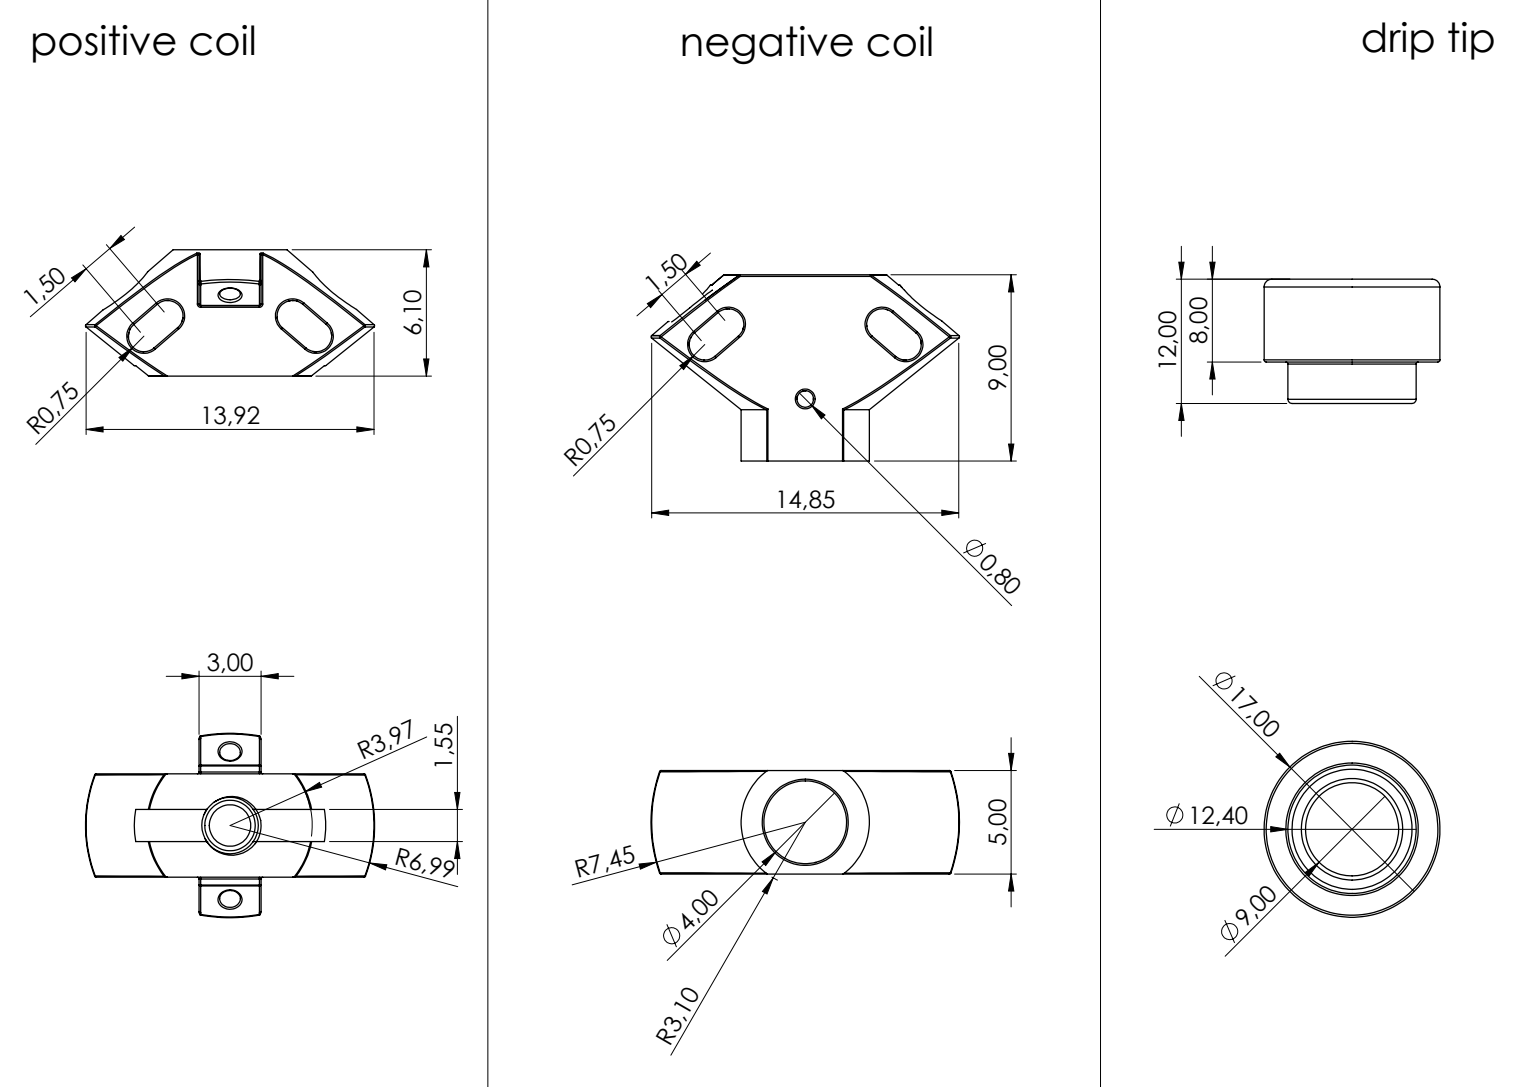
ISO-10303-21;
HEADER;
FILE_DESCRIPTION (('STEP AP214'),
    '1' );
FILE_NAME ('negative coil.step',
    '2026-10-05T20:10:51',
    ( '' ),
    ( '' ),
    'SwSTEP 2.0',
    'SolidWorks 2020',
    '' );
FILE_SCHEMA (( 'AUTOMOTIVE_DESIGN' ));
ENDSEC;

DATA;
#7=CARTESIAN_POINT ( 'NONE',  ( -7.144220599758281054, 7.299621885998258897, 0.7998128361456341429 ) ) ;
#9=CARTESIAN_POINT ( 'NONE',  ( 6.873057527484919937, 6.983264968346048818, 0.7998128361456352531 ) ) ;
#14=CARTESIAN_POINT ( 'NONE',  ( -4.828112100242303306, 4.805421336470338645, -0.7216878364870338292 ) ) ;
#18=CARTESIAN_POINT ( 'NONE',  ( 1.833030277982334422, 2.531131934864056632, -2.500000000000000444 ) ) ;
#23=CARTESIAN_POINT ( 'NONE',  ( -0.4770184558378520734, 2.994739774722604331, -1.942553401570029203 ) ) ;
#37=EDGE_LOOP ( 'NONE', ( #180346, #201044, #89611 ) ) ;
#40=CARTESIAN_POINT ( 'NONE',  ( 4.719646871332936477, 8.520355426614829142, -0.7216878364870357165 ) ) ;
#44=VERTEX_POINT ( 'NONE', #43221 ) ;
#53=CARTESIAN_POINT ( 'NONE',  ( -3.797692425603673705, 6.484372692295976570, 1.082531754730549967 ) ) ;
#55=CARTESIAN_POINT ( 'NONE',  ( 6.710359684120930091, 6.793450817754725257, 0.7998128361456352531 ) ) ;
#59=CARTESIAN_POINT ( 'NONE',  ( -4.167152111353897403, 5.955039778036558040, 1.599625672291270506 ) ) ;
#70=LINE ( 'NONE', #134411, #196122 ) ;
#72=CARTESIAN_POINT ( 'NONE',  ( 6.658462837642789012, 9.821938173008357253, 1.082531754730549078 ) ) ;
#83=ORIENTED_EDGE ( 'NONE', *, *, #112082, .F. ) ;
#101=CARTESIAN_POINT ( 'NONE',  ( 4.553559489343365740, 6.405848385690952718, -1.599625672291269396 ) ) ;
#107=CARTESIAN_POINT ( 'NONE',  ( -5.600926855776882540, 8.588146194164741232, -1.082531754730549967 ) ) ;
#108=DIRECTION ( 'NONE',  ( 0.000000000000000000, 0.000000000000000000, -1.000000000000000000 ) ) ;
#113=CARTESIAN_POINT ( 'NONE',  ( -4.911796789900812144, 8.952456364851418158, 0.7998128361456291469 ) ) ;
#119=ORIENTED_EDGE ( 'NONE', *, *, #79643, .F. ) ;
#122=CARTESIAN_POINT ( 'NONE',  ( -5.956828388357799042, 8.042995434541133193, 1.599625672291263179 ) ) ;
#125=CARTESIAN_POINT ( 'NONE',  ( 5.720439131930858956, 7.397432110343761025, 1.315134405782365956 ) ) ;
#128=CARTESIAN_POINT ( 'NONE',  ( 2.969872605471105320, 6.605953636083950364, 7.500000000000000000 ) ) ;
#130=CARTESIAN_POINT ( 'NONE',  ( 5.833751235630055376, 10.02806988486892514, 0.7998128361456331437 ) ) ;
#137=ADVANCED_FACE ( 'NONE', ( #75695 ), #126301, .T. ) ;
#139=CARTESIAN_POINT ( 'NONE',  ( -4.817943484809863008, 6.714296380401858499, 1.599625672291263179 ) ) ;
#143=CARTESIAN_POINT ( 'NONE',  ( -5.586841817283045408, 8.675676665875643678, 1.199719254218454489 ) ) ;
#147=CARTESIAN_POINT ( 'NONE',  ( 7.038091138825468107, 8.344099429118761790, -1.082531754730548412 ) ) ;
#149=CARTESIAN_POINT ( 'NONE',  ( -7.390603132780803719, 7.794994207765291172, -0.7216878364870338292 ) ) ;
#155=CARTESIAN_POINT ( 'NONE',  ( 4.667750024854814050, 8.667735138964429709, -0.7998128361456381397 ) ) ;
#169=CARTESIAN_POINT ( 'NONE',  ( 6.425920342564602983, 6.885296541689900351, -0.7293792964763821107 ) ) ;
#182=ORIENTED_EDGE ( 'NONE', *, *, #184994, .T. ) ;
#184=CARTESIAN_POINT ( 'NONE',  ( 4.649081266440608928, 8.305916344280937835, -0.4560373724170601606 ) ) ;
#196=CARTESIAN_POINT ( 'NONE',  ( -5.495582220874787538, 7.482514367559947033, -1.250084184017367539 ) ) ;
#210=DIRECTION ( 'NONE',  ( 0.000000000000000000, 0.000000000000000000, 1.000000000000000000 ) ) ;
#214=CARTESIAN_POINT ( 'NONE',  ( -3.644109427023046521, 7.473487774827342278, 0.000000000000000000 ) ) ;
#228=CARTESIAN_POINT ( 'NONE',  ( 4.505052181490820651, 8.477920988373101707, -0.7998128361456381397 ) ) ;
#229=CARTESIAN_POINT ( 'NONE',  ( -7.015401035077363900, 6.062865449010541141, 2.437084766375292144 ) ) ;
#231=CARTESIAN_POINT ( 'NONE',  ( 5.790741006368192778, 8.809596036521288198, -1.082531754730548412 ) ) ;
#247=CARTESIAN_POINT ( 'NONE',  ( -6.771371375382467583, 6.864631124226471037, -0.7998128361456362523 ) ) ;
#248=CARTESIAN_POINT ( 'NONE',  ( 4.146814880933355596, 5.931313009212638931, 1.599625672291261402 ) ) ;
#257=CARTESIAN_POINT ( 'NONE',  ( -6.563028877466991595, 9.814561569423593923, 1.199719254218452935 ) ) ;
#258=CARTESIAN_POINT ( 'NONE',  ( 6.099189001301251523, 8.209082816308541197, 1.599625672291268286 ) ) ;
#260=CARTESIAN_POINT ( 'NONE',  ( -6.387350227218078658, 6.552219065260997510, -2.500000000001207923 ) ) ;
#265=CARTESIAN_POINT ( 'NONE',  ( 5.391302360089590628, 6.318882837306503575, -1.199719254218452047 ) ) ;
#266=AXIS2_PLACEMENT_3D ( 'NONE', #151063, #68698, #100160 ) ;
#271=CARTESIAN_POINT ( 'NONE',  ( -6.579637281422358264, 6.781222396613637571, 0.3437121870633503828 ) ) ;
#281=CARTESIAN_POINT ( 'NONE',  ( -7.391130018105325661, 8.652015104991543026, -1.199719254218452047 ) ) ;
#310=CARTESIAN_POINT ( 'NONE',  ( 6.249382461256315580, 6.255644057745969988, -0.7998128361456481317 ) ) ;
#330=CARTESIAN_POINT ( 'NONE',  ( 4.797606254389322089, 6.690569611577942943, 1.599625672291268286 ) ) ;
#331=CARTESIAN_POINT ( 'NONE',  ( -3.363831509966363598, 5.978201624052440266, -1.082531754730548412 ) ) ;
#356=CARTESIAN_POINT ( 'NONE',  ( -6.791708605802965870, 6.888357893050385705, -0.7998128361456362523 ) ) ;
#358=CARTESIAN_POINT ( 'NONE',  ( 5.194182247366861738, 9.073980031987776584, 0.7216878364870317197 ) ) ;
#363=CARTESIAN_POINT ( 'NONE',  ( -5.336015975430226099, 8.383046517047350932, -1.199719254218453823 ) ) ;
#367=CARTESIAN_POINT ( 'NONE',  ( 2.915646864528636417, 6.623614785250545367, 0.2169541561525832329 ) ) ;
#371=CARTESIAN_POINT ( 'NONE',  ( -6.343235766347277149, 8.493804042195527870, -1.599625672291271394 ) ) ;
#378=CARTESIAN_POINT ( 'NONE',  ( 2.905190055078214595, 6.611415174225076186, 0.7998128361456271485 ) ) ;
#381=EDGE_CURVE ( 'NONE', #182271, #52415, #178195, .T. ) ;
#384=CARTESIAN_POINT ( 'NONE',  ( -4.610654757099099221, 7.536791762327691657, 1.199719254218452935 ) ) ;
#388=CARTESIAN_POINT ( 'NONE',  ( -6.834718835064852449, 8.106831741398025315, 1.082531754730549078 ) ) ;
#390=CARTESIAN_POINT ( 'NONE',  ( -7.227905289416804102, 8.565549271475310533, -1.082531754730549967 ) ) ;
#391=CARTESIAN_POINT ( 'NONE',  ( 7.201315867513990554, 8.430565262634994284, -1.199719254218452047 ) ) ;
#392=EDGE_CURVE ( 'NONE', #179985, #120674, #60482, .T. ) ;
#393=CARTESIAN_POINT ( 'NONE',  ( -4.977251789548269301, 4.979417640660637190, 0.7216878364870257245 ) ) ;
#395=CARTESIAN_POINT ( 'NONE',  ( -4.787437639401290745, 6.678706227425192488, 0.000000000000000000 ) ) ;
#411=CARTESIAN_POINT ( 'NONE',  ( -1.886825320689270225, 2.480000000000016858, -2.459652456995881753 ) ) ;
#412=CARTESIAN_POINT ( 'NONE',  ( 6.218145995260431214, 7.027935176161393294, 1.016989286988238206 ) ) ;
#433=CARTESIAN_POINT ( 'NONE',  ( 5.647444738788365726, 7.344714329438926548, -1.230740020431456028 ) ) ;
#436=B_SPLINE_CURVE_WITH_KNOTS ( 'NONE', 3,
 ( #78019, #42351, #109537, #112728, #74835, #144144, #160344, #111660 ),
 .UNSPECIFIED., .F., .F.,
 ( 4, 2, 2, 4 ),
 ( 0.0006312381939941720749, 0.001000335483781913384, 0.001184884128675783984, 0.001369432773569654585 ),
 .UNSPECIFIED. ) ;
#448=CARTESIAN_POINT ( 'NONE',  ( 6.339319342841494453, 9.553567112360518365, -1.199719254218452047 ) ) ;
#451=CARTESIAN_POINT ( 'NONE',  ( -5.492988512192097161, 6.437516681426083132, 1.199719254218452935 ) ) ;
#465=CARTESIAN_POINT ( 'NONE',  ( 3.898851692381625877, 6.706354853490643642, -1.199719254218452047 ) ) ;
#467=CARTESIAN_POINT ( 'NONE',  ( 5.332099551924443404, 9.442809587212341427, 0.000000000000000000 ) ) ;
#474=CARTESIAN_POINT ( 'NONE',  ( -6.902509602688821744, 8.185920970292658083, -1.082531754730549967 ) ) ;
#475=EDGE_LOOP ( 'NONE', ( #184370, #199799, #47164, #11058, #211319, #194077, #40319, #83, #128481 ) ) ;
#480=CARTESIAN_POINT ( 'NONE',  ( 6.176621499477501054, 9.363752961769195693, -1.199719254218452047 ) ) ;
#493=CARTESIAN_POINT ( 'NONE',  ( -5.722950238744243023, 7.770137593325314285, 1.443375672974058777 ) ) ;
#494=CARTESIAN_POINT ( 'NONE',  ( 5.722950238744211937, 5.849399164722627553, 0.7216878364870328300 ) ) ;
#500=DIRECTION ( 'NONE',  ( 0.000000000000000000, 0.000000000000000000, -1.000000000000000000 ) ) ;
#504=CARTESIAN_POINT ( 'NONE',  ( -4.604929450496978660, 5.401447776115099408, -1.199719254218453823 ) ) ;
#505=CARTESIAN_POINT ( 'NONE',  ( -6.455090533882201775, 8.624301270986276080, -1.443375672974066548 ) ) ;
#509=CARTESIAN_POINT ( 'NONE',  ( 4.543390873910903238, 7.354354215321133204, 1.082531754730548412 ) ) ;
#512=VERTEX_POINT ( 'NONE', #98341 ) ;
#526=CARTESIAN_POINT ( 'NONE',  ( -3.793249116773374396, 7.647484079536056356, 0.7998128361456352531 ) ) ;
#539=CARTESIAN_POINT ( 'NONE',  ( 5.063044020060520900, 4.871582543017558109, 0.7998128361456352531 ) ) ;
#543=ORIENTED_EDGE ( 'NONE', *, *, #68702, .T. ) ;
#578=CARTESIAN_POINT ( 'NONE',  ( 3.770576118376296471, 7.413106214832098750, 0.7216878364870257245 ) ) ;
#584=CARTESIAN_POINT ( 'NONE',  ( 3.702785349863636277, 7.334016984900627811, -0.7216878364870338292 ) ) ;
#597=CARTESIAN_POINT ( 'NONE',  ( -5.550083779947821760, 7.568460058062819407, -1.599625672291271394 ) ) ;
#603=B_SPLINE_CURVE_WITH_KNOTS ( 'NONE', 3,
 ( #59694, #174549, #207007, #60764, #12005, #143131 ),
 .UNSPECIFIED., .F., .F.,
 ( 4, 2, 4 ),
 ( 4.610090873601661862E-18, 9.933499788398740429E-05, 0.0001986699957679714476 ),
 .UNSPECIFIED. ) ;
#606=CARTESIAN_POINT ( 'NONE',  ( 6.556249800660121529, 9.806652646482286073, 1.199719254218452047 ) ) ;
#612=CARTESIAN_POINT ( 'NONE',  ( -6.749980374757255319, 8.968339418673846097, 1.599625672291269396 ) ) ;
#618=CARTESIAN_POINT ( 'NONE',  ( -6.617788377246204945, 6.893376992974917350, -0.7216878364870338292 ) ) ;
#622=CARTESIAN_POINT ( 'NONE',  ( -6.720001414228860881, 7.869031733802326123, -1.199719254218452047 ) ) ;
#627=AXIS2_PLACEMENT_3D ( 'NONE', #201676, #53323, #188656 ) ;
#646=CARTESIAN_POINT ( 'NONE',  ( -7.228432174741334038, 8.462200954400218578, -1.199719254218452047 ) ) ;
#647=CARTESIAN_POINT ( 'NONE',  ( 4.543917759235442944, 5.330267469643351852, 1.199719254218452935 ) ) ;
#649=CARTESIAN_POINT ( 'NONE',  ( -5.387385936583832802, 7.378645907471495846, -1.599625672291271394 ) ) ;
#676=CARTESIAN_POINT ( 'NONE',  ( -6.583366107887490770, 9.838288338247510367, 1.199719254218452935 ) ) ;
#696=DIRECTION ( 'NONE',  ( 0.000000000000000000, 0.000000000000000000, 1.000000000000000000 ) ) ;
#705=CARTESIAN_POINT ( 'NONE',  ( 3.413620815590684199, 7.204584394822967752, 0.7998128361456281477 ) ) ;
#717=CARTESIAN_POINT ( 'NONE',  ( 4.763071791759735163, 8.170823326046956936, 0.7639991172946744014 ) ) ;
#720=CARTESIAN_POINT ( 'NONE',  ( 4.848976215542928792, 5.686169002002086970, 1.199719254218452047 ) ) ;
#725=CARTESIAN_POINT ( 'NONE',  ( -5.448397627845328550, 7.449826213943242514, 1.599625672291263179 ) ) ;
#737=CARTESIAN_POINT ( 'NONE',  ( 6.590672070018850803, 7.822110515511036866, -1.082531754730548412 ) ) ;
#740=CARTESIAN_POINT ( 'NONE',  ( -5.822300622425855110, 5.757381912443740646, 0.7998128361456281477 ) ) ;
#751=CARTESIAN_POINT ( 'NONE',  ( 4.041212305325117882, 6.872442235258051646, -1.199719254218448494 ) ) ;
#752=CARTESIAN_POINT ( 'NONE',  ( 4.248501033035879004, 6.049946853332221153, -1.599625672291273171 ) ) ;
#758=VERTEX_POINT ( 'NONE', #154712 ) ;
#770=CARTESIAN_POINT ( 'NONE',  ( -5.570361349191150779, 5.866663122702686195, 0.5491554309224304653 ) ) ;
#774=CARTESIAN_POINT ( 'NONE',  ( 0.000000000000000000, 0.000000000000000000, 0.000000000000000000 ) ) ;
#776=CARTESIAN_POINT ( 'NONE',  ( 6.481679955784983349, 9.719654494127929922, -1.199719254218452047 ) ) ;
#783=CARTESIAN_POINT ( 'NONE',  ( 6.204791576909545192, 7.267953590263130259, -1.199719254218452047 ) ) ;
#790=CARTESIAN_POINT ( 'NONE',  ( 3.757017964762656703, 7.397288368949487491, -1.734723475976807094E-15 ) ) ;
#793=CARTESIAN_POINT ( 'NONE',  ( 5.709392085130549077, 9.675058176045386205, 0.000000000000000000 ) ) ;
#805=CARTESIAN_POINT ( 'NONE',  ( -6.292392690518209264, 8.434487120394948079, -1.443375672974066548 ) ) ;
#824=VERTEX_POINT ( 'NONE', #187194 ) ;
#825=ADVANCED_FACE ( 'NONE', ( #183991 ), #39943, .T. ) ;
#846=CARTESIAN_POINT ( 'NONE',  ( 6.964048179274811012, 8.153752959689313684, 1.199719254218452047 ) ) ;
#848=CARTESIAN_POINT ( 'NONE',  ( 6.225128807330042591, 7.291680359087043151, -1.199719254218452047 ) ) ;
#862=CARTESIAN_POINT ( 'NONE',  ( -5.483346782084204563, 5.361935765378481378, 0.000000000000000000 ) ) ;
#864=CARTESIAN_POINT ( 'NONE',  ( 6.360183458142179447, 6.592837920686898556, -0.7216878364870458196 ) ) ;
#874=CARTESIAN_POINT ( 'NONE',  ( -5.496904935697871863, 5.377753611261092637, 0.7998128361456281477 ) ) ;
#880=CARTESIAN_POINT ( 'NONE',  ( -7.105881907338169157, 8.423188659050232729, -1.082531754730549967 ) ) ;
#882=CARTESIAN_POINT ( 'NONE',  ( -5.478903473698268023, 5.564677938835638216, -0.7216878364870338292 ) ) ;
#908=CARTESIAN_POINT ( 'NONE',  ( -5.517242166118370150, 5.401480380085008193, 0.7998128361456281477 ) ) ;
#920=CARTESIAN_POINT ( 'NONE',  ( -5.476171693740270463, 7.594609835490887306, -1.347918582746489902 ) ) ;
#941=CARTESIAN_POINT ( 'NONE',  ( 7.062871678076271920, 7.204714810702593120, -0.7998128361456341429 ) ) ;
#961=EDGE_CURVE ( 'NONE', #137116, #194727, #203846, .T. ) ;
#964=CARTESIAN_POINT ( 'NONE',  ( 5.155843554946782703, 9.237177590738404831, -0.7998128361456481317 ) ) ;
#965=CARTESIAN_POINT ( 'NONE',  ( 6.249382461256315580, 6.255644057745969988, -0.7998128361456481317 ) ) ;
#967=CARTESIAN_POINT ( 'NONE',  ( 4.716257332707354699, 6.595662536282280719, -1.599625672291269396 ) ) ;
#978=FACE_OUTER_BOUND ( 'NONE', #59802, .T. ) ;
#979=CARTESIAN_POINT ( 'NONE',  ( 5.819104682239041537, 7.212836251160942957, -1.171789181936284896 ) ) ;
#981=CARTESIAN_POINT ( 'NONE',  ( -6.414416072596849538, 7.616478518518682073, -1.082531754730549967 ) ) ;
#982=CARTESIAN_POINT ( 'NONE',  ( 3.757017964762656703, 7.397288368949487491, -1.734723475976807094E-15 ) ) ;
#1007=CARTESIAN_POINT ( 'NONE',  ( 5.529746549527311039, 7.544733289238903851, -1.599625672291281386 ) ) ;
#1008=CARTESIAN_POINT ( 'NONE',  ( 3.549202351727371862, 7.362762853649070571, -0.7998128361456362523 ) ) ;
#1015=CARTESIAN_POINT ( 'NONE',  ( -6.966220764712169000, 6.002124920821316323, -2.420000000000000373 ) ) ;
#1024=DIRECTION ( 'NONE',  ( -1.000000000000000000, 0.000000000000000000, 0.000000000000000000 ) ) ;
#1027=CARTESIAN_POINT ( 'NONE',  ( -5.030511086842778923, 7.205508557346677279, -1.253558018337496582 ) ) ;
#1033=FACE_OUTER_BOUND ( 'NONE', #150305, .T. ) ;
#1038=CARTESIAN_POINT ( 'NONE',  ( 7.679767667498067496, 7.924426798361372093, 0.000000000000000000 ) ) ;
#1042=CARTESIAN_POINT ( 'NONE',  ( -6.466610638350029916, 6.780223854948245865, 0.3187201834274414058 ) ) ;
#1043=CARTESIAN_POINT ( 'NONE',  ( 7.225569521440261767, 7.394528961293920233, -0.7998128361456341429 ) ) ;
#1077=CARTESIAN_POINT ( 'NONE',  ( -6.794571259104023930, 7.956029886156682274, 1.199719254218452047 ) ) ;
#1079=CARTESIAN_POINT ( 'NONE',  ( 7.686546744304875389, 7.932335721302671949, 0.7998128361456291469 ) ) ;
#1094=CARTESIAN_POINT ( 'NONE',  ( 0.001041342783940506700, 2.586899276670884262, -2.002406093249768926 ) ) ;
#1100=EDGE_CURVE ( 'NONE', #39859, #170847, #133352, .T. ) ;
#1104=CARTESIAN_POINT ( 'NONE',  ( 5.643937085038755797, 9.806620042512378177, -0.7998128361456481317 ) ) ;
#1113=CARTESIAN_POINT ( 'NONE',  ( 6.129694847154206983, 8.244672969803623630, -1.443375672974078761 ) ) ;
#1126=CARTESIAN_POINT ( 'NONE',  ( -4.258669648468323743, 6.061810238003387141, 1.443375672974065660 ) ) ;
#1128=CARTESIAN_POINT ( 'NONE',  ( 6.384963997392946844, 6.413822516572072807, 0.7998128361456352531 ) ) ;
#1133=CARTESIAN_POINT ( 'NONE',  ( -5.191846479390389568, 5.021852078902356631, 0.7998128361456281477 ) ) ;
#1137=( BOUNDED_CURVE ( )  B_SPLINE_CURVE ( 2, ( #18392, #113862, #32530, #15194, #48792, #82334, #130120 ),
 .UNSPECIFIED., .F., .T. ) 
 B_SPLINE_CURVE_WITH_KNOTS ( ( 3, 2, 2, 3 ),
 ( 0.3749999999999998890, 0.3833333333333333592, 0.3916666666666668295, 0.4000000000000002998 ),
 .UNSPECIFIED. ) 
 CURVE ( )  GEOMETRIC_REPRESENTATION_ITEM ( )  RATIONAL_B_SPLINE_CURVE ( ( 1.000000000000001776, 0.8660254037844369313, 1.000000000000000000, 0.8660254037844387076, 1.000000000000000000, 0.8660254037844342667, 1.000000000000004441 ) ) 
 REPRESENTATION_ITEM ( '' )  );
#1178=CARTESIAN_POINT ( 'NONE',  ( 3.217027588192558074, 6.975225629525113824, -1.734723475976807094E-15 ) ) ;
#1180=CARTESIAN_POINT ( 'NONE',  ( -5.472651281771599763, 6.413789912602166687, 1.199719254218452935 ) ) ;
#1184=CARTESIAN_POINT ( 'NONE',  ( -6.251718229232857915, 7.426664367927358512, -1.082531754730549967 ) ) ;
#1189=CARTESIAN_POINT ( 'NONE',  ( -6.505933609711270549, 8.683618192786854095, -1.599625672291271394 ) ) ;
#1197=CARTESIAN_POINT ( 'NONE',  ( -6.200875153403786477, 8.327716660428123419, -1.599625672291271394 ) ) ;
#1200=CARTESIAN_POINT ( 'NONE',  ( 5.098657496608274720, 7.938328561423579011, 1.202842226815619142 ) ) ;
#1205=CARTESIAN_POINT ( 'NONE',  ( 5.345657705538078730, 9.458627433094950021, 0.7998128361456331437 ) ) ;
#1211=DIRECTION ( 'NONE',  ( 0.000000000000000000, 0.000000000000000000, 1.000000000000000000 ) ) ;
#1212=CARTESIAN_POINT ( 'NONE',  ( -3.983063267364693960, 7.868933921892603323, -0.7998128361456481317 ) ) ;
#1216=CARTESIAN_POINT ( 'NONE',  ( -5.749539660647037032, 8.865490816466966351, 1.199719254218454489 ) ) ;
#1223=CARTESIAN_POINT ( 'NONE',  ( -7.878696662872776812, 8.364436659539265406, -0.7216878364870338292 ) ) ;
#1229=CARTESIAN_POINT ( 'NONE',  ( 6.717138760927786834, 6.801359740696030443, -0.7998128361456481317 ) ) ;
#1243=CARTESIAN_POINT ( 'NONE',  ( 5.763319317650291040, 7.363698819737331647, -1.304181885133362195 ) ) ;
#1274=CARTESIAN_POINT ( 'NONE',  ( -5.386282318077409315, 7.574627448853999745, -1.244059264865501557 ) ) ;
#1291=CARTESIAN_POINT ( 'NONE',  ( -4.980641328173854632, 6.904110530993182948, 1.599625672291263179 ) ) ;
#1304=CARTESIAN_POINT ( 'NONE',  ( 6.866278450678116485, 6.975356045404744521, 0.000000000000000000 ) ) ;
#1307=CARTESIAN_POINT ( 'NONE',  ( 5.763624699140868834, 7.817591130454727200, -1.443375672974078761 ) ) ;
#1313=AXIS2_PLACEMENT_3D ( 'NONE', #163918, #211566, #65305 ) ;
#1323=CARTESIAN_POINT ( 'NONE',  ( -5.692444392891315097, 7.734547439830227411, -1.599625672291271394 ) ) ;
#1324=CARTESIAN_POINT ( 'NONE',  ( 6.703580607314123085, 6.785541894813420072, 0.000000000000000000 ) ) ;
#1333=CARTESIAN_POINT ( 'NONE',  ( -5.887983850084758330, 10.09134126839936840, 0.7998128361456291469 ) ) ;
#1334=CARTESIAN_POINT ( 'NONE',  ( 5.996449078994045223, 10.21788403546024782, 0.7998128361456331437 ) ) ;
#1336=DIRECTION ( 'NONE',  ( 0.7592566023653004592, -0.6507913734559639396, 0.000000000000000000 ) ) ;
#1340=CARTESIAN_POINT ( 'NONE',  ( 0.000000000000000000, 9.999999999999998224, -2.000000000000000000 ) ) ;
#1341=CARTESIAN_POINT ( 'NONE',  ( 3.718679271898170491, 7.560485927181699317, 0.7998128361456271485 ) ) ;
#1346=CARTESIAN_POINT ( 'NONE',  ( -6.458928793950097891, 6.861006557743732692, 0.6885227102202008398 ) ) ;
#1355=CARTESIAN_POINT ( 'NONE',  ( -4.516274566683622815, 5.401980094953223066, 1.082531754730549078 ) ) ;
#1408=CARTESIAN_POINT ( 'NONE',  ( 4.716257332707354699, 6.595662536282280719, -1.599625672291269396 ) ) ;
#1409=CARTESIAN_POINT ( 'NONE',  ( -4.394251184604987870, 5.259619482528146150, 1.082531754730549078 ) ) ;
#1433=CARTESIAN_POINT ( 'NONE',  ( -5.769876891067536206, 8.889217585290882795, 1.199719254218454489 ) ) ;
#1439=CARTESIAN_POINT ( 'NONE',  ( -4.995253251992230581, 4.792493313604505367, 0.000000000000000000 ) ) ;
#1446=CARTESIAN_POINT ( 'NONE',  ( -5.738844160334429567, 9.917344963690652548, 0.000000000000000000 ) ) ;
#1448=CARTESIAN_POINT ( 'NONE',  ( 5.011754246625688580, 8.023990808224052529, -1.135194352273690255 ) ) ;
#1453=CARTESIAN_POINT ( 'NONE',  ( 3.203469434578891661, 6.959407783642502565, -0.7998128361456362523 ) ) ;
#1458=CARTESIAN_POINT ( 'NONE',  ( -5.041653019435350380, 6.975290837464928728, -1.599625672291271394 ) ) ;
#1463=CARTESIAN_POINT ( 'NONE',  ( -6.997416678428844072, 8.296645891989347987, 1.082531754730549078 ) ) ;
#1466=CARTESIAN_POINT ( 'NONE',  ( 6.068156270568149324, 9.237210194708310951, 1.199719254218452047 ) ) ;
#1467=CARTESIAN_POINT ( 'NONE',  ( -3.919715807682309094, 6.626733304721049933, 1.082531754730549967 ) ) ;
#1485=CARTESIAN_POINT ( 'NONE',  ( -3.011287625495571607, 6.360174617139689346, -0.7852620323503290978 ) ) ;
#1486=CARTESIAN_POINT ( 'NONE',  ( 6.598740849494261873, 6.770918179921630475, -0.1579934589533253664 ) ) ;
#1495=CARTESIAN_POINT ( 'NONE',  ( 4.542476715900265916, 4.951051008190067826, -0.8264431066547142102 ) ) ;
#1505=CARTESIAN_POINT ( 'NONE',  ( 5.910429572389825026, 7.145202977605201511, -1.123150837922413547 ) ) ;
#1520=AXIS2_PLACEMENT_3D ( 'NONE', #146817, #128498, #131651 ) ;
#1524=CARTESIAN_POINT ( 'NONE',  ( -6.656127069666307072, 6.730179434224282886, 0.7998128361456341429 ) ) ;
#1538=CARTESIAN_POINT ( 'NONE',  ( 5.571474780572990504, 5.464751763615448787, 0.7998128361456352531 ) ) ;
#1540=CARTESIAN_POINT ( 'NONE',  ( 5.643937085038755797, 9.806620042512378177, -0.7998128361456481317 ) ) ;
#1541=CARTESIAN_POINT ( 'NONE',  ( -5.346851039111055748, 6.199209027673978412, -2.420000000000000373 ) ) ;
#1546=CARTESIAN_POINT ( 'NONE',  ( -7.743115126736118015, 8.206258200713163475, 0.7216878364870317197 ) ) ;
#1552=CARTESIAN_POINT ( 'NONE',  ( 6.016786309414542622, 10.24161080428416426, 0.7998128361456341429 ) ) ;
#1559=LINE ( 'NONE', #22067, #152655 ) ;
#1565=CARTESIAN_POINT ( 'NONE',  ( -6.211043768836215229, 8.339580045099285854, 1.443375672974064550 ) ) ;
#1566=CARTESIAN_POINT ( 'NONE',  ( 3.933273961740286317, 7.602920365423422311, 0.7216878364870257245 ) ) ;
#1576=CARTESIAN_POINT ( 'NONE',  ( -3.298376509874564988, 7.070132704820777825, 0.000000000000000000 ) ) ;
#1577=CARTESIAN_POINT ( 'NONE',  ( -6.956742217587851052, 7.288823140040177506, 0.000000000000000000 ) ) ;
#1581=CARTESIAN_POINT ( 'NONE',  ( 5.112833325684902341, 7.058334528089426740, -1.443375672974078761 ) ) ;
#1592=CARTESIAN_POINT ( 'NONE',  ( -5.757633847399098670, 7.274473465504208036, 1.200491007486852002 ) ) ;
#1596=CARTESIAN_POINT ( 'NONE',  ( 0.000000000000000000, 8.920000000000001705, -2.000000000000000000 ) ) ;
#1597=CARTESIAN_POINT ( 'NONE',  ( 5.085717018901939390, 5.105960408239938353, 0.000000000000000000 ) ) ;
#1601=CARTESIAN_POINT ( 'NONE',  ( -4.281342646865346602, 8.216926531310035031, 0.7998128361456352531 ) ) ;
#1614=CARTESIAN_POINT ( 'NONE',  ( 4.903208829997618423, 5.749440385532527564, -1.199719254218450271 ) ) ;
#1624=CARTESIAN_POINT ( 'NONE',  ( -3.947104627881522720, 8.980740528188976057, -0.7749999999999979128 ) ) ;
#1627=CARTESIAN_POINT ( 'NONE',  ( 2.993041990875914493, 6.420974562437304911, 0.3677586026352899218 ) ) ;
#1652=CARTESIAN_POINT ( 'NONE',  ( 5.316205630334249754, 7.295602216847000498, -1.443375672974078761 ) ) ;
#1660=CARTESIAN_POINT ( 'NONE',  ( 5.628043163004202931, 8.619781885929965526, -1.082531754730548412 ) ) ;
#1675=CARTESIAN_POINT ( 'NONE',  ( -7.442499979258930587, 7.647614495415686164, -0.7998128361456362523 ) ) ;
#1685=CARTESIAN_POINT ( 'NONE',  ( -5.029148636026397945, 4.832037928311032182, 0.7998128361456281477 ) ) ;
#1687=CARTESIAN_POINT ( 'NONE',  ( 5.194182247366881278, 5.232503174782402233, 0.7216878364870328300 ) ) ;
#1693=CARTESIAN_POINT ( 'NONE',  ( -7.449279056065764237, 7.655523418356991350, 0.7998128361456341429 ) ) ;
#1699=CARTESIAN_POINT ( 'NONE',  ( -4.326460416536637155, 8.061637896019123062, 0.000000000000000000 ) ) ;
#1702=CARTESIAN_POINT ( 'NONE',  ( -4.938913097128142304, 8.984092056616635347, -0.7998128361456362523 ) ) ;
#1721=CARTESIAN_POINT ( 'NONE',  ( -3.038435823238377687, 6.558942537171132514, -0.7216878364870458196 ) ) ;
#1723=CARTESIAN_POINT ( 'NONE',  ( -5.289089322662584358, 5.343228095960675716, 0.000000000000000000 ) ) ;
#1724=CARTESIAN_POINT ( 'NONE',  ( 3.923105346307896202, 5.670318552149568703, -1.599625672291269396 ) ) ;
#1725=CARTESIAN_POINT ( 'NONE',  ( -4.142898457427624415, 6.991076079377632091, 1.199719254218452935 ) ) ;
#1726=CARTESIAN_POINT ( 'NONE',  ( -6.791708605802965870, 6.888357893050385705, -0.7998128361456362523 ) ) ;
#1782=CARTESIAN_POINT ( 'NONE',  ( 5.435893244436359240, 5.306573304789342416, -0.7998128361456481317 ) ) ;
#1795=CARTESIAN_POINT ( 'NONE',  ( 4.599920620972065777, 8.367456947080912144, 0.1478172174028801744 ) ) ;
#1798=CARTESIAN_POINT ( 'NONE',  ( 6.536439455564150514, 9.679577560583279450, 1.082531754730549078 ) ) ;
#1802=CARTESIAN_POINT ( 'NONE',  ( -6.608673532018475960, 6.674816973635147477, -0.7998128361456362523 ) ) ;
#1807=CARTESIAN_POINT ( 'NONE',  ( -7.878696662872776812, 8.364436659539265406, -0.7216878364870338292 ) ) ;
#1815=CARTESIAN_POINT ( 'NONE',  ( 6.102578539926878598, 7.252668063737060855, -1.082531754730548412 ) ) ;
#1818=CARTESIAN_POINT ( 'NONE',  ( -6.296835998904160014, 6.311006518335105397, 0.000000000000000000 ) ) ;
#1830=CARTESIAN_POINT ( 'NONE',  ( 3.705121118284530279, 7.544668081299086282, -1.734723475976807094E-15 ) ) ;
#1831=CARTESIAN_POINT ( 'NONE',  ( 3.549202351727371862, 7.362762853649070571, -0.7998128361456362523 ) ) ;
#1851=LINE ( 'NONE', #51717, #123874 ) ;
#1854=CARTESIAN_POINT ( 'NONE',  ( 8.018721507839716267, 8.319872945426633137, -0.7998128361456341429 ) ) ;
#1862=CARTESIAN_POINT ( 'NONE',  ( 6.313256805818848960, 7.394496357324014113, 1.199719254218452047 ) ) ;
#1867=CARTESIAN_POINT ( 'NONE',  ( 3.906157654512984134, 7.571284673658201569, -0.7216878364870338292 ) ) ;
#1870=CARTESIAN_POINT ( 'NONE',  ( 6.292392690518195941, 8.434487120394948079, -1.443375672974078761 ) ) ;
#1882=CARTESIAN_POINT ( 'NONE',  ( 6.157602363183391603, 6.969851231138187941, -0.9158007892692658913 ) ) ;
#1883=CARTESIAN_POINT ( 'NONE',  ( -7.621091744657483069, 8.063897588288083895, 0.7216878364870317197 ) ) ;
#1920=CARTESIAN_POINT ( 'NONE',  ( 6.638652492546827766, 7.774124658506663010, 1.199719254218452047 ) ) ;
#1923=CARTESIAN_POINT ( 'NONE',  ( 6.526270840131753737, 8.707344961610770540, -1.599625672291283607 ) ) ;
#1936=CARTESIAN_POINT ( 'NONE',  ( -5.093022980588950865, 5.970890227889075419, -1.199719254218453823 ) ) ;
#1938=CARTESIAN_POINT ( 'NONE',  ( 4.868786560638885597, 7.733982516503781213, 1.082531754730548412 ) ) ;
#1946=CARTESIAN_POINT ( 'NONE',  ( -4.496464221587651799, 5.274905009054215554, 1.199719254218452935 ) ) ;
#1952=CARTESIAN_POINT ( 'NONE',  ( -7.770231434407805615, 8.237893892996801526, 0.000000000000000000 ) ) ;
#1953=EDGE_LOOP ( 'NONE', ( #157859, #138577, #171255, #137292, #164830, #143916, #204873, #56553, #39831, #143622, #110813, #20199, #67902, #39672 ) ) ;
#1954=CARTESIAN_POINT ( 'NONE',  ( -4.665414256878287702, 8.457084043084382330, -0.7216878364870338292 ) ) ;
#1977=CARTESIAN_POINT ( 'NONE',  ( -3.630551273409382329, 7.457669928944732796, 0.7998128361456352531 ) ) ;
#1979=DIRECTION ( 'NONE',  ( 0.7592566023653005702, -0.6507913734559639396, 0.000000000000000000 ) ) ;
#1988=CARTESIAN_POINT ( 'NONE',  ( -4.839158742459761520, 8.201312040681516535, -0.9517655008395020655 ) ) ;
#1990=CYLINDRICAL_SURFACE ( 'NONE', #71546, 1.250000000000000000 ) ;
#2005=CARTESIAN_POINT ( 'NONE',  ( 6.873057527484919937, 6.983264968346048818, 0.7998128361456352531 ) ) ;
#2026=CARTESIAN_POINT ( 'NONE',  ( 7.191674137406095291, 7.354984346587396082, 0.000000000000000000 ) ) ;
#2027=CARTESIAN_POINT ( 'NONE',  ( 4.037295881819344956, 7.932205305423046582, -0.7998128361456362523 ) ) ;
#2029=CARTESIAN_POINT ( 'NONE',  ( 4.420840606507738357, 7.315341919971147355, 1.199719254218451159 ) ) ;
#2041=CARTESIAN_POINT ( 'NONE',  ( 5.228576739797318851, 7.698598165248225378, -1.206158463488806953 ) ) ;
#2042=CARTESIAN_POINT ( 'NONE',  ( -6.278834536460198734, 6.497930845391236332, 0.7216878364870257245 ) ) ;
#2043=CARTESIAN_POINT ( 'NONE',  ( 5.451787166470912993, 6.493411461371761284, -1.082531754730548412 ) ) ;
#2055=ORIENTED_EDGE ( 'NONE', *, *, #133829, .T. ) ;
#2065=CARTESIAN_POINT ( 'NONE',  ( -4.082413651046300274, 6.816547455312373494, 1.082531754730549967 ) ) ;
#2071=CARTESIAN_POINT ( 'NONE',  ( 6.690022453700429139, 6.769724048930809701, 0.7998128361456331437 ) ) ;
#2095=CARTESIAN_POINT ( 'NONE',  ( -6.966220764712148572, 6.002124920821316323, 2.420000000000000373 ) ) ;
#2099=CARTESIAN_POINT ( 'NONE',  ( 5.182959862174088883, 9.268813282503625572, 0.7998128361456331437 ) ) ;
#2104=CARTESIAN_POINT ( 'NONE',  ( -5.349061533644712263, 7.606979636585072591, 1.237473162191610188 ) ) ;
#2105=CARTESIAN_POINT ( 'NONE',  ( 5.515134625708930649, 9.656350506627580543, 0.000000000000000000 ) ) ;
#2135=CARTESIAN_POINT ( 'NONE',  ( -6.257970421159510188, 9.458660037064859694, 1.199719254218452047 ) ) ;
#2137=CARTESIAN_POINT ( 'NONE',  ( 5.365994935958575240, 9.482354201918870018, 0.7998128361456341429 ) ) ;
#2138=CARTESIAN_POINT ( 'NONE',  ( 2.972033609136344623, 6.549060441754430251, -0.4946758370507741698 ) ) ;
#2146=FACE_OUTER_BOUND ( 'NONE', #82357, .T. ) ;
#2158=CARTESIAN_POINT ( 'NONE',  ( 7.666209513884374438, 7.908608952478760834, 0.7998128361456281477 ) ) ;
#2167=CARTESIAN_POINT ( 'NONE',  ( 6.156811154381533591, 9.236677875870187293, -1.082531754730548412 ) ) ;
#2171=CARTESIAN_POINT ( 'NONE',  ( -3.179715765502671321, 5.975770656120749535, -2.419999999999998597 ) ) ;
#2172=ORIENTED_EDGE ( 'NONE', *, *, #47152, .T. ) ;
#2182=CARTESIAN_POINT ( 'NONE',  ( -4.150204419558982671, 7.856005899545188242, 0.7216878364870338292 ) ) ;
#2185=CARTESIAN_POINT ( 'NONE',  ( 5.550083779947807550, 7.568460058062819407, -1.599625672291283607 ) ) ;
#2188=CARTESIAN_POINT ( 'NONE',  ( -7.095713291905736853, 9.371694488680407886, 1.599625672291269396 ) ) ;
#2190=CARTESIAN_POINT ( 'NONE',  ( -2.844178363816758814, 6.540234867753325076, -0.7998128361456481317 ) ) ;
#2202=CARTESIAN_POINT ( 'NONE',  ( -0.3254290916866059979, 3.359077955639389046, -1.974305197405200163 ) ) ;
#2231=CARTESIAN_POINT ( 'NONE',  ( 3.879041347285658414, 6.579279767591636130, -1.082531754730548412 ) ) ;
#2236=CARTESIAN_POINT ( 'NONE',  ( 5.174371902270911150, 6.065797303184739420, 1.199719254218452047 ) ) ;
#2239=CARTESIAN_POINT ( 'NONE',  ( -5.795184315198522285, 5.725746220678519904, -0.7998128361456362523 ) ) ;
#2240=CARTESIAN_POINT ( 'NONE',  ( -5.842637852846352509, 5.781108681267656202, 0.7998128361456282587 ) ) ;
#2243=CARTESIAN_POINT ( 'NONE',  ( -6.427974226210522168, 6.671927150099951298, 0.000000000000000000 ) ) ;
#2249=VERTEX_POINT ( 'NONE', #52631 ) ;
#2250=CARTESIAN_POINT ( 'NONE',  ( -7.273023059088104425, 7.449891421883056530, 0.000000000000000000 ) ) ;
#2255=CARTESIAN_POINT ( 'NONE',  ( 3.598535064101026748, 7.346084821328116909, 0.3627869759331026622 ) ) ;
#2256=CARTESIAN_POINT ( 'NONE',  ( 6.535912570239620578, 9.782925877658371405, 1.199719254218452047 ) ) ;
#2258=CARTESIAN_POINT ( 'NONE',  ( -6.466312919074983512, 6.508729591867735031, -0.7998128361456362523 ) ) ;
#2260=CARTESIAN_POINT ( 'NONE',  ( 5.017113787211129328, 8.018716392533608683, 1.139262206072016559 ) ) ;
#2265=CARTESIAN_POINT ( 'NONE',  ( 7.018280793729500644, 8.217024343219755167, -1.199719254218452047 ) ) ;
#2272=CARTESIAN_POINT ( 'NONE',  ( -3.467853430045390706, 7.267855778353407459, 0.7998128361456352531 ) ) ;
#2276=CARTESIAN_POINT ( 'NONE',  ( -6.557303570864871034, 7.679217583210999010, -1.199719254218452047 ) ) ;
#2280=CARTESIAN_POINT ( 'NONE',  ( 6.902509602688803980, 9.146290184594002781, -1.443375672974064550 ) ) ;
#2282=CARTESIAN_POINT ( 'NONE',  ( -7.417719440008134768, 7.826629899530511025, 0.7216878364870317197 ) ) ;
#2288=CARTESIAN_POINT ( 'NONE',  ( 5.773793314573267388, 7.829454515125894964, 1.599625672291268286 ) ) ;
#2304=CARTESIAN_POINT ( 'NONE',  ( 5.862225131719664972, 7.287605523280396902, -1.268052015211480033 ) ) ;
#2324=ADVANCED_FACE ( 'NONE', ( #36371 ), #212046, .T. ) ;
#2333=CARTESIAN_POINT ( 'NONE',  ( -6.444026653998019327, 6.794751805161505231, -0.4079633569072909638 ) ) ;
#2352=CARTESIAN_POINT ( 'NONE',  ( -3.820365424000704557, 7.679119771301277098, -0.7998128361456481317 ) ) ;
#2366=VERTEX_POINT ( 'NONE', #89981 ) ;
#2367=CARTESIAN_POINT ( 'NONE',  ( 7.367930134383754215, 7.560616343061329125, -0.7998128361456341429 ) ) ;
#2368=CARTESIAN_POINT ( 'NONE',  ( 3.464990776744291345, 6.200183785247111778, 1.199719254218452047 ) ) ;
#2370=CARTESIAN_POINT ( 'NONE',  ( 7.485510208076452621, 7.905719128943566432, 0.000000000000000000 ) ) ;
#2378=TOROIDAL_SURFACE ( 'NONE', #154552, 2.080000000000000071, 0.08000000000000000167 ) ;
#2384=CARTESIAN_POINT ( 'NONE',  ( -6.120580001926503755, 6.105374521861167914, -0.7998128361456362523 ) ) ;
#2385=CARTESIAN_POINT ( 'NONE',  ( 5.554000203453580475, 6.508696987897830688, -1.199719254218452047 ) ) ;
#2393=CARTESIAN_POINT ( 'NONE',  ( -7.208094944320834863, 8.438474185576302133, -1.199719254218452047 ) ) ;
#2394=CARTESIAN_POINT ( 'NONE',  ( 6.912678218121202534, 9.158153569265168770, 1.599625672291268286 ) ) ;
#2401=CARTESIAN_POINT ( 'NONE',  ( 4.549643065837591038, 7.465611455855944101, -1.199719254218452047 ) ) ;
#2409=CARTESIAN_POINT ( 'NONE',  ( -4.709679585977568195, 8.347295923589904021, 0.7007048023343342980 ) ) ;
#2419=CARTESIAN_POINT ( 'NONE',  ( -2.997761361953021009, 6.511488999004883205, -0.7216878364870458196 ) ) ;
#2422=CARTESIAN_POINT ( 'NONE',  ( -6.966220764712148572, 6.002124920821316323, 2.500000000000000444 ) ) ;
#2427=CARTESIAN_POINT ( 'NONE',  ( 3.255366281057017197, 6.812028071292901998, -0.7216878364870338292 ) ) ;
#2467=CARTESIAN_POINT ( 'NONE',  ( 4.370663978927085580, 5.060324124126027279, -1.009771797811724214 ) ) ;
#2469=ADVANCED_FACE ( 'NONE', ( #168689 ), #64454, .T. ) ;
#2470=CARTESIAN_POINT ( 'NONE',  ( 3.542423274920540432, 7.354853930707762721, -1.734723475976807094E-15 ) ) ;
#2471=CARTESIAN_POINT ( 'NONE',  ( -5.641601317062259646, 5.754492089426966217, -0.7216878364870338292 ) ) ;
#2497=CARTESIAN_POINT ( 'NONE',  ( -5.094831863685302942, 9.165997284266655498, 0.7998128361456291469 ) ) ;
#2499=CARTESIAN_POINT ( 'NONE',  ( 7.309254211098760834, 8.660456346770972758, 1.082531754730549967 ) ) ;
#2505=CARTESIAN_POINT ( 'NONE',  ( -5.157951095356222204, 4.982307464195829816, 0.000000000000000000 ) ) ;
#2512=CARTESIAN_POINT ( 'NONE',  ( -5.641074431737709283, 8.738948049406083385, -1.199719254218452047 ) ) ;
#2519=CARTESIAN_POINT ( 'NONE',  ( 4.523580528814945545, 5.306540700819438960, 1.199719254218452047 ) ) ;
#2524=CARTESIAN_POINT ( 'NONE',  ( -5.692444392891315097, 7.734547439830227411, -1.599625672291271394 ) ) ;
#2528=CARTESIAN_POINT ( 'NONE',  ( -5.912764389335557702, 8.951956649983198844, 1.082531754730550855 ) ) ;
#2531=CARTESIAN_POINT ( 'NONE',  ( 5.031484404002891431, 5.042689024191078673, 0.7216878364870328300 ) ) ;
#2532=CARTESIAN_POINT ( 'NONE',  ( -6.071018923869249129, 10.30488218781460574, 0.7998128361456291469 ) ) ;
#2551=CARTESIAN_POINT ( 'NONE',  ( 6.468016842275610578, 6.857101109195174793, 0.6445861549769070775 ) ) ;
#2557=PLANE ( 'NONE',  #139685 ) ;
#2564=B_SPLINE_CURVE_WITH_KNOTS ( 'NONE', 3,
 ( #171227, #154989, #56421, #6574 ),
 .UNSPECIFIED., .F., .F.,
 ( 4, 4 ),
 ( 5.038702538383248430E-05, 0.0001172081591904372197 ),
 .UNSPECIFIED. ) ;
#2576=CARTESIAN_POINT ( 'NONE',  ( 5.488371254093075358, 7.473176909139983337, -1.250075884424824757 ) ) ;
#2592=CARTESIAN_POINT ( 'NONE',  ( 7.526711554241970248, 8.810193563817646734, -1.199719254218452047 ) ) ;
#2595=CARTESIAN_POINT ( 'NONE',  ( -4.932134020321308654, 8.976183133675331050, 0.7998128361456291469 ) ) ;
#2608=CARTESIAN_POINT ( 'NONE',  ( 4.603875680292229156, 7.528882839386387360, 1.199719254218452047 ) ) ;
#2615=CARTESIAN_POINT ( 'NONE',  ( -7.227905289416814760, 7.605180057173966723, -0.7216878364870338292 ) ) ;
#2620=CARTESIAN_POINT ( 'NONE',  ( 5.352436782344940802, 9.466536356036257871, 0.000000000000000000 ) ) ;
#2631=CARTESIAN_POINT ( 'NONE',  ( -6.048345925472225382, 8.149765894507963182, 1.443375672974058777 ) ) ;
#2632=CARTESIAN_POINT ( 'NONE',  ( 5.221298555038576872, 9.105615724271411082, 0.000000000000000000 ) ) ;
#2643=CARTESIAN_POINT ( 'NONE',  ( -4.767627293860968507, 5.591261926706423857, -1.199719254218453823 ) ) ;
#2644=CARTESIAN_POINT ( 'NONE',  ( -4.065465959251405081, 5.836405933916976707, -1.599625672291271394 ) ) ;
#2647=CARTESIAN_POINT ( 'NONE',  ( 4.353576723319599218, 8.093273587265928271, -0.7216878364870357165 ) ) ;
#2660=CARTESIAN_POINT ( 'NONE',  ( -6.370507937826336509, 6.842553425211714391, 0.6026486057824770315 ) ) ;
#2665=CARTESIAN_POINT ( 'NONE',  ( 4.638297949650961982, 5.544340708415133712, -1.082531754730548412 ) ) ;
#2668=CARTESIAN_POINT ( 'NONE',  ( -4.793689830883590020, 7.750332681742931662, 1.199719254218452935 ) ) ;
#2682=CARTESIAN_POINT ( 'NONE',  ( 5.551137550152489553, 5.441024994791534120, 0.7998128361456352531 ) ) ;
#2693=CARTESIAN_POINT ( 'NONE',  ( 5.346851039111029991, 6.199209027673978412, 7.500000000000000000 ) ) ;
#2719=CARTESIAN_POINT ( 'NONE',  ( 4.421367491832258523, 8.172362817197399210, 0.7216878364870257245 ) ) ;
#2724=CARTESIAN_POINT ( 'NONE',  ( 6.658462837642799670, 7.901199744405670522, 1.082531754730549967 ) ) ;
#2739=CARTESIAN_POINT ( 'NONE',  ( -5.582925393777276035, 9.735439736040634173, 0.7998128361456291469 ) ) ;
#2750=CARTESIAN_POINT ( 'NONE',  ( 5.031484404002889654, 6.003058238492422483, 1.082531754730549078 ) ) ;
#2757=CARTESIAN_POINT ( 'NONE',  ( -6.720001414228860881, 7.869031733802326123, -1.199719254218452047 ) ) ;
#2762=CARTESIAN_POINT ( 'NONE',  ( -5.560252395380252288, 7.580323442733986283, 1.443375672974058777 ) ) ;
#2765=CARTESIAN_POINT ( 'NONE',  ( -5.250750630242457362, 9.347902511916677426, 0.000000000000000000 ) ) ;
#2785=CARTESIAN_POINT ( 'NONE',  ( -2.875737979874388284, 6.369128386579808954, -0.7216878364870458196 ) ) ;
#2787=CARTESIAN_POINT ( 'NONE',  ( -3.811250578772977349, 7.460559751961507224, -0.7216878364870458196 ) ) ;
#2788=CARTESIAN_POINT ( 'NONE',  ( 5.899733120602060232, 6.912052057904395141, -1.199719254218452047 ) ) ;
#2789=CARTESIAN_POINT ( 'NONE',  ( -6.005335696210345020, 5.970922831858983315, 0.7998128361456281477 ) ) ;
#2790=CARTESIAN_POINT ( 'NONE',  ( -6.967964602780620353, 7.093989889524320525, 0.000000000000000000 ) ) ;
#2813=CARTESIAN_POINT ( 'NONE',  ( -7.095713291905736853, 9.371694488680407886, 1.599625672291269396 ) ) ;
#2834=DIRECTION ( 'NONE',  ( -0.6507913734559641616, -0.7592566023653004592, 0.000000000000000000 ) ) ;
#2837=CARTESIAN_POINT ( 'NONE',  ( 2.977454500823585093, 6.499579965040511276, -0.5808385047149626779 ) ) ;
#2845=CARTESIAN_POINT ( 'NONE',  ( 5.734172623936983904, 5.654565914206774124, 0.7998128361456352531 ) ) ;
#2847=CARTESIAN_POINT ( 'NONE',  ( -3.894033820048823813, 8.999999999999998224, -0.7749999999999979128 ) ) ;
#2858=CARTESIAN_POINT ( 'NONE',  ( 4.594747986498664005, 8.374059380672374431, -0.03693212167796278145 ) ) ;
#2861=CARTESIAN_POINT ( 'NONE',  ( 7.851580356089786328, 8.332800968292465527, 0.000000000000000000 ) ) ;
#2867=CARTESIAN_POINT ( 'NONE',  ( -5.367048706163331850, 7.354919138647580290, -1.599625672291271394 ) ) ;
#2879=CARTESIAN_POINT ( 'NONE',  ( 6.373741612200174878, 6.608655767087927124, 0.7216878364870328300 ) ) ;
#2882=CARTESIAN_POINT ( 'NONE',  ( -7.123883369337781879, 7.275895117174344229, 0.7998128361456341429 ) ) ;
#2893=CARTESIAN_POINT ( 'NONE',  ( 5.876533236880477240, 5.820653295974182129, 0.7998128361456352531 ) ) ;
#2894=CARTESIAN_POINT ( 'NONE',  ( 4.552505719138623341, 8.533283448962240669, 0.7998128361456341429 ) ) ;
#2917=ORIENTED_EDGE ( 'NONE', *, *, #1100, .F. ) ;
#2918=CARTESIAN_POINT ( 'NONE',  ( 5.948130214252392634, 7.161930257618140949, 1.164772078525571075 ) ) ;
#2924=CARTESIAN_POINT ( 'NONE',  ( 2.898410978271408922, 6.603506251283770112, -0.7998128361456362523 ) ) ;
#2930=CARTESIAN_POINT ( 'NONE',  ( 5.722423353419669567, 8.833855124701747386, 1.199719254218451159 ) ) ;
#2935=CARTESIAN_POINT ( 'NONE',  ( 4.082413651490639062, 7.776916670132135501, 0.000000000000000000 ) ) ;
#2938=CARTESIAN_POINT ( 'NONE',  ( 2.891631901464575272, 6.595597328342462262, 0.000000000000000000 ) ) ;
#2947=CARTESIAN_POINT ( 'NONE',  ( 4.379179108948761723, 7.028642110670195287, -1.191602461106481936 ) ) ;
#2950=CARTESIAN_POINT ( 'NONE',  ( 6.403672513108120690, 6.804938187689173468, -0.5019199613840990004 ) ) ;
#2952=CARTESIAN_POINT ( 'NONE',  ( -6.997416678428844072, 8.296645891989347987, 1.082531754730549078 ) ) ;
#2969=DIRECTION ( 'NONE',  ( 1.000000000000000000, 0.000000000000000000, 0.000000000000000000 ) ) ;
#2989=CARTESIAN_POINT ( 'NONE',  ( 7.178115983792402233, 7.339166500704784823, 0.7998128361456281477 ) ) ;
#2991=CARTESIAN_POINT ( 'NONE',  ( 7.212011367826596242, 7.378711115411311638, 0.000000000000000000 ) ) ;
#3003=CARTESIAN_POINT ( 'NONE',  ( -4.610654757099099221, 7.536791762327691657, 1.199719254218452935 ) ) ;
#3005=CARTESIAN_POINT ( 'NONE',  ( 5.194182247366868843, 8.113610817686430110, 1.082531754730548412 ) ) ;
#3013=CARTESIAN_POINT ( 'NONE',  ( -4.442231607132987925, 5.211633625523774960, -1.199719254218453823 ) ) ;
#3021=CARTESIAN_POINT ( 'NONE',  ( -6.075462232699549325, 9.141770800574526845, 1.082531754730549967 ) ) ;
#3023=CARTESIAN_POINT ( 'NONE',  ( -4.475600106286965918, 8.235634200727838916, 0.7216878364870338292 ) ) ;
#3046=CARTESIAN_POINT ( 'NONE',  ( -6.479871072688648148, 6.524547437750345402, 0.000000000000000000 ) ) ;
#3048=CYLINDRICAL_SURFACE ( 'NONE', #146909, 1.250000000000000000 ) ;
#3056=CARTESIAN_POINT ( 'NONE',  ( -4.762026763822442277, 8.287006692039220468, -0.8189809589772244491 ) ) ;
#3095=CARTESIAN_POINT ( 'NONE',  ( 5.855142236255289845, 7.924361590421551860, -1.599625672291281386 ) ) ;
#3096=CARTESIAN_POINT ( 'NONE',  ( 4.688087255275310561, 8.691461907788344377, -0.7998128361456381397 ) ) ;
#3098=CARTESIAN_POINT ( 'NONE',  ( 4.258142763143749399, 7.125527769379820242, 1.199719254218451159 ) ) ;
#3101=CARTESIAN_POINT ( 'NONE',  ( -4.064664930713566271, 3.791393346161858080, -2.445650103046228985 ) ) ;
#3110=CARTESIAN_POINT ( 'NONE',  ( 5.834480046583573554, 7.201333694826374199, -1.164487238324034557 ) ) ;
#3112=CARTESIAN_POINT ( 'NONE',  ( -6.143253000323532831, 7.300121600866474658, 1.082531754730548412 ) ) ;
#3113=CARTESIAN_POINT ( 'NONE',  ( 5.722950238744211937, 5.849399164722627553, 0.7216878364870328300 ) ) ;
#3121=EDGE_CURVE ( 'NONE', #36876, #158170, #96130, .T. ) ;
#3134=CARTESIAN_POINT ( 'NONE',  ( -6.414416072596857532, 6.656109304217339151, -0.7216878364870338292 ) ) ;
#3139=CARTESIAN_POINT ( 'NONE',  ( 6.801350335910821165, 7.963938809097990124, 1.199719254218452047 ) ) ;
#3162=CARTESIAN_POINT ( 'NONE',  ( -5.398914348987532641, 6.259949555863199677, -2.500000000000000444 ) ) ;
#3167=CARTESIAN_POINT ( 'NONE',  ( 7.343676480457483002, 8.596652644402405841, -1.199719254218452047 ) ) ;
#3171=CARTESIAN_POINT ( 'NONE',  ( 5.677832469072920496, 9.846164657218904992, 0.000000000000000000 ) ) ;
#3198=CARTESIAN_POINT ( 'NONE',  ( 4.584065335196260804, 6.441438539186039591, 1.443375672974065660 ) ) ;
#3204=CARTESIAN_POINT ( 'NONE',  ( -5.759181390754928742, 9.941071732514568993, 0.000000000000000000 ) ) ;
#3206=CARTESIAN_POINT ( 'NONE',  ( 6.770317605177710085, 8.992066187497757213, 1.599625672291268286 ) ) ;
#3211=CARTESIAN_POINT ( 'NONE',  ( -3.024877669624710386, 6.543124691288523920, 0.000000000000000000 ) ) ;
#3216=CARTESIAN_POINT ( 'NONE',  ( 0.000000000000000000, 2.999999999999999112, -2.500000000000000444 ) ) ;
#3233=CARTESIAN_POINT ( 'NONE',  ( 5.982890925380405456, 10.20206618957764100, 0.000000000000000000 ) ) ;
#3242=CARTESIAN_POINT ( 'NONE',  ( 6.455090533882185788, 8.624301270986276080, -1.443375672974078761 ) ) ;
#3253=CARTESIAN_POINT ( 'NONE',  ( -5.153507786970275006, 7.105788066255672497, -1.443375672974066548 ) ) ;
#3256=CARTESIAN_POINT ( 'NONE',  ( 6.984385409695311964, 8.177479728513226576, 1.199719254218452935 ) ) ;
#3261=CARTESIAN_POINT ( 'NONE',  ( -8.100070429521727178, 8.414780020722290033, 0.7998128361456341429 ) ) ;
#3263=SPHERICAL_SURFACE ( 'NONE', #125756, 0.08000000000000000167 ) ;
#3273=LINE ( 'NONE', #134409, #50861 ) ;
#3275=CARTESIAN_POINT ( 'NONE',  ( 3.714048807681376463, 7.355992446056095702, -0.08329438042602502201 ) ) ;
#3310=CARTESIAN_POINT ( 'NONE',  ( -5.255720823952942489, 6.160704378480398979, -1.199719254218453823 ) ) ;
#3314=CARTESIAN_POINT ( 'NONE',  ( -6.577113915960849155, 6.845923454808663600, -0.7216878364870338292 ) ) ;
#3321=CARTESIAN_POINT ( 'NONE',  ( -7.123883369337781879, 7.275895117174344229, 0.7998128361456341429 ) ) ;
#3329=CARTESIAN_POINT ( 'NONE',  ( -6.656127069666307072, 6.730179434224282886, 0.7998128361456341429 ) ) ;
#3331=CARTESIAN_POINT ( 'NONE',  ( 4.639288533706844575, 8.435234533841581950, -0.4270733708018232822 ) ) ;
#3336=CARTESIAN_POINT ( 'NONE',  ( 5.806634928402749196, 9.996434193103704402, -0.7998128361456481317 ) ) ;
#3355=CARTESIAN_POINT ( 'NONE',  ( -6.983858524370814003, 9.241197259889665006, 1.443375672974064550 ) ) ;
#3362=CARTESIAN_POINT ( 'NONE',  ( 5.830888582329017744, 8.960397891762626799, -1.199719254218452047 ) ) ;
#3377=CARTESIAN_POINT ( 'NONE',  ( 6.007156502879952953, 7.179297369210805080, -1.191424252104013037 ) ) ;
#3390=ORIENTED_EDGE ( 'NONE', *, *, #85316, .T. ) ;
#3400=CARTESIAN_POINT ( 'NONE',  ( -4.669937115657131876, 8.128295656576590034, -0.7159178489368930309 ) ) ;
#3405=CARTESIAN_POINT ( 'NONE',  ( -6.486551268120854807, 6.767445667853342783, -0.2095380678983837508 ) ) ;
#3425=CARTESIAN_POINT ( 'NONE',  ( -5.978219388983010418, 5.939287140093762574, -0.7998128361456362523 ) ) ;
#3441=CARTESIAN_POINT ( 'NONE',  ( 4.004454267989866700, 5.765225627445230927, 1.599625672291262513 ) ) ;
#3452=CARTESIAN_POINT ( 'NONE',  ( 4.868786560638885597, 7.733982516503781213, 1.082531754730548412 ) ) ;
#3456=CARTESIAN_POINT ( 'NONE',  ( -6.074935347375019390, 9.245119117649618801, 1.199719254218452047 ) ) ;
#3457=CARTESIAN_POINT ( 'NONE',  ( 4.193214648376505593, 8.114110533073061404, 0.000000000000000000 ) ) ;
#3466=CARTESIAN_POINT ( 'NONE',  ( -3.156015896931072540, 6.904045323053366268, 0.000000000000000000 ) ) ;
#3467=CARTESIAN_POINT ( 'NONE',  ( 5.671053392266061977, 9.838255734277600695, 0.7998128361456331437 ) ) ;
#3474=CARTESIAN_POINT ( 'NONE',  ( 5.525830126021535449, 8.604496359403894346, -1.199719254218452047 ) ) ;
#3479=CARTESIAN_POINT ( 'NONE',  ( -5.242543201390849283, 7.800132786123255002, 1.293859303942331840 ) ) ;
#3488=CARTESIAN_POINT ( 'NONE',  ( -3.309598895067336510, 6.875299454304925284, 0.000000000000000000 ) ) ;
#3491=CARTESIAN_POINT ( 'NONE',  ( -5.339680242214989825, 4.685059543140638105, 2.440369273555149210 ) ) ;
#3497=CARTESIAN_POINT ( 'NONE',  ( 3.933273961740298752, 5.682181936820735579, 1.443375672974058777 ) ) ;
#3501=CARTESIAN_POINT ( 'NONE',  ( -6.069210040772897052, 7.109775131437022999, -1.199719254218453823 ) ) ;
#3526=EDGE_LOOP ( 'NONE', ( #192939, #177773 ) ) ;
#3538=CARTESIAN_POINT ( 'NONE',  ( 0.4774960025711667555, 3.000292809610445754, 1.942428730326982711 ) ) ;
#3540=CARTESIAN_POINT ( 'NONE',  ( 6.215487077222150880, 6.216099443039444949, 0.000000000000000000 ) ) ;
#3542=CARTESIAN_POINT ( 'NONE',  ( -4.584065335196305213, 6.441438539186039591, 1.443375672974058777 ) ) ;
#3564=ORIENTED_EDGE ( 'NONE', *, *, #105759, .T. ) ;
#3565=CARTESIAN_POINT ( 'NONE',  ( -5.257529707049291900, 9.355811434857983500, 0.7998128361456291469 ) ) ;
#3578=CARTESIAN_POINT ( 'NONE',  ( -6.180537922983287302, 8.303989891604203422, -1.599625672291271394 ) ) ;
#3580=FACE_OUTER_BOUND ( 'NONE', #92498, .T. ) ;
#3589=CARTESIAN_POINT ( 'NONE',  ( -5.576146316970437944, 9.727530813099326323, 0.000000000000000000 ) ) ;
#3592=CARTESIAN_POINT ( 'NONE',  ( -7.105881907338169157, 8.423188659050232729, -1.082531754730549967 ) ) ;
#3597=CARTESIAN_POINT ( 'NONE',  ( 3.675669042636310557, 6.342012078834061484, -1.082531754730549967 ) ) ;
#3598=CARTESIAN_POINT ( 'NONE',  ( -4.516274566683622815, 5.401980094953223066, 1.082531754730549078 ) ) ;
#3616=CARTESIAN_POINT ( 'NONE',  ( 6.596403382356258227, 6.772441155557838321, -0.1798620802159808241 ) ) ;
#3622=( BOUNDED_CURVE ( )  B_SPLINE_CURVE ( 2, ( #210191, #208060, #46661, #58630, #142045, #10921, #27183 ),
 .UNSPECIFIED., .F., .T. ) 
 B_SPLINE_CURVE_WITH_KNOTS ( ( 3, 2, 2, 3 ),
 ( 0.3500000000000000888, 0.3583333333333333925, 0.3666666666666666963, 0.3750000000000000000 ),
 .UNSPECIFIED. ) 
 CURVE ( )  GEOMETRIC_REPRESENTATION_ITEM ( )  RATIONAL_B_SPLINE_CURVE ( ( 0.9999999999999982236, 0.8660254037844404840, 1.000000000000000000, 0.8660254037844387076, 1.000000000000000000, 0.8660254037844387076, 1.000000000000000000 ) ) 
 REPRESENTATION_ITEM ( '' )  );
#3636=CARTESIAN_POINT ( 'NONE',  ( 5.886377668569586774, 7.162856863344262415, 1.137212067324339104 ) ) ;
#3651=EDGE_CURVE ( 'NONE', #96370, #115058, #48028, .T. ) ;
#3654=CARTESIAN_POINT ( 'NONE',  ( -5.108390017298964914, 9.181815130149269422, 0.000000000000000000 ) ) ;
#3666=CARTESIAN_POINT ( 'NONE',  ( 6.222266154028957885, 6.224008365980749247, 0.7998128361456352531 ) ) ;
#3673=( BOUNDED_SURFACE ( )  B_SPLINE_SURFACE ( 1, 2, ( 
 ( #76699, #125547, #9572, #157984, #209883, #127687, #61521, #96181, #109286, #95114, #161163, #26882, #192571, #92985, #12749, #110348, #159030, #176351, #78823, #144944, #210951, #62577, #126608, #79892, #190445, #94051, #11695, #75649, #77769, #10623, #142815, #194713, #60451, #112472, #178481, #42104, #108217, #174241, #25814, #208821, #195790, #183794, #101481, #18075, #14875, #83084, #167551, #149163, #131893, #35403, #47428, #117802, #113543, #179546, #196850, #198953, #65747, #19152, #132948, #48487, #17008, #99361, #214119, #31167, #114605, #82024, #50595, #740, #66806, #148116, #129810, #115655, #97240, #130853, #147059, #181650, #67876, #116720, #80967, #63655, #64710, #213079, #182720, #163294, #32221, #146002, #212012, #200029, #34338, #180596, #98294, #100413, #51681, #166483, #84162, #164356, #15940, #197901, #49531, #165412, #150250, #33276, #1818, #134022, #40776, #151314, #121027, #119939, #169681, #20214, #154512, #86302, #152372, #123178, #70017, #106882, #136133, #37549, #203229, #72161, #88452, #170752, #102549, #171822, #3950, #185915, #22338, #71090, #172908, #205371, #137207, #138270, #186994, #87374, #38625, #153444, #73234, #103629, #202149, #204284, #89527, #53810, #155580, #21269, #168612, #118862, #5016, #54874, #104701, #6093, #189137, #55941, #122094, #139341, #188058, #39687, #105798, #85225, #68953, #23416, #7164, #57006, #135074, #2882, #201087, #52728, #184848, #36476, #12511, #177162, #158778, #156653, #209634, #141507, #206444, #76451, #207516, #26631, #127436, #91673, #190194, #28780, #9321, #191252, #8246, #74330, #59135, #144704, #94863, #24482, #11444, #125294, #109027, #173990, #41852, #124234, #25562, #128503, #107962, #77519, #160917, #159842, #43977, #112231, #90594, #142559, #157726, #60199, #42917, #110096, #208565, #58071, #75395, #46113, #93802, #176107, #140432, #27707, #210715, #175046, #61274, #111162, #92733, #126360, #10374, #192319, #143640, #193406, #62343, #45050, #78582, #194471, #132266, #183105, #85604, #3261, #118176, #48860, #32597, #151692, #116037 ),
 ( #134399, #2190, #148492, #69329, #66123, #17384, #68266, #117104, #86674, #36845, #34714, #184163, #114974, #165799, #102927, #201461, #131231, #35784, #99728, #1133, #198274, #59, #16317, #49916, #20588, #82402, #101860, #135440, #52049, #150629, #4322, #197219, #100785, #182024, #166867, #149547, #200401, #18461, #98672, #33654, #152741, #167928, #19527, #180975, #53105, #168989, #83468, #119238, #185221, #164728, #84539, #67195, #133332, #199336, #50982, #111272, #60308, #203596, #45158, #71465, #125398, #27816, #159954, #126467, #202529, #186293, #93913, #55248, #11558, #137578, #110204, #6468, #77628, #88829, #5388, #192430, #72544, #191363, #10484, #70392, #21633, #138642, #176214, #207622, #121395, #154884, #109142, #175155, #59239, #26741, #43030, #61387, #105083, #187368, #44085, #143750, #38998, #209745, #171121, #153817, #104004, #22715, #87741, #92844, #158888, #177275, #76558, #142668, #127546, #208679, #193517, #28891, #136509, #54178, #94975, #161021, #120318, #37930, #170048, #97109, #29959, #32082, #13687, #597, #165273, #146928, #144814, #197762, #129674, #194576, #64582, #195659, #14746, #115519, #79757, #178351, #16868, #211881, #179414, #210821, #46222, #63522, #65607, #212945, #100271, #213987, #47293, #98170, #180466, #80838, #112339, #113408, #163161, #131757, #15805, #164218, #130723, #62446, #196714, #96045, #31035, #145873, #48355, #149022, #81891, #162098, #128609, #114466, #147977, #49400, #181514, #33143, #198814, #78689, #66663, #99223, #50460, #12616, #82948, #132810, #116579, #182574, #34196, #84012, #102400, #1675, #119785, #153285, #201995, #200937, #22182, #121941, #17928, #53653, #52585, #36322, #101330, #21115, #167411, #19003, #204131, #151168, #187907, #2739, #118713, #69871, #4861, #169535, #37398, #183650, #38475, #85084, #184701, #103473, #152226, #39537, #72009, #3797, #70940, #87221, #137050, #203076, #55784, #68810, #54720, #120869, #134932, #135980, #168468, #186843, #185766, #20066, #104552, #170596, #88298, #154359, #5938, #86155, #166336, #150103, #138122 ) ),
 .UNSPECIFIED., .F., .F., .T. ) 
 B_SPLINE_SURFACE_WITH_KNOTS ( ( 2, 2 ),
 ( 3, 2, 2, 2, 2, 2, 2, 2, 2, 2, 2, 2, 2, 2, 2, 2, 2, 2, 2, 2, 2, 2, 2, 2, 2, 2, 2, 2, 2, 2, 2, 2, 2, 2, 2, 2, 2, 2, 2, 2, 2, 2, 2, 2, 2, 2, 2, 2, 2, 2, 2, 2, 2, 2, 2, 2, 2, 2, 2, 2, 2, 2, 2, 2, 2, 2, 2, 2, 2, 2, 2, 2, 2, 2, 2, 2, 2, 2, 2, 2, 2, 2, 2, 2, 2, 2, 2, 2, 2, 2, 2, 2, 2, 2, 2, 2, 2, 2, 2, 2, 2, 2, 2, 2, 2, 2, 2, 2, 2, 2, 2, 2, 2, 2, 2, 2, 2, 2, 2, 2, 3 ),
 ( 0.000000000000000000, 1.000000000000000000 ),
 ( 0.000000000000000000, 0.008333333333333333218, 0.01666666666666666644, 0.02500000000000000139, 0.03333333333333333287, 0.04166666666666666435, 0.05000000000000000278, 0.05833333333333333426, 0.06666666666666666574, 0.07499999999999999722, 0.08333333333333332871, 0.09166666666666666019, 0.1000000000000000056, 0.1083333333333333370, 0.1166666666666666685, 0.1250000000000000000, 0.1333333333333333315, 0.1416666666666666630, 0.1499999999999999944, 0.1583333333333333259, 0.1666666666666666574, 0.1749999999999999889, 0.1833333333333333204, 0.1916666666666666796, 0.2000000000000000111, 0.2083333333333333426, 0.2166666666666666741, 0.2250000000000000056, 0.2333333333333333370, 0.2416666666666666685, 0.2500000000000000000, 0.2583333333333333592, 0.2666666666666666630, 0.2750000000000000222, 0.2833333333333333259, 0.2916666666666666852, 0.2999999999999999889, 0.3083333333333333481, 0.3166666666666666519, 0.3250000000000000111, 0.3333333333333333148, 0.3416666666666666741, 0.3499999999999999778, 0.3583333333333333370, 0.3666666666666666408, 0.3750000000000000000, 0.3833333333333333592, 0.3916666666666666630, 0.4000000000000000222, 0.4083333333333333259, 0.4166666666666666852, 0.4249999999999999889, 0.4333333333333333481, 0.4416666666666666519, 0.4500000000000000111, 0.4583333333333333148, 0.4666666666666666741, 0.4749999999999999778, 0.4833333333333333370, 0.4916666666666666408, 0.5000000000000000000, 0.5083333333333333037, 0.5166666666666667185, 0.5250000000000000222, 0.5333333333333333259, 0.5416666666666666297, 0.5500000000000000444, 0.5583333333333333481, 0.5666666666666666519, 0.5749999999999999556, 0.5833333333333333703, 0.5916666666666666741, 0.5999999999999999778, 0.6083333333333332815, 0.6166666666666666963, 0.6250000000000000000, 0.6333333333333333037, 0.6416666666666667185, 0.6500000000000000222, 0.6583333333333333259, 0.6666666666666666297, 0.6750000000000000444, 0.6833333333333333481, 0.6916666666666666519, 0.6999999999999999556, 0.7083333333333333703, 0.7166666666666666741, 0.7249999999999999778, 0.7333333333333332815, 0.7416666666666666963, 0.7500000000000000000, 0.7583333333333333037, 0.7666666666666667185, 0.7750000000000000222, 0.7833333333333333259, 0.7916666666666666297, 0.8000000000000000444, 0.8083333333333333481, 0.8166666666666666519, 0.8249999999999999556, 0.8333333333333333703, 0.8416666666666666741, 0.8499999999999999778, 0.8583333333333332815, 0.8666666666666666963, 0.8750000000000000000, 0.8833333333333333037, 0.8916666666666667185, 0.9000000000000000222, 0.9083333333333333259, 0.9166666666666666297, 0.9250000000000000444, 0.9333333333333333481, 0.9416666666666666519, 0.9499999999999999556, 0.9583333333333333703, 0.9666666666666666741, 0.9749999999999999778, 0.9833333333333332815, 0.9916666666666666963, 1.000000000000000000 ),
 .UNSPECIFIED. ) 
 GEOMETRIC_REPRESENTATION_ITEM ( )  RATIONAL_B_SPLINE_SURFACE ( (
 ( 1.000000000000000000, 0.8660254037844387076, 1.000000000000000000, 0.8660254037844387076, 1.000000000000000000, 0.8660254037844387076, 1.000000000000000000, 0.8660254037844387076, 1.000000000000000000, 0.8660254037844387076, 1.000000000000000000, 0.8660254037844387076, 1.000000000000000000, 0.8660254037844387076, 1.000000000000000000, 0.8660254037844387076, 1.000000000000000000, 0.8660254037844387076, 1.000000000000000000, 0.8660254037844387076, 1.000000000000000000, 0.8660254037844387076, 1.000000000000000000, 0.8660254037844387076, 1.000000000000000000, 0.8660254037844387076, 1.000000000000000000, 0.8660254037844387076, 1.000000000000000000, 0.8660254037844387076, 1.000000000000000000, 0.8660254037844387076, 1.000000000000000000, 0.8660254037844387076, 1.000000000000000000, 0.8660254037844387076, 1.000000000000000000, 0.8660254037844387076, 1.000000000000000000, 0.8660254037844387076, 1.000000000000000000, 0.8660254037844387076, 1.000000000000000000, 0.8660254037844387076, 1.000000000000000000, 0.8660254037844387076, 1.000000000000000000, 0.8660254037844387076, 1.000000000000000000, 0.8660254037844387076, 1.000000000000000000, 0.8660254037844387076, 1.000000000000000000, 0.8660254037844387076, 1.000000000000000000, 0.8660254037844387076, 1.000000000000000000, 0.8660254037844387076, 1.000000000000000000, 0.8660254037844387076, 1.000000000000000000, 0.8660254037844387076, 1.000000000000000000, 0.8660254037844387076, 1.000000000000000000, 0.8660254037844387076, 1.000000000000000000, 0.8660254037844387076, 1.000000000000000000, 0.8660254037844387076, 1.000000000000000000, 0.8660254037844387076, 1.000000000000000000, 0.8660254037844387076, 1.000000000000000000, 0.8660254037844387076, 1.000000000000000000, 0.8660254037844387076, 1.000000000000000000, 0.8660254037844387076, 1.000000000000000000, 0.8660254037844387076, 1.000000000000000000, 0.8660254037844387076, 1.000000000000000000, 0.8660254037844387076, 1.000000000000000000, 0.8660254037844387076, 1.000000000000000000, 0.8660254037844387076, 1.000000000000000000, 0.8660254037844387076, 1.000000000000000000, 0.8660254037844387076, 1.000000000000000000, 0.8660254037844387076, 1.000000000000000000, 0.8660254037844387076, 1.000000000000000000, 0.8660254037844387076, 1.000000000000000000, 0.8660254037844387076, 1.000000000000000000, 0.8660254037844387076, 1.000000000000000000, 0.8660254037844387076, 1.000000000000000000, 0.8660254037844387076, 1.000000000000000000, 0.8660254037844387076, 1.000000000000000000, 0.8660254037844387076, 1.000000000000000000, 0.8660254037844387076, 1.000000000000000000, 0.8660254037844387076, 1.000000000000000000, 0.8660254037844387076, 1.000000000000000000, 0.8660254037844387076, 1.000000000000000000, 0.8660254037844387076, 1.000000000000000000, 0.8660254037844387076, 1.000000000000000000, 0.8660254037844387076, 1.000000000000000000, 0.8660254037844387076, 1.000000000000000000, 0.8660254037844387076, 1.000000000000000000, 0.8660254037844387076, 1.000000000000000000, 0.8660254037844387076, 1.000000000000000000, 0.8660254037844387076, 1.000000000000000000, 0.8660254037844387076, 1.000000000000000000, 0.8660254037844387076, 1.000000000000000000, 0.8660254037844387076, 1.000000000000000000, 0.8660254037844387076, 1.000000000000000000, 0.8660254037844387076, 1.000000000000000000, 0.8660254037844387076, 1.000000000000000000, 0.8660254037844387076, 1.000000000000000000, 0.8660254037844387076, 1.000000000000000000, 0.8660254037844387076, 1.000000000000000000, 0.8660254037844387076, 1.000000000000000000, 0.8660254037844387076, 1.000000000000000000, 0.8660254037844387076, 1.000000000000000000, 0.8660254037844387076, 1.000000000000000000, 0.8660254037844387076, 1.000000000000000000, 0.8660254037844387076, 1.000000000000000000, 0.8660254037844387076, 1.000000000000000000, 0.8660254037844387076, 1.000000000000000000, 0.8660254037844387076, 1.000000000000000000, 0.8660254037844387076, 1.000000000000000000, 0.8660254037844387076, 1.000000000000000000, 0.8660254037844387076, 1.000000000000000000, 0.8660254037844387076, 1.000000000000000000, 0.8660254037844387076, 1.000000000000000000, 0.8660254037844387076, 1.000000000000000000, 0.8660254037844387076, 1.000000000000000000, 0.8660254037844387076, 1.000000000000000000, 0.8660254037844387076, 1.000000000000000000, 0.8660254037844387076, 1.000000000000000000, 0.8660254037844387076, 1.000000000000000000, 0.8660254037844387076, 1.000000000000000000, 0.8660254037844387076, 1.000000000000000000, 0.8660254037844387076, 1.000000000000000000, 0.8660254037844387076, 1.000000000000000000, 0.8660254037844387076, 1.000000000000000000, 0.8660254037844387076, 1.000000000000000000, 0.8660254037844387076, 1.000000000000000000, 0.8660254037844387076, 1.000000000000000000, 0.8660254037844387076, 1.000000000000000000, 0.8660254037844387076, 1.000000000000000000, 0.8660254037844387076, 1.000000000000000000, 0.8660254037844387076, 1.000000000000000000, 0.8660254037844387076, 1.000000000000000000, 0.8660254037844387076, 1.000000000000000000, 0.8660254037844387076, 1.000000000000000000, 0.8660254037844387076, 1.000000000000000000, 0.8660254037844387076, 1.000000000000000000, 0.8660254037844387076, 1.000000000000000000, 0.8660254037844387076, 1.000000000000000000, 0.8660254037844387076, 1.000000000000000000, 0.8660254037844387076, 1.000000000000000000, 0.8660254037844387076, 1.000000000000000000, 0.8660254037844387076, 1.000000000000000000),
 ( 1.000000000000000000, 0.8660254037844387076, 1.000000000000000000, 0.8660254037844387076, 1.000000000000000000, 0.8660254037844387076, 1.000000000000000000, 0.8660254037844387076, 1.000000000000000000, 0.8660254037844387076, 1.000000000000000000, 0.8660254037844387076, 1.000000000000000000, 0.8660254037844387076, 1.000000000000000000, 0.8660254037844387076, 1.000000000000000000, 0.8660254037844387076, 1.000000000000000000, 0.8660254037844387076, 1.000000000000000000, 0.8660254037844387076, 1.000000000000000000, 0.8660254037844387076, 1.000000000000000000, 0.8660254037844387076, 1.000000000000000000, 0.8660254037844387076, 1.000000000000000000, 0.8660254037844387076, 1.000000000000000000, 0.8660254037844387076, 1.000000000000000000, 0.8660254037844387076, 1.000000000000000000, 0.8660254037844387076, 1.000000000000000000, 0.8660254037844387076, 1.000000000000000000, 0.8660254037844387076, 1.000000000000000000, 0.8660254037844387076, 1.000000000000000000, 0.8660254037844387076, 1.000000000000000000, 0.8660254037844387076, 1.000000000000000000, 0.8660254037844387076, 1.000000000000000000, 0.8660254037844387076, 1.000000000000000000, 0.8660254037844387076, 1.000000000000000000, 0.8660254037844387076, 1.000000000000000000, 0.8660254037844387076, 1.000000000000000000, 0.8660254037844387076, 1.000000000000000000, 0.8660254037844387076, 1.000000000000000000, 0.8660254037844387076, 1.000000000000000000, 0.8660254037844387076, 1.000000000000000000, 0.8660254037844387076, 1.000000000000000000, 0.8660254037844387076, 1.000000000000000000, 0.8660254037844387076, 1.000000000000000000, 0.8660254037844387076, 1.000000000000000000, 0.8660254037844387076, 1.000000000000000000, 0.8660254037844387076, 1.000000000000000000, 0.8660254037844387076, 1.000000000000000000, 0.8660254037844387076, 1.000000000000000000, 0.8660254037844387076, 1.000000000000000000, 0.8660254037844387076, 1.000000000000000000, 0.8660254037844387076, 1.000000000000000000, 0.8660254037844387076, 1.000000000000000000, 0.8660254037844387076, 1.000000000000000000, 0.8660254037844387076, 1.000000000000000000, 0.8660254037844387076, 1.000000000000000000, 0.8660254037844387076, 1.000000000000000000, 0.8660254037844387076, 1.000000000000000000, 0.8660254037844387076, 1.000000000000000000, 0.8660254037844387076, 1.000000000000000000, 0.8660254037844387076, 1.000000000000000000, 0.8660254037844387076, 1.000000000000000000, 0.8660254037844387076, 1.000000000000000000, 0.8660254037844387076, 1.000000000000000000, 0.8660254037844387076, 1.000000000000000000, 0.8660254037844387076, 1.000000000000000000, 0.8660254037844387076, 1.000000000000000000, 0.8660254037844387076, 1.000000000000000000, 0.8660254037844387076, 1.000000000000000000, 0.8660254037844387076, 1.000000000000000000, 0.8660254037844387076, 1.000000000000000000, 0.8660254037844387076, 1.000000000000000000, 0.8660254037844387076, 1.000000000000000000, 0.8660254037844387076, 1.000000000000000000, 0.8660254037844387076, 1.000000000000000000, 0.8660254037844387076, 1.000000000000000000, 0.8660254037844387076, 1.000000000000000000, 0.8660254037844387076, 1.000000000000000000, 0.8660254037844387076, 1.000000000000000000, 0.8660254037844387076, 1.000000000000000000, 0.8660254037844387076, 1.000000000000000000, 0.8660254037844387076, 1.000000000000000000, 0.8660254037844387076, 1.000000000000000000, 0.8660254037844387076, 1.000000000000000000, 0.8660254037844387076, 1.000000000000000000, 0.8660254037844387076, 1.000000000000000000, 0.8660254037844387076, 1.000000000000000000, 0.8660254037844387076, 1.000000000000000000, 0.8660254037844387076, 1.000000000000000000, 0.8660254037844387076, 1.000000000000000000, 0.8660254037844387076, 1.000000000000000000, 0.8660254037844387076, 1.000000000000000000, 0.8660254037844387076, 1.000000000000000000, 0.8660254037844387076, 1.000000000000000000, 0.8660254037844387076, 1.000000000000000000, 0.8660254037844387076, 1.000000000000000000, 0.8660254037844387076, 1.000000000000000000, 0.8660254037844387076, 1.000000000000000000, 0.8660254037844387076, 1.000000000000000000, 0.8660254037844387076, 1.000000000000000000, 0.8660254037844387076, 1.000000000000000000, 0.8660254037844387076, 1.000000000000000000, 0.8660254037844387076, 1.000000000000000000, 0.8660254037844387076, 1.000000000000000000, 0.8660254037844387076, 1.000000000000000000, 0.8660254037844387076, 1.000000000000000000, 0.8660254037844387076, 1.000000000000000000, 0.8660254037844387076, 1.000000000000000000, 0.8660254037844387076, 1.000000000000000000, 0.8660254037844387076, 1.000000000000000000, 0.8660254037844387076, 1.000000000000000000, 0.8660254037844387076, 1.000000000000000000, 0.8660254037844387076, 1.000000000000000000, 0.8660254037844387076, 1.000000000000000000, 0.8660254037844387076, 1.000000000000000000, 0.8660254037844387076, 1.000000000000000000, 0.8660254037844387076, 1.000000000000000000, 0.8660254037844387076, 1.000000000000000000, 0.8660254037844387076, 1.000000000000000000, 0.8660254037844387076, 1.000000000000000000, 0.8660254037844387076, 1.000000000000000000, 0.8660254037844387076, 1.000000000000000000, 0.8660254037844387076, 1.000000000000000000, 0.8660254037844387076, 1.000000000000000000, 0.8660254037844387076, 1.000000000000000000, 0.8660254037844387076, 1.000000000000000000, 0.8660254037844387076, 1.000000000000000000, 0.8660254037844387076, 1.000000000000000000, 0.8660254037844387076, 1.000000000000000000) ) ) 
 REPRESENTATION_ITEM ( '' )  SURFACE ( )  );
#3674=CARTESIAN_POINT ( 'NONE',  ( -7.065207446052822249, 7.415365906582643163, -0.7216878364870338292 ) ) ;
#3678=CARTESIAN_POINT ( 'NONE',  ( 5.338878628731272613, 9.450718510153643948, -0.7998128361456481317 ) ) ;
#3686=DIRECTION ( 'NONE',  ( 0.000000000000000000, 0.000000000000000000, -1.000000000000000000 ) ) ;
#3693=CARTESIAN_POINT ( 'NONE',  ( -6.116136693540540570, 10.14959355252370266, 0.000000000000000000 ) ) ;
#3694=CARTESIAN_POINT ( 'NONE',  ( 5.045042558060919724, 8.899983727797476263, -0.7216878364870458196 ) ) ;
#3704=CARTESIAN_POINT ( 'NONE',  ( -3.959863383643135393, 6.777535159962392086, 1.199719254218452935 ) ) ;
#3705=CARTESIAN_POINT ( 'NONE',  ( -3.526002468005825286, 6.271364091718859335, -1.199719254218450271 ) ) ;
#3707=CARTESIAN_POINT ( 'NONE',  ( 6.658462837642799670, 6.940830530104329377, 0.7216878364870328300 ) ) ;
#3715=CARTESIAN_POINT ( 'NONE',  ( -6.257301848505791853, 6.998106085372876706, 0.9978569239010106617 ) ) ;
#3720=CARTESIAN_POINT ( 'NONE',  ( -4.603423314590644466, 8.384863137925270493, -0.01591256823598764802 ) ) ;
#3726=CARTESIAN_POINT ( 'NONE',  ( 3.607878275012313285, 6.262922849939428716, 1.082531754730549078 ) ) ;
#3729=CARTESIAN_POINT ( 'NONE',  ( -4.468294144155606773, 7.370704380560280100, 1.199719254218452935 ) ) ;
#3740=CARTESIAN_POINT ( 'NONE',  ( 3.528865121306874464, 7.339036084825155015, -0.7998128361456362523 ) ) ;
#3776=CIRCLE ( 'NONE', #107649, 0.07999999999999994615 ) ;
#3777=CARTESIAN_POINT ( 'NONE',  ( 5.614485009834906393, 6.683225611963085733, -1.082531754730548412 ) ) ;
#3782=CARTESIAN_POINT ( 'NONE',  ( 5.763624699140868834, 7.817591130454727200, -1.443375672974078761 ) ) ;
#3797=CARTESIAN_POINT ( 'NONE',  ( -5.772739544368596043, 9.956889578397179363, -0.7998128361456362523 ) ) ;
#3807=CARTESIAN_POINT ( 'NONE',  ( -2.993318053567081360, 6.714231172462041819, 0.000000000000000000 ) ) ;
#3809=CARTESIAN_POINT ( 'NONE',  ( 3.729901657090938460, 7.365652676665848553, 0.7216878364870257245 ) ) ;
#3816=CARTESIAN_POINT ( 'NONE',  ( -7.435720902452096936, 7.639705572474380091, 0.000000000000000000 ) ) ;
#3821=CARTESIAN_POINT ( 'NONE',  ( -5.966997003790217136, 9.975597247814986801, -0.7216878364870338292 ) ) ;
#3824=CARTESIAN_POINT ( 'NONE',  ( -6.587282531393266360, 8.778525268082516320, 1.599625672291269396 ) ) ;
#3846=CARTESIAN_POINT ( 'NONE',  ( -4.543390873910949423, 6.393985001019784953, 1.443375672974058777 ) ) ;
#3848=CARTESIAN_POINT ( 'NONE',  ( 4.064412189046650248, 7.963840997188264659, 0.7998128361456271485 ) ) ;
#3849=CARTESIAN_POINT ( 'NONE',  ( -5.842637852846353397, 5.781108681267656202, 0.7998128361456281477 ) ) ;
#3850=CARTESIAN_POINT ( 'NONE',  ( -5.745623237141265882, 9.925253886631958622, 0.7998128361456291469 ) ) ;
#3854=EDGE_CURVE ( 'NONE', #157380, #188684, #180468, .T. ) ;
#3858=ORIENTED_EDGE ( 'NONE', *, *, #8612, .T. ) ;
#3882=AXIS2_PLACEMENT_3D ( 'NONE', #113039, #62086, #78321 ) ;
#3905=ORIENTED_EDGE ( 'NONE', *, *, #25840, .T. ) ;
#3908=CARTESIAN_POINT ( 'NONE',  ( 4.213551878797002992, 8.137837301896977849, 0.000000000000000000 ) ) ;
#3925=CARTESIAN_POINT ( 'NONE',  ( 5.890091390494168522, 5.836471141856793388, 0.000000000000000000 ) ) ;
#3930=CARTESIAN_POINT ( 'NONE',  ( -5.237192476628793614, 9.332084666034067055, 0.7998128361456291469 ) ) ;
#3947=CARTESIAN_POINT ( 'NONE',  ( 6.048345925472191631, 7.189396680206621149, 1.082531754730549967 ) ) ;
#3950=CARTESIAN_POINT ( 'NONE',  ( -6.069210040772897052, 7.109775131437022999, -1.199719254218453823 ) ) ;
#3961=CARTESIAN_POINT ( 'NONE',  ( 3.607351389687783794, 6.366271167014519783, 1.199719254218451159 ) ) ;
#3962=CARTESIAN_POINT ( 'NONE',  ( 4.064412189046650248, 7.963840997188264659, 0.7998128361456271485 ) ) ;
#3983=CARTESIAN_POINT ( 'NONE',  ( 5.894874513638865388, 7.262872338272549300, -1.253420816524719150 ) ) ;
#3984=DIRECTION ( 'NONE',  ( -0.000000000000000000, -1.000000000000000000, -0.000000000000000000 ) ) ;
#3992=CARTESIAN_POINT ( 'NONE',  ( 4.115782150200256950, 6.959440387612411349, 1.199719254218452047 ) ) ;
#3997=CARTESIAN_POINT ( 'NONE',  ( 6.099189001301251523, 8.209082816308541197, 1.599625672291268286 ) ) ;
#4002=CARTESIAN_POINT ( 'NONE',  ( 4.068855497876973537, 7.761098824249525130, -0.7216878364870338292 ) ) ;
#4005=CARTESIAN_POINT ( 'NONE',  ( 7.024532985656128936, 9.288650798055913427, 1.443375672974065660 ) ) ;
#4017=CARTESIAN_POINT ( 'NONE',  ( 6.490673131624099312, 6.748652840683030618, -0.08655830178419705867 ) ) ;
#4018=CARTESIAN_POINT ( 'NONE',  ( -5.804299160426224624, 9.785783097223662352, -0.7216878364870338292 ) ) ;
#4025=CARTESIAN_POINT ( 'NONE',  ( -5.480535539083196461, 6.054881262792200403, 1.008611741575331289 ) ) ;
#4036=ORIENTED_EDGE ( 'NONE', *, *, #72494, .F. ) ;
#4052=CARTESIAN_POINT ( 'NONE',  ( 4.830447868218803897, 8.857549289555754157, -0.7998128361456481317 ) ) ;
#4054=CARTESIAN_POINT ( 'NONE',  ( 7.550965208168244125, 7.774157262476569130, -0.7998128361456341429 ) ) ;
#4069=CARTESIAN_POINT ( 'NONE',  ( -3.447516199624892419, 7.244129009529488350, 0.7998128361456352531 ) ) ;
#4071=CARTESIAN_POINT ( 'NONE',  ( 6.997416677984476863, 7.336276677169590421, 0.000000000000000000 ) ) ;
#4087=CARTESIAN_POINT ( 'NONE',  ( -6.780486220610186798, 8.043560357867583832, -1.082531754730549967 ) ) ;
#4089=CARTESIAN_POINT ( 'NONE',  ( -5.560252395380252288, 7.580323442733986283, 1.443375672974058777 ) ) ;
#4113=CARTESIAN_POINT ( 'NONE',  ( -6.317173229324657413, 6.334733287159020954, 0.000000000000000000 ) ) ;
#4123=CARTESIAN_POINT ( 'NONE',  ( 6.966220764712146796, 6.002124920821316323, -2.500000000000000444 ) ) ;
#4124=CARTESIAN_POINT ( 'NONE',  ( -5.393601776927423153, 7.665310133586674901, -1.338224700579364379 ) ) ;
#4145=CARTESIAN_POINT ( 'NONE',  ( 4.618660464418627321, 8.442828270562628745, 0.5404566954739065121 ) ) ;
#4147=CARTESIAN_POINT ( 'NONE',  ( 2.969872605471133742, 6.610326516918480166, 0.1088621377024363707 ) ) ;
#4152=DIRECTION ( 'NONE',  ( 0.000000000000000000, 0.000000000000000000, -1.000000000000000000 ) ) ;
#4156=CARTESIAN_POINT ( 'NONE',  ( 4.386945222473598527, 7.275797305264619652, -1.199719254218452047 ) ) ;
#4164=CARTESIAN_POINT ( 'NONE',  ( 4.877901405866606588, 8.912911750144889567, 0.7998128361456341429 ) ) ;
#4166=CARTESIAN_POINT ( 'NONE',  ( 4.342354338126830804, 8.288106837781779035, -0.7998128361456381397 ) ) ;
#4179=CARTESIAN_POINT ( 'NONE',  ( 4.807910157829258679, 8.239027388120819140, -0.8806314816870459694 ) ) ;
#4181=CARTESIAN_POINT ( 'NONE',  ( -6.753369912938502750, 7.051555451282599307, 0.000000000000000000 ) ) ;
#4182=CARTESIAN_POINT ( 'NONE',  ( 5.722950238744200391, 7.770137593325314285, 1.443375672974065660 ) ) ;
#4191=CARTESIAN_POINT ( 'NONE',  ( 3.697477691155363289, 7.355658039646863600, 0.1550784054364961473 ) ) ;
#4193=ORIENTED_EDGE ( 'NONE', *, *, #105660, .F. ) ;
#4200=( BOUNDED_SURFACE ( )  B_SPLINE_SURFACE ( 1, 2, ( 
 ( #106976, #176197, #23515, #156751, #92826, #174080, #142651, #206537, #192413, #110187, #93896, #25651, #140524, #40871, #173001, #61370, #205469, #58167, #39788, #8339, #158870, #89621, #155673, #73331, #57101, #123269, #189232, #24582, #41942, #108055, #91762, #157817, #47274, #64562, #129654, #131739, #98153, #32064, #63501, #48337, #115501, #213970, #195639, #81872, #13667, #65590, #147957, #197744, #46202, #28870, #149002, #112318, #62428, #49382, #113387, #78670, #181496, #196697, #164199, #163143, #130706, #96027, #33124, #99203, #162078, #29941, #165253, #578, #16846, #114448, #82929, #66644, #12597, #161003, #193500, #178333, #179396, #94955, #45141, #15787, #111253, #177256, #144796, #212927, #210803, #128591, #194557, #79739, #145856, #180447, #31016, #211862, #97090, #80819, #14727, #146908, #170577, #103454, #3777, #102380, #17907, #152207, #137029, #203055, #52565, #135961, #150082, #132789, #88273, #83993, #101310, #1652, #198791, #69851, #116560, #2719, #50441, #18981, #201977, #85064, #67710, #184682, #199868, #118696, #117636, #54699, #183628, #133860, #51511, #120850, #182553, #35235, #53633, #36303, #21097, #119766, #168449, #167391, #185745, #186823, #38453, #20048, #37379, #151149, #34177, #154340, #68791, #134910, #200918, #100249, #169515, #166318, #86136, #87200, #153264, #4840, #70918, #104531, #22159, #5916, #57900, #56837, #76286, #123008, #89354, #139165, #208403, #204112, #188962, #75227, #206278, #174883, #125127, #40603, #55764, #106709, #73066, #207352, #60037, #74163, #24311, #172735, #93631, #8075, #140255, #155403, #6986, #205196, #25397, #156486, #105615, #142395, #92572, #90417, #121921, #23242, #124065, #190030, #157557, #41683, #10212, #191085, #42754, #107794, #141338, #126190, #158615, #173819, #26464, #91497, #192152, #43816, #109930, #9151, #187888, #27536, #58972, #108858, #175940, #159673, #171645, #71990, #138101, #39517, #195381, #162886, #128340, #180199, #31821, #194306, #62183, #97897, #181247, #163956, #80557, #15534, #131491, #44885, #193238, #65344, #210547 ),
 ( #197495, #94702, #61107, #130456, #114201, #129401, #160743, #64311, #145608, #127266, #196444, #48089, #176996, #110991, #45947, #81618, #147702, #112067, #178068, #213720, #32874, #49138, #146656, #115254, #98951, #28612, #12337, #11275, #29685, #95769, #78418, #77354, #143467, #209463, #144538, #161824, #30758, #13413, #79488, #211603, #63239, #47012, #212670, #113128, #179133, #96837, #14468, #51263, #68545, #185508, #102141, #134674, #18736, #132548, #2470, #69612, #135720, #34990, #200677, #50195, #165002, #169273, #198547, #1408, #182305, #82678, #52326, #148761, #117388, #330, #67468, #118456, #133616, #33932, #167149, #166073, #101061, #83745, #201744, #149838, #116314, #100008, #53385, #66403, #199618, #184442, #84820, #19807, #36060, #17661, #183384, #150908, #168208, #85891, #119521, #151968, #3540, #37131, #20859, #103211, #16595, #161462, #13042, #79121, #97532, #14098, #177706, #148403, #164641, #145237, #61814, #95410, #62867, #212305, #15172, #80188, #82308, #48769, #197131, #146293, #213366, #66032, #16225, #63940, #32505, #178778, #214402, #98580, #132180, #211242, #193935, #99637, #129034, #195010, #198186, #130094, #29316, #49821, #147337, #114884, #113838, #81259, #196089, #47721, #46643, #112765, #30390, #163589, #179834, #96478, #115946, #181935, #162525, #127982, #31455, #64987, #131142, #180883, #33566, #165705, #17294, #144183, #210174, #45582, #111699, #106892, #19433, #186201, #118086, #172919, #40787, #24494, #150536, #133237, #41862, #2099, #166775, #90605, #85513, #183011, #156665, #86584, #202436, #53013, #20499, #200312, #8257, #74340, #51963, #134304, #140444, #107972, #206455, #152650, #58082, #124244, #117012, #50889, #190203, #68174, #167835, #199242, #174000, #54090, #1038, #83371, #34628, #102840, #149455, #100698, #18371, #67101, #84448, #4234, #151599, #120228, #184072, #185129, #3167, #168896, #35691, #101767, #70304, #119147, #69238, #136420, #135355, #201372, #36754, #98736, #163743, #179987, #32657, #164793, #178932, #15322, #2256, #34777, #212457, #162680, #132333 ) ),
 .UNSPECIFIED., .F., .F., .T. ) 
 B_SPLINE_SURFACE_WITH_KNOTS ( ( 2, 2 ),
 ( 3, 2, 2, 2, 2, 2, 2, 2, 2, 2, 2, 2, 2, 2, 2, 2, 2, 2, 2, 2, 2, 2, 2, 2, 2, 2, 2, 2, 2, 2, 2, 2, 2, 2, 2, 2, 2, 2, 2, 2, 2, 2, 2, 2, 2, 2, 2, 2, 2, 2, 2, 2, 2, 2, 2, 2, 2, 2, 2, 2, 2, 2, 2, 2, 2, 2, 2, 2, 2, 2, 2, 2, 2, 2, 2, 2, 2, 2, 2, 2, 2, 2, 2, 2, 2, 2, 2, 2, 2, 2, 2, 2, 2, 2, 2, 2, 2, 2, 2, 2, 2, 2, 2, 2, 2, 2, 2, 2, 2, 2, 2, 2, 2, 2, 2, 2, 2, 2, 2, 2, 3 ),
 ( 0.000000000000000000, 1.000000000000000000 ),
 ( 0.000000000000000000, 0.008333333333333333218, 0.01666666666666666644, 0.02500000000000000139, 0.03333333333333333287, 0.04166666666666666435, 0.05000000000000000278, 0.05833333333333333426, 0.06666666666666666574, 0.07499999999999999722, 0.08333333333333332871, 0.09166666666666666019, 0.1000000000000000056, 0.1083333333333333370, 0.1166666666666666685, 0.1250000000000000000, 0.1333333333333333315, 0.1416666666666666630, 0.1499999999999999944, 0.1583333333333333259, 0.1666666666666666574, 0.1749999999999999889, 0.1833333333333333204, 0.1916666666666666796, 0.2000000000000000111, 0.2083333333333333426, 0.2166666666666666741, 0.2250000000000000056, 0.2333333333333333370, 0.2416666666666666685, 0.2500000000000000000, 0.2583333333333333592, 0.2666666666666666630, 0.2750000000000000222, 0.2833333333333333259, 0.2916666666666666852, 0.2999999999999999889, 0.3083333333333333481, 0.3166666666666666519, 0.3250000000000000111, 0.3333333333333333148, 0.3416666666666666741, 0.3499999999999999778, 0.3583333333333333370, 0.3666666666666666408, 0.3750000000000000000, 0.3833333333333333592, 0.3916666666666666630, 0.4000000000000000222, 0.4083333333333333259, 0.4166666666666666852, 0.4249999999999999889, 0.4333333333333333481, 0.4416666666666666519, 0.4500000000000000111, 0.4583333333333333148, 0.4666666666666666741, 0.4749999999999999778, 0.4833333333333333370, 0.4916666666666666408, 0.5000000000000000000, 0.5083333333333333037, 0.5166666666666667185, 0.5250000000000000222, 0.5333333333333333259, 0.5416666666666666297, 0.5500000000000000444, 0.5583333333333333481, 0.5666666666666666519, 0.5749999999999999556, 0.5833333333333333703, 0.5916666666666666741, 0.5999999999999999778, 0.6083333333333332815, 0.6166666666666666963, 0.6250000000000000000, 0.6333333333333333037, 0.6416666666666667185, 0.6500000000000000222, 0.6583333333333333259, 0.6666666666666666297, 0.6750000000000000444, 0.6833333333333333481, 0.6916666666666666519, 0.6999999999999999556, 0.7083333333333333703, 0.7166666666666666741, 0.7249999999999999778, 0.7333333333333332815, 0.7416666666666666963, 0.7500000000000000000, 0.7583333333333333037, 0.7666666666666667185, 0.7750000000000000222, 0.7833333333333333259, 0.7916666666666666297, 0.8000000000000000444, 0.8083333333333333481, 0.8166666666666666519, 0.8249999999999999556, 0.8333333333333333703, 0.8416666666666666741, 0.8499999999999999778, 0.8583333333333332815, 0.8666666666666666963, 0.8750000000000000000, 0.8833333333333333037, 0.8916666666666667185, 0.9000000000000000222, 0.9083333333333333259, 0.9166666666666666297, 0.9250000000000000444, 0.9333333333333333481, 0.9416666666666666519, 0.9499999999999999556, 0.9583333333333333703, 0.9666666666666666741, 0.9749999999999999778, 0.9833333333333332815, 0.9916666666666666963, 1.000000000000000000 ),
 .UNSPECIFIED. ) 
 GEOMETRIC_REPRESENTATION_ITEM ( )  RATIONAL_B_SPLINE_SURFACE ( (
 ( 1.000000000000000000, 0.8660254037844387076, 1.000000000000000000, 0.8660254037844387076, 1.000000000000000000, 0.8660254037844387076, 1.000000000000000000, 0.8660254037844387076, 1.000000000000000000, 0.8660254037844387076, 1.000000000000000000, 0.8660254037844387076, 1.000000000000000000, 0.8660254037844387076, 1.000000000000000000, 0.8660254037844387076, 1.000000000000000000, 0.8660254037844387076, 1.000000000000000000, 0.8660254037844387076, 1.000000000000000000, 0.8660254037844387076, 1.000000000000000000, 0.8660254037844387076, 1.000000000000000000, 0.8660254037844387076, 1.000000000000000000, 0.8660254037844387076, 1.000000000000000000, 0.8660254037844387076, 1.000000000000000000, 0.8660254037844387076, 1.000000000000000000, 0.8660254037844387076, 1.000000000000000000, 0.8660254037844387076, 1.000000000000000000, 0.8660254037844387076, 1.000000000000000000, 0.8660254037844387076, 1.000000000000000000, 0.8660254037844387076, 1.000000000000000000, 0.8660254037844387076, 1.000000000000000000, 0.8660254037844387076, 1.000000000000000000, 0.8660254037844387076, 1.000000000000000000, 0.8660254037844387076, 1.000000000000000000, 0.8660254037844387076, 1.000000000000000000, 0.8660254037844387076, 1.000000000000000000, 0.8660254037844387076, 1.000000000000000000, 0.8660254037844387076, 1.000000000000000000, 0.8660254037844387076, 1.000000000000000000, 0.8660254037844387076, 1.000000000000000000, 0.8660254037844387076, 1.000000000000000000, 0.8660254037844387076, 1.000000000000000000, 0.8660254037844387076, 1.000000000000000000, 0.8660254037844387076, 1.000000000000000000, 0.8660254037844387076, 1.000000000000000000, 0.8660254037844387076, 1.000000000000000000, 0.8660254037844387076, 1.000000000000000000, 0.8660254037844387076, 1.000000000000000000, 0.8660254037844387076, 1.000000000000000000, 0.8660254037844387076, 1.000000000000000000, 0.8660254037844387076, 1.000000000000000000, 0.8660254037844387076, 1.000000000000000000, 0.8660254037844387076, 1.000000000000000000, 0.8660254037844387076, 1.000000000000000000, 0.8660254037844387076, 1.000000000000000000, 0.8660254037844387076, 1.000000000000000000, 0.8660254037844387076, 1.000000000000000000, 0.8660254037844387076, 1.000000000000000000, 0.8660254037844387076, 1.000000000000000000, 0.8660254037844387076, 1.000000000000000000, 0.8660254037844387076, 1.000000000000000000, 0.8660254037844387076, 1.000000000000000000, 0.8660254037844387076, 1.000000000000000000, 0.8660254037844387076, 1.000000000000000000, 0.8660254037844387076, 1.000000000000000000, 0.8660254037844387076, 1.000000000000000000, 0.8660254037844387076, 1.000000000000000000, 0.8660254037844387076, 1.000000000000000000, 0.8660254037844387076, 1.000000000000000000, 0.8660254037844387076, 1.000000000000000000, 0.8660254037844387076, 1.000000000000000000, 0.8660254037844387076, 1.000000000000000000, 0.8660254037844387076, 1.000000000000000000, 0.8660254037844387076, 1.000000000000000000, 0.8660254037844387076, 1.000000000000000000, 0.8660254037844387076, 1.000000000000000000, 0.8660254037844387076, 1.000000000000000000, 0.8660254037844387076, 1.000000000000000000, 0.8660254037844387076, 1.000000000000000000, 0.8660254037844387076, 1.000000000000000000, 0.8660254037844387076, 1.000000000000000000, 0.8660254037844387076, 1.000000000000000000, 0.8660254037844387076, 1.000000000000000000, 0.8660254037844387076, 1.000000000000000000, 0.8660254037844387076, 1.000000000000000000, 0.8660254037844387076, 1.000000000000000000, 0.8660254037844387076, 1.000000000000000000, 0.8660254037844387076, 1.000000000000000000, 0.8660254037844387076, 1.000000000000000000, 0.8660254037844387076, 1.000000000000000000, 0.8660254037844387076, 1.000000000000000000, 0.8660254037844387076, 1.000000000000000000, 0.8660254037844387076, 1.000000000000000000, 0.8660254037844387076, 1.000000000000000000, 0.8660254037844387076, 1.000000000000000000, 0.8660254037844387076, 1.000000000000000000, 0.8660254037844387076, 1.000000000000000000, 0.8660254037844387076, 1.000000000000000000, 0.8660254037844387076, 1.000000000000000000, 0.8660254037844387076, 1.000000000000000000, 0.8660254037844387076, 1.000000000000000000, 0.8660254037844387076, 1.000000000000000000, 0.8660254037844387076, 1.000000000000000000, 0.8660254037844387076, 1.000000000000000000, 0.8660254037844387076, 1.000000000000000000, 0.8660254037844387076, 1.000000000000000000, 0.8660254037844387076, 1.000000000000000000, 0.8660254037844387076, 1.000000000000000000, 0.8660254037844387076, 1.000000000000000000, 0.8660254037844387076, 1.000000000000000000, 0.8660254037844387076, 1.000000000000000000, 0.8660254037844387076, 1.000000000000000000, 0.8660254037844387076, 1.000000000000000000, 0.8660254037844387076, 1.000000000000000000, 0.8660254037844387076, 1.000000000000000000, 0.8660254037844387076, 1.000000000000000000, 0.8660254037844387076, 1.000000000000000000, 0.8660254037844387076, 1.000000000000000000, 0.8660254037844387076, 1.000000000000000000, 0.8660254037844387076, 1.000000000000000000, 0.8660254037844387076, 1.000000000000000000, 0.8660254037844387076, 1.000000000000000000, 0.8660254037844387076, 1.000000000000000000, 0.8660254037844387076, 1.000000000000000000, 0.8660254037844387076, 1.000000000000000000, 0.8660254037844387076, 1.000000000000000000, 0.8660254037844387076, 1.000000000000000000, 0.8660254037844387076, 1.000000000000000000, 0.8660254037844387076, 1.000000000000000000),
 ( 1.000000000000000000, 0.8660254037844387076, 1.000000000000000000, 0.8660254037844387076, 1.000000000000000000, 0.8660254037844387076, 1.000000000000000000, 0.8660254037844387076, 1.000000000000000000, 0.8660254037844387076, 1.000000000000000000, 0.8660254037844387076, 1.000000000000000000, 0.8660254037844387076, 1.000000000000000000, 0.8660254037844387076, 1.000000000000000000, 0.8660254037844387076, 1.000000000000000000, 0.8660254037844387076, 1.000000000000000000, 0.8660254037844387076, 1.000000000000000000, 0.8660254037844387076, 1.000000000000000000, 0.8660254037844387076, 1.000000000000000000, 0.8660254037844387076, 1.000000000000000000, 0.8660254037844387076, 1.000000000000000000, 0.8660254037844387076, 1.000000000000000000, 0.8660254037844387076, 1.000000000000000000, 0.8660254037844387076, 1.000000000000000000, 0.8660254037844387076, 1.000000000000000000, 0.8660254037844387076, 1.000000000000000000, 0.8660254037844387076, 1.000000000000000000, 0.8660254037844387076, 1.000000000000000000, 0.8660254037844387076, 1.000000000000000000, 0.8660254037844387076, 1.000000000000000000, 0.8660254037844387076, 1.000000000000000000, 0.8660254037844387076, 1.000000000000000000, 0.8660254037844387076, 1.000000000000000000, 0.8660254037844387076, 1.000000000000000000, 0.8660254037844387076, 1.000000000000000000, 0.8660254037844387076, 1.000000000000000000, 0.8660254037844387076, 1.000000000000000000, 0.8660254037844387076, 1.000000000000000000, 0.8660254037844387076, 1.000000000000000000, 0.8660254037844387076, 1.000000000000000000, 0.8660254037844387076, 1.000000000000000000, 0.8660254037844387076, 1.000000000000000000, 0.8660254037844387076, 1.000000000000000000, 0.8660254037844387076, 1.000000000000000000, 0.8660254037844387076, 1.000000000000000000, 0.8660254037844387076, 1.000000000000000000, 0.8660254037844387076, 1.000000000000000000, 0.8660254037844387076, 1.000000000000000000, 0.8660254037844387076, 1.000000000000000000, 0.8660254037844387076, 1.000000000000000000, 0.8660254037844387076, 1.000000000000000000, 0.8660254037844387076, 1.000000000000000000, 0.8660254037844387076, 1.000000000000000000, 0.8660254037844387076, 1.000000000000000000, 0.8660254037844387076, 1.000000000000000000, 0.8660254037844387076, 1.000000000000000000, 0.8660254037844387076, 1.000000000000000000, 0.8660254037844387076, 1.000000000000000000, 0.8660254037844387076, 1.000000000000000000, 0.8660254037844387076, 1.000000000000000000, 0.8660254037844387076, 1.000000000000000000, 0.8660254037844387076, 1.000000000000000000, 0.8660254037844387076, 1.000000000000000000, 0.8660254037844387076, 1.000000000000000000, 0.8660254037844387076, 1.000000000000000000, 0.8660254037844387076, 1.000000000000000000, 0.8660254037844387076, 1.000000000000000000, 0.8660254037844387076, 1.000000000000000000, 0.8660254037844387076, 1.000000000000000000, 0.8660254037844387076, 1.000000000000000000, 0.8660254037844387076, 1.000000000000000000, 0.8660254037844387076, 1.000000000000000000, 0.8660254037844387076, 1.000000000000000000, 0.8660254037844387076, 1.000000000000000000, 0.8660254037844387076, 1.000000000000000000, 0.8660254037844387076, 1.000000000000000000, 0.8660254037844387076, 1.000000000000000000, 0.8660254037844387076, 1.000000000000000000, 0.8660254037844387076, 1.000000000000000000, 0.8660254037844387076, 1.000000000000000000, 0.8660254037844387076, 1.000000000000000000, 0.8660254037844387076, 1.000000000000000000, 0.8660254037844387076, 1.000000000000000000, 0.8660254037844387076, 1.000000000000000000, 0.8660254037844387076, 1.000000000000000000, 0.8660254037844387076, 1.000000000000000000, 0.8660254037844387076, 1.000000000000000000, 0.8660254037844387076, 1.000000000000000000, 0.8660254037844387076, 1.000000000000000000, 0.8660254037844387076, 1.000000000000000000, 0.8660254037844387076, 1.000000000000000000, 0.8660254037844387076, 1.000000000000000000, 0.8660254037844387076, 1.000000000000000000, 0.8660254037844387076, 1.000000000000000000, 0.8660254037844387076, 1.000000000000000000, 0.8660254037844387076, 1.000000000000000000, 0.8660254037844387076, 1.000000000000000000, 0.8660254037844387076, 1.000000000000000000, 0.8660254037844387076, 1.000000000000000000, 0.8660254037844387076, 1.000000000000000000, 0.8660254037844387076, 1.000000000000000000, 0.8660254037844387076, 1.000000000000000000, 0.8660254037844387076, 1.000000000000000000, 0.8660254037844387076, 1.000000000000000000, 0.8660254037844387076, 1.000000000000000000, 0.8660254037844387076, 1.000000000000000000, 0.8660254037844387076, 1.000000000000000000, 0.8660254037844387076, 1.000000000000000000, 0.8660254037844387076, 1.000000000000000000, 0.8660254037844387076, 1.000000000000000000, 0.8660254037844387076, 1.000000000000000000, 0.8660254037844387076, 1.000000000000000000, 0.8660254037844387076, 1.000000000000000000, 0.8660254037844387076, 1.000000000000000000, 0.8660254037844387076, 1.000000000000000000, 0.8660254037844387076, 1.000000000000000000, 0.8660254037844387076, 1.000000000000000000, 0.8660254037844387076, 1.000000000000000000, 0.8660254037844387076, 1.000000000000000000, 0.8660254037844387076, 1.000000000000000000, 0.8660254037844387076, 1.000000000000000000, 0.8660254037844387076, 1.000000000000000000, 0.8660254037844387076, 1.000000000000000000, 0.8660254037844387076, 1.000000000000000000, 0.8660254037844387076, 1.000000000000000000, 0.8660254037844387076, 1.000000000000000000) ) ) 
 REPRESENTATION_ITEM ( '' )  SURFACE ( )  );
#4202=CARTESIAN_POINT ( 'NONE',  ( -4.868786560638931782, 6.773613302202437403, 1.443375672974058777 ) ) ;
#4207=CARTESIAN_POINT ( 'NONE',  ( 5.180097208873055692, 8.201141289397330780, -1.199719254218450271 ) ) ;
#4227=ORIENTED_EDGE ( 'NONE', *, *, #28879, .T. ) ;
#4234=CARTESIAN_POINT ( 'NONE',  ( 6.749980374757213575, 8.968339418673846097, 1.599625672291268286 ) ) ;
#4248=CARTESIAN_POINT ( 'NONE',  ( 1.807716826991497161, 2.517780620582467765, 2.499994708711101854 ) ) ;
#4263=CARTESIAN_POINT ( 'NONE',  ( 4.963693636378940788, 5.923969009597785274, -1.082531754730548412 ) ) ;
#4270=CARTESIAN_POINT ( 'NONE',  ( 6.230854113932139171, 9.427024345299638952, 1.199719254218452047 ) ) ;
#4276=ORIENTED_EDGE ( 'NONE', *, *, #48686, .F. ) ;
#4284=CARTESIAN_POINT ( 'NONE',  ( -5.015590482412729756, 4.816220082428420923, 0.000000000000000000 ) ) ;
#4285=CARTESIAN_POINT ( 'NONE',  ( -4.462041952228944730, 7.259447140025469203, -1.082531754730549967 ) ) ;
#4293=CARTESIAN_POINT ( 'NONE',  ( 5.820193082016415609, 10.01225203898631655, 0.000000000000000000 ) ) ;
#4302=CARTESIAN_POINT ( 'NONE',  ( 5.076602173674213070, 4.887400388900169368, 0.000000000000000000 ) ) ;
#4312=CARTESIAN_POINT ( 'NONE',  ( -3.147653791585729444, 8.999999999999998224, 2.419999999999999485 ) ) ;
#4314=CARTESIAN_POINT ( 'NONE',  ( -5.560252395380252288, 7.580323442733986283, 1.443375672974058777 ) ) ;
#4317=CARTESIAN_POINT ( 'NONE',  ( 5.854088466050551887, 10.05179665369283981, 0.7998128361456341429 ) ) ;
#4320=CARTESIAN_POINT ( 'NONE',  ( -8.106849506328558164, 8.422688943663599659, 0.000000000000000000 ) ) ;
#4322=CARTESIAN_POINT ( 'NONE',  ( -5.340986169140711226, 5.195848383611072485, 0.000000000000000000 ) ) ;
#4336=CARTESIAN_POINT ( 'NONE',  ( -0.4437274321079128780, 2.826106777454868713, -1.950208266479945163 ) ) ;
#4367=CARTESIAN_POINT ( 'NONE',  ( -4.796552484184649856, 8.818004674849227342, -0.7998128361456362523 ) ) ;
#4371=CARTESIAN_POINT ( 'NONE',  ( -4.122561227007127016, 6.967349310553715647, 1.199719254218452935 ) ) ;
#4375=CARTESIAN_POINT ( 'NONE',  ( -5.221298554594238084, 8.145246509451649075, 1.082531754730549967 ) ) ;
#4377=CARTESIAN_POINT ( 'NONE',  ( 2.969872605471133742, 6.602209919732136001, 0.2729278363745436531 ) ) ;
#4381=CARTESIAN_POINT ( 'NONE',  ( -6.099189001301292379, 8.209082816308541197, 1.599625672291263179 ) ) ;
#4389=CARTESIAN_POINT ( 'NONE',  ( -7.228432174741334038, 8.462200954400218578, -1.199719254218452047 ) ) ;
#4391=CARTESIAN_POINT ( 'NONE',  ( 4.595358334023878832, 8.489709390108890474, -0.01759220550971198060 ) ) ;
#4394=CARTESIAN_POINT ( 'NONE',  ( 3.809456170543648046, 8.470288933811609411, 2.500000000000000444 ) ) ;
#4396=CARTESIAN_POINT ( 'NONE',  ( 4.411198876399872404, 6.239761003923544713, -1.599625672291273171 ) ) ;
#4410=CARTESIAN_POINT ( 'NONE',  ( 4.529832720297257254, 8.298905583739861314, 0.000000000000000000 ) ) ;
#4420=CARTESIAN_POINT ( 'NONE',  ( 6.690022453700429139, 6.769724048930809701, 0.7998128361456331437 ) ) ;
#4435=CARTESIAN_POINT ( 'NONE',  ( 5.494857653270467601, 7.581134149042087600, -1.337725346733337872 ) ) ;
#4456=CARTESIAN_POINT ( 'NONE',  ( -4.866920030118153662, 7.975534482151904747, -1.006773929442051685 ) ) ;
#4461=CARTESIAN_POINT ( 'NONE',  ( -6.502837976706968171, 6.831778935668112673, 0.5908271424688981144 ) ) ;
#4470=( BOUNDED_CURVE ( )  B_SPLINE_CURVE ( 2, ( #155751, #19326, #53979 ),
 .UNSPECIFIED., .F., .T. ) 
 B_SPLINE_CURVE_WITH_KNOTS ( ( 3, 3 ),
 ( 0.4749999999999995892, 0.4816879153505086442 ),
 .UNSPECIFIED. ) 
 CURVE ( )  GEOMETRIC_REPRESENTATION_ITEM ( )  RATIONAL_B_SPLINE_CURVE ( ( 1.000000000000006217, 0.8924787089670062068, 0.9575398082074682016 ) ) 
 REPRESENTATION_ITEM ( '' )  );
#4479=CARTESIAN_POINT ( 'NONE',  ( -4.847922445338252118, 7.813604065273374921, -1.199719254218453823 ) ) ;
#4481=ORIENTED_EDGE ( 'NONE', *, *, #22105, .F. ) ;
#4498=CARTESIAN_POINT ( 'NONE',  ( 3.088225128862704949, 6.824956093640315302, 0.7998128361456281477 ) ) ;
#4500=CARTESIAN_POINT ( 'NONE',  ( 7.987161891782087686, 8.490979426600148372, -0.7216878364870317197 ) ) ;
#4505=CARTESIAN_POINT ( 'NONE',  ( -6.385081391588430577, 6.907945078588741517, 0.8473268098342846555 ) ) ;
#4512=CARTESIAN_POINT ( 'NONE',  ( -6.448838341955544173, 7.552674816150118708, 1.199719254218452047 ) ) ;
#4514=CARTESIAN_POINT ( 'NONE',  ( 6.201928923608456046, 6.200281597156833691, 0.7998128361456352531 ) ) ;
#4523=CARTESIAN_POINT ( 'NONE',  ( -3.644109427023046521, 7.473487774827342278, 0.000000000000000000 ) ) ;
#4524=CARTESIAN_POINT ( 'NONE',  ( 7.075376061485196821, 9.347967719856493218, 1.599625672291268286 ) ) ;
#4526=FACE_OUTER_BOUND ( 'NONE', #155740, .T. ) ;
#4531=CARTESIAN_POINT ( 'NONE',  ( 6.550524494058025837, 7.671308660269694712, -1.199719254218452047 ) ) ;
#4536=CARTESIAN_POINT ( 'NONE',  ( -4.785410049391000342, 8.260660143818395085, 0.8633373473483215710 ) ) ;
#4547=CARTESIAN_POINT ( 'NONE',  ( -4.787437638956927977, 7.639075441208117212, -1.082531754730549967 ) ) ;
#4558=CARTESIAN_POINT ( 'NONE',  ( 4.638297949650961982, 5.544340708415133712, -1.082531754730548412 ) ) ;
#4561=CARTESIAN_POINT ( 'NONE',  ( -6.286140498591554326, 7.362860665558790707, 1.199719254218452047 ) ) ;
#4565=EDGE_CURVE ( 'NONE', #112384, #212524, #189638, .T. ) ;
#4575=CARTESIAN_POINT ( 'NONE',  ( 4.934241560730721510, 4.721313007132757811, 0.000000000000000000 ) ) ;
#4580=CARTESIAN_POINT ( 'NONE',  ( 4.875038752565570732, 7.845239757038595663, -1.199719254218452047 ) ) ;
#4599=CARTESIAN_POINT ( 'NONE',  ( -0.3866901564497973731, 3.102326550341738098, 2.027579305719746205 ) ) ;
#4601=CARTESIAN_POINT ( 'NONE',  ( -4.611181642423629157, 7.433443445252599702, 1.082531754730549967 ) ) ;
#4626=CARTESIAN_POINT ( 'NONE',  ( -5.932574734431526942, 9.079031735882207244, 1.199719254218454489 ) ) ;
#4643=CARTESIAN_POINT ( 'NONE',  ( -7.208094944320834863, 8.438474185576302133, -1.199719254218452047 ) ) ;
#4645=CARTESIAN_POINT ( 'NONE',  ( 5.207906507908255378, 7.834591108650524660, -1.266300940072472736 ) ) ;
#4649=CARTESIAN_POINT ( 'NONE',  ( 3.054329744828568227, 6.785411478933790264, 0.000000000000000000 ) ) ;
#4654=CARTESIAN_POINT ( 'NONE',  ( -5.749539660647037032, 8.865490816466966351, 1.199719254218454489 ) ) ;
#4657=CARTESIAN_POINT ( 'NONE',  ( -3.461074353238556167, 7.259946855412102273, 0.000000000000000000 ) ) ;
#4661=CARTESIAN_POINT ( 'NONE',  ( 5.194182247366881278, 5.232503174782402233, 0.7216878364870328300 ) ) ;
#4662=CARTESIAN_POINT ( 'NONE',  ( -4.868786560638931782, 6.773613302202437403, 1.443375672974058777 ) ) ;
#4667=CARTESIAN_POINT ( 'NONE',  ( -5.123001941117347968, 7.070197912760590064, 1.599625672291263401 ) ) ;
#4676=CARTESIAN_POINT ( 'NONE',  ( 4.960304097753311048, 6.880383762169266504, 1.599625672291268286 ) ) ;
#4681=CARTESIAN_POINT ( 'NONE',  ( 5.057296774772758852, 7.978757421411086348, 1.172581024337983724 ) ) ;
#4688=CARTESIAN_POINT ( 'NONE',  ( 5.851225812749518695, 8.984124660586543243, -1.199719254218452047 ) ) ;
#4698=CARTESIAN_POINT ( 'NONE',  ( 5.582388601459258304, 7.396495182493852738, 1.242574333668546638 ) ) ;
#4718=CARTESIAN_POINT ( 'NONE',  ( -4.471156797456668386, 8.438376373666578445, -0.7998128361456362523 ) ) ;
#4723=CARTESIAN_POINT ( 'NONE',  ( 8.014278199453780616, 8.522615118883788199, 0.000000000000000000 ) ) ;
#4731=CARTESIAN_POINT ( 'NONE',  ( 4.199993725183334803, 8.122019456014369254, -0.7998128361456362523 ) ) ;
#4733=CARTESIAN_POINT ( 'NONE',  ( 7.614839552730775729, 8.913009562054615031, 1.199719254218452047 ) ) ;
#4742=CARTESIAN_POINT ( 'NONE',  ( 3.675669042636310557, 6.342012078834061484, -1.082531754730549967 ) ) ;
#4749=CARTESIAN_POINT ( 'NONE',  ( 4.517335436343452137, 8.499999999999996447, 0.7749999999999996891 ) ) ;
#4756=CARTESIAN_POINT ( 'NONE',  ( -5.939880696562884310, 9.943961556049767836, 0.7216878364870267237 ) ) ;
#4757=CARTESIAN_POINT ( 'NONE',  ( 6.292392690518195941, 8.434487120394948079, -1.443375672974078761 ) ) ;
#4766=CARTESIAN_POINT ( 'NONE',  ( -4.797606254389363833, 6.690569611577942943, 1.599625672291263179 ) ) ;
#4767=CARTESIAN_POINT ( 'NONE',  ( -5.157951095356222204, 4.982307464195829816, 0.000000000000000000 ) ) ;
#4769=CARTESIAN_POINT ( 'NONE',  ( 6.170369307550823912, 7.331757292631694511, 1.082531754730549967 ) ) ;
#4781=CARTESIAN_POINT ( 'NONE',  ( -4.634775730458505549, 8.344889633747440527, 0.3497604727749434872 ) ) ;
#4788=DIRECTION ( 'NONE',  ( 0.000000000000000000, 0.000000000000000000, -1.000000000000000000 ) ) ;
#4789=CARTESIAN_POINT ( 'NONE',  ( -5.601453741101424022, 6.564059448486966986, -1.199719254218453823 ) ) ;
#4800=CARTESIAN_POINT ( 'NONE',  ( 6.527324610336440180, 6.579909898339485252, 0.7998128361456331437 ) ) ;
#4812=VECTOR ( 'NONE', #172412, 1000.000000000000000 ) ;
#4819=ADVANCED_FACE ( 'NONE', ( #193864 ), #44446, .F. ) ;
#4840=CARTESIAN_POINT ( 'NONE',  ( 6.861835142292147083, 7.178098218861903135, 0.7216878364870328300 ) ) ;
#4844=CARTESIAN_POINT ( 'NONE',  ( 6.848276988234151652, 7.162280372460873679, -0.7216878364870317197 ) ) ;
#4861=CARTESIAN_POINT ( 'NONE',  ( -6.149505192250180663, 9.332117270003974951, -1.199719254218452047 ) ) ;
#4873=CARTESIAN_POINT ( 'NONE',  ( 3.228249973385329596, 6.780392379009261283, -1.734723475976807094E-15 ) ) ;
#4879=CARTESIAN_POINT ( 'NONE',  ( -5.340986169140711226, 5.195848383611072485, 0.000000000000000000 ) ) ;
#4885=CARTESIAN_POINT ( 'NONE',  ( -7.607533591043815768, 8.048079742405473525, 0.000000000000000000 ) ) ;
#4888=CARTESIAN_POINT ( 'NONE',  ( -7.099629715411508890, 8.311931418515415615, 1.199719254218452047 ) ) ;
#4901=DIRECTION ( 'NONE',  ( 0.000000000000000000, 0.000000000000000000, -1.000000000000000000 ) ) ;
#4908=CARTESIAN_POINT ( 'NONE',  ( -3.675669043080673770, 7.302381293653823491, 0.000000000000000000 ) ) ;
#4910=CARTESIAN_POINT ( 'NONE',  ( -5.112833325684916552, 7.058334528089422300, -1.443375672974066548 ) ) ;
#4911=CARTESIAN_POINT ( 'NONE',  ( 6.073126464278658432, 6.050012061272033392, 0.000000000000000000 ) ) ;
#4912=CARTESIAN_POINT ( 'NONE',  ( -3.820365424000704557, 7.679119771301277098, -0.7998128361456481317 ) ) ;
#4913=CARTESIAN_POINT ( 'NONE',  ( -5.284646014276622950, 9.387447126623207794, -0.7998128361456362523 ) ) ;
#4916=CARTESIAN_POINT ( 'NONE',  ( -5.608757509019071996, 5.629766575911039794, 0.4613631940431175416 ) ) ;
#4953=CLOSED_SHELL ( 'NONE', ( #198823, #171874, #825, #2469, #197741, #47697, #205413, #23197, #90561, #130667, #13106, #154164, #153476, #166301, #75225, #119571, #52703, #143729, #195068, #161161, #126757, #47786, #65725, #174690, #143847, #18503, #204388, #101033, #122550, #30052, #10413, #172137, #207688, #84503, #29165, #150410, #141036, #5117, #4819, #68995, #99839, #26329, #6086, #132105, #19712, #123390, #62771, #210940, #171934, #209739, #197319, #116928, #181368, #46215, #138304, #178206, #142040, #28362, #61359, #44869, #213826, #86494, #16855, #187300, #196987, #43023, #199535, #35756, #61310, #210611, #60406, #68147, #123510, #56246, #208109, #58868, #69918, #92443, #15911, #20778, #133964, #210996, #148626, #204370, #8727, #7986, #142207, #169369, #81246, #155525, #142497, #163536, #179890, #78945, #54584, #94614, #28852, #9276, #133817, #74015, #124376, #37654, #174784, #210032, #154511, #146239, #144646, #38233, #140053, #141252, #86624, #128257, #90630, #144786, #11620, #146903, #200229, #192889, #131589, #2324, #108393, #104607, #205436, #64327, #112460, #121265, #19638, #25767, #80358, #104194, #113853, #151358, #86956, #137, #119208, #195211, #118228, #156600, #210578, #154061, #27655, #175607, #29382, #41806, #20517, #94911, #108688, #143589, #118366, #107722, #173726, #111324, #31661, #61863, #198603, #35667, #134368, #190241, #104712, #11185, #40373, #193838, #205563, #120359, #105962, #189169, #134276, #10673, #57150, #172933, #49558, #23348, #13844, #89786, #197363, #159829 ) ) ;
#4961=FACE_OUTER_BOUND ( 'NONE', #116639, .T. ) ;
#4969=CARTESIAN_POINT ( 'NONE',  ( 3.739016502318667445, 7.584212696005614873, 0.7998128361456271485 ) ) ;
#4987=CARTESIAN_POINT ( 'NONE',  ( 4.746236293235721604, 7.694970221153795364, 1.199719254218451159 ) ) ;
#4993=CARTESIAN_POINT ( 'NONE',  ( -5.749539660647037032, 8.865490816466966351, 1.199719254218454489 ) ) ;
#4998=CARTESIAN_POINT ( 'NONE',  ( 4.766573523656222555, 7.718696989977711809, 1.199719254218452047 ) ) ;
#4999=EDGE_CURVE ( 'NONE', #50747, #93524, #187783, .T. ) ;
#5013=CARTESIAN_POINT ( 'NONE',  ( 7.051649292883499953, 7.399548061218447437, -0.7216878364870317197 ) ) ;
#5015=CARTESIAN_POINT ( 'NONE',  ( -3.689227196694341515, 7.318199139536432973, -0.7216878364870458196 ) ) ;
#5016=CARTESIAN_POINT ( 'NONE',  ( -5.315678745009726924, 8.359319748223434487, -1.199719254218453823 ) ) ;
#5018=CARTESIAN_POINT ( 'NONE',  ( -5.800227658267527175, 5.731630120925694349, -0.5022995730114099278 ) ) ;
#5027=CARTESIAN_POINT ( 'NONE',  ( 4.716257332707354699, 6.595662536282280719, -1.599625672291269396 ) ) ;
#5028=CARTESIAN_POINT ( 'NONE',  ( 4.712340909201580885, 7.655425606447271214, -1.199719254218452047 ) ) ;
#5052=CARTESIAN_POINT ( 'NONE',  ( 4.258669648468303315, 7.982548666606043675, 0.7216878364870509266 ) ) ;
#5055=CARTESIAN_POINT ( 'NONE',  ( 4.736594563127852098, 6.619389305106191834, -1.599625672291273171 ) ) ;
#5059=CARTESIAN_POINT ( 'NONE',  ( 7.506374323821472849, 8.786466794993730289, -1.199719254218452047 ) ) ;
#5064=CARTESIAN_POINT ( 'NONE',  ( 6.102578539926878598, 7.252668063737060855, -1.082531754730548412 ) ) ;
#5068=CARTESIAN_POINT ( 'NONE',  ( 4.065465959251388206, 5.836405933916976707, -1.599625672291269396 ) ) ;
#5079=CARTESIAN_POINT ( 'NONE',  ( 5.925280661667059690, 7.134359284303951831, -1.114000666120490868 ) ) ;
#5080=CARTESIAN_POINT ( 'NONE',  ( -5.790741006812557323, 9.769965251341050205, 0.000000000000000000 ) ) ;
#5089=CARTESIAN_POINT ( 'NONE',  ( 0.3993783336448741283, 2.892526381812567493, -2.025045271722654583 ) ) ;
#5113=CARTESIAN_POINT ( 'NONE',  ( 6.180537922983273091, 8.303989891604203422, -1.599625672291281386 ) ) ;
#5115=CARTESIAN_POINT ( 'NONE',  ( 7.700104897918568447, 7.948153567185284096, 0.000000000000000000 ) ) ;
#5117=ADVANCED_FACE ( 'NONE', ( #213302 ), #31385, .F. ) ;
#5131=CARTESIAN_POINT ( 'NONE',  ( -5.659602779061863487, 5.567567761852417085, 0.7998128361456281477 ) ) ;
#5133=CARTESIAN_POINT ( 'NONE',  ( 4.855228407025239612, 8.678533884922511987, 0.000000000000000000 ) ) ;
#5141=EDGE_CURVE ( 'NONE', #176704, #206450, #9819, .T. ) ;
#5142=CARTESIAN_POINT ( 'NONE',  ( -5.646044625448194410, 5.551749915969804938, 0.000000000000000000 ) ) ;
#5148=CARTESIAN_POINT ( 'NONE',  ( -3.474632506852224356, 7.275764701294714420, -0.7998128361456481317 ) ) ;
#5150=CARTESIAN_POINT ( 'NONE',  ( -6.346625304972878467, 7.537389289624049304, 1.082531754730548412 ) ) ;
#5163=AXIS2_PLACEMENT_3D ( 'NONE', #101028, #113373, #44052 ) ;
#5176=CARTESIAN_POINT ( 'NONE',  ( -4.444040490229335560, 8.406740681901359480, 0.7998128361456352531 ) ) ;
#5187=CARTESIAN_POINT ( 'NONE',  ( -6.586110727467836767, 6.776993156853382771, -0.3129968654442937814 ) ) ;
#5202=EDGE_CURVE ( 'NONE', #60255, #183115, #50764, .T. ) ;
#5209=CARTESIAN_POINT ( 'NONE',  ( 1.899821779672239419, 8.994870868756308369, -0.7749999999999996891 ) ) ;
#5218=CARTESIAN_POINT ( 'NONE',  ( 5.574337433874081427, 6.532423756721743580, -1.199719254218452047 ) ) ;
#5227=CARTESIAN_POINT ( 'NONE',  ( 5.580062740476173566, 8.667767742934335828, 1.199719254218451159 ) ) ;
#5229=CARTESIAN_POINT ( 'NONE',  ( 5.559725510055676168, 8.644040974110419384, 1.199719254218451159 ) ) ;
#5241=CARTESIAN_POINT ( 'NONE',  ( 6.093313910611117379, 7.014445836765536235, -0.9825430356366869900 ) ) ;
#5243=CARTESIAN_POINT ( 'NONE',  ( 6.224601922449876312, 6.434659462379210382, 0.000000000000000000 ) ) ;
#5245=B_SPLINE_CURVE_WITH_KNOTS ( 'NONE', 3,
 ( #15324, #153623, #169858, #51049, #47881, #116099 ),
 .UNSPECIFIED., .F., .F.,
 ( 4, 2, 4 ),
 ( 0.000000000000000000, 0.002403937268455933786, 0.004807874536911865837 ),
 .UNSPECIFIED. ) ;
#5251=CARTESIAN_POINT ( 'NONE',  ( -4.496464221587651799, 5.274905009054215554, 1.199719254218452935 ) ) ;
#5256=CARTESIAN_POINT ( 'NONE',  ( 0.3910932212915787520, 3.280071935319364584, -1.963192794826990495 ) ) ;
#5261=CARTESIAN_POINT ( 'NONE',  ( -5.777182852754558340, 5.912670547734647286, 0.000000000000000000 ) ) ;
#5266=CARTESIAN_POINT ( 'NONE',  ( 5.722423353419669567, 8.833855124701747386, 1.199719254218451159 ) ) ;
#5274=DIRECTION ( 'NONE',  ( 0.000000000000000000, 1.000000000000000000, 0.000000000000000000 ) ) ;
#5300=EDGE_LOOP ( 'NONE', ( #79413, #9856, #93170, #114096 ) ) ;
#5321=CARTESIAN_POINT ( 'NONE',  ( 4.177320726786311056, 5.966903162707725805, -1.443375672974068769 ) ) ;
#5329=CARTESIAN_POINT ( 'NONE',  ( 5.580062740476173566, 8.667767742934335828, 1.199719254218451159 ) ) ;
#5332=CARTESIAN_POINT ( 'NONE',  ( -5.817857314039913241, 5.960124085900898372, 0.000000000000000000 ) ) ;
#5343=AXIS2_PLACEMENT_3D ( 'NONE', #191787, #206976, #175571 ) ;
#5364=CARTESIAN_POINT ( 'NONE',  ( 7.363486825997814123, 7.763358516518489516, 0.000000000000000000 ) ) ;
#5379=CARTESIAN_POINT ( 'NONE',  ( -4.326460416536637155, 8.061637896019123062, 0.000000000000000000 ) ) ;
#5383=CARTESIAN_POINT ( 'NONE',  ( 5.515134625708930649, 9.656350506627580543, 0.000000000000000000 ) ) ;
#5388=CARTESIAN_POINT ( 'NONE',  ( -4.359828915246279024, 7.244161613499399799, -1.199719254218455378 ) ) ;
#5389=CARTESIAN_POINT ( 'NONE',  ( 7.065207446497155708, 9.336104335703744539, 0.000000000000000000 ) ) ;
#5397=DIRECTION ( 'NONE',  ( -1.000000000000000000, 0.000000000000000000, 0.000000000000000000 ) ) ;
#5432=CARTESIAN_POINT ( 'NONE',  ( -6.577640801285370209, 7.702944352034914566, -1.199719254218452047 ) ) ;
#5436=CARTESIAN_POINT ( 'NONE',  ( -4.936050443827081580, 7.916420063510339666, 1.199719254218452935 ) ) ;
#5441=CARTESIAN_POINT ( 'NONE',  ( -7.892254816486440561, 8.380254505421877553, 0.000000000000000000 ) ) ;
#5442=CARTESIAN_POINT ( 'NONE',  ( 6.902509602688803980, 9.146290184594002781, -1.443375672974064550 ) ) ;
#5448=CARTESIAN_POINT ( 'NONE',  ( -3.169574050544739841, 6.919863168935977527, -0.7998128361456481317 ) ) ;
#5455=CARTESIAN_POINT ( 'NONE',  ( -5.935437387732586778, 10.14670372898850381, -0.7998128361456362523 ) ) ;
#5456=EDGE_LOOP ( 'NONE', ( #57254, #59418, #188811, #140618 ) ) ;
#5457=CARTESIAN_POINT ( 'NONE',  ( 4.749341595749815070, 8.305088035112140332, 0.7662636247844747395 ) ) ;
#5460=CARTESIAN_POINT ( 'NONE',  ( 4.370663978927085580, 5.060324124126027279, -1.009771797811724214 ) ) ;
#5462=CARTESIAN_POINT ( 'NONE',  ( 6.481679955784983349, 9.719654494127929922, -1.199719254218452047 ) ) ;
#5474=CARTESIAN_POINT ( 'NONE',  ( -7.747558435566414659, 8.003516027774422170, -0.7998128361456362523 ) ) ;
#5486=CARTESIAN_POINT ( 'NONE',  ( 7.126746022638799971, 8.343567110280638133, 1.199719254218452047 ) ) ;
#5498=CARTESIAN_POINT ( 'NONE',  ( -0.3706017150059756071, 3.173913102025869737, -2.032929028842745733 ) ) ;
#5499=CARTESIAN_POINT ( 'NONE',  ( 6.564609147483420060, 6.793222102749934876, 0.3624652974001541517 ) ) ;
#5525=CARTESIAN_POINT ( 'NONE',  ( -6.387810837761664473, 6.908839790476999809, 0.8166356711787735589 ) ) ;
#5544=CARTESIAN_POINT ( 'NONE',  ( -5.257529707049291900, 9.355811434857983500, 0.7998128361456291469 ) ) ;
#5561=CARTESIAN_POINT ( 'NONE',  ( 4.248501033035879004, 6.049946853332221153, -1.599625672291273171 ) ) ;
#5565=CARTESIAN_POINT ( 'NONE',  ( 5.095443103064356549, 4.909381473188671130, 0.08826871305007774615 ) ) ;
#5578=CARTESIAN_POINT ( 'NONE',  ( 6.066347387471824781, 6.042103138330730872, -0.7998128361456481317 ) ) ;
#5589=CARTESIAN_POINT ( 'NONE',  ( -5.842637852846353397, 5.781108681267656202, 0.7998128361456281477 ) ) ;
#5590=CARTESIAN_POINT ( 'NONE',  ( 4.004454267989866700, 5.765225627445230927, 1.599625672291262513 ) ) ;
#5594=CARTESIAN_POINT ( 'NONE',  ( -6.473091995881817162, 6.516638514809040217, 0.7998128361456281477 ) ) ;
#5596=CARTESIAN_POINT ( 'NONE',  ( 6.658989722967328717, 7.797851427330578566, 1.199719254218452935 ) ) ;
#5601=CARTESIAN_POINT ( 'NONE',  ( -4.586114404036374381, 8.497146329035404122, -0.08355658565369419866 ) ) ;
#5610=CARTESIAN_POINT ( 'NONE',  ( -5.275531169048909952, 7.248148678680751189, -1.443375672974066548 ) ) ;
#5623=CARTESIAN_POINT ( 'NONE',  ( 4.041739190649647817, 6.769093918182960579, -1.082531754730548412 ) ) ;
#5626=CARTESIAN_POINT ( 'NONE',  ( -5.586841817283045408, 8.675676665875643678, 1.199719254218454489 ) ) ;
#5640=CARTESIAN_POINT ( 'NONE',  ( 3.627688620108284745, 6.389997935838436227, 1.199719254218452047 ) ) ;
#5667=CARTESIAN_POINT ( 'NONE',  ( -5.234856708652269042, 7.200695141551334721, 1.443375672974058777 ) ) ;
#5693=CARTESIAN_POINT ( 'NONE',  ( -6.794571259104023930, 7.956029886156682274, 1.199719254218452047 ) ) ;
#5695=CARTESIAN_POINT ( 'NONE',  ( 6.821160681006781523, 9.051383109298340557, 1.443375672974063439 ) ) ;
#5700=CARTESIAN_POINT ( 'NONE',  ( -5.320648938720212051, 5.172121614787156929, 0.000000000000000000 ) ) ;
#5703=CARTESIAN_POINT ( 'NONE',  ( 5.885648082108199119, 6.999582529615296700, 1.082531754730549967 ) ) ;
#5708=CARTESIAN_POINT ( 'NONE',  ( -4.625266680917477835, 5.425174544939014964, -1.199719254218453823 ) ) ;
#5710=CARTESIAN_POINT ( 'NONE',  ( 5.300918301777743480, 7.749796750553542779, -1.302405036909856761 ) ) ;
#5714=CARTESIAN_POINT ( 'NONE',  ( 5.123001941117305336, 7.070197912760590064, 1.599625672291268286 ) ) ;
#5720=CARTESIAN_POINT ( 'NONE',  ( -7.123883369337781879, 7.275895117174344229, 0.7998128361456341429 ) ) ;
#5723=CARTESIAN_POINT ( 'NONE',  ( -3.902768115887413014, 5.646591783325653147, -1.599625672291283607 ) ) ;
#5726=CARTESIAN_POINT ( 'NONE',  ( 4.692530564105613422, 7.528350520548263702, -1.082531754730548412 ) ) ;
#5727=CARTESIAN_POINT ( 'NONE',  ( 5.546694241322223107, 5.643767167730274537, -0.7216878364870458196 ) ) ;
#5728=CARTESIAN_POINT ( 'NONE',  ( -5.112833325684920993, 6.097965313788082931, -1.082531754730549967 ) ) ;
#5735=CARTESIAN_POINT ( 'NONE',  ( 5.174371902270911150, 6.065797303184739420, 1.199719254218452047 ) ) ;
#5748=CARTESIAN_POINT ( 'NONE',  ( 5.669760509565840323, 7.437725440679550992, 1.325564871123290356 ) ) ;
#5751=CARTESIAN_POINT ( 'NONE',  ( 0.4461838333974484927, 2.877219473291486640, 1.949594826320268481 ) ) ;
#5757=CARTESIAN_POINT ( 'NONE',  ( 6.710359684120930091, 6.793450817754725257, 0.7998128361456352531 ) ) ;
#5767=CARTESIAN_POINT ( 'NONE',  ( 6.307155384238837037, 6.868572428096745064, 0.7081091520576547893 ) ) ;
#5786=CARTESIAN_POINT ( 'NONE',  ( -6.954406449166956605, 7.078172043641714595, -0.7998128361456362523 ) ) ;
#5791=CARTESIAN_POINT ( 'NONE',  ( -3.746784212325278141, 7.355493017976345804, 0.6363135798663853704 ) ) ;
#5800=CARTESIAN_POINT ( 'NONE',  ( 6.384963997392946844, 6.413822516572072807, 0.7998128361456352531 ) ) ;
#5811=CARTESIAN_POINT ( 'NONE',  ( 4.913904330310220558, 4.697586238308844919, 0.000000000000000000 ) ) ;
#5815=CARTESIAN_POINT ( 'NONE',  ( 5.370438244344566847, 5.438135171256338829, 0.000000000000000000 ) ) ;
#5823=DIRECTION ( 'NONE',  ( 1.000000000000000000, -3.135042426464105837E-15, 0.000000000000000000 ) ) ;
#5834=CARTESIAN_POINT ( 'NONE',  ( -5.478903473698241378, 9.406154796041011679, -0.7216878364870338292 ) ) ;
#5835=CARTESIAN_POINT ( 'NONE',  ( 6.888951449519509218, 7.209733910627123876, -0.7216878364870317197 ) ) ;
#5844=ORIENTED_EDGE ( 'NONE', *, *, #102451, .F. ) ;
#5845=CARTESIAN_POINT ( 'NONE',  ( -4.960304097753355457, 6.880383762169266504, 1.599625672291263179 ) ) ;
#5846=CARTESIAN_POINT ( 'NONE',  ( -3.634467696915153034, 6.397906858779740524, 1.199719254218452935 ) ) ;
#5849=CARTESIAN_POINT ( 'NONE',  ( 5.519577934094851202, 8.493239118869080784, 1.082531754730547524 ) ) ;
#5859=CARTESIAN_POINT ( 'NONE',  ( -4.640257700270903563, 8.337993449908045918, -0.3781808898682629261 ) ) ;
#5863=CARTESIAN_POINT ( 'NONE',  ( 5.289089323106923146, 6.303597310780433283, -1.082531754730548412 ) ) ;
#5867=CARTESIAN_POINT ( 'NONE',  ( -6.479871072688648148, 6.524547437750345402, 0.000000000000000000 ) ) ;
#5878=CARTESIAN_POINT ( 'NONE',  ( 5.123001941117305336, 7.070197912760590064, 1.599625672291268286 ) ) ;
#5916=CARTESIAN_POINT ( 'NONE',  ( 5.966997003790217136, 8.054858819212300958, -1.443375672974078761 ) ) ;
#5923=CARTESIAN_POINT ( 'NONE',  ( 5.356880090730850696, 9.263794182579101033, 0.7216878364870317197 ) ) ;
#5938=CARTESIAN_POINT ( 'NONE',  ( -7.608060475923978494, 8.905100639113307182, 1.199719254218452047 ) ) ;
#5950=CARTESIAN_POINT ( 'NONE',  ( 3.879041346841291649, 7.539648981374564407, 1.040834085586084257E-14 ) ) ;
#5956=CARTESIAN_POINT ( 'NONE',  ( -6.050681693448748177, 10.28115541899069463, 0.7998128361456291469 ) ) ;
#5961=CARTESIAN_POINT ( 'NONE',  ( -6.617788377246196951, 7.853746207276256719, -1.082531754730549967 ) ) ;
#5965=CARTESIAN_POINT ( 'NONE',  ( -7.425025402139490360, 8.691559719698066289, 1.199719254218452047 ) ) ;
#5970=CARTESIAN_POINT ( 'NONE',  ( -4.984557751679625781, 5.844347460828191565, 1.199719254218452935 ) ) ;
#5985=CARTESIAN_POINT ( 'NONE',  ( -4.990809943606281607, 6.915973915664348937, -1.443375672974066548 ) ) ;
#5987=CARTESIAN_POINT ( 'NONE',  ( -5.600926855776901192, 5.707038551260711579, -0.7216878364870338292 ) ) ;
#5989=CARTESIAN_POINT ( 'NONE',  ( 4.389807875774629942, 8.343469298370917997, 0.7998128361456271485 ) ) ;
#5990=CARTESIAN_POINT ( 'NONE',  ( -6.981522756394290319, 7.109807735406931783, 0.7998128361456341429 ) ) ;
#5991=CARTESIAN_POINT ( 'NONE',  ( -6.200875153403786477, 8.327716660428123419, -1.599625672291271394 ) ) ;
#6012=CARTESIAN_POINT ( 'NONE',  ( 5.037736595929563244, 8.035053907629919223, -1.199719254218452047 ) ) ;
#6039=CARTESIAN_POINT ( 'NONE',  ( 5.085343294144600179, 4.914812813773358435, 0.1758235994440172922 ) ) ;
#6040=CARTESIAN_POINT ( 'NONE',  ( -1.855128211190531395, 8.960462962215050453, -0.7749999999999996891 ) ) ;
#6047=ORIENTED_EDGE ( 'NONE', *, *, #50358, .F. ) ;
#6051=CARTESIAN_POINT ( 'NONE',  ( 6.008198349511364000, 7.038594824965278995, 1.199719254218453823 ) ) ;
#6054=LINE ( 'NONE', #55898, #37491 ) ;
#6069=CARTESIAN_POINT ( 'NONE',  ( 4.258142763143749399, 7.125527769379820242, 1.199719254218451159 ) ) ;
#6074=CARTESIAN_POINT ( 'NONE',  ( -5.250750630242457362, 9.347902511916677426, 0.000000000000000000 ) ) ;
#6078=CARTESIAN_POINT ( 'NONE',  ( 6.086684617892325733, 6.065829907154645539, -0.7998128361456481317 ) ) ;
#6086=ADVANCED_FACE ( 'NONE', ( #204780 ), #118293, .F. ) ;
#6090=CARTESIAN_POINT ( 'NONE',  ( 5.370438244788902971, 9.279612028980123384, -0.7216878364870458196 ) ) ;
#6092=CARTESIAN_POINT ( 'NONE',  ( -5.343321937561608337, 5.406499480009534508, 0.7216878364870257245 ) ) ;
#6093=CARTESIAN_POINT ( 'NONE',  ( -6.934069218746458318, 7.054445274817795486, -0.7998128361456362523 ) ) ;
#6104=CARTESIAN_POINT ( 'NONE',  ( 6.378184920586140727, 6.405913593630768510, 0.000000000000000000 ) ) ;
#6105=CARTESIAN_POINT ( 'NONE',  ( 6.059568310664962709, 6.034194215389424798, 0.7998128361456352531 ) ) ;
#6123=CARTESIAN_POINT ( 'NONE',  ( 5.662876554447811017, 7.443216037249618999, -1.326882488215734845 ) ) ;
#6132=CARTESIAN_POINT ( 'NONE',  ( 5.086243903782109221, 5.962981304947771122, -1.199719254218452047 ) ) ;
#6136=CARTESIAN_POINT ( 'NONE',  ( 5.110497557708379546, 4.926945003606695295, -0.7998128361456481317 ) ) ;
#6140=CARTESIAN_POINT ( 'NONE',  ( 6.238160076063542725, 6.450477308261824305, -0.7216878364870458196 ) ) ;
#6142=CARTESIAN_POINT ( 'NONE',  ( -4.145761110728687804, 8.058748072483927771, -0.7998128361456481317 ) ) ;
#6144=CARTESIAN_POINT ( 'NONE',  ( 3.203469434578891661, 6.959407783642502565, -0.7998128361456362523 ) ) ;
#6156=CARTESIAN_POINT ( 'NONE',  ( 6.361499291607088935, 6.832587723092125032, 0.6030276918116053153 ) ) ;
#6157=CARTESIAN_POINT ( 'NONE',  ( -6.563555762791521531, 9.711213252348503744, 1.082531754730549967 ) ) ;
#6166=CARTESIAN_POINT ( 'NONE',  ( 0.4134119952316945845, 3.004821906555924738, -2.020258976488587432 ) ) ;
#6178=VECTOR ( 'NONE', #132004, 1000.000000000000000 ) ;
#6188=ORIENTED_EDGE ( 'NONE', *, *, #207750, .F. ) ;
#6192=CARTESIAN_POINT ( 'NONE',  ( 6.156284269057003655, 9.340026192945279249, -1.199719254218452047 ) ) ;
#6194=CARTESIAN_POINT ( 'NONE',  ( 7.374709211190586089, 7.568525266002632534, 0.000000000000000000 ) ) ;
#6208=CARTESIAN_POINT ( 'NONE',  ( -3.935609729716867289, 7.813571461303467913, 0.7998128361456352531 ) ) ;
#6210=CARTESIAN_POINT ( 'NONE',  ( 6.549997608733495902, 7.774656977344789333, -1.082531754730548412 ) ) ;
#6220=CARTESIAN_POINT ( 'NONE',  ( -5.041653019435350380, 6.975290837464928728, -1.599625672291271394 ) ) ;
#6223=CARTESIAN_POINT ( 'NONE',  ( -5.180624094197616714, 5.216685329418210948, 0.7216878364870257245 ) ) ;
#6227=CARTESIAN_POINT ( 'NONE',  ( -3.851398154733808088, 6.650992392901508232, -1.199719254218450271 ) ) ;
#6236=EDGE_CURVE ( 'NONE', #94475, #67360, #7009, .T. ) ;
#6253=CARTESIAN_POINT ( 'NONE',  ( -3.955946960137363799, 7.837298230127379917, 0.7998128361456352531 ) ) ;
#6264=CARTESIAN_POINT ( 'NONE',  ( -6.245422037512663671, 7.006708691962935553, -1.003398212925192157 ) ) ;
#6271=DIRECTION ( 'NONE',  ( 0.6029061840396385819, 0.7978120914393070917, 0.000000000000000000 ) ) ;
#6279=CARTESIAN_POINT ( 'NONE',  ( -6.466312919074983512, 6.508729591867735031, -0.7998128361456362523 ) ) ;
#6286=DIRECTION ( 'NONE',  ( 0.000000000000000000, 1.000000000000000000, 0.000000000000000000 ) ) ;
#6297=CARTESIAN_POINT ( 'NONE',  ( 5.086243903782109221, 5.962981304947771122, -1.199719254218452047 ) ) ;
#6299=CARTESIAN_POINT ( 'NONE',  ( 3.987289958883693419, 7.308088843452864580, 0.8820050823528166051 ) ) ;
#6307=CARTESIAN_POINT ( 'NONE',  ( 7.374709211190586089, 7.568525266002632534, 0.000000000000000000 ) ) ;
#6309=CARTESIAN_POINT ( 'NONE',  ( 4.667750024854814050, 8.667735138964429709, -0.7998128361456381397 ) ) ;
#6322=CARTESIAN_POINT ( 'NONE',  ( 6.490673131624099312, 6.748652840683030618, -0.08655830178419705867 ) ) ;
#6324=CARTESIAN_POINT ( 'NONE',  ( 6.061904079085887354, 6.244845311787889486, 0.000000000000000000 ) ) ;
#6333=CARTESIAN_POINT ( 'NONE',  ( -3.149236820124241110, 6.896136400112061970, -0.7998128361456481317 ) ) ;
#6343=CARTESIAN_POINT ( 'NONE',  ( -5.058600711230246461, 7.955432358860325515, 1.082531754730549967 ) ) ;
#6347=CARTESIAN_POINT ( 'NONE',  ( 4.681308178468477799, 8.683552984847038303, 0.000000000000000000 ) ) ;
#6353=EDGE_CURVE ( 'NONE', #29314, #824, #190404, .T. ) ;
#6367=CARTESIAN_POINT ( 'NONE',  ( 6.879836604291781121, 6.991173891287354003, -0.7998128361456341429 ) ) ;
#6406=CARTESIAN_POINT ( 'NONE',  ( 5.289089323106923146, 6.303597310780433283, -1.082531754730548412 ) ) ;
#6411=CARTESIAN_POINT ( 'NONE',  ( -3.947104627881522720, 8.980740528188976057, -0.7749999999999979128 ) ) ;
#6413=CARTESIAN_POINT ( 'NONE',  ( 6.016786309414542622, 10.24161080428416426, 0.7998128361456341429 ) ) ;
#6417=CARTESIAN_POINT ( 'NONE',  ( -5.343321937561608337, 5.406499480009534508, 0.7216878364870257245 ) ) ;
#6422=CARTESIAN_POINT ( 'NONE',  ( -4.260029445439560192, 7.236136616047151193, 2.499999999999999556 ) ) ;
#6429=CARTESIAN_POINT ( 'NONE',  ( 4.787437639401280087, 6.678706227425192488, 0.000000000000000000 ) ) ;
#6446=CARTESIAN_POINT ( 'NONE',  ( 4.716257332707354699, 6.595662536282280719, -1.599625672291269396 ) ) ;
#6459=CARTESIAN_POINT ( 'NONE',  ( -6.468648687495877958, 6.719380688266201496, 0.000000000000000000 ) ) ;
#6462=CARTESIAN_POINT ( 'NONE',  ( 5.742760583840166966, 8.857581893525663830, 1.199719254218452047 ) ) ;
#6468=CARTESIAN_POINT ( 'NONE',  ( -3.793249116773374396, 7.647484079536056356, 0.7998128361456352531 ) ) ;
#6472=DIRECTION ( 'NONE',  ( 0.7592566023652990159, -0.6507913734559659380, 0.000000000000000000 ) ) ;
#6497=EDGE_LOOP ( 'NONE', ( #136821, #141895, #174489, #183087 ) ) ;
#6512=CARTESIAN_POINT ( 'NONE',  ( -6.933015448541747006, 9.181880338089085214, 1.599625672291269396 ) ) ;
#6515=CARTESIAN_POINT ( 'NONE',  ( -4.437261413422502798, 8.398831758960053406, 0.000000000000000000 ) ) ;
#6516=CARTESIAN_POINT ( 'NONE',  ( -5.061990249855849555, 6.999017606288843396, -1.599625672291271394 ) ) ;
#6520=CARTESIAN_POINT ( 'NONE',  ( -6.414416072596837104, 9.537216947121368804, -1.082531754730549967 ) ) ;
#6521=CARTESIAN_POINT ( 'NONE',  ( 6.983858524370772258, 9.241197259889668558, 1.443375672974063439 ) ) ;
#6527=CARTESIAN_POINT ( 'NONE',  ( -4.787964524281469458, 5.614988695530339413, -1.199719254218453823 ) ) ;
#6535=CARTESIAN_POINT ( 'NONE',  ( -6.149505192250180663, 9.332117270003974951, -1.199719254218452047 ) ) ;
#6536=ORIENTED_EDGE ( 'NONE', *, *, #201142, .T. ) ;
#6537=CARTESIAN_POINT ( 'NONE',  ( 5.088145468715395303, 7.830155539619080507, -1.136959649167136543 ) ) ;
#6542=CARTESIAN_POINT ( 'NONE',  ( 4.947799714344386146, 4.737130853015369958, -0.7998128361456481317 ) ) ;
#6552=CARTESIAN_POINT ( 'NONE',  ( -6.831329296439251131, 9.063246493969506545, -1.599625672291271394 ) ) ;
#6565=CARTESIAN_POINT ( 'NONE',  ( 3.573456005653643519, 6.326726552307992080, -1.199719254218453823 ) ) ;
#6573=CYLINDRICAL_SURFACE ( 'NONE', #33875, 1.250000000000000000 ) ;
#6574=CARTESIAN_POINT ( 'NONE',  ( 4.549612403093820312, 8.500000000000243361, -0.2314049244472246580 ) ) ;
#6578=CARTESIAN_POINT ( 'NONE',  ( -0.2366305240106678365, 2.663423291230584411, 2.061984645680444928 ) ) ;
#6579=CARTESIAN_POINT ( 'NONE',  ( 6.059925523928845870, 7.140772946495586915, 1.155538509043469997 ) ) ;
#6607=CARTESIAN_POINT ( 'NONE',  ( -6.533345026022147728, 6.811601368426168257, 0.5105341503897353750 ) ) ;
#6627=CARTESIAN_POINT ( 'NONE',  ( -5.607179047703544583, 8.699403434699558346, 1.199719254218454489 ) ) ;
#6647=CARTESIAN_POINT ( 'NONE',  ( 8.122743427918724279, 8.649157885426255632, 0.7216878364870267237 ) ) ;
#6657=EDGE_CURVE ( 'NONE', #194727, #183165, #94290, .T. ) ;
#6658=CARTESIAN_POINT ( 'NONE',  ( 4.834028091705433461, 8.209959199513299666, 0.9267959391740541175 ) ) ;
#6675=CARTESIAN_POINT ( 'NONE',  ( -3.955946960137363799, 7.837298230127379917, 0.7998128361456352531 ) ) ;
#6677=CARTESIAN_POINT ( 'NONE',  ( 5.248941747146098180, 6.152795455539095570, -1.199719254218452047 ) ) ;
#6680=CARTESIAN_POINT ( 'NONE',  ( -6.448838341955544173, 7.552674816150118708, 1.199719254218452047 ) ) ;
#6681=CARTESIAN_POINT ( 'NONE',  ( 3.231779075379137556, 6.036511184309975242, -0.9899555337401846344 ) ) ;
#6683=CARTESIAN_POINT ( 'NONE',  ( 5.905458427204159477, 9.047396044116986502, 1.199719254218452047 ) ) ;
#6690=CARTESIAN_POINT ( 'NONE',  ( -4.733024909954385073, 8.320217716143888609, 0.7565452571775049817 ) ) ;
#6699=CARTESIAN_POINT ( 'NONE',  ( -4.868786560638931782, 6.773613302202437403, 1.443375672974058777 ) ) ;
#6707=CARTESIAN_POINT ( 'NONE',  ( 3.106226591306694651, 6.638031766584184368, 0.000000000000000000 ) ) ;
#6711=CARTESIAN_POINT ( 'NONE',  ( -6.343235766347277149, 8.493804042195527870, -1.599625672291271394 ) ) ;
#6739=VERTEX_POINT ( 'NONE', #92160 ) ;
#6751=CARTESIAN_POINT ( 'NONE',  ( -4.340018570150309785, 7.117086527600392287, -1.082531754730551743 ) ) ;
#6773=CARTESIAN_POINT ( 'NONE',  ( -5.302647476276252547, 5.359045941843285199, 0.7216878364870257245 ) ) ;
#6779=CARTESIAN_POINT ( 'NONE',  ( -4.122561227007127016, 6.967349310553715647, 1.199719254218452935 ) ) ;
#6782=DIRECTION ( 'NONE',  ( 0.000000000000000000, -1.000000000000000000, 0.000000000000000000 ) ) ;
#6787=CARTESIAN_POINT ( 'NONE',  ( -5.191846479390389568, 5.021852078902356631, 0.7998128361456281477 ) ) ;
#6789=CARTESIAN_POINT ( 'NONE',  ( 6.604949037901548969, 6.766875157141204689, 0.08182522243922914218 ) ) ;
#6793=CARTESIAN_POINT ( 'NONE',  ( 5.554000203453580475, 6.508696987897830688, -1.199719254218452047 ) ) ;
#6799=CARTESIAN_POINT ( 'NONE',  ( -5.424143973919053785, 8.485862515284315677, 1.199719254218454489 ) ) ;
#6802=CARTESIAN_POINT ( 'NONE',  ( -4.442231607132987925, 5.211633625523774960, -1.199719254218453823 ) ) ;
#6807=CARTESIAN_POINT ( 'NONE',  ( 4.367134876933267407, 8.109091433148536865, 0.000000000000000000 ) ) ;
#6808=CARTESIAN_POINT ( 'NONE',  ( -5.031484404002922517, 6.963427452793760963, 1.443375672974058777 ) ) ;
#6812=CARTESIAN_POINT ( 'NONE',  ( -4.502189528189771472, 7.410248995266807803, -1.199719254218453823 ) ) ;
#6815=CARTESIAN_POINT ( 'NONE',  ( 3.691562964670865199, 7.528850235416478576, -0.7998128361456362523 ) ) ;
#6819=CARTESIAN_POINT ( 'NONE',  ( -4.489270214782448143, 8.251570750202326110, -0.005118047378703463254 ) ) ;
#6820=CARTESIAN_POINT ( 'NONE',  ( 2.969872605471521432, 6.598710015541000118, -0.2115686265727617921 ) ) ;
#6822=CARTESIAN_POINT ( 'NONE',  ( 4.583538449871731757, 7.505156070562471804, 1.199719254218451159 ) ) ;
#6827=CARTESIAN_POINT ( 'NONE',  ( 4.812217717264355876, 8.234349973070900219, 0.8868998539744571419 ) ) ;
#6837=CARTESIAN_POINT ( 'NONE',  ( 6.038177310039780643, 8.137902509836795417, -1.599625672291283607 ) ) ;
#6847=CARTESIAN_POINT ( 'NONE',  ( 5.448178351099921102, 7.506598249424609293, 1.250114376932524252 ) ) ;
#6864=CARTESIAN_POINT ( 'NONE',  ( -5.769876891067536206, 8.889217585290882795, 1.199719254218454489 ) ) ;
#6878=CARTESIAN_POINT ( 'NONE',  ( 5.254667053748194760, 8.288139441751686931, 1.199719254218452047 ) ) ;
#6886=CARTESIAN_POINT ( 'NONE',  ( 4.577813143269636065, 5.369812084349879555, -1.199719254218450271 ) ) ;
#6889=CARTESIAN_POINT ( 'NONE',  ( 5.682275777458854371, 5.801945626556378244, 0.7216878364870328300 ) ) ;
#6899=DIRECTION ( 'NONE',  ( 0.6507913734559640506, -0.7592566023653003482, 0.000000000000000000 ) ) ;
#6904=CARTESIAN_POINT ( 'NONE',  ( -5.451787166470911217, 9.374519104275787384, 0.7216878364870267237 ) ) ;
#6905=CARTESIAN_POINT ( 'NONE',  ( 7.377044979611483200, 7.779176362401098999, -0.7216878364870317197 ) ) ;
#6915=CARTESIAN_POINT ( 'NONE',  ( -5.472651281771599763, 6.413789912602166687, 1.199719254218452935 ) ) ;
#6916=CARTESIAN_POINT ( 'NONE',  ( -3.797165540279144214, 6.587721009371067638, 1.199719254218452935 ) ) ;
#6918=CARTESIAN_POINT ( 'NONE',  ( 6.672020991256494504, 6.956648375986938859, 0.000000000000000000 ) ) ;
#6930=CARTESIAN_POINT ( 'NONE',  ( -4.604539980425653489, 8.383423159197839425, -0.07723066608773809794 ) ) ;
#6933=CARTESIAN_POINT ( 'NONE',  ( 6.061904079085887354, 6.244845311787889486, 0.000000000000000000 ) ) ;
#6938=CARTESIAN_POINT ( 'NONE',  ( -7.117104292530948229, 7.267986194233038155, -0.7998128361456362523 ) ) ;
#6950=CARTESIAN_POINT ( 'NONE',  ( 3.881377115262159894, 7.750300077773022878, 0.7998128361456271485 ) ) ;
#6983=EDGE_CURVE ( 'NONE', #154266, #99737, #40279, .T. ) ;
#6986=CARTESIAN_POINT ( 'NONE',  ( 5.383996398402570271, 9.295429874862735531, 0.000000000000000000 ) ) ;
#6991=CARTESIAN_POINT ( 'NONE',  ( 6.604230223188150894, 9.758666789477915771, -1.082531754730548412 ) ) ;
#7009=B_SPLINE_CURVE_WITH_KNOTS ( 'NONE', 3,
 ( #69454, #71586, #39117, #18583, #202653, #68388, #19651 ),
 .UNSPECIFIED., .F., .F.,
 ( 4, 3, 4 ),
 ( 3.172092245977020233E-15, 6.255038410197399793E-05, 0.0001580841567447031405 ),
 .UNSPECIFIED. ) ;
#7018=CARTESIAN_POINT ( 'NONE',  ( -5.517242166118370150, 5.401480380085008193, 0.7998128361456281477 ) ) ;
#7020=CARTESIAN_POINT ( 'NONE',  ( 6.333067150914820864, 6.561202228921677815, 0.7216878364870328300 ) ) ;
#7026=CARTESIAN_POINT ( 'NONE',  ( -4.842197138736131556, 5.678260079060780008, 1.199719254218452935 ) ) ;
#7030=CARTESIAN_POINT ( 'NONE',  ( -6.400857919427531684, 9.521399101757175742, 1.082531754730549967 ) ) ;
#7033=CARTESIAN_POINT ( 'NONE',  ( -4.207966135563095733, 7.175396087857926375, 7.500000000000000000 ) ) ;
#7038=CARTESIAN_POINT ( 'NONE',  ( -5.635349125135588721, 6.603604063193491136, 1.199719254218452935 ) ) ;
#7048=CARTESIAN_POINT ( 'NONE',  ( -2.823841133396259639, 6.516508098929413961, -0.7998128361456481317 ) ) ;
#7051=CARTESIAN_POINT ( 'NONE',  ( 2.989799202408753853, 6.433716316886197717, 0.3763814980636948637 ) ) ;
#7054=CARTESIAN_POINT ( 'NONE',  ( -3.512971199716682591, 7.112567143062499930, 0.000000000000000000 ) ) ;
#7055=VERTEX_POINT ( 'NONE', #178820 ) ;
#7056=CARTESIAN_POINT ( 'NONE',  ( -6.604230223188181093, 6.877559146573883453, 0.7216878364870317197 ) ) ;
#7057=CARTESIAN_POINT ( 'NONE',  ( 6.412080304620304538, 6.445458208337293549, -0.7998128361456481317 ) ) ;
#7058=CARTESIAN_POINT ( 'NONE',  ( -4.444040490229335560, 8.406740681901359480, 0.7998128361456352531 ) ) ;
#7059=CARTESIAN_POINT ( 'NONE',  ( -7.469616286486262524, 7.679250187180907794, 0.7998128361456341429 ) ) ;
#7079=CARTESIAN_POINT ( 'NONE',  ( 5.840530312436913007, 10.03597880781023299, 0.000000000000000000 ) ) ;
#7119=CARTESIAN_POINT ( 'NONE',  ( 5.061990249855835344, 6.999017606288844284, -1.599625672291273171 ) ) ;
#7122=CARTESIAN_POINT ( 'NONE',  ( -4.004454267989906668, 5.765225627445230927, 1.599625672291270506 ) ) ;
#7137=CARTESIAN_POINT ( 'NONE',  ( 6.052789233858158369, 6.026285292448116948, 0.000000000000000000 ) ) ;
#7145=CARTESIAN_POINT ( 'NONE',  ( -6.424584688029276514, 8.588711117491191871, 1.599625672291269396 ) ) ;
#7150=CARTESIAN_POINT ( 'NONE',  ( 5.896870467300973750, 5.844380064798101237, 0.7998128361456352531 ) ) ;
#7155=DIRECTION ( 'NONE',  ( 0.000000000000000000, 1.496258514059622730E-16, -1.000000000000000000 ) ) ;
#7161=CARTESIAN_POINT ( 'NONE',  ( 6.034787771858531435, 10.05468647722803865, 0.000000000000000000 ) ) ;
#7163=CARTESIAN_POINT ( 'NONE',  ( -4.828112100242294424, 5.765790550771681566, -1.082531754730549967 ) ) ;
#7164=CARTESIAN_POINT ( 'NONE',  ( -6.557303570864871034, 7.679217583210999010, -1.199719254218452047 ) ) ;
#7175=CARTESIAN_POINT ( 'NONE',  ( 5.367048706163317640, 7.354919138647580290, -1.599625672291281386 ) ) ;
#7176=CARTESIAN_POINT ( 'NONE',  ( 6.737475991348287785, 6.825086509519945999, -0.7998128361456481317 ) ) ;
#7179=CARTESIAN_POINT ( 'NONE',  ( 7.550965208168244125, 7.774157262476569130, -0.7998128361456341429 ) ) ;
#7198=CARTESIAN_POINT ( 'NONE',  ( 5.585032934186686226, 5.480569609498057382, 0.000000000000000000 ) ) ;
#7202=CARTESIAN_POINT ( 'NONE',  ( 4.224247379109608680, 7.085983154673295203, -1.199719254218452047 ) ) ;
#7207=CARTESIAN_POINT ( 'NONE',  ( 5.982890925380405456, 10.20206618957764100, 0.000000000000000000 ) ) ;
#7211=CARTESIAN_POINT ( 'NONE',  ( 4.421367491832258523, 8.172362817197399210, 0.7216878364870257245 ) ) ;
#7213=CARTESIAN_POINT ( 'NONE',  ( -5.794130544993808307, 7.853181283949808744, 1.599625672291263179 ) ) ;
#7215=CARTESIAN_POINT ( 'NONE',  ( 6.861835142292135536, 9.098836647464588978, 1.443375672974065660 ) ) ;
#7216=ORIENTED_EDGE ( 'NONE', *, *, #4999, .F. ) ;
#7225=CARTESIAN_POINT ( 'NONE',  ( -7.919371124158132602, 8.411890197705517380, -0.7216878364870338292 ) ) ;
#7244=EDGE_CURVE ( 'NONE', #63064, #109831, #112400, .T. ) ;
#7245=EDGE_LOOP ( 'NONE', ( #76066, #19170, #76185, #121161, #170992, #129106, #195463, #46906, #32354, #38643, #43676, #201622, #71640, #97228, #116706, #543, #72477, #42284, #138579, #164376 ) ) ;
#7250=CIRCLE ( 'NONE', #166374, 2.080000000000000071 ) ;
#7260=CARTESIAN_POINT ( 'NONE',  ( 5.982890925380405456, 10.20206618957764100, 0.000000000000000000 ) ) ;
#7262=CARTESIAN_POINT ( 'NONE',  ( 6.339319342841494453, 9.553567112360518365, -1.199719254218452047 ) ) ;
#7268=EDGE_CURVE ( 'NONE', #9317, #157271, #151758, .T. ) ;
#7275=CARTESIAN_POINT ( 'NONE',  ( -5.424143973919053785, 8.485862515284315677, 1.199719254218454489 ) ) ;
#7277=CARTESIAN_POINT ( 'NONE',  ( 6.983858524370782916, 7.320458831286981827, 0.7216878364870328300 ) ) ;
#7287=CARTESIAN_POINT ( 'NONE',  ( -4.773352600463090845, 7.726605912919016106, 1.199719254218452935 ) ) ;
#7292=CARTESIAN_POINT ( 'NONE',  ( -3.011319516011047082, 6.527306845405913549, 0.7216878364870328300 ) ) ;
#7296=CARTESIAN_POINT ( 'NONE',  ( -5.008811405605897882, 4.808311159487113073, 0.7998128361456281477 ) ) ;
#7321=CARTESIAN_POINT ( 'NONE',  ( -5.143339171537843590, 7.093924681584509173, 1.599625672291263179 ) ) ;
#7324=CARTESIAN_POINT ( 'NONE',  ( -4.787964524281469458, 5.614988695530339413, -1.199719254218453823 ) ) ;
#7348=CARTESIAN_POINT ( 'NONE',  ( -5.119085517611572378, 8.129960982925583224, 1.199719254218452935 ) ) ;
#7364=CARTESIAN_POINT ( 'NONE',  ( -5.793963627187476817, 6.347147481417366066, 0.7933461710243456810 ) ) ;
#7368=CARTESIAN_POINT ( 'NONE',  ( 4.655245641445829641, 6.524482229810530498, 1.599625672291269396 ) ) ;
#7376=CARTESIAN_POINT ( 'NONE',  ( 5.528692779322568640, 9.672168352510192690, 0.7998128361456341429 ) ) ;
#7378=CARTESIAN_POINT ( 'NONE',  ( 6.692885107001518286, 7.837396042037102717, -1.199719254218452047 ) ) ;
#7387=CARTESIAN_POINT ( 'NONE',  ( 4.393008644795362905, 7.016788222801661590, 1.284222742053114041 ) ) ;
#7391=CARTESIAN_POINT ( 'NONE',  ( 6.400493444083267036, 6.807005473012165631, 0.5116258143813920967 ) ) ;
#7394=CARTESIAN_POINT ( 'NONE',  ( 6.712695452541852070, 7.004101914153185504, 0.000000000000000000 ) ) ;
#7401=CARTESIAN_POINT ( 'NONE',  ( -3.363304624641834106, 6.081549941127532222, -1.199719254218452047 ) ) ;
#7404=ORIENTED_EDGE ( 'NONE', *, *, #207587, .F. ) ;
#7411=CARTESIAN_POINT ( 'NONE',  ( -5.275531169048909952, 7.248148678680751189, -1.443375672974066548 ) ) ;
#7432=CARTESIAN_POINT ( 'NONE',  ( -5.952598981286905122, 7.203796195765662880, -1.286163493473730934 ) ) ;
#7434=CARTESIAN_POINT ( 'NONE',  ( 6.801350335910821165, 7.963938809097990124, 1.199719254218452047 ) ) ;
#7458=FACE_OUTER_BOUND ( 'NONE', #209093, .T. ) ;
#7476=CARTESIAN_POINT ( 'NONE',  ( 4.041739190649647817, 6.769093918182960579, -1.082531754730548412 ) ) ;
#7486=CARTESIAN_POINT ( 'NONE',  ( -5.329763783947941036, 5.390681634126922361, 0.000000000000000000 ) ) ;
#7517=CARTESIAN_POINT ( 'NONE',  ( 3.054329744828568227, 6.785411478933790264, 0.000000000000000000 ) ) ;
#7520=DIRECTION ( 'NONE',  ( 0.9829311923673920148, -0.1839735607939816386, 0.000000000000000000 ) ) ;
#7522=EDGE_CURVE ( 'NONE', #7836, #136449, #86622, .T. ) ;
#7530=CARTESIAN_POINT ( 'NONE',  ( -6.672020991700860826, 7.917017590806697314, 1.082531754730549078 ) ) ;
#7532=CARTESIAN_POINT ( 'NONE',  ( 6.875920180786008196, 8.050936961452347163, -1.199719254218452047 ) ) ;
#7550=CARTESIAN_POINT ( 'NONE',  ( -5.153507786970285665, 5.185049637652990207, -0.7216878364870338292 ) ) ;
#7584=CARTESIAN_POINT ( 'NONE',  ( -6.394605727500880299, 7.489403432619674561, -1.199719254218452047 ) ) ;
#7585=CARTESIAN_POINT ( 'NONE',  ( -4.471156797456669274, 8.438376373666580221, -0.7998128361456361413 ) ) ;
#7589=CARTESIAN_POINT ( 'NONE',  ( -7.743115126736118015, 8.206258200713163475, 0.7216878364870317197 ) ) ;
#7590=CARTESIAN_POINT ( 'NONE',  ( 8.122743427918724279, 8.649157885426255632, 0.7216878364870267237 ) ) ;
#7596=CARTESIAN_POINT ( 'NONE',  ( -2.830620210203090181, 6.524417021870718258, 0.000000000000000000 ) ) ;
#7605=CARTESIAN_POINT ( 'NONE',  ( -8.093291352714894415, 8.406871097780989288, -0.7998128361456362523 ) ) ;
#7607=CARTESIAN_POINT ( 'NONE',  ( 4.868750418105482147, 8.172599172502351905, -0.9747704861028365642 ) ) ;
#7610=CIRCLE ( 'NONE', #17959, 0.7499999999999997780 ) ;
#7611=CARTESIAN_POINT ( 'NONE',  ( -4.207966135563093957, 7.175396087857926375, -0.9899555337401829691 ) ) ;
#7613=CARTESIAN_POINT ( 'NONE',  ( 4.760848217054122422, 5.583353003765119560, -1.199719254218452047 ) ) ;
#7633=CARTESIAN_POINT ( 'NONE',  ( 6.156284269057003655, 9.340026192945279249, -1.199719254218452047 ) ) ;
#7650=CARTESIAN_POINT ( 'NONE',  ( 5.703612580814390043, 7.410739916031705121, 1.319003781635886163 ) ) ;
#7652=CARTESIAN_POINT ( 'NONE',  ( -4.950135482320926705, 6.868520377498098739, -1.443375672974066548 ) ) ;
#7673=VECTOR ( 'NONE', #205828, 1000.000000000000000 ) ;
#7679=CARTESIAN_POINT ( 'NONE',  ( 3.770049233051776749, 6.556085317605844232, 1.199719254218451159 ) ) ;
#7693=CARTESIAN_POINT ( 'NONE',  ( 3.576974914035945030, 7.342233597957815938, -0.3073933414947004894 ) ) ;
#7697=CARTESIAN_POINT ( 'NONE',  ( -4.769436176957319695, 8.786368983084006601, 0.7998128361456281477 ) ) ;
#7708=DIRECTION ( 'NONE',  ( 0.6095094443608750634, 0.000000000000000000, 0.7927788072564109223 ) ) ;
#7715=CARTESIAN_POINT ( 'NONE',  ( 5.598591087800349086, 5.496387455380669529, -0.7998128361456481317 ) ) ;
#7727=CARTESIAN_POINT ( 'NONE',  ( 5.931307043615195340, 7.129970210930432373, 1.110187140972586306 ) ) ;
#7743=ORIENTED_EDGE ( 'NONE', *, *, #62843, .F. ) ;
#7745=CARTESIAN_POINT ( 'NONE',  ( -5.354544322754380303, 5.211666229493680191, 0.7998128361456281477 ) ) ;
#7747=CARTESIAN_POINT ( 'NONE',  ( 4.603875680292229156, 7.528882839386387360, 1.199719254218452047 ) ) ;
#7750=CARTESIAN_POINT ( 'NONE',  ( -4.450819567036169211, 8.414649604842665553, -0.7998128361456362523 ) ) ;
#7754=CARTESIAN_POINT ( 'NONE',  ( 6.984385409695311964, 8.177479728513226576, 1.199719254218452935 ) ) ;
#7759=CARTESIAN_POINT ( 'NONE',  ( -5.679622069920094773, 7.427521650927588759, -1.335666627332438683 ) ) ;
#7766=CARTESIAN_POINT ( 'NONE',  ( -5.031484404002922517, 6.963427452793760963, 1.443375672974058777 ) ) ;
#7775=CARTESIAN_POINT ( 'NONE',  ( 4.367134877377630175, 7.148722219365612141, -1.082531754730548412 ) ) ;
#7779=CARTESIAN_POINT ( 'NONE',  ( -7.370792787684826486, 8.628288336167626582, -1.199719254218452047 ) ) ;
#7784=ORIENTED_EDGE ( 'NONE', *, *, #32673, .T. ) ;
#7799=CARTESIAN_POINT ( 'NONE',  ( -4.886220305951450626, 4.880249661270116057, -0.6067207380149993723 ) ) ;
#7821=CARTESIAN_POINT ( 'NONE',  ( -5.641601317062247212, 7.675230518029648508, -1.443375672974066548 ) ) ;
#7836=VERTEX_POINT ( 'NONE', #141820 ) ;
#7848=EDGE_LOOP ( 'NONE', ( #62901, #115179, #180099, #101146, #185364 ) ) ;
#7849=CARTESIAN_POINT ( 'NONE',  ( -4.678972410047611774, 5.591794245544547515, 1.082531754730549078 ) ) ;
#7854=AXIS2_PLACEMENT_3D ( 'NONE', #135107, #88484, #101514 ) ;
#7855=CARTESIAN_POINT ( 'NONE',  ( -4.659162064951642535, 5.464719159645540003, 1.199719254218452935 ) ) ;
#7859=CARTESIAN_POINT ( 'NONE',  ( 4.929342268689171469, 7.989555622611471897, -1.003472558803005565 ) ) ;
#7864=CARTESIAN_POINT ( 'NONE',  ( -3.318713740295064163, 7.093859473644694269, 0.000000000000000000 ) ) ;
#7866=CARTESIAN_POINT ( 'NONE',  ( 6.576141308597898139, 6.785670920958930985, -0.3094590540993913952 ) ) ;
#7870=CARTESIAN_POINT ( 'NONE',  ( 5.716698046817569434, 6.698511138489155137, -1.199719254218452047 ) ) ;
#7875=CARTESIAN_POINT ( 'NONE',  ( -6.074935347375019390, 9.245119117649618801, 1.199719254218452047 ) ) ;
#7879=CARTESIAN_POINT ( 'NONE',  ( -5.307090785106547415, 5.156303768904543894, -0.7998128361456362523 ) ) ;
#7884=CARTESIAN_POINT ( 'NONE',  ( 6.170369307550823912, 7.331757292631694511, 1.082531754730549967 ) ) ;
#7885=CARTESIAN_POINT ( 'NONE',  ( -4.407809337774280856, 7.196175756495025055, 1.082531754730549967 ) ) ;
#7892=CARTESIAN_POINT ( 'NONE',  ( 2.878073747850912412, 6.579779482459851003, -0.7998128361456362523 ) ) ;
#7903=CARTESIAN_POINT ( 'NONE',  ( 4.757636082118741783, 8.295611710538327799, 0.7840751985381082534 ) ) ;
#7914=CARTESIAN_POINT ( 'NONE',  ( 5.363132282657546490, 8.414682208812571673, -1.199719254218452047 ) ) ;
#7926=CARTESIAN_POINT ( 'NONE',  ( 6.297309100973213170, 6.875137029808006339, 0.7249047842670247599 ) ) ;
#7943=CARTESIAN_POINT ( 'NONE',  ( -6.526270840131767059, 8.707344961610770540, -1.599625672291271394 ) ) ;
#7947=DIRECTION ( 'NONE',  ( 0.7592566023653005702, 0.6507913734559639396, 0.000000000000000000 ) ) ;
#7955=CARTESIAN_POINT ( 'NONE',  ( 7.062871678076271920, 7.204714810702593120, -0.7998128361456341429 ) ) ;
#7959=CARTESIAN_POINT ( 'NONE',  ( -4.207966135563093957, 7.175396087857926375, 1.072179110320391260 ) ) ;
#7961=CARTESIAN_POINT ( 'NONE',  ( -6.089020385868850305, 10.11795786024005572, -0.7216878364870338292 ) ) ;
#7963=CARTESIAN_POINT ( 'NONE',  ( 4.740510986633625024, 5.559626234941203116, -1.199719254218450271 ) ) ;
#7966=CARTESIAN_POINT ( 'NONE',  ( 4.217995187182922656, 6.014356699837137832, 1.443375672974058777 ) ) ;
#7982=CARTESIAN_POINT ( 'NONE',  ( -7.160114521792834807, 8.486460042580672436, 1.082531754730549078 ) ) ;
#7983=CARTESIAN_POINT ( 'NONE',  ( 7.349928672384119288, 8.707909884937221179, 1.082531754730549967 ) ) ;
#7986=ADVANCED_FACE ( 'NONE', ( #210208 ), #166937, .T. ) ;
#7995=CARTESIAN_POINT ( 'NONE',  ( -4.111865726694519552, 8.019203457777400956, 0.000000000000000000 ) ) ;
#7996=CARTESIAN_POINT ( 'NONE',  ( -4.274563570058511175, 8.209017608368725405, 0.000000000000000000 ) ) ;
#7998=CARTESIAN_POINT ( 'NONE',  ( 6.821160681006793070, 7.130644680695653825, 0.7216878364870328300 ) ) ;
#8010=CARTESIAN_POINT ( 'NONE',  ( -5.005744162364479166, 7.928486884654230238, -1.069363714833789558 ) ) ;
#8014=CARTESIAN_POINT ( 'NONE',  ( 5.126391479742934187, 6.113783160189109722, -1.082531754730548412 ) ) ;
#8019=CARTESIAN_POINT ( 'NONE',  ( -6.954406449166956605, 7.078172043641714595, -0.7998128361456362523 ) ) ;
#8033=CARTESIAN_POINT ( 'NONE',  ( 5.727393547130178675, 5.646656991265468939, 0.000000000000000000 ) ) ;
#8037=( BOUNDED_CURVE ( )  B_SPLINE_CURVE ( 2, ( #98377, #62661, #29114, #128819, #79984, #65836, #213169 ),
 .UNSPECIFIED., .F., .T. ) 
 B_SPLINE_CURVE_WITH_KNOTS ( ( 3, 2, 2, 3 ),
 ( 0.3500000000000000888, 0.3583333333333335036, 0.3666666666666668628, 0.3750000000000002776 ),
 .UNSPECIFIED. ) 
 CURVE ( )  GEOMETRIC_REPRESENTATION_ITEM ( )  RATIONAL_B_SPLINE_CURVE ( ( 0.9999999999999982236, 0.8660254037844404840, 1.000000000000000000, 0.8660254037844387076, 1.000000000000000000, 0.8660254037844342667, 1.000000000000004441 ) ) 
 REPRESENTATION_ITEM ( '' )  );
#8042=FACE_OUTER_BOUND ( 'NONE', #164786, .T. ) ;
#8058=CARTESIAN_POINT ( 'NONE',  ( 5.346851039111009563, 6.199209027673978412, 1.092492203018504471 ) ) ;
#8075=CARTESIAN_POINT ( 'NONE',  ( 6.292392690518195941, 8.434487120394948079, -1.443375672974078761 ) ) ;
#8080=CARTESIAN_POINT ( 'NONE',  ( 5.492461626867537916, 9.421972641405202964, -0.7216878364870458196 ) ) ;
#8107=CARTESIAN_POINT ( 'NONE',  ( -5.815521545619021460, 5.749472989502435460, -0.7998128361456362523 ) ) ;
#8109=CARTESIAN_POINT ( 'NONE',  ( 6.197485614778188712, 6.403023770095574108, -0.7216878364870458196 ) ) ;
#8115=CARTESIAN_POINT ( 'NONE',  ( -3.494969737272722643, 7.299491470118629088, -0.7998128361456481317 ) ) ;
#8120=CARTESIAN_POINT ( 'NONE',  ( -5.750066545971566079, 8.762142499391876171, 1.082531754730550855 ) ) ;
#8124=CARTESIAN_POINT ( 'NONE',  ( -7.774674742793745708, 8.035151719539642912, 0.7998128361456341429 ) ) ;
#8128=CARTESIAN_POINT ( 'NONE',  ( -4.553559489343377287, 6.405848385690952718, -1.599625672291271394 ) ) ;
#8144=CARTESIAN_POINT ( 'NONE',  ( -6.156811154381562012, 6.355570232966157640, 0.7216878364870257245 ) ) ;
#8145=ORIENTED_EDGE ( 'NONE', *, *, #159414, .F. ) ;
#8146=CARTESIAN_POINT ( 'NONE',  ( -6.590672069574513792, 6.861741300691274859, 0.000000000000000000 ) ) ;
#8147=CARTESIAN_POINT ( 'NONE',  ( 5.091969210384201361, 8.098325291160362482, 1.199719254218452047 ) ) ;
#8148=CARTESIAN_POINT ( 'NONE',  ( -5.306037014901836990, 7.283738832175834510, 1.599625672291263179 ) ) ;
#8168=CARTESIAN_POINT ( 'NONE',  ( 5.515134625708930649, 9.656350506627580543, 0.000000000000000000 ) ) ;
#8202=CARTESIAN_POINT ( 'NONE',  ( 5.737035277238070385, 6.722237907313067140, -1.199719254218452047 ) ) ;
#8205=CARTESIAN_POINT ( 'NONE',  ( -2.830620210203090181, 6.524417021870718258, 0.000000000000000000 ) ) ;
#8208=CARTESIAN_POINT ( 'NONE',  ( -4.895902867866254837, 7.765618208269001066, 1.082531754730549967 ) ) ;
#8219=CARTESIAN_POINT ( 'NONE',  ( 4.085803189671889157, 5.860132702740892263, -1.599625672291273171 ) ) ;
#8220=CARTESIAN_POINT ( 'NONE',  ( 4.044074958626150185, 7.940114228364351767, 0.7998128361456271485 ) ) ;
#8234=CARTESIAN_POINT ( 'NONE',  ( 5.143339171537801846, 7.093924681584509173, 1.599625672291269396 ) ) ;
#8244=CARTESIAN_POINT ( 'NONE',  ( 7.024532985656136930, 8.328281583754568729, 1.082531754730549967 ) ) ;
#8245=CARTESIAN_POINT ( 'NONE',  ( -5.492461627311929995, 5.580495784718250363, 0.000000000000000000 ) ) ;
#8246=CARTESIAN_POINT ( 'NONE',  ( -6.882699257592852504, 8.058845884393651460, -1.199719254218452047 ) ) ;
#8257=CARTESIAN_POINT ( 'NONE',  ( 5.332099551924443404, 9.442809587212341427, 0.000000000000000000 ) ) ;
#8258=CARTESIAN_POINT ( 'NONE',  ( 6.690022453700429139, 6.769724048930809701, 0.7998128361456331437 ) ) ;
#8259=CARTESIAN_POINT ( 'NONE',  ( 7.201315867513990554, 8.430565262634994284, -1.199719254218452047 ) ) ;
#8262=CARTESIAN_POINT ( 'NONE',  ( 5.840530312436913007, 10.03597880781023299, 0.000000000000000000 ) ) ;
#8281=CARTESIAN_POINT ( 'NONE',  ( 4.655245641445829641, 6.524482229810530498, 1.599625672291269396 ) ) ;
#8282=DIRECTION ( 'NONE',  ( 0.000000000000000000, 1.000000000000000000, 0.000000000000000000 ) ) ;
#8283=CIRCLE ( 'NONE', #77555, 0.7499999999999997780 ) ;
#8285=CARTESIAN_POINT ( 'NONE',  ( 5.585032934186686226, 5.480569609498057382, 0.000000000000000000 ) ) ;
#8292=CARTESIAN_POINT ( 'NONE',  ( 7.828907357248368726, 8.098423103070084395, 0.7998128361456281477 ) ) ;
#8295=CARTESIAN_POINT ( 'NONE',  ( 6.536439455564168277, 6.798469917679251573, 0.7216878364870328300 ) ) ;
#8297=CARTESIAN_POINT ( 'NONE',  ( -6.981522756394290319, 7.109807735406931783, 0.7998128361456341429 ) ) ;
#8299=CARTESIAN_POINT ( 'NONE',  ( 5.727393547130178675, 5.646656991265468939, 0.000000000000000000 ) ) ;
#8307=CARTESIAN_POINT ( 'NONE',  ( -4.073660332270687690, 7.638349725183815053, -0.4663290683490532995 ) ) ;
#8310=CARTESIAN_POINT ( 'NONE',  ( -3.149236820124241110, 6.896136400112061970, -0.7998128361456481317 ) ) ;
#8320=CARTESIAN_POINT ( 'NONE',  ( 0.3548627404530421137, 3.214704059642509826, -1.969391935101212576 ) ) ;
#8339=CARTESIAN_POINT ( 'NONE',  ( 3.119784744920330422, 6.653849612466795627, 0.7216878364870257245 ) ) ;
#8345=CARTESIAN_POINT ( 'NONE',  ( 6.749980374757213575, 8.968339418673846097, 1.599625672291268286 ) ) ;
#8346=CARTESIAN_POINT ( 'NONE',  ( 3.228249973385329596, 6.780392379009261283, -1.734723475976807094E-15 ) ) ;
#8358=CARTESIAN_POINT ( 'NONE',  ( -5.367048706163331850, 7.354919138647580290, -1.599625672291271394 ) ) ;
#8360=CARTESIAN_POINT ( 'NONE',  ( 8.136301581532414673, 8.664975731308866003, 0.000000000000000000 ) ) ;
#8370=CARTESIAN_POINT ( 'NONE',  ( -3.800028193580205382, 7.655393002477360653, -0.7998128361456481317 ) ) ;
#8379=CARTESIAN_POINT ( 'NONE',  ( -3.311934663488232733, 7.085950550703385531, -0.7998128361456481317 ) ) ;
#8400=CARTESIAN_POINT ( 'NONE',  ( -5.498713818794216834, 8.572860667638675380, -1.199719254218452047 ) ) ;
#8402=CARTESIAN_POINT ( 'NONE',  ( -2.979759899953417612, 6.698413326579433225, 0.7998128361456352531 ) ) ;
#8415=ORIENTED_EDGE ( 'NONE', *, *, #18341, .T. ) ;
#8419=CARTESIAN_POINT ( 'NONE',  ( 7.013428937081386927, 5.939655416065874327, 2.436399677959149468 ) ) ;
#8426=CARTESIAN_POINT ( 'NONE',  ( -6.981522756394290319, 7.109807735406931783, 0.7998128361456341429 ) ) ;
#8433=CARTESIAN_POINT ( 'NONE',  ( 6.495764994278795612, 9.632124022417032805, 1.082531754730549078 ) ) ;
#8441=CARTESIAN_POINT ( 'NONE',  ( -5.515163814073178905, 6.606792650666174715, 1.108724247552300701 ) ) ;
#8446=CARTESIAN_POINT ( 'NONE',  ( 4.329849954717849947, 6.144853928627882489, 1.599625672291262513 ) ) ;
#8453=CARTESIAN_POINT ( 'NONE',  ( 6.713222337422018349, 7.861122810861019161, -1.199719254218452047 ) ) ;
#8455=CARTESIAN_POINT ( 'NONE',  ( 6.554440917563797875, 6.611545590104705994, -0.7998128361456481317 ) ) ;
#8469=CARTESIAN_POINT ( 'NONE',  ( 6.474762296362193581, 6.758873339713582062, -0.2294044474360455721 ) ) ;
#8471=CARTESIAN_POINT ( 'NONE',  ( 5.072158865288233898, 7.971250205261355859, 1.082531754730549078 ) ) ;
#8479=CARTESIAN_POINT ( 'NONE',  ( -3.311934663488232733, 7.085950550703385531, -0.7998128361456481317 ) ) ;
#8484=EDGE_CURVE ( 'NONE', #199128, #100096, #140417, .T. ) ;
#8487=VERTEX_POINT ( 'NONE', #210057 ) ;
#8490=CARTESIAN_POINT ( 'NONE',  ( -6.577113915960849155, 6.845923454808663600, -0.7216878364870338292 ) ) ;
#8495=CARTESIAN_POINT ( 'NONE',  ( 5.806634928402749196, 9.996434193103704402, -0.7998128361456481317 ) ) ;
#8496=CARTESIAN_POINT ( 'NONE',  ( -4.570876033279031248, 6.929166027572136954, -1.217404184480129326 ) ) ;
#8513=CARTESIAN_POINT ( 'NONE',  ( 5.773793314573267388, 7.829454515125894964, 1.599625672291268286 ) ) ;
#8532=CARTESIAN_POINT ( 'NONE',  ( -6.882699257592852504, 8.058845884393651460, -1.199719254218452047 ) ) ;
#8554=CARTESIAN_POINT ( 'NONE',  ( 4.909461021924240498, 7.781436054670031410, 1.082531754730549078 ) ) ;
#8564=CARTESIAN_POINT ( 'NONE',  ( -3.797692425603673705, 6.484372692295976570, 1.082531754730549967 ) ) ;
#8594=CARTESIAN_POINT ( 'NONE',  ( 3.040771591214902259, 6.769593633051179005, -0.7998128361456362523 ) ) ;
#8606=CARTESIAN_POINT ( 'NONE',  ( -7.268579750702160780, 8.613002809641560731, -1.082531754730549967 ) ) ;
#8608=CARTESIAN_POINT ( 'NONE',  ( 3.241808126998965811, 6.796210224891872542, 0.7216878364870257245 ) ) ;
#8612=EDGE_CURVE ( 'NONE', #129277, #92086, #212458, .T. ) ;
#8625=CARTESIAN_POINT ( 'NONE',  ( 4.577813143269636065, 5.369812084349879555, -1.199719254218450271 ) ) ;
#8627=CARTESIAN_POINT ( 'NONE',  ( 6.966220764712143243, 6.002124920821316323, -2.420000000000000373 ) ) ;
#8631=PLANE ( 'NONE',  #28342 ) ;
#8644=ORIENTED_EDGE ( 'NONE', *, *, #64428, .T. ) ;
#8660=CARTESIAN_POINT ( 'NONE',  ( -7.469616286486262524, 7.679250187180907794, 0.7998128361456341429 ) ) ;
#8663=CARTESIAN_POINT ( 'NONE',  ( -6.622231685632140596, 6.690634819517756959, 0.000000000000000000 ) ) ;
#8664=CARTESIAN_POINT ( 'NONE',  ( -6.479871072688648148, 6.524547437750345402, 0.000000000000000000 ) ) ;
#8668=CARTESIAN_POINT ( 'NONE',  ( -6.794044373779495771, 8.059378203231773341, 1.082531754730549078 ) ) ;
#8674=CARTESIAN_POINT ( 'NONE',  ( -6.291865805193673111, 9.498204651771386509, -1.199719254218452047 ) ) ;
#8682=CARTESIAN_POINT ( 'NONE',  ( -7.944151662964566540, 8.232874793072271657, 0.000000000000000000 ) ) ;
#8684=CARTESIAN_POINT ( 'NONE',  ( 5.504185490526544378, 7.460110003252303557, -1.249659907641489820 ) ) ;
#8688=CARTESIAN_POINT ( 'NONE',  ( 3.088225128862704949, 6.824956093640315302, 0.7998128361456281477 ) ) ;
#8711=CARTESIAN_POINT ( 'NONE',  ( 5.833751235630055376, 10.02806988486892514, 0.7998128361456331437 ) ) ;
#8725=CARTESIAN_POINT ( 'NONE',  ( 0.1452347671247937455, 3.480000000000001759, 2.000000000000002220 ) ) ;
#8727=ADVANCED_FACE ( 'NONE', ( #169414 ), #209905, .T. ) ;
#8730=CARTESIAN_POINT ( 'NONE',  ( 6.090086331970060662, 7.118959255344424086, 1.132899493623270359 ) ) ;
#8731=CARTESIAN_POINT ( 'NONE',  ( -4.123088111887291518, 7.824370207261548416, 0.000000000000000000 ) ) ;
#8745=ORIENTED_EDGE ( 'NONE', *, *, #133776, .F. ) ;
#8760=CARTESIAN_POINT ( 'NONE',  ( 5.076602173674213070, 4.887400388900169368, 0.000000000000000000 ) ) ;
#8777=CARTESIAN_POINT ( 'NONE',  ( -5.769876891067536206, 8.889217585290882795, 1.199719254218454489 ) ) ;
#8779=ORIENTED_EDGE ( 'NONE', *, *, #18478, .T. ) ;
#8784=EDGE_CURVE ( 'NONE', #69383, #90338, #199976, .T. ) ;
#8794=CARTESIAN_POINT ( 'NONE',  ( 4.573896719763862251, 6.429575154514868274, -1.599625672291273171 ) ) ;
#8806=CARTESIAN_POINT ( 'NONE',  ( 5.448178351099921102, 7.506598249424609293, 1.250114376932524252 ) ) ;
#8827=CARTESIAN_POINT ( 'NONE',  ( -5.276058054373441664, 6.184431147304315424, -1.199719254218453823 ) ) ;
#8829=CARTESIAN_POINT ( 'NONE',  ( 3.725458348705031231, 7.568394850123006279, -1.734723475976807094E-15 ) ) ;
#8832=CARTESIAN_POINT ( 'NONE',  ( -4.762657100150483380, 8.778460060142702304, 0.000000000000000000 ) ) ;
#8834=CARTESIAN_POINT ( 'NONE',  ( 7.472478939787284169, 8.746922180287201698, 1.199719254218452935 ) ) ;
#8838=CARTESIAN_POINT ( 'NONE',  ( -4.979135478818752958, 8.054126424104152804, -1.119915745145182440 ) ) ;
#8846=CARTESIAN_POINT ( 'NONE',  ( -3.784134271545645412, 7.428924060196286483, 0.7216878364870338292 ) ) ;
#8855=CARTESIAN_POINT ( 'NONE',  ( 5.316205630334249754, 7.295602216847000498, -1.443375672974078761 ) ) ;
#8859=CARTESIAN_POINT ( 'NONE',  ( -5.237192476628793614, 9.332084666034067055, 0.7998128361456291469 ) ) ;
#8868=CARTESIAN_POINT ( 'NONE',  ( -4.177320726786328819, 5.966903162707725805, -1.443375672974066548 ) ) ;
#8873=CARTESIAN_POINT ( 'NONE',  ( 3.237364818613055473, 6.998952398349030268, -1.734723475976807094E-15 ) ) ;
#8899=CARTESIAN_POINT ( 'NONE',  ( -6.956742217587851052, 7.288823140040177506, 0.000000000000000000 ) ) ;
#8914=ORIENTED_EDGE ( 'NONE', *, *, #31028, .T. ) ;
#8925=CARTESIAN_POINT ( 'NONE',  ( -3.309598895067336510, 6.875299454304925284, 0.000000000000000000 ) ) ;
#8931=CARTESIAN_POINT ( 'NONE',  ( -3.135678666510573365, 6.880318554229450712, 0.000000000000000000 ) ) ;
#8940=CARTESIAN_POINT ( 'NONE',  ( -3.546339698426324460, 6.295090860542775779, -1.199719254218450271 ) ) ;
#8942=CARTESIAN_POINT ( 'NONE',  ( 6.512538272292041519, 6.827515365185738538, -0.5364851146780359459 ) ) ;
#8946=CARTESIAN_POINT ( 'NONE',  ( 4.472210567661338843, 6.310941310395290493, 1.599625672291261402 ) ) ;
#8953=CARTESIAN_POINT ( 'NONE',  ( -3.546339698426324460, 6.295090860542775779, -1.199719254218450271 ) ) ;
#8959=CARTESIAN_POINT ( 'NONE',  ( -4.122561227007127016, 6.967349310553715647, 1.199719254218452935 ) ) ;
#8965=CARTESIAN_POINT ( 'NONE',  ( 4.706088717274896638, 7.544168365912456764, 1.082531754730548412 ) ) ;
#8967=CARTESIAN_POINT ( 'NONE',  ( -5.790741006368224753, 5.928488393617260321, 0.7216878364870257245 ) ) ;
#8970=CARTESIAN_POINT ( 'NONE',  ( -5.472651281771599763, 6.413789912602166687, 1.199719254218452935 ) ) ;
#8973=CARTESIAN_POINT ( 'NONE',  ( 4.309512724297349884, 6.121127159803966933, 1.599625672291261402 ) ) ;
#8984=CARTESIAN_POINT ( 'NONE',  ( 4.690754089986846509, 8.373302309308519042, 0.6171781843518510113 ) ) ;
#8993=CARTESIAN_POINT ( 'NONE',  ( 7.062871678076271920, 7.204714810702593120, -0.7998128361456341429 ) ) ;
#9003=CARTESIAN_POINT ( 'NONE',  ( 5.148720134264945791, 7.772403765597828418, 1.171659602702241676 ) ) ;
#9010=CARTESIAN_POINT ( 'NONE',  ( 7.205232291019763480, 7.370802192470005565, -0.7998128361456341429 ) ) ;
#9014=CARTESIAN_POINT ( 'NONE',  ( -4.784432227305938312, 8.165582598138012571, -0.7895561949947740299 ) ) ;
#9024=CARTESIAN_POINT ( 'NONE',  ( -7.930593509350902792, 8.217056947189661287, -0.7998128361456362523 ) ) ;
#9029=AXIS2_PLACEMENT_3D ( 'NONE', #126335, #173967, #90573 ) ;
#9038=CARTESIAN_POINT ( 'NONE',  ( 6.851666526859736983, 9.086973262793417661, -1.599625672291269396 ) ) ;
#9047=CARTESIAN_POINT ( 'NONE',  ( 4.095444919779759552, 6.935713618788495793, 1.199719254218451159 ) ) ;
#9050=CARTESIAN_POINT ( 'NONE',  ( 3.390947816749319443, 6.970206529600588397, -1.734723475976807094E-15 ) ) ;
#9065=CARTESIAN_POINT ( 'NONE',  ( -3.772911886352873445, 7.623757310712140800, 0.7998128361456352531 ) ) ;
#9066=CARTESIAN_POINT ( 'NONE',  ( 7.675324359112103423, 8.127168971818530707, 0.7216878364870267237 ) ) ;
#9079=CARTESIAN_POINT ( 'NONE',  ( -5.098748287191073203, 8.106234214101666780, 1.199719254218452935 ) ) ;
#9080=CARTESIAN_POINT ( 'NONE',  ( -5.255720823952942489, 6.160704378480398979, -1.199719254218453823 ) ) ;
#9082=CARTESIAN_POINT ( 'NONE',  ( 7.309254211098767051, 7.700087132469628948, 0.7216878364870267237 ) ) ;
#9084=ORIENTED_EDGE ( 'NONE', *, *, #112034, .F. ) ;
#9088=DIRECTION ( 'NONE',  ( -0.9446243521954068578, 3.252606517456503205E-14, -0.3281536732072456997 ) ) ;
#9093=CARTESIAN_POINT ( 'NONE',  ( -5.764421489320544545, 7.269302474779911982, -1.197982331091128616 ) ) ;
#9098=CARTESIAN_POINT ( 'NONE',  ( 5.072158865288243668, 6.050511776658669127, 1.082531754730549078 ) ) ;
#9102=CARTESIAN_POINT ( 'NONE',  ( -6.444921918449773024, 8.612437886315108315, 1.599625672291269396 ) ) ;
#9116=CARTESIAN_POINT ( 'NONE',  ( 6.052789233858158369, 6.026285292448116948, 0.000000000000000000 ) ) ;
#9133=CARTESIAN_POINT ( 'NONE',  ( 2.970447988400423789, 6.576210002780722874, 0.4422704740705263871 ) ) ;
#9140=DIRECTION ( 'NONE',  ( 1.000000000000000000, 0.000000000000000000, 0.000000000000000000 ) ) ;
#9151=CARTESIAN_POINT ( 'NONE',  ( 6.699137298928145690, 8.909022496873262753, 1.443375672974065660 ) ) ;
#9156=CARTESIAN_POINT ( 'NONE',  ( 7.485510208076452621, 7.905719128943566432, 0.000000000000000000 ) ) ;
#9183=CARTESIAN_POINT ( 'NONE',  ( -5.354544322754380303, 5.211666229493680191, 0.7998128361456281477 ) ) ;
#9185=CARTESIAN_POINT ( 'NONE',  ( 5.682275777458846377, 7.722684055159064975, 1.443375672974064550 ) ) ;
#9191=CARTESIAN_POINT ( 'NONE',  ( -5.666381855868691808, 5.575476684793721383, 0.000000000000000000 ) ) ;
#9196=CARTESIAN_POINT ( 'NONE',  ( -5.093022980588950865, 5.970890227889075419, -1.199719254218453823 ) ) ;
#9203=CARTESIAN_POINT ( 'NONE',  ( -5.469788628470539926, 5.346117919495872783, -0.7998128361456362523 ) ) ;
#9213=CARTESIAN_POINT ( 'NONE',  ( -2.986538976760251263, 6.706322249520737522, -0.7998128361456481317 ) ) ;
#9216=CARTESIAN_POINT ( 'NONE',  ( -4.163762573172648196, 7.871823745427799501, 0.000000000000000000 ) ) ;
#9217=CARTESIAN_POINT ( 'NONE',  ( -5.058600711230246461, 7.955432358860325515, 1.082531754730549967 ) ) ;
#9218=CARTESIAN_POINT ( 'NONE',  ( 5.040599249230596435, 9.102725900736217568, 0.7998128361456341429 ) ) ;
#9219=CARTESIAN_POINT ( 'NONE',  ( -6.954406449166956605, 7.078172043641714595, -0.7998128361456362523 ) ) ;
#9239=CARTESIAN_POINT ( 'NONE',  ( 5.501576472095266901, 9.640532660744973725, -0.7998128361456481317 ) ) ;
#9247=CIRCLE ( 'NONE', #151046, 0.08000000000000041800 ) ;
#9264=DIRECTION ( 'NONE',  ( -1.000000000000000000, -2.168404344971003504E-14, 0.000000000000000000 ) ) ;
#9267=CARTESIAN_POINT ( 'NONE',  ( 5.076871660599175051, 4.912164349150736520, 0.2100609765546117280 ) ) ;
#9272=AXIS2_PLACEMENT_3D ( 'NONE', #124069, #91501, #54704 ) ;
#9276=ADVANCED_FACE ( 'NONE', ( #31587 ), #175178, .T. ) ;
#9277=CARTESIAN_POINT ( 'NONE',  ( 5.794130544993763898, 7.853181283949808744, 1.599625672291269396 ) ) ;
#9280=CARTESIAN_POINT ( 'NONE',  ( -3.923105346307911745, 5.670318552149568703, -1.599625672291283607 ) ) ;
#9283=CARTESIAN_POINT ( 'NONE',  ( -4.787437638956920871, 8.599444655509458357, -0.7216878364870338292 ) ) ;
#9294=CARTESIAN_POINT ( 'NONE',  ( 5.246079093845007257, 5.085123462432798114, 0.7998128361456352531 ) ) ;
#9295=CARTESIAN_POINT ( 'NONE',  ( 4.518610335104485287, 8.493738834255713854, 0.000000000000000000 ) ) ;
#9301=CARTESIAN_POINT ( 'NONE',  ( 4.004454267989866700, 5.765225627445230927, 1.599625672291262513 ) ) ;
#9307=CARTESIAN_POINT ( 'NONE',  ( 5.357406976055401948, 6.279338222599979424, 1.199719254218452935 ) ) ;
#9317=VERTEX_POINT ( 'NONE', #118900 ) ;
#9319=CARTESIAN_POINT ( 'NONE',  ( 6.373741612200160667, 9.489763409991955001, 1.082531754730549078 ) ) ;
#9320=CARTESIAN_POINT ( 'NONE',  ( -4.014622883422336308, 5.777089012116397804, -1.443375672974066548 ) ) ;
#9321=CARTESIAN_POINT ( 'NONE',  ( -5.803772275101700906, 8.928762199997411386, -1.199719254218452047 ) ) ;
#9334=CARTESIAN_POINT ( 'NONE',  ( 4.505052181490820651, 8.477920988373101707, -0.7998128361456381397 ) ) ;
#9335=CARTESIAN_POINT ( 'NONE',  ( 5.525830126021535449, 8.604496359403894346, -1.199719254218452047 ) ) ;
#9338=CARTESIAN_POINT ( 'NONE',  ( 3.065552130021340194, 6.590578228417936835, 0.000000000000000000 ) ) ;
#9355=CARTESIAN_POINT ( 'NONE',  ( 4.817943484809818600, 6.714296380401858499, 1.599625672291269396 ) ) ;
#9361=CARTESIAN_POINT ( 'NONE',  ( 6.073126464278658432, 6.050012061272033392, 0.000000000000000000 ) ) ;
#9366=CARTESIAN_POINT ( 'NONE',  ( 7.180978637093494044, 8.406838493811077839, -1.199719254218452047 ) ) ;
#9371=CARTESIAN_POINT ( 'NONE',  ( 5.045042558060919724, 8.899983727797476263, -0.7216878364870458196 ) ) ;
#9373=CARTESIAN_POINT ( 'NONE',  ( -6.656127069666307072, 6.730179434224282886, 0.7998128361456341429 ) ) ;
#9374=CARTESIAN_POINT ( 'NONE',  ( 3.867818961648523235, 7.734482231890414283, 1.040834085586084257E-14 ) ) ;
#9381=CARTESIAN_POINT ( 'NONE',  ( -5.807383341681398470, 6.267539566907733395, -0.6908299548700506110 ) ) ;
#9384=CARTESIAN_POINT ( 'NONE',  ( -3.962726036944197894, 7.845207153068690431, -0.7998128361456481317 ) ) ;
#9399=( BOUNDED_CURVE ( )  B_SPLINE_CURVE ( 2, ( #114988, #98683, #151706, #164739, #69342, #50995, #198285 ),
 .UNSPECIFIED., .F., .T. ) 
 B_SPLINE_CURVE_WITH_KNOTS ( ( 3, 2, 2, 3 ),
 ( 0.3750000000000000000, 0.3833333333333335258, 0.3916666666666670515, 0.4000000000000005773 ),
 .UNSPECIFIED. ) 
 CURVE ( )  GEOMETRIC_REPRESENTATION_ITEM ( )  RATIONAL_B_SPLINE_CURVE ( ( 1.000000000000000000, 0.8660254037844387076, 1.000000000000000000, 0.8660254037844387076, 1.000000000000000000, 0.8660254037844298258, 1.000000000000008882 ) ) 
 REPRESENTATION_ITEM ( '' )  );
#9419=CARTESIAN_POINT ( 'NONE',  ( 8.005163354226054295, 8.304055099544019214, 0.000000000000000000 ) ) ;
#9420=CARTESIAN_POINT ( 'NONE',  ( 5.989670002187236442, 10.20997511251894529, -0.7998128361456481317 ) ) ;
#9433=CARTESIAN_POINT ( 'NONE',  ( -6.448838341955544173, 7.552674816150118708, 1.199719254218452047 ) ) ;
#9435=CARTESIAN_POINT ( 'NONE',  ( 6.007671464186812749, 10.02305078494439883, 0.7216878364870317197 ) ) ;
#9443=CARTESIAN_POINT ( 'NONE',  ( -6.310394152517827315, 6.326824364217716656, 0.7998128361456281477 ) ) ;
#9450=CARTESIAN_POINT ( 'NONE',  ( -3.851925040058345573, 5.587274861525073355, -1.443375672974078761 ) ) ;
#9454=CARTESIAN_POINT ( 'NONE',  ( -3.786470039966538970, 7.639575156594750283, 0.000000000000000000 ) ) ;
#9477=CARTESIAN_POINT ( 'NONE',  ( -6.363572996767778100, 8.517530811019446091, -1.599625672291271394 ) ) ;
#9479=CARTESIAN_POINT ( 'NONE',  ( -4.736594563127865420, 6.619389305106191834, -1.599625672291271394 ) ) ;
#9488=CARTESIAN_POINT ( 'NONE',  ( -6.285146472706256482, 6.979120928820362835, -0.9578508296879204575 ) ) ;
#9501=DIRECTION ( 'NONE',  ( 0.000000000000000000, 0.000000000000000000, -1.000000000000000000 ) ) ;
#9506=CARTESIAN_POINT ( 'NONE',  ( -5.794130544993808307, 7.853181283949808744, 1.599625672291263179 ) ) ;
#9532=CARTESIAN_POINT ( 'NONE',  ( 5.987861119090863049, 7.014868056141362551, 1.199719254218452047 ) ) ;
#9535=CARTESIAN_POINT ( 'NONE',  ( -2.265491011392835929, 2.737016401661231502, -2.500000000000000444 ) ) ;
#9542=B_SPLINE_CURVE_WITH_KNOTS ( 'NONE', 3,
 ( #97006, #175048, #144706, #145774, #208567, #176109, #11446, #178242, #179309, #194473 ),
 .UNSPECIFIED., .F., .F.,
 ( 4, 3, 3, 4 ),
 ( 0.000000000000000000, 4.379906072315623141E-05, 0.0001100530589225749337, 0.0001772280998810008272 ),
 .UNSPECIFIED. ) ;
#9545=CARTESIAN_POINT ( 'NONE',  ( 5.997574213172828905, 7.082153300894140635, -1.064076030282636420 ) ) ;
#9547=CARTESIAN_POINT ( 'NONE',  ( 5.397554552016204710, 9.311247720745345902, 0.7216878364870317197 ) ) ;
#9555=CARTESIAN_POINT ( 'NONE',  ( -4.176793841461789114, 7.030620694084159794, -1.199719254218455378 ) ) ;
#9563=CARTESIAN_POINT ( 'NONE',  ( -6.766928066552171828, 7.067373297165212342, 0.7216878364870317197 ) ) ;
#9572=CARTESIAN_POINT ( 'NONE',  ( -3.363304624641834106, 6.081549941127532222, -1.199719254218452047 ) ) ;
#9579=CARTESIAN_POINT ( 'NONE',  ( -6.069210040772897052, 7.109775131437022999, -1.199719254218453823 ) ) ;
#9582=CARTESIAN_POINT ( 'NONE',  ( 8.154303043976348420, 8.478051404252736845, 0.7998128361456281477 ) ) ;
#9595=FACE_OUTER_BOUND ( 'NONE', #5456, .T. ) ;
#9599=CARTESIAN_POINT ( 'NONE',  ( -5.427006627220116286, 9.553534508390610469, -0.7998128361456362523 ) ) ;
#9602=CARTESIAN_POINT ( 'NONE',  ( 7.354371980770088690, 7.544798497178720531, 0.000000000000000000 ) ) ;
#9620=CARTESIAN_POINT ( 'NONE',  ( 5.343321937561575474, 8.287607122913563273, -1.082531754730548412 ) ) ;
#9626=CARTESIAN_POINT ( 'NONE',  ( 8.174640274396848483, 8.501778173076651512, 0.7998128361456291469 ) ) ;
#9630=CARTESIAN_POINT ( 'NONE',  ( -4.340018570150306232, 8.077455741901736985, -0.7216878364870338292 ) ) ;
#9659=VERTEX_POINT ( 'NONE', #188094 ) ;
#9663=CARTESIAN_POINT ( 'NONE',  ( 4.472210567661338843, 6.310941310395290493, 1.599625672291261402 ) ) ;
#9674=CARTESIAN_POINT ( 'NONE',  ( -5.478903473698241378, 9.406154796041011679, -0.7216878364870338292 ) ) ;
#9677=CARTESIAN_POINT ( 'NONE',  ( 3.228249973385329596, 6.780392379009261283, -1.734723475976807094E-15 ) ) ;
#9695=CARTESIAN_POINT ( 'NONE',  ( -4.828112100242294424, 5.765790550771681566, -1.082531754730549967 ) ) ;
#9727=CARTESIAN_POINT ( 'NONE',  ( -6.583366107887490770, 9.838288338247510367, 1.199719254218452935 ) ) ;
#9730=CARTESIAN_POINT ( 'NONE',  ( -5.641074431737709283, 8.738948049406083385, -1.199719254218452047 ) ) ;
#9735=CARTESIAN_POINT ( 'NONE',  ( -7.729556973122450714, 8.190440354830551328, 0.000000000000000000 ) ) ;
#9736=CARTESIAN_POINT ( 'NONE',  ( 7.634649897826744080, 9.040084647953621655, 1.082531754730549078 ) ) ;
#9743=CARTESIAN_POINT ( 'NONE',  ( -5.029148636026397945, 4.832037928311032182, 0.7998128361456281477 ) ) ;
#9752=CARTESIAN_POINT ( 'NONE',  ( 5.726091835933811325, 7.283405380927965744, -1.209259067671350163 ) ) ;
#9757=CARTESIAN_POINT ( 'NONE',  ( 6.235824307642648279, 6.239826211863360506, 0.000000000000000000 ) ) ;
#9781=CARTESIAN_POINT ( 'NONE',  ( 3.923105346307896202, 5.670318552149568703, -1.599625672291269396 ) ) ;
#9794=CARTESIAN_POINT ( 'NONE',  ( 6.472394699177205446, 6.854181287346997387, 0.6349317888264572884 ) ) ;
#9795=CARTESIAN_POINT ( 'NONE',  ( -3.919715807682309094, 6.626733304721049933, 1.082531754730549967 ) ) ;
#9818=CIRCLE ( 'NONE', #44481, 0.7500000000000011102 ) ;
#9819=CIRCLE ( 'NONE', #151612, 3.100000000000000089 ) ;
#9824=CARTESIAN_POINT ( 'NONE',  ( 4.415115299905642665, 5.179997933758551554, -1.199719254218450271 ) ) ;
#9844=CARTESIAN_POINT ( 'NONE',  ( -5.119085517611572378, 8.129960982925583224, 1.199719254218452935 ) ) ;
#9856=ORIENTED_EDGE ( 'NONE', *, *, #139194, .T. ) ;
#9858=CARTESIAN_POINT ( 'NONE',  ( 4.278479993564246797, 7.149254538203735798, 1.199719254218452047 ) ) ;
#9867=CARTESIAN_POINT ( 'NONE',  ( 4.728828643816226140, 8.210394131765152537, 0.6915292512235807765 ) ) ;
#9868=CARTESIAN_POINT ( 'NONE',  ( -0.4205927090898516907, 3.223357252100233605, 1.955451565440526007 ) ) ;
#9869=CARTESIAN_POINT ( 'NONE',  ( 4.816695983655697511, 8.110494931179941247, 0.8576603160085185529 ) ) ;
#9870=CARTESIAN_POINT ( 'NONE',  ( 4.876338901402099246, 8.164033411617232616, 0.9883146796138141399 ) ) ;
#9871=CARTESIAN_POINT ( 'NONE',  ( -3.650099463454746118, 7.352759259900637723, 0.1599090995409638560 ) ) ;
#9889=CARTESIAN_POINT ( 'NONE',  ( -5.173318132066234476, 8.193232366456022930, -1.199719254218453823 ) ) ;
#9891=CARTESIAN_POINT ( 'NONE',  ( 6.073126464278658432, 6.050012061272033392, 0.000000000000000000 ) ) ;
#9895=CARTESIAN_POINT ( 'NONE',  ( -5.773793314573309132, 7.829454515125894964, 1.599625672291263179 ) ) ;
#9899=DIRECTION ( 'NONE',  ( -0.9446243521954068578, 0.000000000000000000, 0.3281536732072456997 ) ) ;
#9904=CARTESIAN_POINT ( 'NONE',  ( -4.684263184503158151, 8.377143357790286515, -0.6327197186303500365 ) ) ;
#9905=CARTESIAN_POINT ( 'NONE',  ( 0.000000000000000000, 8.920000000000001705, 0.000000000000000000 ) ) ;
#9909=AXIS2_PLACEMENT_3D ( 'NONE', #174462, #92151, #26038 ) ;
#9923=CARTESIAN_POINT ( 'NONE',  ( 6.387299765813869712, 6.624473612970537495, 0.000000000000000000 ) ) ;
#9927=CARTESIAN_POINT ( 'NONE',  ( -6.505933609711270549, 8.683618192786854095, -1.599625672291271394 ) ) ;
#9941=CARTESIAN_POINT ( 'NONE',  ( 5.411639590510088027, 6.342609606130419131, -1.199719254218452047 ) ) ;
#9989=CARTESIAN_POINT ( 'NONE',  ( -3.160459205317013076, 6.701303149596211206, -0.7216878364870458196 ) ) ;
#9996=CARTESIAN_POINT ( 'NONE',  ( -3.797165540279144214, 6.587721009371067638, 1.199719254218452935 ) ) ;
#10005=CARTESIAN_POINT ( 'NONE',  ( -4.197131071882288289, 7.054347462908075350, -1.199719254218455378 ) ) ;
#10007=CARTESIAN_POINT ( 'NONE',  ( 5.413027408713817046, 7.651055653456078076, -1.328921179265474262 ) ) ;
#10011=CARTESIAN_POINT ( 'NONE',  ( 5.011674058906918638, 5.875983152593414971, 1.199719254218452047 ) ) ;
#10018=CARTESIAN_POINT ( 'NONE',  ( -5.191846479390389568, 5.021852078902356631, 0.7998128361456281477 ) ) ;
#10021=CARTESIAN_POINT ( 'NONE',  ( -4.447956913735107598, 7.346977611736363656, 1.199719254218452935 ) ) ;
#10026=CARTESIAN_POINT ( 'NONE',  ( 4.190878879955609371, 7.903459436674603822, -0.7216878364870338292 ) ) ;
#10027=CARTESIAN_POINT ( 'NONE',  ( -7.065207446052822249, 7.415365906582643163, -0.7216878364870338292 ) ) ;
#10036=CARTESIAN_POINT ( 'NONE',  ( 3.902768115887398803, 5.646591783325653147, -1.599625672291269396 ) ) ;
#10044=PRESENTATION_STYLE_ASSIGNMENT (( #76118 ) ) ;
#10047=CIRCLE ( 'NONE', #37733, 0.8299999999999999600 ) ;
#10056=CARTESIAN_POINT ( 'NONE',  ( -2.810282979782591006, 6.500690253046801814, 0.000000000000000000 ) ) ;
#10065=CARTESIAN_POINT ( 'NONE',  ( 4.611577566919329740, 8.352668595566711929, -0.2595669225248058432 ) ) ;
#10072=CARTESIAN_POINT ( 'NONE',  ( 6.530187263637528439, 7.647581891445782709, -1.199719254218452047 ) ) ;
#10077=CARTESIAN_POINT ( 'NONE',  ( -4.603881723180708541, 8.384271979250147666, 0.04571010684512218092 ) ) ;
#10085=CARTESIAN_POINT ( 'NONE',  ( -7.282664789195997912, 8.525472337930658284, 1.199719254218452047 ) ) ;
#10097=CARTESIAN_POINT ( 'NONE',  ( 7.225569521440261767, 7.394528961293920233, -0.7998128361456341429 ) ) ;
#10101=CARTESIAN_POINT ( 'NONE',  ( -5.608478439449225306, 5.609308656285654671, -0.4224404339892348093 ) ) ;
#10107=CARTESIAN_POINT ( 'NONE',  ( 5.174371902270911150, 6.065797303184739420, 1.199719254218452047 ) ) ;
#10110=CARTESIAN_POINT ( 'NONE',  ( 4.678972410047582464, 8.472901888448573615, -0.7216878364870357165 ) ) ;
#10122=CARTESIAN_POINT ( 'NONE',  ( -4.390861645979385663, 6.216034235099629157, -1.599625672291271394 ) ) ;
#10123=CARTESIAN_POINT ( 'NONE',  ( 6.861835142292135536, 9.098836647464588978, 1.443375672974065660 ) ) ;
#10135=CARTESIAN_POINT ( 'NONE',  ( -5.261446130555064826, 8.296048364692991228, 1.199719254218452935 ) ) ;
#10136=CARTESIAN_POINT ( 'NONE',  ( -5.147255595043616516, 6.034161611419515125, 1.199719254218452935 ) ) ;
#10138=CARTESIAN_POINT ( 'NONE',  ( 7.038091138825468107, 8.344099429118761790, -1.082531754730548412 ) ) ;
#10149=CARTESIAN_POINT ( 'NONE',  ( -5.779986827147332029, 7.257483166437310729, -1.191988747605486010 ) ) ;
#10151=CARTESIAN_POINT ( 'NONE',  ( -5.764827401431626974, 7.068052664419927744, -2.440105445505980075 ) ) ;
#10156=CARTESIAN_POINT ( 'NONE',  ( 4.095971805104276164, 7.792734516014745871, 0.7216878364870257245 ) ) ;
#10161=CARTESIAN_POINT ( 'NONE',  ( -6.957269102468015554, 8.145844036748005834, 1.199719254218452047 ) ) ;
#10177=CARTESIAN_POINT ( 'NONE',  ( 4.505052181490820651, 8.477920988373101707, -0.7998128361456381397 ) ) ;
#10193=CARTESIAN_POINT ( 'NONE',  ( 2.971087601478215934, 6.563059292275168488, 0.4682405089187134384 ) ) ;
#10212=CARTESIAN_POINT ( 'NONE',  ( 6.048345925472178308, 9.110135108809304327, 1.082531754730549967 ) ) ;
#10218=CARTESIAN_POINT ( 'NONE',  ( 5.329763783503544516, 9.232158490813878515, -0.7216878364870458196 ) ) ;
#10242=CARTESIAN_POINT ( 'NONE',  ( -4.359828915246279024, 7.244161613499399799, -1.199719254218455378 ) ) ;
#10244=CARTESIAN_POINT ( 'NONE',  ( 4.950135482320912494, 6.868520377498098739, -1.443375672974068769 ) ) ;
#10249=CARTESIAN_POINT ( 'NONE',  ( -4.197131071882288289, 7.054347462908075350, -1.199719254218455378 ) ) ;
#10253=EDGE_CURVE ( 'NONE', #34262, #758, #122624, .T. ) ;
#10255=ORIENTED_EDGE ( 'NONE', *, *, #183912, .F. ) ;
#10256=CARTESIAN_POINT ( 'NONE',  ( -5.483346782084204563, 5.361935765378481378, 0.000000000000000000 ) ) ;
#10262=CARTESIAN_POINT ( 'NONE',  ( -4.098307573080856692, 8.003385611894792362, 0.7998128361456352531 ) ) ;
#10270=CARTESIAN_POINT ( 'NONE',  ( -3.149236820124241110, 6.896136400112061970, -0.7998128361456481317 ) ) ;
#10273=CARTESIAN_POINT ( 'NONE',  ( -6.048345925472225382, 8.149765894507963182, 1.443375672974058777 ) ) ;
#10275=CARTESIAN_POINT ( 'NONE',  ( -5.600926855776888758, 7.627776979863398310, -1.443375672974066548 ) ) ;
#10276=CARTESIAN_POINT ( 'NONE',  ( 4.715203562502613188, 8.723097599553565118, 0.7998128361456341429 ) ) ;
#10277=CARTESIAN_POINT ( 'NONE',  ( -4.847922445338252118, 7.813604065273374921, -1.199719254218453823 ) ) ;
#10296=CARTESIAN_POINT ( 'NONE',  ( 5.338878628731272613, 9.450718510153643948, -0.7998128361456481317 ) ) ;
#10314=CIRCLE ( 'NONE', #107335, 0.08000000000000020983 ) ;
#10316=CARTESIAN_POINT ( 'NONE',  ( 4.609415035364720303, 8.472105597856021575, 0.2450749143364742144 ) ) ;
#10328=CARTESIAN_POINT ( 'NONE',  ( 5.956828388357757298, 8.042995434541133193, 1.599625672291269396 ) ) ;
#10334=CARTESIAN_POINT ( 'NONE',  ( -5.600926855776877211, 9.548515408466085930, -0.7216878364870338292 ) ) ;
#10345=CARTESIAN_POINT ( 'NONE',  ( 4.947799714344386146, 4.737130853015369958, -0.7998128361456481317 ) ) ;
#10346=CARTESIAN_POINT ( 'NONE',  ( 6.150558962454855561, 7.204682206732687000, 1.199719254218452047 ) ) ;
#10355=CARTESIAN_POINT ( 'NONE',  ( 2.911969131885072670, 6.619324097166378706, 0.000000000000000000 ) ) ;
#10361=CARTESIAN_POINT ( 'NONE',  ( 5.200434439293556643, 8.224868058221247225, -1.199719254218452047 ) ) ;
#10372=CARTESIAN_POINT ( 'NONE',  ( 6.617788377246179188, 8.814115421577600529, -1.443375672974078761 ) ) ;
#10373=CARTESIAN_POINT ( 'NONE',  ( -6.143253000767895600, 6.339752387083549934, 0.000000000000000000 ) ) ;
#10374=CARTESIAN_POINT ( 'NONE',  ( -7.425025402139490360, 8.691559719698066289, 1.199719254218452047 ) ) ;
#10386=ORIENTED_EDGE ( 'NONE', *, *, #83202, .T. ) ;
#10387=CARTESIAN_POINT ( 'NONE',  ( 4.908934136599710563, 7.884784371745123366, 1.199719254218451159 ) ) ;
#10388=CARTESIAN_POINT ( 'NONE',  ( 5.742760583840166966, 8.857581893525663830, 1.199719254218452047 ) ) ;
#10391=CARTESIAN_POINT ( 'NONE',  ( 3.729901657090948230, 6.405283462364505631, 1.082531754730549078 ) ) ;
#10408=EDGE_CURVE ( 'NONE', #191915, #200036, #10885, .T. ) ;
#10411=CARTESIAN_POINT ( 'NONE',  ( 5.246079093845007257, 5.085123462432798114, 0.7998128361456352531 ) ) ;
#10413=ADVANCED_FACE ( 'NONE', ( #111677 ), #79098, .F. ) ;
#10415=CARTESIAN_POINT ( 'NONE',  ( 4.386945222473598527, 7.275797305264619652, -1.199719254218452047 ) ) ;
#10421=DIRECTION ( 'NONE',  ( 0.000000000000000000, 0.000000000000000000, 1.000000000000000000 ) ) ;
#10425=CARTESIAN_POINT ( 'NONE',  ( 5.695833931516881776, 9.659240330162777610, -0.7216878364870458196 ) ) ;
#10428=CARTESIAN_POINT ( 'NONE',  ( -5.281783360975562225, 8.319775133516907673, 1.199719254218452935 ) ) ;
#10429=CARTESIAN_POINT ( 'NONE',  ( 5.123001941117305336, 7.070197912760590064, 1.599625672291268286 ) ) ;
#10439=CARTESIAN_POINT ( 'NONE',  ( -4.176793841461789114, 7.030620694084159794, -1.199719254218455378 ) ) ;
#10467=ORIENTED_EDGE ( 'NONE', *, *, #129354, .T. ) ;
#10472=CARTESIAN_POINT ( 'NONE',  ( 4.923019175093585886, 5.876515471431535076, -1.082531754730548412 ) ) ;
#10484=CARTESIAN_POINT ( 'NONE',  ( -5.991777542596674166, 5.955104985976372944, 0.000000000000000000 ) ) ;
#10486=CARTESIAN_POINT ( 'NONE',  ( -4.450819567036169211, 8.414649604842665553, -0.7998128361456362523 ) ) ;
#10489=CARTESIAN_POINT ( 'NONE',  ( 6.116136693096175136, 9.189224337703940648, -1.082531754730548412 ) ) ;
#10499=CARTESIAN_POINT ( 'NONE',  ( -5.936491157937300756, 8.019268665717216749, 1.599625672291263179 ) ) ;
#10504=CYLINDRICAL_SURFACE ( 'NONE', #199519, 1.250000000000000000 ) ;
#10506=CARTESIAN_POINT ( 'NONE',  ( -4.611181642423629157, 7.433443445252599702, 1.082531754730549967 ) ) ;
#10510=CARTESIAN_POINT ( 'NONE',  ( -4.797606254389363833, 6.690569611577942943, 1.599625672291263179 ) ) ;
#10519=AXIS2_PLACEMENT_3D ( 'NONE', #166262, #133803, #81817 ) ;
#10531=CARTESIAN_POINT ( 'NONE',  ( -5.932574734431526942, 9.079031735882207244, 1.199719254218454489 ) ) ;
#10533=CARTESIAN_POINT ( 'NONE',  ( -5.601453741101424022, 6.564059448486966986, -1.199719254218453823 ) ) ;
#10559=CARTESIAN_POINT ( 'NONE',  ( -4.281342646865346602, 8.216926531310035031, 0.7998128361456352531 ) ) ;
#10567=CARTESIAN_POINT ( 'NONE',  ( 3.947104627881618200, 8.980740528188865923, 0.7749999999999996891 ) ) ;
#10571=EDGE_CURVE ( 'NONE', #26620, #83476, #10314, .T. ) ;
#10584=CARTESIAN_POINT ( 'NONE',  ( 7.635176783151273128, 8.936736330878529699, 1.199719254218452935 ) ) ;
#10586=CARTESIAN_POINT ( 'NONE',  ( 8.154303043976348420, 8.478051404252736845, 0.7998128361456281477 ) ) ;
#10594=CARTESIAN_POINT ( 'NONE',  ( 6.142902043169038429, 7.013529245237516641, 0.9864344219776898237 ) ) ;
#10598=CARTESIAN_POINT ( 'NONE',  ( 5.654245663017247736, 7.339362581565530341, 1.229167601055790815 ) ) ;
#10600=CARTESIAN_POINT ( 'NONE',  ( 5.058600711674583472, 8.915801573680086634, 0.000000000000000000 ) ) ;
#10607=CARTESIAN_POINT ( 'NONE',  ( -4.716257332707368910, 6.595662536282280719, -1.599625672291271394 ) ) ;
#10615=CARTESIAN_POINT ( 'NONE',  ( -7.241463443030476732, 7.620997903056574430, 0.000000000000000000 ) ) ;
#10618=CARTESIAN_POINT ( 'NONE',  ( 7.517069824134078537, 7.734612647770044092, 0.000000000000000000 ) ) ;
#10619=CARTESIAN_POINT ( 'NONE',  ( -5.317849202849146195, 6.330384893147431136, -1.092305163593216388 ) ) ;
#10623=CARTESIAN_POINT ( 'NONE',  ( -5.307090785106547415, 5.156303768904543894, -0.7998128361456362523 ) ) ;
#10632=CARTESIAN_POINT ( 'NONE',  ( 2.898410978271408922, 6.603506251283770112, -0.7998128361456362523 ) ) ;
#10653=CARTESIAN_POINT ( 'NONE',  ( -7.584860592202423035, 7.813701877183096833, -0.7998128361456362523 ) ) ;
#10656=CARTESIAN_POINT ( 'NONE',  ( 7.015418140428412386, 7.149352350113456822, 0.7998128361456331437 ) ) ;
#10671=CARTESIAN_POINT ( 'NONE',  ( 3.851925040058331806, 5.587274861525073355, -1.443375672974066548 ) ) ;
#10673=ADVANCED_FACE ( 'NONE', ( #148380 ), #99618, .T. ) ;
#10676=CARTESIAN_POINT ( 'NONE',  ( 6.048345925472191631, 7.189396680206621149, 1.082531754730549967 ) ) ;
#10683=CARTESIAN_POINT ( 'NONE',  ( 7.635176783151273128, 8.936736330878529699, 1.199719254218452935 ) ) ;
#10687=CARTESIAN_POINT ( 'NONE',  ( -6.183927461608886844, 7.347575139032721303, 1.082531754730548412 ) ) ;
#10691=VERTEX_POINT ( 'NONE', #198165 ) ;
#10692=CARTESIAN_POINT ( 'NONE',  ( 2.973470450930305820, 6.532579092154530365, -0.5245438083391358308 ) ) ;
#10712=DIRECTION ( 'NONE',  ( 0.000000000000000000, 1.000000000000000000, 0.000000000000000000 ) ) ;
#10718=ORIENTED_EDGE ( 'NONE', *, *, #203693, .T. ) ;
#10722=CARTESIAN_POINT ( 'NONE',  ( 4.577813143269636065, 5.369812084349879555, -1.199719254218450271 ) ) ;
#10733=CARTESIAN_POINT ( 'NONE',  ( -6.048345925472225382, 8.149765894507963182, 1.443375672974058777 ) ) ;
#10736=CARTESIAN_POINT ( 'NONE',  ( 3.553645660113312399, 7.160020680191912845, -1.734723475976807094E-15 ) ) ;
#10757=CARTESIAN_POINT ( 'NONE',  ( 3.544905708052195514, 7.357750102694700978, 0.1464419079581855410 ) ) ;
#10782=CARTESIAN_POINT ( 'NONE',  ( -8.120407659942227241, 8.438506789546210030, 0.7998128361456341429 ) ) ;
#10785=CARTESIAN_POINT ( 'NONE',  ( -6.611536185319534908, 7.742488966741438716, 1.199719254218452047 ) ) ;
#10786=CARTESIAN_POINT ( 'NONE',  ( -5.025714415505916577, 8.007183762769660262, 1.161964715574652196 ) ) ;
#10787=CARTESIAN_POINT ( 'NONE',  ( -5.037045483985590266, 7.982112132234349566, -1.219308355916954412 ) ) ;
#10798=CARTESIAN_POINT ( 'NONE',  ( -5.991777542596674166, 5.955104985976372944, 0.000000000000000000 ) ) ;
#10811=CARTESIAN_POINT ( 'NONE',  ( 4.115782150200256950, 6.959440387612411349, 1.199719254218452047 ) ) ;
#10814=ORIENTED_EDGE ( 'NONE', *, *, #43321, .F. ) ;
#10832=CARTESIAN_POINT ( 'NONE',  ( 4.518610335104485287, 8.493738834255713854, 0.000000000000000000 ) ) ;
#10833=CARTESIAN_POINT ( 'NONE',  ( 4.386945222473598527, 7.275797305264619652, -1.199719254218452047 ) ) ;
#10847=CARTESIAN_POINT ( 'NONE',  ( 5.602183562003149042, 7.492195738860313092, 1.335281325244306982 ) ) ;
#10848=CARTESIAN_POINT ( 'NONE',  ( -4.462041952228954500, 6.299077925724123617, -1.443375672974066548 ) ) ;
#10849=CARTESIAN_POINT ( 'NONE',  ( 3.106226591306694651, 6.638031766584184368, 0.000000000000000000 ) ) ;
#10872=EDGE_LOOP ( 'NONE', ( #73651, #77938 ) ) ;
#10877=CARTESIAN_POINT ( 'NONE',  ( 5.713835393516482952, 5.630839145382857680, 0.7998128361456352531 ) ) ;
#10885=LINE ( 'NONE', #75908, #107172 ) ;
#10896=CARTESIAN_POINT ( 'NONE',  ( -7.605197822622922210, 7.837428646007010613, -0.7998128361456362523 ) ) ;
#10904=ORIENTED_EDGE ( 'NONE', *, *, #205115, .F. ) ;
#10909=ORIENTED_EDGE ( 'NONE', *, *, #46958, .F. ) ;
#10912=CARTESIAN_POINT ( 'NONE',  ( 4.050854035433010480, 7.948023151305657841, 0.000000000000000000 ) ) ;
#10921=CARTESIAN_POINT ( 'NONE',  ( -6.089020385868876062, 6.276481003034692030, -0.7216878364870337181 ) ) ;
#10923=CARTESIAN_POINT ( 'NONE',  ( 5.148720134264945791, 7.772403765597828418, 1.171659602702241676 ) ) ;
#10924=CARTESIAN_POINT ( 'NONE',  ( 5.707977696796493916, 7.405608897698303217, 1.328948192410238649 ) ) ;
#10943=CARTESIAN_POINT ( 'NONE',  ( -5.387385936583832802, 7.378645907471495846, -1.599625672291271394 ) ) ;
#10945=CARTESIAN_POINT ( 'NONE',  ( 3.790386463472274148, 6.579812086429759788, 1.199719254218452047 ) ) ;
#10949=CARTESIAN_POINT ( 'NONE',  ( -7.045397100956844127, 8.248660034984974132, -1.199719254218452047 ) ) ;
#10953=CARTESIAN_POINT ( 'NONE',  ( 7.849244587668864348, 8.122149871893999062, 0.7998128361456291469 ) ) ;
#10958=CARTESIAN_POINT ( 'NONE',  ( -5.897079639132071449, 7.258985838325384243, -1.264812401031592204 ) ) ;
#10977=CARTESIAN_POINT ( 'NONE',  ( 5.939880696562888751, 7.062853913145737295, -1.082531754730548412 ) ) ;
#10980=CARTESIAN_POINT ( 'NONE',  ( -6.912678218121246942, 9.158153569265168770, 1.599625672291269396 ) ) ;
#10995=CARTESIAN_POINT ( 'NONE',  ( 3.898851692381625877, 6.706354853490643642, -1.199719254218452047 ) ) ;
#11021=LINE ( 'NONE', #175688, #104367 ) ;
#11045=CARTESIAN_POINT ( 'NONE',  ( -4.950135482320939140, 4.947781948895412008, -0.7216878364870338292 ) ) ;
#11046=EDGE_CURVE ( 'NONE', #93819, #29771, #166021, .T. ) ;
#11052=CARTESIAN_POINT ( 'NONE',  ( -5.285699784481336927, 7.260012063351913625, 1.599625672291263179 ) ) ;
#11058=ORIENTED_EDGE ( 'NONE', *, *, #149314, .F. ) ;
#11063=CARTESIAN_POINT ( 'NONE',  ( -5.764151584465413869, 6.753873599078290546, -1.199719254218453823 ) ) ;
#11065=CARTESIAN_POINT ( 'NONE',  ( 6.083581728852979431, 7.123651168416324175, -1.137916992902558100 ) ) ;
#11070=CARTESIAN_POINT ( 'NONE',  ( 5.855142236255289845, 7.924361590421551860, -1.599625672291281386 ) ) ;
#11076=CARTESIAN_POINT ( 'NONE',  ( -2.993318053567081360, 6.714231172462041819, 0.000000000000000000 ) ) ;
#11083=CARTESIAN_POINT ( 'NONE',  ( -4.960304097753355457, 6.880383762169266504, 1.599625672291263179 ) ) ;
#11086=CARTESIAN_POINT ( 'NONE',  ( 5.682275777458846377, 7.722684055159064975, 1.443375672974064550 ) ) ;
#11087=CARTESIAN_POINT ( 'NONE',  ( -6.251718229232857915, 7.426664367927358512, -1.082531754730549967 ) ) ;
#11091=CARTESIAN_POINT ( 'NONE',  ( -5.367048706163331850, 7.354919138647580290, -1.599625672291271394 ) ) ;
#11095=CARTESIAN_POINT ( 'NONE',  ( 6.229045230835819069, 6.231917288922055320, -0.7998128361456481317 ) ) ;
#11101=SURFACE_SIDE_STYLE ('',( #143299 ) ) ;
#11106=CIRCLE ( 'NONE', #17884, 0.08000000000000020983 ) ;
#11123=CARTESIAN_POINT ( 'NONE',  ( 4.876420697298537554, 8.045338245374718866, 0.9427337716215690167 ) ) ;
#11131=CARTESIAN_POINT ( 'NONE',  ( 5.155843554946782703, 9.237177590738404831, -0.7998128361456481317 ) ) ;
#11136=CARTESIAN_POINT ( 'NONE',  ( -4.662190612263335865, 8.310640895677696705, -0.4745246276153299858 ) ) ;
#11142=CARTESIAN_POINT ( 'NONE',  ( -7.553827861469316396, 8.841829255582865699, -1.199719254218452047 ) ) ;
#11153=CARTESIAN_POINT ( 'NONE',  ( -6.291865805193673111, 9.498204651771386509, -1.199719254218452047 ) ) ;
#11155=CARTESIAN_POINT ( 'NONE',  ( 5.742760583840166966, 8.857581893525663830, 1.199719254218452047 ) ) ;
#11159=LINE ( 'NONE', #128229, #92249 ) ;
#11165=CARTESIAN_POINT ( 'NONE',  ( 3.705121118284530279, 7.544668081299086282, -1.734723475976807094E-15 ) ) ;
#11169=CARTESIAN_POINT ( 'NONE',  ( 5.031484404002879884, 6.963427452793765404, 1.443375672974065660 ) ) ;
#11177=CARTESIAN_POINT ( 'NONE',  ( -5.472807559815892731, 7.501441282320147508, 1.250076539767187578 ) ) ;
#11178=SHAPE_REPRESENTATION ( 'negative coil', ( #200407 ), #193485 ) ;
#11184=CARTESIAN_POINT ( 'NONE',  ( -3.311934663488232733, 7.085950550703385531, -0.7998128361456481317 ) ) ;
#11185=ADVANCED_FACE ( 'NONE', ( #136399 ), #168874, .T. ) ;
#11186=CARTESIAN_POINT ( 'NONE',  ( 7.702440666339465558, 8.158804663583751449, -0.7216878364870317197 ) ) ;
#11197=CARTESIAN_POINT ( 'NONE',  ( -7.449279056065764237, 7.655523418356991350, 0.7998128361456341429 ) ) ;
#11198=CARTESIAN_POINT ( 'NONE',  ( -6.296835998904160014, 6.311006518335105397, 0.000000000000000000 ) ) ;
#11200=CARTESIAN_POINT ( 'NONE',  ( 5.668717623845194176, 9.627604637879139560, 0.000000000000000000 ) ) ;
#11206=VECTOR ( 'NONE', #134834, 1000.000000000000114 ) ;
#11213=CARTESIAN_POINT ( 'NONE',  ( -6.190206388764837975, 6.963036634120459922, -0.8879648754220506035 ) ) ;
#11217=CARTESIAN_POINT ( 'NONE',  ( 5.153507786970260796, 7.105788066255672497, -1.443375672974078761 ) ) ;
#11222=CARTESIAN_POINT ( 'NONE',  ( -7.632314129850253259, 7.869064337772231355, 0.7998128361456341429 ) ) ;
#11241=CARTESIAN_POINT ( 'NONE',  ( 4.830447868218803897, 8.857549289555754157, -0.7998128361456481317 ) ) ;
#11254=AXIS2_PLACEMENT_3D ( 'NONE', #22281, #2834, #169632 ) ;
#11267=ORIENTED_EDGE ( 'NONE', *, *, #148738, .T. ) ;
#11275=CARTESIAN_POINT ( 'NONE',  ( 4.228163802615382494, 6.026220084508304708, -1.599625672291269396 ) ) ;
#11303=ORIENTED_EDGE ( 'NONE', *, *, #162598, .F. ) ;
#11304=CARTESIAN_POINT ( 'NONE',  ( -5.991777542596674166, 5.955104985976372944, 0.000000000000000000 ) ) ;
#11306=CARTESIAN_POINT ( 'NONE',  ( 6.672020991256494504, 6.956648375986938859, 0.000000000000000000 ) ) ;
#11311=CARTESIAN_POINT ( 'NONE',  ( -5.926849427829407269, 6.943687749669614995, -1.199719254218453823 ) ) ;
#11316=CARTESIAN_POINT ( 'NONE',  ( -5.632486471834530661, 5.535932070087196344, -0.7998128361456362523 ) ) ;
#11318=AXIS2_PLACEMENT_3D ( 'NONE', #60726, #163577, #47709 ) ;
#11319=CARTESIAN_POINT ( 'NONE',  ( -5.764883781430355292, 7.068005876895869122, 2.440105357730325331 ) ) ;
#11324=CARTESIAN_POINT ( 'NONE',  ( -4.450819567036169211, 8.414649604842665553, -0.7998128361456362523 ) ) ;
#11333=CARTESIAN_POINT ( 'NONE',  ( -5.646044625448194410, 5.551749915969804938, 0.000000000000000000 ) ) ;
#11336=CARTESIAN_POINT ( 'NONE',  ( -5.316205630334255972, 8.255971431148344308, -1.082531754730549967 ) ) ;
#11337=CARTESIAN_POINT ( 'NONE',  ( -5.926322542504877333, 7.047036066744706950, -1.082531754730549967 ) ) ;
#11338=CARTESIAN_POINT ( 'NONE',  ( 5.956828388357757298, 8.042995434541133193, 1.599625672291269396 ) ) ;
#11339=CARTESIAN_POINT ( 'NONE',  ( -5.769876891067536206, 8.889217585290882795, 1.199719254218454489 ) ) ;
#11352=ORIENTED_EDGE ( 'NONE', *, *, #160804, .F. ) ;
#11357=CARTESIAN_POINT ( 'NONE',  ( 6.068156270568149324, 9.237210194708310951, 1.199719254218452047 ) ) ;
#11360=AXIS2_PLACEMENT_3D ( 'NONE', #61323, #206490, #59176 ) ;
#11378=CARTESIAN_POINT ( 'NONE',  ( 4.595358334023878832, 8.489709390108890474, -0.01759220550971198060 ) ) ;
#11392=VECTOR ( 'NONE', #196537, 1000.000000000000000 ) ;
#11393=CARTESIAN_POINT ( 'NONE',  ( 4.715203562502613188, 8.723097599553565118, 0.7998128361456341429 ) ) ;
#11396=CARTESIAN_POINT ( 'NONE',  ( -4.625266680917477835, 5.425174544939014964, -1.199719254218453823 ) ) ;
#11400=CARTESIAN_POINT ( 'NONE',  ( -6.251718229232846369, 9.347402796530044355, -1.082531754730549967 ) ) ;
#11411=CIRCLE ( 'NONE', #122067, 2.000000000000000000 ) ;
#11414=CARTESIAN_POINT ( 'NONE',  ( 7.856023664475727308, 8.130058794835305136, -0.7998128361456341429 ) ) ;
#11415=CARTESIAN_POINT ( 'NONE',  ( 4.844006021832467646, 8.873367135438366304, 0.000000000000000000 ) ) ;
#11422=FACE_OUTER_BOUND ( 'NONE', #155978, .T. ) ;
#11428=CARTESIAN_POINT ( 'NONE',  ( 4.850785098639300408, 8.881276058379668825, -0.7998128361456481317 ) ) ;
#11429=ORIENTED_EDGE ( 'NONE', *, *, #18201, .F. ) ;
#11442=CARTESIAN_POINT ( 'NONE',  ( -5.994113311017573054, 6.165756082374834079, 0.7216878364870257245 ) ) ;
#11444=CARTESIAN_POINT ( 'NONE',  ( -5.912237504011027767, 9.055304967058290799, 1.199719254218454489 ) ) ;
#11446=CARTESIAN_POINT ( 'NONE',  ( -4.873355750086138194, 4.879908661787099255, 0.5084451132007505869 ) ) ;
#11458=CARTESIAN_POINT ( 'NONE',  ( 4.850785098639300408, 8.881276058379668825, -0.7998128361456481317 ) ) ;
#11461=CARTESIAN_POINT ( 'NONE',  ( 3.512971199272317602, 6.152197928242737923, -1.082531754730549967 ) ) ;
#11481=CARTESIAN_POINT ( 'NONE',  ( 3.898851692381625877, 6.706354853490643642, -1.199719254218452047 ) ) ;
#11483=CARTESIAN_POINT ( 'NONE',  ( -4.625266680917477835, 5.425174544939014964, -1.199719254218453823 ) ) ;
#11486=CARTESIAN_POINT ( 'NONE',  ( 5.224688093219824303, 7.188831756880171397, -1.599625672291283607 ) ) ;
#11498=CARTESIAN_POINT ( 'NONE',  ( 6.373741612200162443, 8.529394195690610303, 1.443375672974065660 ) ) ;
#11500=CARTESIAN_POINT ( 'NONE',  ( -6.469175572376043348, 7.576401584974034265, 1.199719254218452047 ) ) ;
#11501=CARTESIAN_POINT ( 'NONE',  ( 5.903649544107831382, 5.852288987739402870, -0.7998128361456481317 ) ) ;
#11511=CARTESIAN_POINT ( 'NONE',  ( -4.960304097753355457, 6.880383762169266504, 1.599625672291263179 ) ) ;
#11546=CARTESIAN_POINT ( 'NONE',  ( 3.079110283634975964, 6.606396074300548982, 0.7216878364870257245 ) ) ;
#11558=CARTESIAN_POINT ( 'NONE',  ( -5.330290668828105538, 6.247702530834755130, 1.199719254218452935 ) ) ;
#11560=CARTESIAN_POINT ( 'NONE',  ( -5.803772275101700906, 8.928762199997411386, -1.199719254218452047 ) ) ;
#11562=CARTESIAN_POINT ( 'NONE',  ( 5.817857313595521163, 9.801600942587855414, -0.7216878364870458196 ) ) ;
#11572=CARTESIAN_POINT ( 'NONE',  ( -7.123883369337781879, 7.275895117174344229, 0.7998128361456341429 ) ) ;
#11578=CARTESIAN_POINT ( 'NONE',  ( -3.512971199716682591, 7.112567143062499930, 0.000000000000000000 ) ) ;
#11581=CARTESIAN_POINT ( 'NONE',  ( -5.581116510680924847, 6.540332679663050541, -1.199719254218453823 ) ) ;
#11589=CARTESIAN_POINT ( 'NONE',  ( -6.368956045697454549, 6.779621784316542055, -0.6049335659975106916 ) ) ;
#11600=CARTESIAN_POINT ( 'NONE',  ( -6.954406449166956605, 7.078172043641714595, -0.7998128361456362523 ) ) ;
#11602=CARTESIAN_POINT ( 'NONE',  ( -3.630551273409382329, 7.457669928944732796, 0.7998128361456352531 ) ) ;
#11620=ADVANCED_FACE ( 'NONE', ( #29031 ), #3673, .T. ) ;
#11628=CARTESIAN_POINT ( 'NONE',  ( -5.932574734431526942, 9.079031735882207244, 1.199719254218454489 ) ) ;
#11657=CARTESIAN_POINT ( 'NONE',  ( 7.991605200612358573, 8.288237253661408843, 0.7998128361456281477 ) ) ;
#11669=CARTESIAN_POINT ( 'NONE',  ( 4.978641999450219124, 7.938775605734648799, 1.052364473307040305 ) ) ;
#11671=CARTESIAN_POINT ( 'NONE',  ( 6.048345925472183637, 8.149765894507963182, 1.443375672974065660 ) ) ;
#11677=CARTESIAN_POINT ( 'NONE',  ( -5.632486471834530661, 5.535932070087196344, -0.7998128361456362523 ) ) ;
#11685=CARTESIAN_POINT ( 'NONE',  ( -6.143253000323532831, 7.300121600866474658, 1.082531754730548412 ) ) ;
#11688=CARTESIAN_POINT ( 'NONE',  ( 7.856023664475727308, 8.130058794835305136, -0.7998128361456341429 ) ) ;
#11690=CARTESIAN_POINT ( 'NONE',  ( 5.063152511717405879, 4.908155404373435005, -0.2552525419090029835 ) ) ;
#11695=CARTESIAN_POINT ( 'NONE',  ( -3.688700311369816909, 6.461178242310183784, -1.199719254218450271 ) ) ;
#11705=CARTESIAN_POINT ( 'NONE',  ( 4.934241560730721510, 4.721313007132757811, 0.000000000000000000 ) ) ;
#11719=CARTESIAN_POINT ( 'NONE',  ( -3.752568318859959007, 7.355240624044412812, 0.6449737300090957470 ) ) ;
#11724=CARTESIAN_POINT ( 'NONE',  ( 5.508355548902068577, 9.648441583686274470, 0.7998128361456331437 ) ) ;
#11726=CARTESIAN_POINT ( 'NONE',  ( -5.584154938098890852, 7.410262610144577877, 1.243513269814926492 ) ) ;
#11732=CARTESIAN_POINT ( 'NONE',  ( 5.611095471209277541, 7.639640364534566075, 1.599625672291268286 ) ) ;
#11741=CARTESIAN_POINT ( 'NONE',  ( 5.234856708652235291, 5.279956712948652431, 0.7216878364870338292 ) ) ;
#11744=CARTESIAN_POINT ( 'NONE',  ( 4.245111494854632461, 7.966730820723463502, 0.000000000000000000 ) ) ;
#11756=CARTESIAN_POINT ( 'NONE',  ( -5.153507786970275006, 7.105788066255672497, -1.443375672974066548 ) ) ;
#11762=CARTESIAN_POINT ( 'NONE',  ( 4.572363442555127833, 8.499999999999996447, 0.3169179603640607246 ) ) ;
#11789=CARTESIAN_POINT ( 'NONE',  ( 6.215487077222150880, 6.216099443039444949, 0.000000000000000000 ) ) ;
#11793=DIRECTION ( 'NONE',  ( -0.6507913734559641616, -0.7592566023653004592, 0.000000000000000000 ) ) ;
#11802=CARTESIAN_POINT ( 'NONE',  ( -7.295696057929500711, 7.684269287105433222, 0.7216878364870317197 ) ) ;
#11805=CARTESIAN_POINT ( 'NONE',  ( 4.163762572728282763, 6.911454530608037494, -1.082531754730548412 ) ) ;
#11821=FACE_OUTER_BOUND ( 'NONE', #53816, .T. ) ;
#11846=CARTESIAN_POINT ( 'NONE',  ( -3.492107083971660586, 6.231819477012331632, 1.199719254218452935 ) ) ;
#11853=CARTESIAN_POINT ( 'NONE',  ( -5.643072231634639557, 5.548282123187322945, -0.1753453157342581004 ) ) ;
#11856=CARTESIAN_POINT ( 'NONE',  ( -6.912678218121246942, 9.158153569265168770, 1.599625672291269396 ) ) ;
#11857=CARTESIAN_POINT ( 'NONE',  ( -4.866517195131829787, 8.171732932056599452, 0.9908671576431731243 ) ) ;
#11858=CARTESIAN_POINT ( 'NONE',  ( -5.608633734226008194, 5.643391804966442216, 0.4859901473732997079 ) ) ;
#11862=CARTESIAN_POINT ( 'NONE',  ( -8.041394506236766659, 8.554250810130591631, -0.7216878364870338292 ) ) ;
#11869=CARTESIAN_POINT ( 'NONE',  ( -4.950662367645459305, 5.804802846121667415, -1.199719254218453823 ) ) ;
#11883=CARTESIAN_POINT ( 'NONE',  ( 5.923986774528332333, 5.876015756563318426, -0.7998128361456481317 ) ) ;
#11888=ORIENTED_EDGE ( 'NONE', *, *, #167055, .T. ) ;
#11909=CARTESIAN_POINT ( 'NONE',  ( 5.499767588998890844, 6.445425604367387429, 1.199719254218451159 ) ) ;
#11910=CARTESIAN_POINT ( 'NONE',  ( 4.760848217054122422, 5.583353003765119560, -1.199719254218452047 ) ) ;
#11912=CARTESIAN_POINT ( 'NONE',  ( 5.239300017038202917, 5.077214539491492928, 0.000000000000000000 ) ) ;
#11926=CARTESIAN_POINT ( 'NONE',  ( 4.655672573246532941, 8.415299432525721102, 0.4976263304441782553 ) ) ;
#11927=CARTESIAN_POINT ( 'NONE',  ( -3.960390268523300339, 7.634556056670224855, 1.214306433183764966E-14 ) ) ;
#11928=CARTESIAN_POINT ( 'NONE',  ( -3.035422819611498735, 6.295728927258597452, 0.6346236910419257304 ) ) ;
#11953=CARTESIAN_POINT ( 'NONE',  ( 8.000720045840086669, 8.506797273001177828, 0.7216878364870267237 ) ) ;
#11972=CARTESIAN_POINT ( 'NONE',  ( -5.582925393777276035, 9.735439736040634173, 0.7998128361456291469 ) ) ;
#11977=CARTESIAN_POINT ( 'NONE',  ( -5.608717438317167847, 5.638785078248324645, 0.4778177780641221228 ) ) ;
#11987=CARTESIAN_POINT ( 'NONE',  ( 4.199993725183334803, 8.122019456014369254, -0.7998128361456362523 ) ) ;
#12001=AXIS2_PLACEMENT_3D ( 'NONE', #81531, #79397, #144447 ) ;
#12005=CARTESIAN_POINT ( 'NONE',  ( -3.981404450745295254, 7.309521899770400566, -0.7443278975401018682 ) ) ;
#12013=CARTESIAN_POINT ( 'NONE',  ( -6.190835592010745181, 6.962597444594667451, 0.8873991478343831174 ) ) ;
#12014=CARTESIAN_POINT ( 'NONE',  ( 2.925527285498711549, 6.635141943048991742, 0.7998128361456281477 ) ) ;
#12020=CARTESIAN_POINT ( 'NONE',  ( -5.224688093219839402, 7.188831756880171397, -1.599625672291271394 ) ) ;
#12022=CARTESIAN_POINT ( 'NONE',  ( 4.552505719138623341, 8.533283448962240669, 0.7998128361456341429 ) ) ;
#12027=CARTESIAN_POINT ( 'NONE',  ( -6.424584688029276514, 8.588711117491191871, 1.599625672291269396 ) ) ;
#12034=CARTESIAN_POINT ( 'NONE',  ( -4.728114892278019177, 8.325812319508695936, -0.7463954279460782715 ) ) ;
#12054=CARTESIAN_POINT ( 'NONE',  ( 5.912764389335563919, 6.070849007079172743, -0.7216878364870458196 ) ) ;
#12056=DIRECTION ( 'NONE',  ( -1.000000000000000000, 0.000000000000000000, 0.000000000000000000 ) ) ;
#12073=CARTESIAN_POINT ( 'NONE',  ( 5.574337433874081427, 6.532423756721743580, -1.199719254218452047 ) ) ;
#12080=DIRECTION ( 'NONE',  ( 0.000000000000000000, -1.000000000000000000, 0.000000000000000000 ) ) ;
#12111=LINE ( 'NONE', #65114, #190282 ) ;
#12120=CARTESIAN_POINT ( 'NONE',  ( -3.634994581795317536, 7.254927755487573293, 0.000000000000000000 ) ) ;
#12128=CARTESIAN_POINT ( 'NONE',  ( -6.286140498591554326, 7.362860665558790707, 1.199719254218452047 ) ) ;
#12133=VERTEX_POINT ( 'NONE', #109950 ) ;
#12137=CARTESIAN_POINT ( 'NONE',  ( -3.644109427023046521, 7.473487774827342278, 0.000000000000000000 ) ) ;
#12140=CARTESIAN_POINT ( 'NONE',  ( 6.597622414017595638, 6.771646741010207471, 0.1687998040609314243 ) ) ;
#12145=CARTESIAN_POINT ( 'NONE',  ( 6.042093733545556233, 7.078139439671806699, -1.199719254218452047 ) ) ;
#12152=CARTESIAN_POINT ( 'NONE',  ( -4.004454267989906668, 5.765225627445230927, 1.599625672291270506 ) ) ;
#12156=AXIS2_PLACEMENT_3D ( 'NONE', #120248, #134330, #152673 ) ;
#12159=CARTESIAN_POINT ( 'NONE',  ( -6.459533842268148973, 6.500820668926428958, 0.000000000000000000 ) ) ;
#12162=CARTESIAN_POINT ( 'NONE',  ( -3.629765072269336201, 7.456752694281346905, -0.3535274064819134421 ) ) ;
#12163=CARTESIAN_POINT ( 'NONE',  ( 5.763624699140868834, 7.817591130454727200, -1.443375672974078761 ) ) ;
#12164=CARTESIAN_POINT ( 'NONE',  ( -6.631346530415505036, 7.869564052640446228, 1.082531754730549078 ) ) ;
#12168=CARTESIAN_POINT ( 'NONE',  ( -4.288121723672178476, 8.224835454251337552, -0.7998128361456361413 ) ) ;
#12171=CARTESIAN_POINT ( 'NONE',  ( 4.366607992053101128, 7.252070536440704096, -1.199719254218448494 ) ) ;
#12177=CARTESIAN_POINT ( 'NONE',  ( 6.554440917563796987, 6.611545590104705994, -0.7998128361456481317 ) ) ;
#12195=CARTESIAN_POINT ( 'NONE',  ( 5.346441918567009566, 7.700601260040275342, -1.357055567468886670 ) ) ;
#12199=CARTESIAN_POINT ( 'NONE',  ( 4.633164669693822901, 8.325607986553848150, 0.3865003237762173471 ) ) ;
#12205=CARTESIAN_POINT ( 'NONE',  ( 5.508355548902068577, 9.648441583686274470, 0.7998128361456331437 ) ) ;
#12210=CARTESIAN_POINT ( 'NONE',  ( -5.000347810418038996, 7.933946187056884369, 1.064693650161437022 ) ) ;
#12216=CARTESIAN_POINT ( 'NONE',  ( -7.608060475923978494, 8.905100639113307182, 1.199719254218452047 ) ) ;
#12226=CARTESIAN_POINT ( 'NONE',  ( -7.587723245503481095, 8.881373870289390737, 1.199719254218452047 ) ) ;
#12228=CARTESIAN_POINT ( 'NONE',  ( 7.550965208168244125, 7.774157262476569130, -0.7998128361456341429 ) ) ;
#12236=CARTESIAN_POINT ( 'NONE',  ( 5.611095471209277541, 7.639640364534566075, 1.599625672291268286 ) ) ;
#12239=CARTESIAN_POINT ( 'NONE',  ( 4.692530563661249765, 8.488719734331187539, 0.000000000000000000 ) ) ;
#12246=FACE_OUTER_BOUND ( 'NONE', #86439, .T. ) ;
#12247=CARTESIAN_POINT ( 'NONE',  ( -6.378792857440260811, 6.837131066116997502, 0.5844455422965456615 ) ) ;
#12254=CARTESIAN_POINT ( 'NONE',  ( -3.634467696915153034, 6.397906858779740524, 1.199719254218452935 ) ) ;
#12255=CARTESIAN_POINT ( 'NONE',  ( 5.560252395380198998, 9.501061871336672127, 0.7216878364870317197 ) ) ;
#12265=CARTESIAN_POINT ( 'NONE',  ( -6.720001414228860881, 7.869031733802326123, -1.199719254218452047 ) ) ;
#12266=CARTESIAN_POINT ( 'NONE',  ( -4.288121723672178476, 8.224835454251337552, -0.7998128361456362523 ) ) ;
#12268=CARTESIAN_POINT ( 'NONE',  ( 5.994113310573177422, 10.00723293906178846, 0.000000000000000000 ) ) ;
#12272=DIRECTION ( 'NONE',  ( -0.6507913734559630514, -0.7592566023653011253, 0.000000000000000000 ) ) ;
#12279=CARTESIAN_POINT ( 'NONE',  ( -5.917914848013369422, 7.154962168230770025, -1.123475595150375650 ) ) ;
#12286=CARTESIAN_POINT ( 'NONE',  ( -7.282664789195997912, 8.525472337930658284, 1.199719254218452047 ) ) ;
#12303=CARTESIAN_POINT ( 'NONE',  ( 4.532168488718122390, 8.509556680138327778, 0.7998128361456271485 ) ) ;
#12337=CARTESIAN_POINT ( 'NONE',  ( 4.740510986633625024, 5.559626234941203116, -1.199719254218450271 ) ) ;
#12353=FACE_BOUND ( 'NONE', #150257, .T. ) ;
#12369=CARTESIAN_POINT ( 'NONE',  ( -4.145761110728687804, 8.058748072483927771, -0.7998128361456481317 ) ) ;
#12371=CARTESIAN_POINT ( 'NONE',  ( 7.309254211098767051, 7.700087132469628948, 0.7216878364870267237 ) ) ;
#12376=CARTESIAN_POINT ( 'NONE',  ( -4.817943484809863008, 6.714296380401858499, 1.599625672291263179 ) ) ;
#12381=CARTESIAN_POINT ( 'NONE',  ( -2.823841133396259639, 6.516508098929413961, -0.7998128361456481317 ) ) ;
#12383=CARTESIAN_POINT ( 'NONE',  ( -1.808247988047325228, 2.517446015412732940, 2.499984125739859842 ) ) ;
#12388=CARTESIAN_POINT ( 'NONE',  ( -5.906512197408906317, 6.919960980845699439, -1.199719254218453823 ) ) ;
#12398=CARTESIAN_POINT ( 'NONE',  ( -4.716257332707368910, 6.595662536282280719, -1.599625672291271394 ) ) ;
#12401=CARTESIAN_POINT ( 'NONE',  ( -6.129694847154222970, 7.284303755502281597, -1.082531754730549967 ) ) ;
#12402=CARTESIAN_POINT ( 'NONE',  ( -7.065207446052822249, 7.415365906582643163, -0.7216878364870338292 ) ) ;
#12403=CARTESIAN_POINT ( 'NONE',  ( 6.821687566331318564, 7.987665577921906568, 1.199719254218452935 ) ) ;
#12405=CARTESIAN_POINT ( 'NONE',  ( -6.444921918449773024, 8.612437886315108315, 1.599625672291269396 ) ) ;
#12443=CARTESIAN_POINT ( 'NONE',  ( 4.669458948634179762, 8.398658883068243597, -0.5498995856093937817 ) ) ;
#12461=CARTESIAN_POINT ( 'NONE',  ( 6.387826650694035990, 7.481494509678370264, -1.199719254218452047 ) ) ;
#12464=CARTESIAN_POINT ( 'NONE',  ( -5.815521545619021460, 5.749472989502435460, -0.7998128361456362523 ) ) ;
#12468=CARTESIAN_POINT ( 'NONE',  ( -7.892254816486440561, 8.380254505421877553, 0.000000000000000000 ) ) ;
#12480=CARTESIAN_POINT ( 'NONE',  ( 5.820193082016415609, 10.01225203898631655, 0.000000000000000000 ) ) ;
#12481=CARTESIAN_POINT ( 'NONE',  ( 4.355912491740495440, 8.303924683664389406, 0.000000000000000000 ) ) ;
#12496=CARTESIAN_POINT ( 'NONE',  ( 6.658989722967328717, 7.797851427330578566, 1.199719254218452935 ) ) ;
#12510=CARTESIAN_POINT ( 'NONE',  ( -4.828112100242291760, 6.726159765073026264, -1.443375672974066548 ) ) ;
#12511=CARTESIAN_POINT ( 'NONE',  ( -5.088052786878465739, 9.158088361325352977, 0.000000000000000000 ) ) ;
#12517=ORIENTED_EDGE ( 'NONE', *, *, #115159, .T. ) ;
#12523=CARTESIAN_POINT ( 'NONE',  ( 5.851225812749518695, 8.984124660586543243, -1.199719254218452047 ) ) ;
#12526=CARTESIAN_POINT ( 'NONE',  ( 8.188198428010544205, 8.517596018959260107, 0.000000000000000000 ) ) ;
#12540=CARTESIAN_POINT ( 'NONE',  ( 6.062430963966053632, 7.101866208495718702, -1.199719254218452047 ) ) ;
#12542=CARTESIAN_POINT ( 'NONE',  ( -4.817943484809863008, 6.714296380401858499, 1.599625672291263179 ) ) ;
#12545=CARTESIAN_POINT ( 'NONE',  ( 6.222266154028957885, 6.224008365980749247, 0.7998128361456352531 ) ) ;
#12555=CARTESIAN_POINT ( 'NONE',  ( 7.377044979611483200, 7.779176362401098999, -0.7216878364870317197 ) ) ;
#12557=CARTESIAN_POINT ( 'NONE',  ( -7.781453819600577582, 8.043060642480948985, 0.000000000000000000 ) ) ;
#12558=CARTESIAN_POINT ( 'NONE',  ( 5.204350862799327793, 7.165104988056252289, -1.599625672291281386 ) ) ;
#12559=ORIENTED_EDGE ( 'NONE', *, *, #167354, .T. ) ;
#12569=CARTESIAN_POINT ( 'NONE',  ( -5.204350862799341115, 7.165104988056252289, -1.599625672291271394 ) ) ;
#12597=CARTESIAN_POINT ( 'NONE',  ( 5.736508392357904107, 5.865217010605237924, 0.000000000000000000 ) ) ;
#12604=CARTESIAN_POINT ( 'NONE',  ( 4.624739795592929248, 6.488892076315451618, -1.443375672974068769 ) ) ;
#12616=CARTESIAN_POINT ( 'NONE',  ( -6.282224075085783177, 8.422623735723785643, 1.599625672291269396 ) ) ;
#12618=CARTESIAN_POINT ( 'NONE',  ( -5.250750630242457362, 9.347902511916677426, 0.000000000000000000 ) ) ;
#12620=CARTESIAN_POINT ( 'NONE',  ( 7.038091138825468107, 8.344099429118761790, -1.082531754730548412 ) ) ;
#12631=CARTESIAN_POINT ( 'NONE',  ( -6.231907884136888676, 7.299589282028351001, -1.199719254218453823 ) ) ;
#12637=CARTESIAN_POINT ( 'NONE',  ( -4.340018570150309785, 7.117086527600392287, -1.082531754730551743 ) ) ;
#12642=CARTESIAN_POINT ( 'NONE',  ( -4.261005416444848315, 8.193199762486115034, 0.7998128361456352531 ) ) ;
#12660=CARTESIAN_POINT ( 'NONE',  ( -6.740338644649361832, 7.892758502626242567, -1.199719254218452047 ) ) ;
#12662=CARTESIAN_POINT ( 'NONE',  ( -5.276058054373441664, 6.184431147304315424, -1.199719254218453823 ) ) ;
#12685=CARTESIAN_POINT ( 'NONE',  ( -6.631873415740034083, 7.766215735565355160, 1.199719254218452047 ) ) ;
#12711=CARTESIAN_POINT ( 'NONE',  ( 6.831329296439236032, 9.063246493969506545, -1.599625672291267398 ) ) ;
#12726=CARTESIAN_POINT ( 'NONE',  ( 5.779562687394081522, 7.242644825714458001, 1.188994900607452054 ) ) ;
#12728=CARTESIAN_POINT ( 'NONE',  ( 6.455090533882185788, 8.624301270986276080, -1.443375672974078761 ) ) ;
#12733=CARTESIAN_POINT ( 'NONE',  ( -4.098307573080856692, 8.003385611894792362, 0.7998128361456352531 ) ) ;
#12740=CARTESIAN_POINT ( 'NONE',  ( -6.929625909916163451, 7.257187447756535903, 0.7216878364870317197 ) ) ;
#12749=CARTESIAN_POINT ( 'NONE',  ( -3.526002468005825286, 6.271364091718859335, -1.199719254218450271 ) ) ;
#12759=CARTESIAN_POINT ( 'NONE',  ( 3.573456005653643519, 6.326726552307992080, -1.199719254218453823 ) ) ;
#12775=CARTESIAN_POINT ( 'NONE',  ( -3.147653791585727667, 8.920000000000001705, -2.419999999999998597 ) ) ;
#12779=CARTESIAN_POINT ( 'NONE',  ( -6.237633190739009237, 9.434933268240943249, 1.199719254218452047 ) ) ;
#12782=CARTESIAN_POINT ( 'NONE',  ( 7.018280793729500644, 8.217024343219755167, -1.199719254218452047 ) ) ;
#12784=CARTESIAN_POINT ( 'NONE',  ( -5.520246714036333380, 7.462180650995058784, 1.249303437716933196 ) ) ;
#12790=CARTESIAN_POINT ( 'NONE',  ( 3.867818961648523235, 7.734482231890414283, 1.040834085586084257E-14 ) ) ;
#12793=CARTESIAN_POINT ( 'NONE',  ( -5.582187619986996197, 5.827946089707462640, -0.5328595319416041809 ) ) ;
#12798=CARTESIAN_POINT ( 'NONE',  ( 4.584065335196271462, 5.481069324884694005, 1.082531754730549078 ) ) ;
#12801=CARTESIAN_POINT ( 'NONE',  ( -4.588905297609556122, 8.492063665195846767, -0.2916239738018167604 ) ) ;
#12802=CARTESIAN_POINT ( 'NONE',  ( 4.258669648468268676, 7.982548666606070320, 0.7216878364870257245 ) ) ;
#12803=ORIENTED_EDGE ( 'NONE', *, *, #68702, .F. ) ;
#12813=CARTESIAN_POINT ( 'NONE',  ( -5.153507786970267013, 8.066157280557016307, -1.082531754730549967 ) ) ;
#12839=DIRECTION ( 'NONE',  ( -0.000000000000000000, 1.000000000000000000, -0.000000000000000000 ) ) ;
#12846=CARTESIAN_POINT ( 'NONE',  ( 5.017399365509065845, 8.011327138806002779, -1.199719254218450271 ) ) ;
#12848=CARTESIAN_POINT ( 'NONE',  ( 5.417364897112183719, 8.477953592343014932, 1.199719254218451159 ) ) ;
#12859=CARTESIAN_POINT ( 'NONE',  ( -7.322812365156824654, 8.676274193172000437, 1.082531754730549078 ) ) ;
#12861=AXIS2_PLACEMENT_3D ( 'NONE', #129983, #127864, #163472 ) ;
#12863=CARTESIAN_POINT ( 'NONE',  ( 4.597623488365603528, 5.496887170248887067, -1.082531754730548412 ) ) ;
#12872=CARTESIAN_POINT ( 'NONE',  ( 5.100855621065027101, 7.816023350749504495, -1.153872196553248131 ) ) ;
#12878=CARTESIAN_POINT ( 'NONE',  ( -5.316205630334263965, 7.295602216847000498, -1.443375672974066548 ) ) ;
#12880=CARTESIAN_POINT ( 'NONE',  ( -5.492461627311929995, 5.580495784718250363, 0.000000000000000000 ) ) ;
#12883=CARTESIAN_POINT ( 'NONE',  ( 4.769174622299096278, 4.736660945536613099, -0.4712523532527379544 ) ) ;
#12887=CARTESIAN_POINT ( 'NONE',  ( 3.542423274920540432, 7.354853930707762721, -1.734723475976807094E-15 ) ) ;
#12905=CARTESIAN_POINT ( 'NONE',  ( 4.689424523294686509, 8.358602041046323095, -0.7454045323363467368 ) ) ;
#12916=CARTESIAN_POINT ( 'NONE',  ( -7.937372586157736443, 8.224965870130965584, 0.7998128361456341429 ) ) ;
#12917=CARTESIAN_POINT ( 'NONE',  ( -4.688377817131518910, 8.372325690950924937, 0.6434091164432588217 ) ) ;
#12927=CARTESIAN_POINT ( 'NONE',  ( -5.167592825464113915, 6.057888380243431570, 1.199719254218452935 ) ) ;
#12942=CARTESIAN_POINT ( 'NONE',  ( 6.222266154028957885, 6.224008365980749247, 0.7998128361456352531 ) ) ;
#12960=AXIS2_PLACEMENT_3D ( 'NONE', #121436, #39036, #189541 ) ;
#12969=CARTESIAN_POINT ( 'NONE',  ( 4.529305835417093640, 7.441884687032027657, -1.199719254218450271 ) ) ;
#12970=CARTESIAN_POINT ( 'NONE',  ( 3.549202351727371862, 7.362762853649070571, -0.7998128361456362523 ) ) ;
#12972=CARTESIAN_POINT ( 'NONE',  ( 4.415115299905642665, 5.179997933758551554, -1.199719254218450271 ) ) ;
#12985=CARTESIAN_POINT ( 'NONE',  ( 5.004104291928844539, 8.031804922028364047, 1.127571413376940335 ) ) ;
#12986=CARTESIAN_POINT ( 'NONE',  ( -6.441532379824190357, 6.687744995982559892, 0.7216878364870257245 ) ) ;
#12987=CARTESIAN_POINT ( 'NONE',  ( 5.085717018901939390, 5.105960408239938353, 0.000000000000000000 ) ) ;
#13012=CARTESIAN_POINT ( 'NONE',  ( 4.030516805012513082, 7.924296382481737844, 0.000000000000000000 ) ) ;
#13014=CARTESIAN_POINT ( 'NONE',  ( 3.790386463472274148, 6.579812086429759788, 1.199719254218452047 ) ) ;
#13031=CARTESIAN_POINT ( 'NONE',  ( -6.607619761813764647, 8.802252036906432764, 1.599625672291269396 ) ) ;
#13042=CARTESIAN_POINT ( 'NONE',  ( 4.193214648376505593, 8.114110533073061404, 0.000000000000000000 ) ) ;
#13048=CARTESIAN_POINT ( 'NONE',  ( 4.389807875774629942, 8.343469298370917997, 0.7998128361456271485 ) ) ;
#13057=CARTESIAN_POINT ( 'NONE',  ( -0.4461809497497640775, 3.122791860410086606, 1.949595486268987043 ) ) ;
#13058=CIRCLE ( 'NONE', #44172, 3.100000000000000089 ) ;
#13060=CARTESIAN_POINT ( 'NONE',  ( 4.594558193676899549, 8.374302254291812631, 0.02480325318809234458 ) ) ;
#13072=CARTESIAN_POINT ( 'NONE',  ( -6.328041841479842056, 6.870487382198048998, 0.6860574420480938240 ) ) ;
#13074=ORIENTED_EDGE ( 'NONE', *, *, #68041, .T. ) ;
#13080=CARTESIAN_POINT ( 'NONE',  ( -6.317173229324657413, 6.334733287159020954, 0.000000000000000000 ) ) ;
#13082=CARTESIAN_POINT ( 'NONE',  ( 4.766573523656222555, 7.718696989977711809, 1.199719254218452047 ) ) ;
#13083=CARTESIAN_POINT ( 'NONE',  ( -1.806654366501805775, 2.518449987798942136, 2.500000000000000444 ) ) ;
#13086=CARTESIAN_POINT ( 'NONE',  ( -7.435720902452096936, 7.639705572474380091, 0.000000000000000000 ) ) ;
#13096=CARTESIAN_POINT ( 'NONE',  ( -0.2903009011402963302, 2.705340922360735423, -2.053590887664075382 ) ) ;
#13102=EDGE_CURVE ( 'NONE', #12133, #207685, #12111, .T. ) ;
#13106=ADVANCED_FACE ( 'NONE', ( #128103 ), #114302, .T. ) ;
#13116=CARTESIAN_POINT ( 'NONE',  ( 5.804299160426222848, 7.865044668620976509, -1.443375672974078761 ) ) ;
#13120=VERTEX_POINT ( 'NONE', #144310 ) ;
#13123=VERTEX_POINT ( 'NONE', #109699 ) ;
#13131=CARTESIAN_POINT ( 'NONE',  ( -3.662110889467009578, 7.286563447771212232, 0.7216878364870338292 ) ) ;
#13135=CARTESIAN_POINT ( 'NONE',  ( 6.059568310664962709, 6.034194215389424798, 0.7998128361456352531 ) ) ;
#13190=CARTESIAN_POINT ( 'NONE',  ( -5.112833325684920993, 6.097965313788082931, -1.082531754730549967 ) ) ;
#13197=CARTESIAN_POINT ( 'NONE',  ( -4.450819567036169211, 8.414649604842665553, -0.7998128361456362523 ) ) ;
#13204=ORIENTED_EDGE ( 'NONE', *, *, #81172, .F. ) ;
#13208=CARTESIAN_POINT ( 'NONE',  ( -3.481411583659053566, 7.283673624236017830, 0.000000000000000000 ) ) ;
#13211=CARTESIAN_POINT ( 'NONE',  ( 6.459053645710411296, 6.863086831863287607, 0.6637952124323226455 ) ) ;
#13216=CARTESIAN_POINT ( 'NONE',  ( 6.852720297064418986, 6.959538199522133262, 0.7998128361456331437 ) ) ;
#13223=CARTESIAN_POINT ( 'NONE',  ( -7.370792787684826486, 8.628288336167626582, -1.199719254218452047 ) ) ;
#13225=EDGE_LOOP ( 'NONE', ( #109414, #214149, #122485, #212579, #28246 ) ) ;
#13229=CARTESIAN_POINT ( 'NONE',  ( -6.069210040772897052, 7.109775131437022999, -1.199719254218453823 ) ) ;
#13234=CARTESIAN_POINT ( 'NONE',  ( 5.343321937117211817, 9.247976336696488886, 0.000000000000000000 ) ) ;
#13236=CARTESIAN_POINT ( 'NONE',  ( -5.085717018457573957, 8.947437264926888290, 0.7216878364870267237 ) ) ;
#13243=CARTESIAN_POINT ( 'NONE',  ( 6.201928923608456046, 6.200281597156833691, 0.7998128361456352531 ) ) ;
#13267=CARTESIAN_POINT ( 'NONE',  ( 4.963960565410041603, 8.060099936542098220, -1.154953748940761971 ) ) ;
#13272=CARTESIAN_POINT ( 'NONE',  ( 5.107728353013315292, 7.811434107096660640, 1.148430247377411728 ) ) ;
#13281=CARTESIAN_POINT ( 'NONE',  ( 5.182959862174088883, 9.268813282503625572, 0.7998128361456331437 ) ) ;
#13286=CARTESIAN_POINT ( 'NONE',  ( -6.033312665451926904, 7.071988487544162538, -1.043104321438679039 ) ) ;
#13292=CARTESIAN_POINT ( 'NONE',  ( -4.963693635934603776, 4.963599794778024155, 0.000000000000000000 ) ) ;
#13302=CARTESIAN_POINT ( 'NONE',  ( -5.517242166118370150, 5.401480380085008193, 0.7998128361456281477 ) ) ;
#13308=CARTESIAN_POINT ( 'NONE',  ( 6.116136693540529912, 10.14959355252369910, 1.530808498934192557E-16 ) ) ;
#13312=CARTESIAN_POINT ( 'NONE',  ( 4.692003678781083487, 7.631698837623355658, -1.199719254218450271 ) ) ;
#13315=CARTESIAN_POINT ( 'NONE',  ( 5.194182247366869731, 7.153241603385088965, 1.443375672974064550 ) ) ;
#13329=CARTESIAN_POINT ( 'NONE',  ( -3.610214042988883598, 7.433943160120816351, 0.7998128361456352531 ) ) ;
#13330=CARTESIAN_POINT ( 'NONE',  ( 3.854260808034858155, 7.718664386007802136, -0.7998128361456362523 ) ) ;
#13341=CARTESIAN_POINT ( 'NONE',  ( -5.399890319992785237, 9.521898816625391504, 0.7998128361456291469 ) ) ;
#13342=CARTESIAN_POINT ( 'NONE',  ( 6.638652492546827766, 7.774124658506663010, 1.199719254218452047 ) ) ;
#13344=CARTESIAN_POINT ( 'NONE',  ( 7.810905894804431426, 8.285347430126213553, 0.000000000000000000 ) ) ;
#13348=ORIENTED_EDGE ( 'NONE', *, *, #46280, .F. ) ;
#13349=CARTESIAN_POINT ( 'NONE',  ( 3.067887898442204442, 6.801229324816399746, 0.7998128361456271485 ) ) ;
#13356=CARTESIAN_POINT ( 'NONE',  ( -6.146561906247310247, 6.992958819738270826, -0.9370148970899976337 ) ) ;
#13365=CARTESIAN_POINT ( 'NONE',  ( -7.553827861469316396, 8.841829255582865699, -1.199719254218452047 ) ) ;
#13371=CARTESIAN_POINT ( 'NONE',  ( -5.467155955761412223, 6.078795959345912436, -0.9674530110256196469 ) ) ;
#13380=CARTESIAN_POINT ( 'NONE',  ( 6.879836604291781121, 6.991173891287354003, -0.7998128361456341429 ) ) ;
#13413=CARTESIAN_POINT ( 'NONE',  ( 5.415556014015861841, 5.282846535965431300, -0.7998128361456481317 ) ) ;
#13444=CARTESIAN_POINT ( 'NONE',  ( -4.633854640820660009, 8.628190524257904670, -0.7998128361456362523 ) ) ;
#13446=CARTESIAN_POINT ( 'NONE',  ( 6.495764994278809823, 7.711385593814346073, 1.082531754730549967 ) ) ;
#13448=AXIS2_PLACEMENT_3D ( 'NONE', #116369, #51314, #135772 ) ;
#13452=CARTESIAN_POINT ( 'NONE',  ( -4.980641328173854632, 6.904110530993182948, 1.599625672291263179 ) ) ;
#13457=CARTESIAN_POINT ( 'NONE',  ( -5.157951095356222204, 4.982307464195829816, 0.000000000000000000 ) ) ;
#13462=CARTESIAN_POINT ( 'NONE',  ( -6.608673532018475960, 6.674816973635147477, -0.7998128361456362523 ) ) ;
#13472=CARTESIAN_POINT ( 'NONE',  ( -3.772911886352873445, 7.623757310712140800, 0.7998128361456352531 ) ) ;
#13476=CARTESIAN_POINT ( 'NONE',  ( -5.261973015879593873, 8.192700047617899273, 1.082531754730549967 ) ) ;
#13477=CARTESIAN_POINT ( 'NONE',  ( -6.251718229232856139, 8.387033582228697881, -1.443375672974066548 ) ) ;
#13478=CARTESIAN_POINT ( 'NONE',  ( 6.984385409695311964, 8.177479728513226576, 1.199719254218452935 ) ) ;
#13479=CARTESIAN_POINT ( 'NONE',  ( -5.271087860662956537, 9.371629280740593870, 0.000000000000000000 ) ) ;
#13499=B_SPLINE_CURVE_WITH_KNOTS ( 'NONE', 3,
 ( #71285, #50795, #4147, #149365 ),
 .UNSPECIFIED., .F., .F.,
 ( 4, 4 ),
 ( 0.0004304244924211256284, 0.0006956056399114353287 ),
 .UNSPECIFIED. ) ;
#13501=ORIENTED_EDGE ( 'NONE', *, *, #208272, .F. ) ;
#13520=CARTESIAN_POINT ( 'NONE',  ( 4.650542599771462449, 8.421518672640367242, 0.4769741307986720136 ) ) ;
#13536=CARTESIAN_POINT ( 'NONE',  ( 5.580062740476173566, 8.667767742934335828, 1.199719254218451159 ) ) ;
#13539=CARTESIAN_POINT ( 'NONE',  ( -4.132202957115018727, 8.042930226601317401, 0.000000000000000000 ) ) ;
#13543=CARTESIAN_POINT ( 'NONE',  ( -6.739811759324831897, 7.996106819701333634, -1.082531754730549967 ) ) ;
#13551=CARTESIAN_POINT ( 'NONE',  ( 6.073126464278658432, 6.050012061272033392, 0.000000000000000000 ) ) ;
#13553=CARTESIAN_POINT ( 'NONE',  ( 4.830447868218803897, 8.857549289555754157, -0.7998128361456481317 ) ) ;
#13558=CARTESIAN_POINT ( 'NONE',  ( -4.791166081694341550, 4.882818525799564213, 0.4357780244859492669 ) ) ;
#13562=CARTESIAN_POINT ( 'NONE',  ( 3.923105346307896202, 5.670318552149568703, -1.599625672291269396 ) ) ;
#13568=CARTESIAN_POINT ( 'NONE',  ( 7.361151057576892143, 7.552707420120024828, 0.7998128361456291469 ) ) ;
#13578=CARTESIAN_POINT ( 'NONE',  ( -2.952042078427798533, 6.300591463180486684, -0.5728661040586968678 ) ) ;
#13581=CARTESIAN_POINT ( 'NONE',  ( -4.001064729808656573, 7.682009594836471500, 1.214306433183764966E-14 ) ) ;
#13582=CARTESIAN_POINT ( 'NONE',  ( 3.770576118376296471, 7.413106214832098750, 0.7216878364870257245 ) ) ;
#13587=EDGE_LOOP ( 'NONE', ( #51154, #55833, #99286, #12803 ) ) ;
#13591=EDGE_LOOP ( 'NONE', ( #18635, #112933, #190831, #148500, #160653, #41297, #114528 ) ) ;
#13593=CARTESIAN_POINT ( 'NONE',  ( -6.211043768836215229, 8.339580045099285854, 1.443375672974064550 ) ) ;
#13594=CARTESIAN_POINT ( 'NONE',  ( 5.989670002187236442, 10.20997511251894529, -0.7998128361456481317 ) ) ;
#13597=CARTESIAN_POINT ( 'NONE',  ( 5.370438244344566847, 5.438135171256338829, 0.000000000000000000 ) ) ;
#13615=CARTESIAN_POINT ( 'NONE',  ( 4.213551878797002992, 8.137837301896977849, 0.000000000000000000 ) ) ;
#13617=CARTESIAN_POINT ( 'NONE',  ( -3.142457743317409680, 6.888227477170756785, 0.7998128361456352531 ) ) ;
#13628=CARTESIAN_POINT ( 'NONE',  ( 7.187230829020129441, 8.518095734345896730, 1.082531754730549967 ) ) ;
#13630=CARTESIAN_POINT ( 'NONE',  ( -6.257970421159510188, 9.458660037064859694, 1.199719254218452047 ) ) ;
#13631=CARTESIAN_POINT ( 'NONE',  ( 6.852720297064418986, 6.959538199522133262, 0.7998128361456331437 ) ) ;
#13640=CARTESIAN_POINT ( 'NONE',  ( -6.283277845290492714, 6.295188672452495915, -0.7998128361456362523 ) ) ;
#13652=CARTESIAN_POINT ( 'NONE',  ( 6.116136693540529912, 10.14959355252369910, 1.530808498934192557E-16 ) ) ;
#13667=CARTESIAN_POINT ( 'NONE',  ( 3.933273961740296087, 6.642551151122080277, 1.082531754730549078 ) ) ;
#13673=EDGE_CURVE ( 'NONE', #78850, #130236, #86084, .T. ) ;
#13674=CARTESIAN_POINT ( 'NONE',  ( 5.573810548549551491, 6.635772073796838200, -1.082531754730548412 ) ) ;
#13675=ORIENTED_EDGE ( 'NONE', *, *, #156704, .F. ) ;
#13687=CARTESIAN_POINT ( 'NONE',  ( -5.010620288702242853, 8.003418215864698482, -1.199719254218453823 ) ) ;
#13689=CARTESIAN_POINT ( 'NONE',  ( -5.912237504011027767, 9.055304967058290799, 1.199719254218454489 ) ) ;
#13695=CARTESIAN_POINT ( 'NONE',  ( 7.364013710877980401, 8.620379413226322285, -1.199719254218452047 ) ) ;
#13700=CARTESIAN_POINT ( 'NONE',  ( -5.529746549527323474, 7.544733289238903851, -1.599625672291271394 ) ) ;
#13707=CARTESIAN_POINT ( 'NONE',  ( -3.987506576194992824, 7.666191748953863794, 0.7216878364870338292 ) ) ;
#13710=CARTESIAN_POINT ( 'NONE',  ( -5.795184315198522285, 5.725746220678519904, -0.7998128361456362523 ) ) ;
#13730=ORIENTED_EDGE ( 'NONE', *, *, #88854, .F. ) ;
#13731=CARTESIAN_POINT ( 'NONE',  ( -7.930593509350902792, 8.217056947189661287, -0.7998128361456362523 ) ) ;
#13732=CARTESIAN_POINT ( 'NONE',  ( 4.435452530326143616, 5.203724702582467998, -1.199719254218452047 ) ) ;
#13733=CARTESIAN_POINT ( 'NONE',  ( -5.061990249855848667, 6.999017606288844284, -1.599625672291271394 ) ) ;
#13757=CARTESIAN_POINT ( 'NONE',  ( -5.582925393777276035, 9.735439736040634173, 0.7998128361456291469 ) ) ;
#13764=CARTESIAN_POINT ( 'NONE',  ( 1.806654366501771136, 0.000000000000000000, 2.499999999999998668 ) ) ;
#13783=CARTESIAN_POINT ( 'NONE',  ( 6.855582950365507244, 8.027210192628430718, -1.199719254218452047 ) ) ;
#13796=CARTESIAN_POINT ( 'NONE',  ( 4.954704567260191261, 7.963257648925383236, 1.029694947009308859 ) ) ;
#13798=CARTESIAN_POINT ( 'NONE',  ( 7.675324359112103423, 8.127168971818530707, 0.7216878364870267237 ) ) ;
#13806=CARTESIAN_POINT ( 'NONE',  ( -4.014095998097799267, 6.840806543492835345, -1.199719254218450271 ) ) ;
#13812=CARTESIAN_POINT ( 'NONE',  ( -5.600926855776877211, 9.548515408466085930, -0.7216878364870338292 ) ) ;
#13815=CARTESIAN_POINT ( 'NONE',  ( -4.864214080903581205, 4.879786425613829692, -0.6392378712632116322 ) ) ;
#13828=CARTESIAN_POINT ( 'NONE',  ( 6.481679955784983349, 9.719654494127929922, -1.199719254218452047 ) ) ;
#13844=ADVANCED_FACE ( 'NONE', ( #75335 ), #127777, .T. ) ;
#13850=CARTESIAN_POINT ( 'NONE',  ( -3.644109427023046521, 7.473487774827342278, 0.000000000000000000 ) ) ;
#13851=CARTESIAN_POINT ( 'NONE',  ( 5.494797395288433250, 9.632623737803665875, 0.000000000000000000 ) ) ;
#13853=CARTESIAN_POINT ( 'NONE',  ( -6.108552962726611746, 7.019250575032890183, 0.9758408306729206005 ) ) ;
#13859=CARTESIAN_POINT ( 'NONE',  ( 6.066347387471824781, 6.042103138330730872, -0.7998128361456481317 ) ) ;
#13869=CARTESIAN_POINT ( 'NONE',  ( -4.569915857295916872, 8.517381272593750552, -0.02673743978307913799 ) ) ;
#13870=CARTESIAN_POINT ( 'NONE',  ( 5.221298555038576872, 9.105615724271411082, 0.000000000000000000 ) ) ;
#13880=CARTESIAN_POINT ( 'NONE',  ( -4.828112100242279325, 8.646898193675708555, -0.7216878364870338292 ) ) ;
#13908=EDGE_LOOP ( 'NONE', ( #58646, #54612, #102300 ) ) ;
#13912=CARTESIAN_POINT ( 'NONE',  ( 6.703580607314123085, 6.785541894813420072, 0.000000000000000000 ) ) ;
#13915=CARTESIAN_POINT ( 'NONE',  ( 4.362691568547328202, 8.311833606605697256, -0.7998128361456381397 ) ) ;
#13926=CARTESIAN_POINT ( 'NONE',  ( -3.688700311369816909, 6.461178242310183784, -1.199719254218450271 ) ) ;
#13929=CARTESIAN_POINT ( 'NONE',  ( 5.519577934094861860, 6.572500690266394940, 1.082531754730549078 ) ) ;
#13942=CARTESIAN_POINT ( 'NONE',  ( -5.478903473698255588, 7.485416367438324059, -1.443375672974066548 ) ) ;
#13944=CARTESIAN_POINT ( 'NONE',  ( -3.960390268967665328, 6.674186842887300131, 1.082531754730549967 ) ) ;
#13945=CARTESIAN_POINT ( 'NONE',  ( 4.343210567687194157, 7.059472288894379055, 1.256205200019292256 ) ) ;
#13948=CARTESIAN_POINT ( 'NONE',  ( 0.000000000000000000, 8.499999999999996447, 0.000000000000000000 ) ) ;
#13955=DIRECTION ( 'NONE',  ( 0.6507913734559641616, 0.7592566023653004592, 0.000000000000000000 ) ) ;
#13970=CARTESIAN_POINT ( 'NONE',  ( -5.354544322754380303, 5.211666229493680191, 0.7998128361456281477 ) ) ;
#13981=CARTESIAN_POINT ( 'NONE',  ( -6.505933609711270549, 8.683618192786854095, -1.599625672291271394 ) ) ;
#13982=CARTESIAN_POINT ( 'NONE',  ( -4.607972389651186162, 8.469779238289159906, 0.3137405545926199579 ) ) ;
#13987=CARTESIAN_POINT ( 'NONE',  ( -6.224601922005509991, 10.27613631906616476, 0.7216878364870267237 ) ) ;
#13989=CARTESIAN_POINT ( 'NONE',  ( -3.630551273409382329, 7.457669928944732796, 0.7998128361456352531 ) ) ;
#13992=CARTESIAN_POINT ( 'NONE',  ( -4.655245641445871385, 6.524482229810530498, 1.599625672291263179 ) ) ;
#14002=CARTESIAN_POINT ( 'NONE',  ( 4.227110032410640095, 8.153655147779589996, 0.7998128361456271485 ) ) ;
#14014=CARTESIAN_POINT ( 'NONE',  ( 5.076602173674213070, 4.887400388900169368, 0.000000000000000000 ) ) ;
#14024=CARTESIAN_POINT ( 'NONE',  ( 5.180097208873055692, 8.201141289397330780, -1.199719254218450271 ) ) ;
#14025=CARTESIAN_POINT ( 'NONE',  ( 4.248501033035879004, 6.049946853332221153, -1.599625672291273171 ) ) ;
#14027=CARTESIAN_POINT ( 'NONE',  ( 5.252858170651868441, 5.093032385374103299, -0.7998128361456481317 ) ) ;
#14030=CARTESIAN_POINT ( 'NONE',  ( -6.265276382846530545, 6.482112999508623297, 0.000000000000000000 ) ) ;
#14039=CARTESIAN_POINT ( 'NONE',  ( 4.596911992430688265, 8.487755744900498556, -0.08351877912710949092 ) ) ;
#14040=CARTESIAN_POINT ( 'NONE',  ( -5.600926855776888758, 7.627776979863398310, -1.443375672974066548 ) ) ;
#14068=CARTESIAN_POINT ( 'NONE',  ( 4.258142763143749399, 7.125527769379820242, 1.199719254218451159 ) ) ;
#14086=CARTESIAN_POINT ( 'NONE',  ( -5.433785704026946384, 9.561443431331920095, 0.000000000000000000 ) ) ;
#14098=CARTESIAN_POINT ( 'NONE',  ( 5.285699784481295183, 7.260012063351913625, 1.599625672291268286 ) ) ;
#14102=CARTESIAN_POINT ( 'NONE',  ( 5.845500506147374153, 6.848780674373954547, 1.199719254218453823 ) ) ;
#14114=CARTESIAN_POINT ( 'NONE',  ( 4.763071791759735163, 8.170823326046956936, 0.7639991172946744014 ) ) ;
#14131=ORIENTED_EDGE ( 'NONE', *, *, #47472, .F. ) ;
#14135=CARTESIAN_POINT ( 'NONE',  ( -6.089547271193396227, 7.133501900260939443, -1.199719254218453823 ) ) ;
#14137=CARTESIAN_POINT ( 'NONE',  ( 5.712781623311797397, 7.758274208654143855, -1.599625672291283607 ) ) ;
#14141=CARTESIAN_POINT ( 'NONE',  ( -7.598418745816086783, 7.829519723065708092, 0.000000000000000000 ) ) ;
#14149=DIRECTION ( 'NONE',  ( 0.9446243521954068578, -4.336808689942003852E-14, 0.3281536732072456997 ) ) ;
#14150=CARTESIAN_POINT ( 'NONE',  ( -6.453559683527718249, 6.864596255245277057, -0.6992757447422948136 ) ) ;
#14158=AXIS2_PLACEMENT_3D ( 'NONE', #210268, #64036, #209194 ) ;
#14165=CARTESIAN_POINT ( 'NONE',  ( 5.560252395380206103, 8.540692657035327429, 1.082531754730547524 ) ) ;
#14181=CARTESIAN_POINT ( 'NONE',  ( -3.841022230581641050, 7.492630022202825479, -0.07115184559442505607 ) ) ;
#14182=CARTESIAN_POINT ( 'NONE',  ( -3.824808732831001201, 7.476377598362539345, 0.7216878364870338292 ) ) ;
#14185=CARTESIAN_POINT ( 'NONE',  ( 4.715203562502613188, 8.723097599553565118, 0.7998128361456341429 ) ) ;
#14230=CARTESIAN_POINT ( 'NONE',  ( 3.444653546323793947, 6.176457016423196222, 1.199719254218451159 ) ) ;
#14235=CARTESIAN_POINT ( 'NONE',  ( -4.299344108864953995, 7.069632989434141201, -1.082531754730551743 ) ) ;
#14237=FACE_OUTER_BOUND ( 'NONE', #7245, .T. ) ;
#14242=CARTESIAN_POINT ( 'NONE',  ( -4.762657100150483380, 8.778460060142702304, 0.000000000000000000 ) ) ;
#14254=CARTESIAN_POINT ( 'NONE',  ( -4.685224601974262271, 7.623789914682047808, -1.199719254218453823 ) ) ;
#14255=DIRECTION ( 'NONE',  ( 0.7592566023653003482, 0.6507913734559641616, 0.000000000000000000 ) ) ;
#14257=CARTESIAN_POINT ( 'NONE',  ( 5.869365784521903606, 7.282179437329668659, 1.264975801879052453 ) ) ;
#14260=AXIS2_PLACEMENT_3D ( 'NONE', #175846, #56744, #24217 ) ;
#14263=CARTESIAN_POINT ( 'NONE',  ( 5.936491157937257235, 8.019268665717216749, 1.599625672291268286 ) ) ;
#14267=ORIENTED_EDGE ( 'NONE', *, *, #72253, .T. ) ;
#14270=CARTESIAN_POINT ( 'NONE',  ( -4.118644803501354978, 8.027112380718707030, 0.7998128361456352531 ) ) ;
#14274=CARTESIAN_POINT ( 'NONE',  ( -3.786470039966538970, 7.639575156594750283, 0.000000000000000000 ) ) ;
#14278=CARTESIAN_POINT ( 'NONE',  ( 5.953438849732186178, 8.999410187112612647, -1.082531754730548412 ) ) ;
#14280=CARTESIAN_POINT ( 'NONE',  ( -6.468648687051513413, 7.679749902049126220, 1.082531754730549078 ) ) ;
#14286=CARTESIAN_POINT ( 'NONE',  ( 6.042093733545556233, 7.078139439671806699, -1.199719254218452047 ) ) ;
#14318=CARTESIAN_POINT ( 'NONE',  ( 4.735857411151594754, 8.202189375375613878, -0.7076125000919450958 ) ) ;
#14334=CARTESIAN_POINT ( 'NONE',  ( -6.165548087794384458, 6.979908488848794335, -0.9162763116292941268 ) ) ;
#14339=ORIENTED_EDGE ( 'NONE', *, *, #130004, .F. ) ;
#14343=CARTESIAN_POINT ( 'NONE',  ( -3.973948422136981407, 5.729635473950147606, -1.443375672974066548 ) ) ;
#14353=CARTESIAN_POINT ( 'NONE',  ( -4.573896719763875574, 6.429575154514868274, -1.599625672291271394 ) ) ;
#14364=CARTESIAN_POINT ( 'NONE',  ( 4.583538449871731757, 7.505156070562471804, 1.199719254218451159 ) ) ;
#14367=CARTESIAN_POINT ( 'NONE',  ( 5.872089928050205465, 6.023395468912922546, -0.7216878364870458196 ) ) ;
#14380=CARTESIAN_POINT ( 'NONE',  ( -4.664887371553763096, 7.600063145858131364, -1.199719254218453823 ) ) ;
#14381=CARTESIAN_POINT ( 'NONE',  ( 3.217027588192558074, 6.975225629525113824, -1.734723475976807094E-15 ) ) ;
#14393=CARTESIAN_POINT ( 'NONE',  ( -6.936931872047518155, 8.122117267924091166, 1.199719254218452047 ) ) ;
#14394=CARTESIAN_POINT ( 'NONE',  ( 4.857564175446106525, 8.889184981320973122, 0.7998128361456331437 ) ) ;
#14396=CARTESIAN_POINT ( 'NONE',  ( -4.450244736158147418, 7.987476157872628768, -2.500000000000000444 ) ) ;
#14397=ORIENTED_EDGE ( 'NONE', *, *, #185383, .T. ) ;
#14400=CARTESIAN_POINT ( 'NONE',  ( 4.634908411025333130, 6.500755460986618495, 1.599625672291268286 ) ) ;
#14409=CARTESIAN_POINT ( 'NONE',  ( -6.111218785694742195, 7.101581614182197022, 1.130138924470771800 ) ) ;
#14418=CARTESIAN_POINT ( 'NONE',  ( -3.648552735408990166, 6.310376387068841630, -1.082531754730546636 ) ) ;
#14468=CARTESIAN_POINT ( 'NONE',  ( 5.011674058906918638, 5.875983152593414971, 1.199719254218452047 ) ) ;
#14469=CARTESIAN_POINT ( 'NONE',  ( -4.828112100242294424, 5.765790550771681566, -1.082531754730549967 ) ) ;
#14498=CARTESIAN_POINT ( 'NONE',  ( -5.655686355556086120, 6.627330832017406692, 1.199719254218452935 ) ) ;
#14500=CARTESIAN_POINT ( 'NONE',  ( 5.790741006368192778, 8.809596036521288198, -1.082531754730548412 ) ) ;
#14506=CARTESIAN_POINT ( 'NONE',  ( -4.471156797456668386, 8.438376373666578445, -0.7998128361456362523 ) ) ;
#14511=CARTESIAN_POINT ( 'NONE',  ( -5.309953438407606363, 6.223975762010839574, 1.199719254218452935 ) ) ;
#14516=CARTESIAN_POINT ( 'NONE',  ( -5.611095471209320174, 7.639640364534566075, 1.599625672291263179 ) ) ;
#14527=CARTESIAN_POINT ( 'NONE',  ( -4.878955176071358757, 6.785476686873604280, -1.599625672291271394 ) ) ;
#14530=CARTESIAN_POINT ( 'NONE',  ( -5.587368702607575344, 8.572328348800551723, 1.082531754730550855 ) ) ;
#14531=CARTESIAN_POINT ( 'NONE',  ( -6.034787771414192648, 9.094317262408276648, 1.082531754730549967 ) ) ;
#14532=CARTESIAN_POINT ( 'NONE',  ( 7.550965208168244125, 7.774157262476569130, -0.7998128361456341429 ) ) ;
#14533=CARTESIAN_POINT ( 'NONE',  ( -7.618755976236585958, 7.853246491889623648, 0.000000000000000000 ) ) ;
#14560=CIRCLE ( 'NONE', #190976, 4.583333333333340143 ) ;
#14574=CARTESIAN_POINT ( 'NONE',  ( 6.485343392949857844, 6.752073445700102816, -0.1478272009810890908 ) ) ;
#14592=CARTESIAN_POINT ( 'NONE',  ( -3.657667580636712934, 7.489305620709952649, -0.7998128361456481317 ) ) ;
#14605=CARTESIAN_POINT ( 'NONE',  ( 5.761288931164342486, 5.686201605971993978, -0.7998128361456481317 ) ) ;
#14608=CARTESIAN_POINT ( 'NONE',  ( 6.668631453075247073, 8.873432343378178544, -1.599625672291281386 ) ) ;
#14609=CARTESIAN_POINT ( 'NONE',  ( 0.3255492091119998599, 2.641190174458327711, -1.974278555462047668 ) ) ;
#14616=CARTESIAN_POINT ( 'NONE',  ( 3.061108821635398769, 6.793320401875094561, -0.7998128361456362523 ) ) ;
#14622=CARTESIAN_POINT ( 'NONE',  ( 6.547661840756936691, 6.603636667163397256, 0.7998128361456352531 ) ) ;
#14636=CARTESIAN_POINT ( 'NONE',  ( -4.340018570150306232, 8.077455741901736985, -0.7216878364870338292 ) ) ;
#14637=CARTESIAN_POINT ( 'NONE',  ( 5.072158865288233009, 7.010880990960010273, 1.443375672974065660 ) ) ;
#14649=CARTESIAN_POINT ( 'NONE',  ( -4.981695098378565945, 4.776675467721892332, -0.7998128361456362523 ) ) ;
#14650=CARTESIAN_POINT ( 'NONE',  ( -7.783789588021474692, 8.253711738879413673, 0.7216878364870317197 ) ) ;
#14651=CARTESIAN_POINT ( 'NONE',  ( 7.526711554241970248, 8.810193563817646734, -1.199719254218452047 ) ) ;
#14654=CARTESIAN_POINT ( 'NONE',  ( 5.682275777458851707, 6.762314840857718501, 1.082531754730549078 ) ) ;
#14671=CARTESIAN_POINT ( 'NONE',  ( 5.061990249855835344, 6.999017606288844284, -1.599625672291273171 ) ) ;
#14673=CARTESIAN_POINT ( 'NONE',  ( -3.871735385154307263, 6.674719161725423788, -1.199719254218450271 ) ) ;
#14685=CARTESIAN_POINT ( 'NONE',  ( 5.533136088152891929, 9.469426179571447832, -0.7216878364870458196 ) ) ;
#14687=CARTESIAN_POINT ( 'NONE',  ( -5.121948170912633991, 9.197632976031879792, -0.7998128361456362523 ) ) ;
#14688=CARTESIAN_POINT ( 'NONE',  ( 5.285699784481295183, 7.260012063351913625, 1.599625672291268286 ) ) ;
#14698=CARTESIAN_POINT ( 'NONE',  ( -5.936491157937300756, 8.019268665717216749, 1.599625672291263179 ) ) ;
#14701=CARTESIAN_POINT ( 'NONE',  ( -0.4000000000000113465, 3.017365524286432787, 2.023857702507793288 ) ) ;
#14726=EDGE_CURVE ( 'NONE', #169159, #113990, #436, .T. ) ;
#14727=CARTESIAN_POINT ( 'NONE',  ( 5.560252395380215873, 6.619954228432645138, 1.082531754730549078 ) ) ;
#14733=CARTESIAN_POINT ( 'NONE',  ( 6.007671464186837618, 6.181573927739029806, 0.7216878364870328300 ) ) ;
#14746=CARTESIAN_POINT ( 'NONE',  ( -4.620296487206990932, 8.612372678375294299, 0.000000000000000000 ) ) ;
#14748=CARTESIAN_POINT ( 'NONE',  ( -5.237192476628793614, 9.332084666034067055, 0.7998128361456291469 ) ) ;
#14756=CARTESIAN_POINT ( 'NONE',  ( 4.055297343818933697, 5.824542549245813383, 1.443375672974058777 ) ) ;
#14761=DIRECTION ( 'NONE',  ( 0.000000000000000000, 0.000000000000000000, -1.000000000000000000 ) ) ;
#14762=CARTESIAN_POINT ( 'NONE',  ( -4.450819567036169211, 8.414649604842665553, -0.7998128361456362523 ) ) ;
#14768=CARTESIAN_POINT ( 'NONE',  ( -4.177320726786315497, 7.887641591310407208, -0.7216878364870458196 ) ) ;
#14771=CARTESIAN_POINT ( 'NONE',  ( -6.286140498591554326, 7.362860665558790707, 1.199719254218452047 ) ) ;
#14777=CARTESIAN_POINT ( 'NONE',  ( -4.407809337774280856, 7.196175756495025055, 1.082531754730549967 ) ) ;
#14790=ORIENTED_EDGE ( 'NONE', *, *, #64546, .T. ) ;
#14791=CARTESIAN_POINT ( 'NONE',  ( -3.323157048681004699, 6.891117300187535655, -0.7216878364870458196 ) ) ;
#14792=CARTESIAN_POINT ( 'NONE',  ( 5.408776937209000657, 5.274937613024121674, 0.7998128361456352531 ) ) ;
#14793=CARTESIAN_POINT ( 'NONE',  ( -4.956387674247580755, 7.940146832334256111, 1.199719254218452935 ) ) ;
#14817=CARTESIAN_POINT ( 'NONE',  ( -5.745623237141265882, 9.925253886631958622, 0.7998128361456291469 ) ) ;
#14842=CARTESIAN_POINT ( 'NONE',  ( 7.842465510862060896, 8.114240948952696542, 0.000000000000000000 ) ) ;
#14843=CARTESIAN_POINT ( 'NONE',  ( 4.524302555594479358, 8.500379758160722332, 0.3357913727640315371 ) ) ;
#14849=CARTESIAN_POINT ( 'NONE',  ( 3.179715765502657554, 5.975770656120749535, -2.500000000000002220 ) ) ;
#14854=CARTESIAN_POINT ( 'NONE',  ( 5.886377668569586774, 7.162856863344262415, 1.137212067324339104 ) ) ;
#14856=CARTESIAN_POINT ( 'NONE',  ( 4.577813143269636065, 5.369812084349879555, -1.199719254218450271 ) ) ;
#14863=CARTESIAN_POINT ( 'NONE',  ( -6.448838341955544173, 7.552674816150118708, 1.199719254218452047 ) ) ;
#14868=CARTESIAN_POINT ( 'NONE',  ( -7.892254816486440561, 8.380254505421877553, 0.000000000000000000 ) ) ;
#14875=CARTESIAN_POINT ( 'NONE',  ( -4.984557751679625781, 5.844347460828191565, 1.199719254218452935 ) ) ;
#14885=CARTESIAN_POINT ( 'NONE',  ( 3.250922972226694352, 7.014770244231638863, 0.7998128361456281477 ) ) ;
#14917=CARTESIAN_POINT ( 'NONE',  ( 4.878955176071345434, 6.785476686873604280, -1.599625672291269396 ) ) ;
#14926=CARTESIAN_POINT ( 'NONE',  ( 5.885648082108188461, 8.920320958217979879, 1.082531754730549967 ) ) ;
#14937=EDGE_CURVE ( 'NONE', #15686, #155820, #116760, .T. ) ;
#14938=CARTESIAN_POINT ( 'NONE',  ( -5.289089323106922258, 9.184704953684462936, 0.7216878364870267237 ) ) ;
#14971=CARTESIAN_POINT ( 'NONE',  ( 4.206772801990143584, 8.129928378955675328, 0.7998128361456271485 ) ) ;
#14973=CARTESIAN_POINT ( 'NONE',  ( 6.723917837734620484, 6.809268663637336516, 0.000000000000000000 ) ) ;
#14987=CARTESIAN_POINT ( 'NONE',  ( -5.953438850176548947, 9.959779401932374654, 0.000000000000000000 ) ) ;
#14990=CARTESIAN_POINT ( 'NONE',  ( 6.170369307550831017, 6.371388078330353366, 0.7216878364870328300 ) ) ;
#15005=CARTESIAN_POINT ( 'NONE',  ( -5.885648082108231982, 7.959951743916638733, 1.443375672974058777 ) ) ;
#15007=CARTESIAN_POINT ( 'NONE',  ( -3.987506576194992824, 7.666191748953863794, 0.7216878364870338292 ) ) ;
#15008=CARTESIAN_POINT ( 'NONE',  ( 4.207966135563057541, 7.175396087857926375, 1.156120096431498379 ) ) ;
#15013=CARTESIAN_POINT ( 'NONE',  ( -5.616896113772630983, 5.725669352255732036, 0.1283408312532021145 ) ) ;
#15014=DIRECTION ( 'NONE',  ( -1.000000000000000000, 0.000000000000000000, 0.000000000000000000 ) ) ;
#15017=CARTESIAN_POINT ( 'NONE',  ( -6.172557777799569934, 6.616364562750757905, -0.6295236542525488588 ) ) ;
#15025=CARTESIAN_POINT ( 'NONE',  ( -4.995253251992230581, 4.792493313604505367, 0.000000000000000000 ) ) ;
#15036=CARTESIAN_POINT ( 'NONE',  ( -5.327428015527048366, 5.180030537728460338, -0.7998128361456362523 ) ) ;
#15037=CARTESIAN_POINT ( 'NONE',  ( -5.608665566507964328, 5.643324313368172973, -0.3498717110727275204 ) ) ;
#15046=CARTESIAN_POINT ( 'NONE',  ( -5.738844160334429567, 9.917344963690652548, 0.000000000000000000 ) ) ;
#15047=CARTESIAN_POINT ( 'NONE',  ( -5.012442140716328431, 8.020463026761962766, 1.150573971286508845 ) ) ;
#15061=CARTESIAN_POINT ( 'NONE',  ( -0.4000000000000243916, 2.999999999999999112, 7.500000000000000000 ) ) ;
#15068=CARTESIAN_POINT ( 'NONE',  ( 6.821687566331318564, 7.987665577921906568, 1.199719254218452935 ) ) ;
#15077=AXIS2_PLACEMENT_3D ( 'NONE', #208116, #207052, #92286 ) ;
#15096=CARTESIAN_POINT ( 'NONE',  ( 6.042093733545556233, 7.078139439671806699, -1.199719254218452047 ) ) ;
#15097=CARTESIAN_POINT ( 'NONE',  ( 3.888156192069020634, 7.758209000714329839, 1.040834085586084257E-14 ) ) ;
#15099=CARTESIAN_POINT ( 'NONE',  ( 3.230585741806197841, 6.991043475407723307, 0.7998128361456271485 ) ) ;
#15111=CARTESIAN_POINT ( 'NONE',  ( 4.966250736084032447, 8.070317005903060448, 1.090833899539983554 ) ) ;
#15112=CARTESIAN_POINT ( 'NONE',  ( -6.089020385868876062, 6.276481003034692030, -0.7216878364870338292 ) ) ;
#15132=CARTESIAN_POINT ( 'NONE',  ( -4.327420530893566486, 8.660440186815751673, 0.7750000000000001332 ) ) ;
#15138=CARTESIAN_POINT ( 'NONE',  ( 5.879395890181562834, 6.888325289080478697, -1.199719254218452047 ) ) ;
#15142=CARTESIAN_POINT ( 'NONE',  ( 3.627688620108284745, 6.389997935838436227, 1.199719254218452047 ) ) ;
#15172=CARTESIAN_POINT ( 'NONE',  ( 4.355912491740495440, 8.303924683664389406, 0.000000000000000000 ) ) ;
#15176=CARTESIAN_POINT ( 'NONE',  ( 4.864343252252968597, 8.897093904262280972, 0.000000000000000000 ) ) ;
#15186=CARTESIAN_POINT ( 'NONE',  ( 4.720979226589129496, 8.219560628541461966, -0.6735110442024627719 ) ) ;
#15194=CARTESIAN_POINT ( 'NONE',  ( 5.072158865288234786, 7.010880990960011161, 1.443375672974065660 ) ) ;
#15201=CARTESIAN_POINT ( 'NONE',  ( -6.019103170659795943, 7.082126295680237327, 1.053690733614056851 ) ) ;
#15204=CARTESIAN_POINT ( 'NONE',  ( 3.445180431648323882, 6.073108699348104267, 1.082531754730549078 ) ) ;
#15205=ORIENTED_EDGE ( 'NONE', *, *, #188735, .F. ) ;
#15209=CARTESIAN_POINT ( 'NONE',  ( -7.767895665986912057, 8.027242796598338614, -0.7998128361456362523 ) ) ;
#15211=CARTESIAN_POINT ( 'NONE',  ( 5.306037014901791693, 7.283738832175834510, 1.599625672291269396 ) ) ;
#15213=CARTESIAN_POINT ( 'NONE',  ( 3.753485299433081845, 7.393166926064984601, -0.1880404715405732952 ) ) ;
#15216=CARTESIAN_POINT ( 'NONE',  ( -6.237633190739009237, 9.434933268240943249, 1.199719254218452047 ) ) ;
#15223=CARTESIAN_POINT ( 'NONE',  ( -0.1966775781082229224, 3.362145428329805341, -1.992912547350113028 ) ) ;
#15235=CARTESIAN_POINT ( 'NONE',  ( 2.723338755101574638, 3.009222805659324429, 2.500000000000000444 ) ) ;
#15237=ORIENTED_EDGE ( 'NONE', *, *, #11046, .F. ) ;
#15240=CARTESIAN_POINT ( 'NONE',  ( 5.234856708652215751, 9.121433570154021453, 0.7216878364870317197 ) ) ;
#15252=( BOUNDED_CURVE ( )  B_SPLINE_CURVE ( 2, ( #55862, #74258, #107888, #41776, #125217 ),
 .UNSPECIFIED., .F., .T. ) 
 B_SPLINE_CURVE_WITH_KNOTS ( ( 3, 2, 3 ),
 ( 0.04938056888445840203, 0.05000000000000000278, 0.05032235610909231716 ),
 .UNSPECIFIED. ) 
 CURVE ( )  GEOMETRIC_REPRESENTATION_ITEM ( )  RATIONAL_B_SPLINE_CURVE ( ( 0.9815633466012652075, 0.9900414359694351685, 1.000000000000000000, 0.9948174964536085074, 0.9900359397100743086 ) ) 
 REPRESENTATION_ITEM ( '' )  );
#15255=CARTESIAN_POINT ( 'NONE',  ( -3.854349547643701968, 7.486297264622638004, -0.2033521147656738026 ) ) ;
#15256=CARTESIAN_POINT ( 'NONE',  ( -4.502716413514301408, 7.306900678191715848, -1.082531754730549967 ) ) ;
#15258=CARTESIAN_POINT ( 'NONE',  ( 4.389807875774629942, 8.343469298370917997, 0.7998128361456271485 ) ) ;
#15271=ORIENTED_EDGE ( 'NONE', *, *, #181468, .F. ) ;
#15304=CARTESIAN_POINT ( 'NONE',  ( 5.011674058906918638, 5.875983152593414971, 1.199719254218452047 ) ) ;
#15309=CARTESIAN_POINT ( 'NONE',  ( -5.031484404002922517, 6.963427452793760963, 1.443375672974058777 ) ) ;
#15314=EDGE_CURVE ( 'NONE', #120691, #118760, #204537, .T. ) ;
#15316=CARTESIAN_POINT ( 'NONE',  ( -4.599959256786493533, 8.588645909551377855, 0.000000000000000000 ) ) ;
#15322=CARTESIAN_POINT ( 'NONE',  ( 5.996449078994045223, 10.21788403546024782, 0.7998128361456331437 ) ) ;
#15323=CARTESIAN_POINT ( 'NONE',  ( -4.945692173934974178, 8.992000979557944973, 0.000000000000000000 ) ) ;
#15324=CARTESIAN_POINT ( 'NONE',  ( -3.147653791585727667, 8.920000000000001705, 2.499999999999999556 ) ) ;
#15326=CARTESIAN_POINT ( 'NONE',  ( 6.059925523928845870, 7.140772946495586915, 1.155538509043469997 ) ) ;
#15331=CARTESIAN_POINT ( 'NONE',  ( 5.879395890181562834, 6.888325289080478697, -1.199719254218452047 ) ) ;
#15340=CARTESIAN_POINT ( 'NONE',  ( -3.871735385154307263, 6.674719161725423788, -1.199719254218450271 ) ) ;
#15344=CARTESIAN_POINT ( 'NONE',  ( -6.611536185319534908, 7.742488966741438716, 1.199719254218452047 ) ) ;
#15348=CARTESIAN_POINT ( 'NONE',  ( 6.333067150914816423, 7.521571443223021625, 1.082531754730549967 ) ) ;
#15350=CARTESIAN_POINT ( 'NONE',  ( -7.065207446052809814, 9.336104335185325453, -1.443375672974066548 ) ) ;
#15357=CARTESIAN_POINT ( 'NONE',  ( 4.420840606507738357, 7.315341919971147355, 1.199719254218451159 ) ) ;
#15358=ORIENTED_EDGE ( 'NONE', *, *, #50859, .F. ) ;
#15385=CARTESIAN_POINT ( 'NONE',  ( 4.713861384769566953, 8.227931952640012980, -0.6562286284988675389 ) ) ;
#15400=CARTESIAN_POINT ( 'NONE',  ( -4.969355510774519757, 7.965585441469681172, -1.036248007939699178 ) ) ;
#15419=CARTESIAN_POINT ( 'NONE',  ( -4.004454267989906668, 5.765225627445230927, 1.599625672291270506 ) ) ;
#15421=CARTESIAN_POINT ( 'NONE',  ( 6.556249800660121529, 9.806652646482286073, 1.199719254218452047 ) ) ;
#15432=CARTESIAN_POINT ( 'NONE',  ( 6.215487077222150880, 6.216099443039444949, 0.000000000000000000 ) ) ;
#15435=CARTESIAN_POINT ( 'NONE',  ( 5.329763783503544516, 9.232158490813878515, -0.7216878364870458196 ) ) ;
#15447=CARTESIAN_POINT ( 'NONE',  ( -6.635789839245807897, 6.706452665400368218, 0.7998128361456341429 ) ) ;
#15449=CARTESIAN_POINT ( 'NONE',  ( 5.239300017038202917, 5.077214539491492928, 0.000000000000000000 ) ) ;
#15460=CARTESIAN_POINT ( 'NONE',  ( -7.096767062110449942, 7.244259425409119046, -0.7998128361456362523 ) ) ;
#15461=CARTESIAN_POINT ( 'NONE',  ( 7.503511670520385479, 7.718794801887437274, 0.7998128361456281477 ) ) ;
#15463=PLANE ( 'NONE',  #52674 ) ;
#15466=CARTESIAN_POINT ( 'NONE',  ( 4.821333023213275837, 4.797512413269824805, 0.000000000000000000 ) ) ;
#15467=ORIENTED_EDGE ( 'NONE', *, *, #83083, .F. ) ;
#15468=CARTESIAN_POINT ( 'NONE',  ( 5.225741863424510747, 5.061396693608882558, 0.7998128361456352531 ) ) ;
#15471=CARTESIAN_POINT ( 'NONE',  ( -0.4461809497497640775, 3.122791860410086606, 1.949595486268987043 ) ) ;
#15475=CARTESIAN_POINT ( 'NONE',  ( -5.971735067414164710, 7.203215006737162085, 1.225879040106806706 ) ) ;
#15483=CARTESIAN_POINT ( 'NONE',  ( -5.908321080505254841, 10.11506803722328129, 0.7998128361456291469 ) ) ;
#15484=CARTESIAN_POINT ( 'NONE',  ( -6.851666526859749418, 9.086973262793417661, -1.599625672291271394 ) ) ;
#15493=CARTESIAN_POINT ( 'NONE',  ( -4.791166081694341550, 4.882818525799564213, 0.4357780244859492669 ) ) ;
#15507=LINE ( 'NONE', #200650, #154304 ) ;
#15512=EDGE_CURVE ( 'NONE', #109831, #113379, #22916, .T. ) ;
#15534=CARTESIAN_POINT ( 'NONE',  ( 6.048345925472166762, 10.07050432311064903, 0.7216878364870317197 ) ) ;
#15535=CARTESIAN_POINT ( 'NONE',  ( -3.634994582239682526, 6.294558541704648569, 1.082531754730549967 ) ) ;
#15560=CARTESIAN_POINT ( 'NONE',  ( -3.983063267364693960, 7.868933921892603323, -0.7998128361456481317 ) ) ;
#15562=CARTESIAN_POINT ( 'NONE',  ( 5.519577934094851202, 8.493239118869080784, 1.082531754730547524 ) ) ;
#15567=CARTESIAN_POINT ( 'NONE',  ( -5.257529707049291900, 9.355811434857983500, 0.7998128361456291469 ) ) ;
#15576=CARTESIAN_POINT ( 'NONE',  ( -4.288121723672178476, 8.224835454251337552, -0.7998128361456362523 ) ) ;
#15588=CARTESIAN_POINT ( 'NONE',  ( -5.798046968499580345, 6.793418213784815585, 1.199719254218452935 ) ) ;
#15592=CARTESIAN_POINT ( 'NONE',  ( -7.770231434407805615, 8.237893892996801526, 0.000000000000000000 ) ) ;
#15594=CARTESIAN_POINT ( 'NONE',  ( -6.658462837642833421, 8.861568958707010779, 1.443375672974064550 ) ) ;
#15595=CARTESIAN_POINT ( 'NONE',  ( 5.664274315459256748, 9.830346811336296398, -0.7998128361456481317 ) ) ;
#15597=CARTESIAN_POINT ( 'NONE',  ( -5.289089322662584358, 5.343228095960675716, 0.000000000000000000 ) ) ;
#15618=CARTESIAN_POINT ( 'NONE',  ( 6.435676556713933572, 6.878741676577107889, -0.7109887800627444632 ) ) ;
#15629=B_SPLINE_CURVE_WITH_KNOTS ( 'NONE', 3,
 ( #85970, #152045, #153105, #120684, #50276, #37217, #88108 ),
 .UNSPECIFIED., .F., .F.,
 ( 4, 3, 4 ),
 ( 0.000000000000000000, 3.012973846129562487E-05, 4.150524011425761568E-05 ),
 .UNSPECIFIED. ) ;
#15639=CARTESIAN_POINT ( 'NONE',  ( 6.463930056324285189, 6.765849701160138174, -0.2895399612845122039 ) ) ;
#15654=CARTESIAN_POINT ( 'NONE',  ( 7.201315867513990554, 8.430565262634994284, -1.199719254218452047 ) ) ;
#15657=CARTESIAN_POINT ( 'NONE',  ( -5.601453741101424022, 6.564059448486966986, -1.199719254218453823 ) ) ;
#15661=CARTESIAN_POINT ( 'NONE',  ( -8.068510813464099485, 8.585886501895810596, 0.7216878364870317197 ) ) ;
#15671=CARTESIAN_POINT ( 'NONE',  ( 5.747730777550676073, 5.670383760089384495, 0.000000000000000000 ) ) ;
#15673=CARTESIAN_POINT ( 'NONE',  ( 6.587282531393223728, 8.778525268082516320, 1.599625672291268286 ) ) ;
#15680=CARTESIAN_POINT ( 'NONE',  ( -6.929625909916163451, 7.257187447756535903, 0.7216878364870317197 ) ) ;
#15686=VERTEX_POINT ( 'NONE', #143613 ) ;
#15687=CARTESIAN_POINT ( 'NONE',  ( 6.393551957296131683, 9.616838495890963401, 1.199719254218452047 ) ) ;
#15701=CARTESIAN_POINT ( 'NONE',  ( -4.814553946628611136, 8.631080347793099961, 0.000000000000000000 ) ) ;
#15702=CARTESIAN_POINT ( 'NONE',  ( 3.919715808126649659, 7.587102519540811940, 0.000000000000000000 ) ) ;
#15710=EDGE_CURVE ( 'NONE', #156724, #37959, #96025, .T. ) ;
#15714=CARTESIAN_POINT ( 'NONE',  ( -7.431277594066160397, 7.842447745931541370, -0.7216878364870338292 ) ) ;
#15719=CARTESIAN_POINT ( 'NONE',  ( 4.028181036591620412, 7.713645286083276709, -0.7216878364870338292 ) ) ;
#15736=CARTESIAN_POINT ( 'NONE',  ( -3.467853430045390706, 7.267855778353407459, 0.7998128361456352531 ) ) ;
#15749=CARTESIAN_POINT ( 'NONE',  ( 4.095444919779759552, 6.935713618788495793, 1.199719254218451159 ) ) ;
#15751=CARTESIAN_POINT ( 'NONE',  ( -7.306918443122272677, 7.489436036589583345, 0.7998128361456341429 ) ) ;
#15752=CARTESIAN_POINT ( 'NONE',  ( 4.694866332082116678, 8.699370830729650450, 0.7998128361456341429 ) ) ;
#15760=CARTESIAN_POINT ( 'NONE',  ( -6.017840079619296567, 8.114175741012878973, -1.599625672291271394 ) ) ;
#15763=DIRECTION ( 'NONE',  ( -0.6507913734559650498, -0.7592566023652995710, 0.000000000000000000 ) ) ;
#15783=CARTESIAN_POINT ( 'NONE',  ( -1.843739406749240750, 9.999999999999998224, 0.7750000000000013545 ) ) ;
#15787=CARTESIAN_POINT ( 'NONE',  ( 3.933273961740286317, 7.602920365423422311, 0.7216878364870257245 ) ) ;
#15793=CARTESIAN_POINT ( 'NONE',  ( 4.055297343818931033, 6.784911763547157193, 1.082531754730549078 ) ) ;
#15805=CARTESIAN_POINT ( 'NONE',  ( -5.444481204339554736, 8.509589284108232121, 1.199719254218454489 ) ) ;
#15807=CARTESIAN_POINT ( 'NONE',  ( -7.422162748838431412, 7.623887726591770608, -0.7998128361456362523 ) ) ;
#15814=CARTESIAN_POINT ( 'NONE',  ( 6.851666526859736983, 9.086973262793417661, -1.599625672291269396 ) ) ;
#15820=CARTESIAN_POINT ( 'NONE',  ( -5.752402313948099533, 9.933162809573264695, -0.7998128361456362523 ) ) ;
#15826=CARTESIAN_POINT ( 'NONE',  ( -5.966997003790232235, 7.094489604910957148, -1.082531754730549967 ) ) ;
#15829=CARTESIAN_POINT ( 'NONE',  ( -5.586841817283045408, 8.675676665875643678, 1.199719254218454489 ) ) ;
#15852=CARTESIAN_POINT ( 'NONE',  ( -7.282664789195997912, 8.525472337930658284, 1.199719254218452047 ) ) ;
#15853=CARTESIAN_POINT ( 'NONE',  ( 3.250922972226694352, 7.014770244231638863, 0.7998128361456281477 ) ) ;
#15854=CARTESIAN_POINT ( 'NONE',  ( -6.981522756394290319, 7.109807735406931783, 0.7998128361456341429 ) ) ;
#15868=CARTESIAN_POINT ( 'NONE',  ( -0.4000000000000243916, 2.999999999999999112, 7.500000000000000000 ) ) ;
#15878=CARTESIAN_POINT ( 'NONE',  ( -7.456058132872594335, 7.663432341298296535, 0.000000000000000000 ) ) ;
#15906=CARTESIAN_POINT ( 'NONE',  ( 5.259637247458703868, 5.100941308315409373, 0.000000000000000000 ) ) ;
#15911=ADVANCED_FACE ( 'NONE', ( #119659 ), #118589, .F. ) ;
#15919=CARTESIAN_POINT ( 'NONE',  ( 4.739057715201537846, 8.198473722472776615, 0.7146191656044629248 ) ) ;
#15921=CARTESIAN_POINT ( 'NONE',  ( 5.090160327287878594, 4.903218234782778850, -0.7998128361456481317 ) ) ;
#15926=CARTESIAN_POINT ( 'NONE',  ( -6.394605727500880299, 7.489403432619674561, -1.199719254218452047 ) ) ;
#15932=CARTESIAN_POINT ( 'NONE',  ( -6.956742217143487395, 8.249192353823097790, 1.082531754730549078 ) ) ;
#15940=CARTESIAN_POINT ( 'NONE',  ( -4.111865726694519552, 8.019203457777400956, 0.000000000000000000 ) ) ;
#15949=CARTESIAN_POINT ( 'NONE',  ( -6.622231685632140596, 6.690634819517756959, 0.000000000000000000 ) ) ;
#15951=CARTESIAN_POINT ( 'NONE',  ( 4.899292406491845497, 6.809203455697518947, -1.599625672291273171 ) ) ;
#15955=ORIENTED_EDGE ( 'NONE', *, *, #137980, .F. ) ;
#15971=CARTESIAN_POINT ( 'NONE',  ( -6.563028877466991595, 9.814561569423593923, 1.199719254218452935 ) ) ;
#15981=CARTESIAN_POINT ( 'NONE',  ( 5.017399365509065845, 8.011327138806002779, -1.199719254218450271 ) ) ;
#15982=CYLINDRICAL_SURFACE ( 'NONE', #108234, 0.7500000000000011102 ) ;
#15988=CARTESIAN_POINT ( 'NONE',  ( 6.048345925472191631, 6.229027465905275562, 0.7216878364870328300 ) ) ;
#15991=CARTESIAN_POINT ( 'NONE',  ( 5.383996398402570271, 9.295429874862735531, 0.000000000000000000 ) ) ;
#16002=CARTESIAN_POINT ( 'NONE',  ( -7.431277594066160397, 7.842447745931541370, -0.7216878364870338292 ) ) ;
#16039=CARTESIAN_POINT ( 'NONE',  ( 6.540882763950133238, 6.595727744222092959, 0.000000000000000000 ) ) ;
#16041=CARTESIAN_POINT ( 'NONE',  ( 5.794130544993763898, 7.853181283949808744, 1.599625672291269396 ) ) ;
#16053=CARTESIAN_POINT ( 'NONE',  ( -5.171509248969888617, 4.998125310078441075, 0.7998128361456281477 ) ) ;
#16056=CARTESIAN_POINT ( 'NONE',  ( 5.275531169048895741, 7.248148678680751189, -1.443375672974078761 ) ) ;
#16063=CARTESIAN_POINT ( 'NONE',  ( -3.851398154733808088, 6.650992392901508232, -1.199719254218450271 ) ) ;
#16069=CARTESIAN_POINT ( 'NONE',  ( -6.129694847154211423, 9.205042184104968328, -1.082531754730549967 ) ) ;
#16071=CARTESIAN_POINT ( 'NONE',  ( -5.234856708652269042, 7.200695141551334721, 1.443375672974058777 ) ) ;
#16087=CARTESIAN_POINT ( 'NONE',  ( -3.149236820124241110, 6.896136400112061970, -0.7998128361456481317 ) ) ;
#16099=CARTESIAN_POINT ( 'NONE',  ( -3.657667580636712934, 7.489305620709952649, -0.7998128361456481317 ) ) ;
#16108=CARTESIAN_POINT ( 'NONE',  ( -8.086512275908061653, 8.398962174839683215, 0.000000000000000000 ) ) ;
#16109=CARTESIAN_POINT ( 'NONE',  ( -5.072456052330698739, 7.961014115122230450, -1.198640345919316674 ) ) ;
#16128=CARTESIAN_POINT ( 'NONE',  ( 5.956828388357757298, 8.042995434541133193, 1.599625672291269396 ) ) ;
#16133=CARTESIAN_POINT ( 'NONE',  ( -6.143440778383317813, 6.339971461045375456, 7.509178883279419847E-06 ) ) ;
#16151=CARTESIAN_POINT ( 'NONE',  ( 6.047819040147648373, 9.213483425884394507, 1.199719254218452047 ) ) ;
#16152=CARTESIAN_POINT ( 'NONE',  ( 5.200434439293556643, 8.224868058221247225, -1.199719254218452047 ) ) ;
#16154=CARTESIAN_POINT ( 'NONE',  ( 4.553559489343365740, 6.405848385690952718, -1.599625672291269396 ) ) ;
#16166=CARTESIAN_POINT ( 'NONE',  ( 5.213898493288036562, 7.712005038449616379, -1.200564631081424416 ) ) ;
#16167=CARTESIAN_POINT ( 'NONE',  ( -5.356880090730904875, 7.343055753976412525, 1.443375672974058777 ) ) ;
#16168=CARTESIAN_POINT ( 'NONE',  ( 4.963693636378940788, 5.923969009597785274, -1.082531754730548412 ) ) ;
#16183=AXIS2_PLACEMENT_3D ( 'NONE', #190347, #194622, #77675 ) ;
#16187=CARTESIAN_POINT ( 'NONE',  ( -4.517335436343488553, 8.499999999999996447, 0.7749999999999996891 ) ) ;
#16190=EDGE_CURVE ( 'NONE', #161612, #60255, #19521, .T. ) ;
#16195=CARTESIAN_POINT ( 'NONE',  ( 5.228604516725597229, 6.129068686715179126, -1.199719254218450271 ) ) ;
#16197=CARTESIAN_POINT ( 'NONE',  ( 3.736153849017632922, 6.516540702899320081, -1.199719254218453823 ) ) ;
#16225=CARTESIAN_POINT ( 'NONE',  ( 6.042093733545556233, 7.078139439671806699, -1.199719254218452047 ) ) ;
#16229=CARTESIAN_POINT ( 'NONE',  ( -6.486760921661624657, 6.767311426390788753, 0.2083394120615672529 ) ) ;
#16230=CARTESIAN_POINT ( 'NONE',  ( 4.712340909201580885, 7.655425606447271214, -1.199719254218452047 ) ) ;
#16240=CARTESIAN_POINT ( 'NONE',  ( -1.844607821789273627, 8.931289555339859021, 0.7750000000000013545 ) ) ;
#16241=CARTESIAN_POINT ( 'NONE',  ( 4.743613802917549194, 8.193193991156523026, -0.7244234545457691743 ) ) ;
#16258=( BOUNDED_SURFACE ( )  B_SPLINE_SURFACE ( 1, 2, ( 
 ( #117421, #66437, #132579, #118489, #103245, #202844, #1439, #199650, #183418, #35021, #86986, #119553, #120637, #167179, #38241, #18768, #153057, #150942, #2505, #52360, #7855, #190872, #154130, #138961, #8931, #59822, #41466, #42538, #123852, #89144, #5700, #155198, #108641, #187678, #9996, #56628, #172520, #203912, #107575, #173609, #122792, #188751, #40390, #206060, #174669, #141121, #25182, #73941, #191932, #71777, #106494, #140036, #104315, #170364, #207132, #21948, #75011, #204983, #6779, #137893, #24105, #90208, #156272, #158398, #142173, #92361, #57695, #189816, #91283, #157342, #121714, #88058, #58757, #124909, #105401, #26242, #76073, #171439, #72854, #39306, #208189, #125975, #55559, #23029, #78200, #95556, #177853, #81404, #60887, #144325, #196230, #159454, #127047, #77133, #161607, #28389, #212451, #79273, #47872, #130237, #175720, #80336, #65130, #109715, #163735, #11052, #46799, #110774, #30538, #147487, #64095, #146438, #145391, #213509, #96618, #29465, #179980, #45730, #113983, #31601, #61961, #13197, #112912, #94485, #143254, #97677, #211389, #63017, #129186, #195164, #209243, #193007, #15316, #44660, #43596, #131288, #176774, #178923, #160523, #194078, #12128, #27312, #162672, #93417, #14242, #210324, #128118, #111849, #200460, #198331, #52106, #197275, #148547, #82458, #201521, #113, #32651, #36906, #16379, #167986, #181035, #118234, #184218, #3321, #169046, #4381, #101920, #66180, #48915, #132325, #83524, #53169, #100843, #68326, #2250, #134457, #115035, #35841, #19591, #199394, #70453, #98729, #49971, #85664, #86732, #151750, #69390, #18522, #20643, #135498, #117163, #119297, #51040, #185283, #102988, #1189, #166928, #152802, #33712, #164787, #116090, #183166, #84600, #150688, #182081, #99789, #165855, #17440, #149606, #67253, #133388, #34770, #172264, #71527, #72604, #105142, #190615, #189563, #8674, #40128, #121456, #123598, #25988, #139779, #137638, #205806, #136568, #87806, #21694, #140858, #153879, #186354, #42273, #170108, #107315, #120379, #57437, #41208, #157085, #108386, #158150 ),
 ( #7596, #156008, #73680, #202589, #173339, #24919, #138704, #9743, #54241, #91023, #37989, #74756, #171182, #39056, #104061, #154943, #122535, #56371, #174411, #92096, #124658, #106238, #206872, #22772, #58503, #5448, #203657, #204721, #6527, #55307, #88889, #187427, #188496, #23851, #89958, #127870, #96361, #145124, #161346, #60627, #11869, #94229, #30275, #175467, #126790, #62754, #125718, #27053, #43340, #77946, #76872, #211130, #144067, #128914, #194895, #207937, #12927, #13992, #141925, #178663, #191679, #45468, #176522, #79008, #46533, #44402, #210062, #111585, #142992, #109460, #112654, #160267, #61702, #193820, #177595, #93160, #159197, #162415, #10798, #75817, #80076, #208991, #29207, #192745, #95297, #110522, #59559, #28133, #141557, #172959, #39743, #41902, #158831, #58126, #55993, #124285, #54925, #6142, #154566, #59186, #72212, #104755, #109082, #88504, #25612, #38676, #190244, #108013, #75444, #26684, #76500, #174039, #138319, #121077, #204335, #155628, #125341, #24538, #140483, #74382, #206495, #187044, #91724, #157775, #57061, #142611, #170804, #9373, #22395, #207564, #89579, #171875, #122144, #73287, #40827, #189190, #175097, #92786, #42972, #90646, #191304, #7213, #10428, #188112, #105848, #123225, #139390, #23471, #205423, #106936, #156707, #8297, #11500, #79703, #32028, #163107, #179356, #28830, #46165, #128552, #98114, #77571, #94918, #146871, #110146, #143694, #27759, #112279, #193460, #14687, #29902, #212893, #80783, #126410, #30978, #15751, #60253, #114410, #176159, #211823, #61330, #195601, #164165, #64525, #97053, #95987, #81835, #47236, #194517, #130670, #196658, #209686, #208619, #180410, #93855, #162039, #127489, #144756, #177216, #48299, #113351, #192372, #178295, #45104, #44028, #159893, #63460, #111214, #129614, #160967, #12557, #78631, #210767, #62387, #13630, #145818, #52048, #165798, #67193, #69327, #35782, #102925, #180972, #152738, #149545, #185219, #168986, #66121, #101858, #100783, #135437, #32595, #17382, #167926, #4320, #134396, #201459, #2188, #182022, #98671, #33652 ) ),
 .UNSPECIFIED., .F., .F., .F. ) 
 B_SPLINE_SURFACE_WITH_KNOTS ( ( 2, 2 ),
 ( 3, 2, 2, 2, 2, 2, 2, 2, 2, 2, 2, 2, 2, 2, 2, 2, 2, 2, 2, 2, 2, 2, 2, 2, 2, 2, 2, 2, 2, 2, 2, 2, 2, 2, 2, 2, 2, 2, 2, 2, 2, 2, 2, 2, 2, 2, 2, 2, 2, 2, 2, 2, 2, 2, 2, 2, 2, 2, 2, 2, 2, 2, 2, 2, 2, 2, 2, 2, 2, 2, 2, 2, 2, 2, 2, 2, 2, 2, 2, 2, 2, 2, 2, 2, 2, 2, 2, 2, 2, 2, 2, 2, 2, 2, 2, 2, 2, 2, 2, 2, 2, 2, 2, 2, 2, 2, 2, 2, 2, 2, 2, 2, 2, 2, 2, 2, 2, 2, 2, 2, 3 ),
 ( 0.000000000000000000, 1.000000000000000000 ),
 ( 0.000000000000000000, 0.008333333333333333218, 0.01666666666666666644, 0.02500000000000000139, 0.03333333333333333287, 0.04166666666666666435, 0.05000000000000000278, 0.05833333333333333426, 0.06666666666666666574, 0.07499999999999999722, 0.08333333333333332871, 0.09166666666666666019, 0.1000000000000000056, 0.1083333333333333370, 0.1166666666666666685, 0.1250000000000000000, 0.1333333333333333315, 0.1416666666666666630, 0.1499999999999999944, 0.1583333333333333259, 0.1666666666666666574, 0.1749999999999999889, 0.1833333333333333204, 0.1916666666666666796, 0.2000000000000000111, 0.2083333333333333426, 0.2166666666666666741, 0.2250000000000000056, 0.2333333333333333370, 0.2416666666666666685, 0.2500000000000000000, 0.2583333333333333592, 0.2666666666666666630, 0.2750000000000000222, 0.2833333333333333259, 0.2916666666666666852, 0.2999999999999999889, 0.3083333333333333481, 0.3166666666666666519, 0.3250000000000000111, 0.3333333333333333148, 0.3416666666666666741, 0.3499999999999999778, 0.3583333333333333370, 0.3666666666666666408, 0.3750000000000000000, 0.3833333333333333592, 0.3916666666666666630, 0.4000000000000000222, 0.4083333333333333259, 0.4166666666666666852, 0.4249999999999999889, 0.4333333333333333481, 0.4416666666666666519, 0.4500000000000000111, 0.4583333333333333148, 0.4666666666666666741, 0.4749999999999999778, 0.4833333333333333370, 0.4916666666666666408, 0.5000000000000000000, 0.5083333333333333037, 0.5166666666666667185, 0.5250000000000000222, 0.5333333333333333259, 0.5416666666666666297, 0.5500000000000000444, 0.5583333333333333481, 0.5666666666666666519, 0.5749999999999999556, 0.5833333333333333703, 0.5916666666666666741, 0.5999999999999999778, 0.6083333333333332815, 0.6166666666666666963, 0.6250000000000000000, 0.6333333333333333037, 0.6416666666666667185, 0.6500000000000000222, 0.6583333333333333259, 0.6666666666666666297, 0.6750000000000000444, 0.6833333333333333481, 0.6916666666666666519, 0.6999999999999999556, 0.7083333333333333703, 0.7166666666666666741, 0.7249999999999999778, 0.7333333333333332815, 0.7416666666666666963, 0.7500000000000000000, 0.7583333333333333037, 0.7666666666666667185, 0.7750000000000000222, 0.7833333333333333259, 0.7916666666666666297, 0.8000000000000000444, 0.8083333333333333481, 0.8166666666666666519, 0.8249999999999999556, 0.8333333333333333703, 0.8416666666666666741, 0.8499999999999999778, 0.8583333333333332815, 0.8666666666666666963, 0.8750000000000000000, 0.8833333333333333037, 0.8916666666666667185, 0.9000000000000000222, 0.9083333333333333259, 0.9166666666666666297, 0.9250000000000000444, 0.9333333333333333481, 0.9416666666666666519, 0.9499999999999999556, 0.9583333333333333703, 0.9666666666666666741, 0.9749999999999999778, 0.9833333333333332815, 0.9916666666666666963, 1.000000000000000000 ),
 .UNSPECIFIED. ) 
 GEOMETRIC_REPRESENTATION_ITEM ( )  RATIONAL_B_SPLINE_SURFACE ( (
 ( 1.000000000000000000, 0.8660254037844387076, 1.000000000000000000, 0.8660254037844387076, 1.000000000000000000, 0.8660254037844387076, 1.000000000000000000, 0.8660254037844387076, 1.000000000000000000, 0.8660254037844387076, 1.000000000000000000, 0.8660254037844387076, 1.000000000000000000, 0.8660254037844387076, 1.000000000000000000, 0.8660254037844387076, 1.000000000000000000, 0.8660254037844387076, 1.000000000000000000, 0.8660254037844387076, 1.000000000000000000, 0.8660254037844387076, 1.000000000000000000, 0.8660254037844387076, 1.000000000000000000, 0.8660254037844387076, 1.000000000000000000, 0.8660254037844387076, 1.000000000000000000, 0.8660254037844387076, 1.000000000000000000, 0.8660254037844387076, 1.000000000000000000, 0.8660254037844387076, 1.000000000000000000, 0.8660254037844387076, 1.000000000000000000, 0.8660254037844387076, 1.000000000000000000, 0.8660254037844387076, 1.000000000000000000, 0.8660254037844387076, 1.000000000000000000, 0.8660254037844387076, 1.000000000000000000, 0.8660254037844387076, 1.000000000000000000, 0.8660254037844387076, 1.000000000000000000, 0.8660254037844387076, 1.000000000000000000, 0.8660254037844387076, 1.000000000000000000, 0.8660254037844387076, 1.000000000000000000, 0.8660254037844387076, 1.000000000000000000, 0.8660254037844387076, 1.000000000000000000, 0.8660254037844387076, 1.000000000000000000, 0.8660254037844387076, 1.000000000000000000, 0.8660254037844387076, 1.000000000000000000, 0.8660254037844387076, 1.000000000000000000, 0.8660254037844387076, 1.000000000000000000, 0.8660254037844387076, 1.000000000000000000, 0.8660254037844387076, 1.000000000000000000, 0.8660254037844387076, 1.000000000000000000, 0.8660254037844387076, 1.000000000000000000, 0.8660254037844387076, 1.000000000000000000, 0.8660254037844387076, 1.000000000000000000, 0.8660254037844387076, 1.000000000000000000, 0.8660254037844387076, 1.000000000000000000, 0.8660254037844387076, 1.000000000000000000, 0.8660254037844387076, 1.000000000000000000, 0.8660254037844387076, 1.000000000000000000, 0.8660254037844387076, 1.000000000000000000, 0.8660254037844387076, 1.000000000000000000, 0.8660254037844387076, 1.000000000000000000, 0.8660254037844387076, 1.000000000000000000, 0.8660254037844387076, 1.000000000000000000, 0.8660254037844387076, 1.000000000000000000, 0.8660254037844387076, 1.000000000000000000, 0.8660254037844387076, 1.000000000000000000, 0.8660254037844387076, 1.000000000000000000, 0.8660254037844387076, 1.000000000000000000, 0.8660254037844387076, 1.000000000000000000, 0.8660254037844387076, 1.000000000000000000, 0.8660254037844387076, 1.000000000000000000, 0.8660254037844387076, 1.000000000000000000, 0.8660254037844387076, 1.000000000000000000, 0.8660254037844387076, 1.000000000000000000, 0.8660254037844387076, 1.000000000000000000, 0.8660254037844387076, 1.000000000000000000, 0.8660254037844387076, 1.000000000000000000, 0.8660254037844387076, 1.000000000000000000, 0.8660254037844387076, 1.000000000000000000, 0.8660254037844387076, 1.000000000000000000, 0.8660254037844387076, 1.000000000000000000, 0.8660254037844387076, 1.000000000000000000, 0.8660254037844387076, 1.000000000000000000, 0.8660254037844387076, 1.000000000000000000, 0.8660254037844387076, 1.000000000000000000, 0.8660254037844387076, 1.000000000000000000, 0.8660254037844387076, 1.000000000000000000, 0.8660254037844387076, 1.000000000000000000, 0.8660254037844387076, 1.000000000000000000, 0.8660254037844387076, 1.000000000000000000, 0.8660254037844387076, 1.000000000000000000, 0.8660254037844387076, 1.000000000000000000, 0.8660254037844387076, 1.000000000000000000, 0.8660254037844387076, 1.000000000000000000, 0.8660254037844387076, 1.000000000000000000, 0.8660254037844387076, 1.000000000000000000, 0.8660254037844387076, 1.000000000000000000, 0.8660254037844387076, 1.000000000000000000, 0.8660254037844387076, 1.000000000000000000, 0.8660254037844387076, 1.000000000000000000, 0.8660254037844387076, 1.000000000000000000, 0.8660254037844387076, 1.000000000000000000, 0.8660254037844387076, 1.000000000000000000, 0.8660254037844387076, 1.000000000000000000, 0.8660254037844387076, 1.000000000000000000, 0.8660254037844387076, 1.000000000000000000, 0.8660254037844387076, 1.000000000000000000, 0.8660254037844387076, 1.000000000000000000, 0.8660254037844387076, 1.000000000000000000, 0.8660254037844387076, 1.000000000000000000, 0.8660254037844387076, 1.000000000000000000, 0.8660254037844387076, 1.000000000000000000, 0.8660254037844387076, 1.000000000000000000, 0.8660254037844387076, 1.000000000000000000, 0.8660254037844387076, 1.000000000000000000, 0.8660254037844387076, 1.000000000000000000, 0.8660254037844387076, 1.000000000000000000, 0.8660254037844387076, 1.000000000000000000, 0.8660254037844387076, 1.000000000000000000, 0.8660254037844387076, 1.000000000000000000, 0.8660254037844387076, 1.000000000000000000, 0.8660254037844387076, 1.000000000000000000, 0.8660254037844387076, 1.000000000000000000, 0.8660254037844387076, 1.000000000000000000, 0.8660254037844387076, 1.000000000000000000, 0.8660254037844387076, 1.000000000000000000, 0.8660254037844387076, 1.000000000000000000, 0.8660254037844387076, 1.000000000000000000, 0.8660254037844387076, 1.000000000000000000, 0.8660254037844387076, 1.000000000000000000, 0.8660254037844387076, 1.000000000000000000, 0.8660254037844387076, 1.000000000000000000, 0.8660254037844387076, 1.000000000000000000),
 ( 1.000000000000000000, 0.8660254037844387076, 1.000000000000000000, 0.8660254037844387076, 1.000000000000000000, 0.8660254037844387076, 1.000000000000000000, 0.8660254037844387076, 1.000000000000000000, 0.8660254037844387076, 1.000000000000000000, 0.8660254037844387076, 1.000000000000000000, 0.8660254037844387076, 1.000000000000000000, 0.8660254037844387076, 1.000000000000000000, 0.8660254037844387076, 1.000000000000000000, 0.8660254037844387076, 1.000000000000000000, 0.8660254037844387076, 1.000000000000000000, 0.8660254037844387076, 1.000000000000000000, 0.8660254037844387076, 1.000000000000000000, 0.8660254037844387076, 1.000000000000000000, 0.8660254037844387076, 1.000000000000000000, 0.8660254037844387076, 1.000000000000000000, 0.8660254037844387076, 1.000000000000000000, 0.8660254037844387076, 1.000000000000000000, 0.8660254037844387076, 1.000000000000000000, 0.8660254037844387076, 1.000000000000000000, 0.8660254037844387076, 1.000000000000000000, 0.8660254037844387076, 1.000000000000000000, 0.8660254037844387076, 1.000000000000000000, 0.8660254037844387076, 1.000000000000000000, 0.8660254037844387076, 1.000000000000000000, 0.8660254037844387076, 1.000000000000000000, 0.8660254037844387076, 1.000000000000000000, 0.8660254037844387076, 1.000000000000000000, 0.8660254037844387076, 1.000000000000000000, 0.8660254037844387076, 1.000000000000000000, 0.8660254037844387076, 1.000000000000000000, 0.8660254037844387076, 1.000000000000000000, 0.8660254037844387076, 1.000000000000000000, 0.8660254037844387076, 1.000000000000000000, 0.8660254037844387076, 1.000000000000000000, 0.8660254037844387076, 1.000000000000000000, 0.8660254037844387076, 1.000000000000000000, 0.8660254037844387076, 1.000000000000000000, 0.8660254037844387076, 1.000000000000000000, 0.8660254037844387076, 1.000000000000000000, 0.8660254037844387076, 1.000000000000000000, 0.8660254037844387076, 1.000000000000000000, 0.8660254037844387076, 1.000000000000000000, 0.8660254037844387076, 1.000000000000000000, 0.8660254037844387076, 1.000000000000000000, 0.8660254037844387076, 1.000000000000000000, 0.8660254037844387076, 1.000000000000000000, 0.8660254037844387076, 1.000000000000000000, 0.8660254037844387076, 1.000000000000000000, 0.8660254037844387076, 1.000000000000000000, 0.8660254037844387076, 1.000000000000000000, 0.8660254037844387076, 1.000000000000000000, 0.8660254037844387076, 1.000000000000000000, 0.8660254037844387076, 1.000000000000000000, 0.8660254037844387076, 1.000000000000000000, 0.8660254037844387076, 1.000000000000000000, 0.8660254037844387076, 1.000000000000000000, 0.8660254037844387076, 1.000000000000000000, 0.8660254037844387076, 1.000000000000000000, 0.8660254037844387076, 1.000000000000000000, 0.8660254037844387076, 1.000000000000000000, 0.8660254037844387076, 1.000000000000000000, 0.8660254037844387076, 1.000000000000000000, 0.8660254037844387076, 1.000000000000000000, 0.8660254037844387076, 1.000000000000000000, 0.8660254037844387076, 1.000000000000000000, 0.8660254037844387076, 1.000000000000000000, 0.8660254037844387076, 1.000000000000000000, 0.8660254037844387076, 1.000000000000000000, 0.8660254037844387076, 1.000000000000000000, 0.8660254037844387076, 1.000000000000000000, 0.8660254037844387076, 1.000000000000000000, 0.8660254037844387076, 1.000000000000000000, 0.8660254037844387076, 1.000000000000000000, 0.8660254037844387076, 1.000000000000000000, 0.8660254037844387076, 1.000000000000000000, 0.8660254037844387076, 1.000000000000000000, 0.8660254037844387076, 1.000000000000000000, 0.8660254037844387076, 1.000000000000000000, 0.8660254037844387076, 1.000000000000000000, 0.8660254037844387076, 1.000000000000000000, 0.8660254037844387076, 1.000000000000000000, 0.8660254037844387076, 1.000000000000000000, 0.8660254037844387076, 1.000000000000000000, 0.8660254037844387076, 1.000000000000000000, 0.8660254037844387076, 1.000000000000000000, 0.8660254037844387076, 1.000000000000000000, 0.8660254037844387076, 1.000000000000000000, 0.8660254037844387076, 1.000000000000000000, 0.8660254037844387076, 1.000000000000000000, 0.8660254037844387076, 1.000000000000000000, 0.8660254037844387076, 1.000000000000000000, 0.8660254037844387076, 1.000000000000000000, 0.8660254037844387076, 1.000000000000000000, 0.8660254037844387076, 1.000000000000000000, 0.8660254037844387076, 1.000000000000000000, 0.8660254037844387076, 1.000000000000000000, 0.8660254037844387076, 1.000000000000000000, 0.8660254037844387076, 1.000000000000000000, 0.8660254037844387076, 1.000000000000000000, 0.8660254037844387076, 1.000000000000000000, 0.8660254037844387076, 1.000000000000000000, 0.8660254037844387076, 1.000000000000000000, 0.8660254037844387076, 1.000000000000000000, 0.8660254037844387076, 1.000000000000000000, 0.8660254037844387076, 1.000000000000000000, 0.8660254037844387076, 1.000000000000000000, 0.8660254037844387076, 1.000000000000000000, 0.8660254037844387076, 1.000000000000000000, 0.8660254037844387076, 1.000000000000000000, 0.8660254037844387076, 1.000000000000000000, 0.8660254037844387076, 1.000000000000000000, 0.8660254037844387076, 1.000000000000000000, 0.8660254037844387076, 1.000000000000000000, 0.8660254037844387076, 1.000000000000000000, 0.8660254037844387076, 1.000000000000000000, 0.8660254037844387076, 1.000000000000000000, 0.8660254037844387076, 1.000000000000000000, 0.8660254037844387076, 1.000000000000000000, 0.8660254037844387076, 1.000000000000000000) ) ) 
 REPRESENTATION_ITEM ( '' )  SURFACE ( )  );
#16264=CARTESIAN_POINT ( 'NONE',  ( -7.781453819600577582, 8.043060642480948985, 0.000000000000000000 ) ) ;
#16266=CARTESIAN_POINT ( 'NONE',  ( 6.249382461256315580, 6.255644057745969988, -0.7998128361456481317 ) ) ;
#16272=ORIENTED_EDGE ( 'NONE', *, *, #77102, .T. ) ;
#16278=CARTESIAN_POINT ( 'NONE',  ( 0.003115319777771509598, 2.586180586277187388, -2.083632524825635990 ) ) ;
#16296=CARTESIAN_POINT ( 'NONE',  ( 4.909461021924231616, 8.741805268971372556, 0.7216878364870317197 ) ) ;
#16310=CARTESIAN_POINT ( 'NONE',  ( -5.329763783947941036, 5.390681634126922361, 0.000000000000000000 ) ) ;
#16312=CARTESIAN_POINT ( 'NONE',  ( 5.899733120602060232, 6.912052057904395141, -1.199719254218452047 ) ) ;
#16317=CARTESIAN_POINT ( 'NONE',  ( -3.654804927335652209, 6.421633627603656080, 1.199719254218452935 ) ) ;
#16357=EDGE_CURVE ( 'NONE', #101393, #80951, #99247, .T. ) ;
#16366=CARTESIAN_POINT ( 'NONE',  ( 5.252858170651868441, 5.093032385374103299, -0.7998128361456481317 ) ) ;
#16368=CARTESIAN_POINT ( 'NONE',  ( -4.163571889515733204, 7.868871248772474125, 0.07198445825242587304 ) ) ;
#16372=CARTESIAN_POINT ( 'NONE',  ( -4.787437638956935082, 6.678706226906775179, -1.443375672974066548 ) ) ;
#16379=CARTESIAN_POINT ( 'NONE',  ( -5.478376588373717659, 8.549133898814758936, -1.199719254218452047 ) ) ;
#16385=CARTESIAN_POINT ( 'NONE',  ( 3.606672709164983726, 7.347373054203803378, 0.3819235613196003687 ) ) ;
#16387=CARTESIAN_POINT ( 'NONE',  ( -5.387385936583832802, 7.378645907471495846, -1.599625672291271394 ) ) ;
#16390=CARTESIAN_POINT ( 'NONE',  ( 5.803742400754204667, 7.332416669035665358, 1.290654366993408297 ) ) ;
#16395=CARTESIAN_POINT ( 'NONE',  ( 7.503511670520385479, 7.718794801887437274, 0.7998128361456281477 ) ) ;
#16403=CARTESIAN_POINT ( 'NONE',  ( -5.666381855868691808, 5.575476684793721383, 0.000000000000000000 ) ) ;
#16407=CARTESIAN_POINT ( 'NONE',  ( -7.096767062110449942, 7.244259425409119046, -0.7998128361456362523 ) ) ;
#16411=CARTESIAN_POINT ( 'NONE',  ( 6.089020385868848528, 8.197219431637373432, -1.443375672974078761 ) ) ;
#16413=CARTESIAN_POINT ( 'NONE',  ( -5.573810548549546162, 9.516879716700865188, 0.7216878364870267237 ) ) ;
#16419=CARTESIAN_POINT ( 'NONE',  ( 5.318541398310776103, 9.426991741329731056, -0.7998128361456481317 ) ) ;
#16439=CARTESIAN_POINT ( 'NONE',  ( -5.604676892713675862, 5.547648157612228736, -0.09596228114882204840 ) ) ;
#16448=CARTESIAN_POINT ( 'NONE',  ( 4.720979226589129496, 8.219560628541461966, -0.6735110442024627719 ) ) ;
#16462=CARTESIAN_POINT ( 'NONE',  ( -5.857301623663916601, 7.199535845156014524, -1.157093103336486628 ) ) ;
#16481=CARTESIAN_POINT ( 'NONE',  ( -4.787964524281469458, 5.614988695530339413, -1.199719254218453823 ) ) ;
#16493=CARTESIAN_POINT ( 'NONE',  ( 5.529746549527311039, 7.544733289238903851, -1.599625672291281386 ) ) ;
#16496=CARTESIAN_POINT ( 'NONE',  ( 6.712695452097489301, 7.964471127936110229, -1.082531754730548412 ) ) ;
#16510=CARTESIAN_POINT ( 'NONE',  ( -4.274563570058511175, 8.209017608368725405, 0.000000000000000000 ) ) ;
#16511=CARTESIAN_POINT ( 'NONE',  ( 5.740951700743842423, 5.662474837148078421, -0.7998128361456481317 ) ) ;
#16520=CARTESIAN_POINT ( 'NONE',  ( -7.923814432544069142, 8.209148024248356990, 0.000000000000000000 ) ) ;
#16521=CARTESIAN_POINT ( 'NONE',  ( 6.587282531393223728, 8.778525268082516320, 1.599625672291268286 ) ) ;
#16528=CARTESIAN_POINT ( 'NONE',  ( 5.415556014015861841, 5.282846535965431300, -0.7998128361456481317 ) ) ;
#16535=CARTESIAN_POINT ( 'NONE',  ( -5.689102680971802606, 7.419971068449684459, 1.333831099742349480 ) ) ;
#16540=EDGE_CURVE ( 'NONE', #213971, #71609, #82927, .T. ) ;
#16541=AXIS2_PLACEMENT_3D ( 'NONE', #24474, #106873, #159835 ) ;
#16545=CARTESIAN_POINT ( 'NONE',  ( -4.678972410047611774, 5.591794245544547515, 1.082531754730549078 ) ) ;
#16550=CARTESIAN_POINT ( 'NONE',  ( -2.696596522755091208, 2.993039318081801792, 2.500000000000000444 ) ) ;
#16560=ORIENTED_EDGE ( 'NONE', *, *, #3854, .F. ) ;
#16575=CARTESIAN_POINT ( 'NONE',  ( 3.982994815507484354, 7.308283119008860851, -0.9368446653362592080 ) ) ;
#16594=CARTESIAN_POINT ( 'NONE',  ( 0.4144236700470090295, 2.998638349210888343, 1.957873639358022722 ) ) ;
#16595=CARTESIAN_POINT ( 'NONE',  ( 4.692003678781083487, 7.631698837623355658, -1.199719254218450271 ) ) ;
#16597=AXIS2_PLACEMENT_3D ( 'NONE', #77300, #205141, #122951 ) ;
#16598=CARTESIAN_POINT ( 'NONE',  ( -5.017926250833627755, 5.026871178826882947, 0.7216878364870257245 ) ) ;
#16602=EDGE_CURVE ( 'NONE', #23394, #15686, #93334, .T. ) ;
#16625=CARTESIAN_POINT ( 'NONE',  ( -6.818824913030298696, 6.919993584815607335, 0.7998128361456341429 ) ) ;
#16627=CARTESIAN_POINT ( 'NONE',  ( 6.658462837642799670, 7.901199744405670522, 1.082531754730549967 ) ) ;
#16632=CARTESIAN_POINT ( 'NONE',  ( -5.121948170912633991, 9.197632976031879792, -0.7998128361456362523 ) ) ;
#16641=CARTESIAN_POINT ( 'NONE',  ( -6.611536185319534908, 7.742488966741438716, 1.199719254218452047 ) ) ;
#16648=CARTESIAN_POINT ( 'NONE',  ( 3.553118775233146120, 6.302999783484076524, -1.199719254218453823 ) ) ;
#16654=CARTESIAN_POINT ( 'NONE',  ( -4.990283058281743678, 7.979691447040783814, -1.199719254218453823 ) ) ;
#16657=CARTESIAN_POINT ( 'NONE',  ( -6.292392690518209264, 8.434487120394948079, -1.443375672974066548 ) ) ;
#16660=CARTESIAN_POINT ( 'NONE',  ( -6.631346530415505036, 7.869564052640446228, 1.082531754730549078 ) ) ;
#16661=CARTESIAN_POINT ( 'NONE',  ( 7.635176783151273128, 8.936736330878529699, 1.199719254218452935 ) ) ;
#16662=CARTESIAN_POINT ( 'NONE',  ( -6.084577077482911101, 10.32070003369722144, 0.000000000000000000 ) ) ;
#16681=CARTESIAN_POINT ( 'NONE',  ( 6.333059215844621725, 6.948315255594014417, 0.8781869475623119703 ) ) ;
#16701=CARTESIAN_POINT ( 'NONE',  ( 5.925280661667059690, 7.134359284303951831, -1.114000666120490868 ) ) ;
#16714=CARTESIAN_POINT ( 'NONE',  ( 5.515134625708930649, 9.656350506627580543, 0.000000000000000000 ) ) ;
#16717=CARTESIAN_POINT ( 'NONE',  ( -3.481411583659053566, 7.283673624236017830, 0.000000000000000000 ) ) ;
#16731=CARTESIAN_POINT ( 'NONE',  ( 5.520104819419390907, 6.469152373191302985, 1.199719254218452935 ) ) ;
#16733=CARTESIAN_POINT ( 'NONE',  ( 7.517069824134078537, 7.734612647770044092, 0.000000000000000000 ) ) ;
#16739=CARTESIAN_POINT ( 'NONE',  ( -7.580417283372126391, 8.016444050121833698, 0.7216878364870317197 ) ) ;
#16745=CARTESIAN_POINT ( 'NONE',  ( 5.501576472095266901, 9.640532660744973725, -0.7998128361456481317 ) ) ;
#16760=CARTESIAN_POINT ( 'NONE',  ( -5.424670859243583720, 8.382514198209223721, 1.082531754730550855 ) ) ;
#16761=CARTESIAN_POINT ( 'NONE',  ( 4.990809943606266508, 6.915973915664348937, -1.443375672974068769 ) ) ;
#16766=ORIENTED_EDGE ( 'NONE', *, *, #187556, .F. ) ;
#16771=CARTESIAN_POINT ( 'NONE',  ( -4.014095998097799267, 6.840806543492835345, -1.199719254218450271 ) ) ;
#16772=CARTESIAN_POINT ( 'NONE',  ( -5.139949633356594383, 9.010708648975750634, 0.000000000000000000 ) ) ;
#16777=CARTESIAN_POINT ( 'NONE',  ( 4.326460416092276162, 7.101268681199365496, -1.082531754730548412 ) ) ;
#16793=DIRECTION ( 'NONE',  ( -1.000000000000000000, 1.045014142154703195E-15, 0.000000000000000000 ) ) ;
#16795=CARTESIAN_POINT ( 'NONE',  ( -5.815521545619021460, 5.749472989502435460, -0.7998128361456362523 ) ) ;
#16805=CARTESIAN_POINT ( 'NONE',  ( 3.984117037569365305, 5.741498858621315371, 1.599625672291261402 ) ) ;
#16809=CARTESIAN_POINT ( 'NONE',  ( 4.746236293235721604, 7.694970221153795364, 1.199719254218451159 ) ) ;
#16846=CARTESIAN_POINT ( 'NONE',  ( 4.258669648468278446, 7.022179452304728287, 1.082531754730549078 ) ) ;
#16851=CARTESIAN_POINT ( 'NONE',  ( 4.892490983285298967, 4.880530033246584409, 0.06831354469134912066 ) ) ;
#16852=CARTESIAN_POINT ( 'NONE',  ( 5.695833931072550094, 5.817763472438987726, 0.000000000000000000 ) ) ;
#16853=B_SPLINE_CURVE_WITH_KNOTS ( 'NONE', 3,
 ( #195816, #27186, #47455, #171307, #89017, #204849, #73814, #139907, #32249, #19183 ),
 .UNSPECIFIED., .F., .F.,
 ( 4, 3, 3, 4 ),
 ( 0.000000000000000000, 6.198155766681710474E-05, 0.0001239631899706914050, 0.0002326595646014659722 ),
 .UNSPECIFIED. ) ;
#16855=ADVANCED_FACE ( 'NONE', ( #111956 ), #160630, .F. ) ;
#16868=CARTESIAN_POINT ( 'NONE',  ( -6.252245114557387851, 7.323316050852266557, -1.199719254218453823 ) ) ;
#16876=CARTESIAN_POINT ( 'NONE',  ( 7.201315867513990554, 8.430565262634994284, -1.199719254218452047 ) ) ;
#16882=CARTESIAN_POINT ( 'NONE',  ( -8.086512275908061653, 8.398962174839683215, 0.000000000000000000 ) ) ;
#16888=CARTESIAN_POINT ( 'NONE',  ( -4.990809943606269172, 8.836712344267034780, -0.7216878364870338292 ) ) ;
#16892=CARTESIAN_POINT ( 'NONE',  ( -7.110325215724114578, 7.260077271291732082, 0.000000000000000000 ) ) ;
#16914=CARTESIAN_POINT ( 'NONE',  ( -2.984203208339354152, 6.495671153122273722, 0.000000000000000000 ) ) ;
#16915=CARTESIAN_POINT ( 'NONE',  ( 4.573896719763862251, 6.429575154514868274, -1.599625672291273171 ) ) ;
#16916=CARTESIAN_POINT ( 'NONE',  ( -5.794130544993808307, 7.853181283949808744, 1.599625672291263179 ) ) ;
#16935=CARTESIAN_POINT ( 'NONE',  ( -3.810548893104253487, 8.469546410357084554, -2.499999999999999112 ) ) ;
#16940=( BOUNDED_CURVE ( )  B_SPLINE_CURVE ( 2, ( #75776, #22729, #123556 ),
 .UNSPECIFIED., .F., .T. ) 
 B_SPLINE_CURVE_WITH_KNOTS ( ( 3, 3 ),
 ( 0.4750000000000003664, 0.4832995304647380586 ),
 .UNSPECIFIED. ) 
 CURVE ( )  GEOMETRIC_REPRESENTATION_ITEM ( )  RATIONAL_B_SPLINE_CURVE ( ( 0.9999999999999937828, 0.8665688508649624922, 0.9989175146558251228 ) ) 
 REPRESENTATION_ITEM ( '' )  );
#16960=CARTESIAN_POINT ( 'NONE',  ( 0.000000000000000000, 8.999999999999998224, 0.000000000000000000 ) ) ;
#16967=CARTESIAN_POINT ( 'NONE',  ( 2.911969131885072670, 6.619324097166378706, 0.000000000000000000 ) ) ;
#16980=CARTESIAN_POINT ( 'NONE',  ( 4.601545839464173504, 8.365386937211251706, 0.1680730238927778675 ) ) ;
#16983=CARTESIAN_POINT ( 'NONE',  ( 3.390420931869152721, 6.113185632892752075, -1.199719254218452047 ) ) ;
#16989=CARTESIAN_POINT ( 'NONE',  ( -6.611536185319534908, 7.742488966741438716, 1.199719254218452047 ) ) ;
#16993=CIRCLE ( 'NONE', #65541, 3.100000000000000089 ) ;
#16997=CARTESIAN_POINT ( 'NONE',  ( -6.577113915960828727, 9.727031097712693253, -1.082531754730549967 ) ) ;
#17005=CARTESIAN_POINT ( 'NONE',  ( 4.909461021924231616, 8.741805268971372556, 0.7216878364870317197 ) ) ;
#17008=CARTESIAN_POINT ( 'NONE',  ( -3.623772196602547346, 7.449761006003425834, 0.000000000000000000 ) ) ;
#17019=CARTESIAN_POINT ( 'NONE',  ( 3.715816618597135523, 6.492813934075403637, -1.199719254218453823 ) ) ;
#17020=CARTESIAN_POINT ( 'NONE',  ( 5.896870467300973750, 5.844380064798101237, 0.7998128361456352531 ) ) ;
#17040=CARTESIAN_POINT ( 'NONE',  ( 5.371549237029319634, 7.622127557927130148, 1.287608608630997464 ) ) ;
#17042=CARTESIAN_POINT ( 'NONE',  ( 6.831329296439236032, 9.063246493969506545, -1.599625672291267398 ) ) ;
#17049=CARTESIAN_POINT ( 'NONE',  ( 5.397027666691686321, 8.454226823519094935, 1.199719254218451159 ) ) ;
#17056=CARTESIAN_POINT ( 'NONE',  ( 5.411112705629925301, 5.485588709422586362, 0.000000000000000000 ) ) ;
#17058=EDGE_CURVE ( 'NONE', #56474, #19248, #62072, .T. ) ;
#17060=CARTESIAN_POINT ( 'NONE',  ( 5.560252395380206103, 8.540692657035327429, 1.082531754730547524 ) ) ;
#17073=CARTESIAN_POINT ( 'NONE',  ( -5.614485009834902840, 9.564333254867113610, 0.7216878364870267237 ) ) ;
#17096=CARTESIAN_POINT ( 'NONE',  ( 3.705121118284530279, 7.544668081299086282, -1.734723475976807094E-15 ) ) ;
#17106=CARTESIAN_POINT ( 'NONE',  ( 5.855142236255289845, 7.924361590421551860, -1.599625672291281386 ) ) ;
#17108=CARTESIAN_POINT ( 'NONE',  ( 4.552505719138623341, 8.533283448962240669, 0.7998128361456341429 ) ) ;
#17110=EDGE_CURVE ( 'NONE', #138803, #127411, #11159, .T. ) ;
#17122=CARTESIAN_POINT ( 'NONE',  ( -3.526002468005825286, 6.271364091718859335, -1.199719254218450271 ) ) ;
#17126=CARTESIAN_POINT ( 'NONE',  ( 5.899206235277530297, 7.015400374979486209, -1.082531754730548412 ) ) ;
#17134=CARTESIAN_POINT ( 'NONE',  ( -5.334207092333882017, 5.187939460669764635, 0.7998128361456281477 ) ) ;
#17140=CARTESIAN_POINT ( 'NONE',  ( -5.289089323106922258, 9.184704953684462936, 0.7216878364870267237 ) ) ;
#17142=CARTESIAN_POINT ( 'NONE',  ( -4.340018570150309785, 7.117086527600392287, -1.082531754730551743 ) ) ;
#17150=LINE ( 'NONE', #83226, #35742 ) ;
#17153=CIRCLE ( 'NONE', #165925, 0.08000000000000020983 ) ;
#17159=CARTESIAN_POINT ( 'NONE',  ( -4.981695098378565945, 4.776675467721892332, -0.7998128361456362523 ) ) ;
#17170=CARTESIAN_POINT ( 'NONE',  ( -5.490125858891038213, 5.369844688319787451, -0.7998128361456362523 ) ) ;
#17180=CARTESIAN_POINT ( 'NONE',  ( 4.064661395739702421, 3.791390914876744844, -2.445650119220917240 ) ) ;
#17181=CARTESIAN_POINT ( 'NONE',  ( -4.586114404036374381, 8.497146329035404122, -0.08355658565369419866 ) ) ;
#17197=CARTESIAN_POINT ( 'NONE',  ( 6.547661840756936691, 6.603636667163397256, 0.7998128361456352531 ) ) ;
#17220=CARTESIAN_POINT ( 'NONE',  ( 7.679767667498067496, 7.924426798361372093, 0.000000000000000000 ) ) ;
#17221=CARTESIAN_POINT ( 'NONE',  ( 4.227110032410640095, 8.153655147779589996, 0.7998128361456271485 ) ) ;
#17223=CARTESIAN_POINT ( 'NONE',  ( 3.691562964670865199, 7.528850235416478576, -0.7998128361456362523 ) ) ;
#17235=CARTESIAN_POINT ( 'NONE',  ( 5.258270873920524835, 7.671714958958308017, -1.216365610458163715 ) ) ;
#17237=CARTESIAN_POINT ( 'NONE',  ( -4.760321331729590710, 8.567808963744235839, 0.7216878364870267237 ) ) ;
#17238=CARTESIAN_POINT ( 'NONE',  ( 3.431622278034673901, 7.017660067766835930, -1.734723475976807094E-15 ) ) ;
#17263=CARTESIAN_POINT ( 'NONE',  ( 4.355912491740495440, 8.303924683664389406, 0.000000000000000000 ) ) ;
#17265=CARTESIAN_POINT ( 'NONE',  ( 3.573456005653643519, 6.326726552307992080, -1.199719254218453823 ) ) ;
#17294=CARTESIAN_POINT ( 'NONE',  ( 5.505492895601038938, 8.580769590579979678, -1.199719254218452047 ) ) ;
#17298=CARTESIAN_POINT ( 'NONE',  ( -6.423141557142870717, 6.808251908967412724, 0.4733936187572094223 ) ) ;
#17299=CARTESIAN_POINT ( 'NONE',  ( 5.203297092594585393, 9.292540051327542017, 0.7998128361456341429 ) ) ;
#17331=CARTESIAN_POINT ( 'NONE',  ( -5.596483547390937119, 9.751257581923240991, 0.000000000000000000 ) ) ;
#17333=CARTESIAN_POINT ( 'NONE',  ( 7.364013710877980401, 8.620379413226322285, -1.199719254218452047 ) ) ;
#17346=CARTESIAN_POINT ( 'NONE',  ( -6.567035442730039030, 6.789466400107097677, -0.3981859287331638297 ) ) ;
#17354=CARTESIAN_POINT ( 'NONE',  ( 6.156284269057003655, 9.340026192945279249, -1.199719254218452047 ) ) ;
#17363=CARTESIAN_POINT ( 'NONE',  ( 4.895902868310594513, 8.725987423088758632, 0.000000000000000000 ) ) ;
#17370=CARTESIAN_POINT ( 'NONE',  ( -3.130644732418688569, 6.137896444317757272, -0.8662315412496863765 ) ) ;
#17376=CARTESIAN_POINT ( 'NONE',  ( -4.746763178560296836, 6.631252689777363152, 1.443375672974058777 ) ) ;
#17379=CARTESIAN_POINT ( 'NONE',  ( 4.362691568547328202, 8.311833606605697256, -0.7998128361456381397 ) ) ;
#17382=CARTESIAN_POINT ( 'NONE',  ( -7.553827861469316396, 8.841829255582865699, -1.199719254218452047 ) ) ;
#17384=CARTESIAN_POINT ( 'NONE',  ( -5.002032328799064231, 4.800402236545811441, -0.7998128361456362523 ) ) ;
#17397=CARTESIAN_POINT ( 'NONE',  ( 3.791513125430877373, 7.352524219418101303, -0.3677586026353037996 ) ) ;
#17409=ORIENTED_EDGE ( 'NONE', *, *, #120455, .F. ) ;
#17418=B_SPLINE_SURFACE_WITH_KNOTS ( 'NONE', 1, 3, ( 
 ( #196729, #48369, #114482, #180479, #32098, #201576, #184272, #168041, #135552, #67304, #150742, #19643, #18575, #20697, #53222, #119353, #166985, #151803, #4435, #103044, #84653, #185340, #117218, #169099, #36963, #86788, #149664, #132385, #38045, #1243, #165910, #152857, #2304, #182138, #70504, #85716, #136620, #52159, #3377, #199451, #202646, #54295, #51093, #133445, #120433, #104114, #186407, #69444, #170162, #82513, #99846, #34821, #116151, #183216, #68380, #198385, #148600, #169, #66236, #50027, #33768, #101973, #17495, #134510, #83582, #200514, #100896, #118286, #35896, #124708, #141976, #123653, #172313, #107371, #59616, #206925, #173392, #205860, #121508, #41261, #26039, #92152, #156062, #24975, #188549, #154994, #5499, #58554, #91078, #125773, #158205, #9794, #39110, #189615, #74811, #71580, #57492, #138755, #157138, #87859, #187480, #106293, #75869, #23902, #207988, #171231, #22826, #108443, #43390, #191734, #109511, #88941, #8730, #6579, #174463, #40179, #21751, #105194, #153931, #137688, #140912, #190667, #72659, #42327, #203709, #90008, #204773, #55356, #7650, #56428, #122587, #73735, #139832, #10847, #28185, #46585, #63881, #48711, #94281, #179776, #175519, #145177, #76920, #110573, #160322, #161401, #79059, #93215, #77998, #131085, #163524, #126840, #27107, #61755, #12985, #211182, #15111, #212247, #177650, #193875, #159247, #127923, #143047, #112704, #45523, #30330, #192798, #130035, #209042, #81200, #44457, #176575, #196026, #146230, #31393, #62808, #210115, #11926, #144121, #97468, #111639, #128969, #80125, #96414, #194949, #47662, #147278, #178714, #64935, #213310, #197074, #60678, #29259, #95351, #162463, #14039, #113773, #184015, #118028, #100641, #116956, #133182, #152592, #32450, #84394, #65972, #36699, #214342, #180823, #82251, #68111, #69181, #182955, #181874, #35631, #101709, #166718, #34570, #199182, #4179, #98519, #150481, #132121, #102784 ),
 ( #164581, #85457, #167781, #70249, #168842, #119093, #198131, #134248, #19377, #16166, #2041, #17235, #151543, #148342, #49763, #50829, #20445, #18308, #86527, #115889, #33510, #201315, #136363, #202383, #114825, #99583, #200254, #165647, #52954, #67045, #83310, #149397, #185073, #979, #3110, #135301, #51906, #24716, #89759, #204517, #38850, #9545, #188286, #103855, #90819, #173135, #5241, #169904, #121251, #139572, #156882, #141730, #187221, #58302, #54033, #23651, #21492, #203448, #104933, #39926, #172057, #186147, #170975, #75621, #42073, #71317, #120170, #154739, #106035, #155808, #108187, #8469, #56165, #72396, #37781, #6322, #87602, #205599, #138496, #123397, #137430, #74555, #153673, #174213, #55102, #22574, #140656, #206670, #124457, #7391, #88680, #122329, #73471, #190416, #57237, #189361, #25786, #41002, #107112, #91897, #157953, #29003, #97220, #31146, #179527, #125519, #163272, #94026, #43148, #76674, #60425, #127662, #96159, #113518, #95090, #143864, #78799, #14854, #178460, #144923, #177389, #92959, #12726, #211991, #63632, #193624, #210929, #10598, #207738, #80944, #159005, #176326, #142789, #59362, #62555, #191480, #77743, #162211, #128718, #129786, #209857, #208795, #45266, #126585, #111386, #192546, #195767, #44199, #110320, #27933, #47406, #109261, #160065, #175269, #11669, #13796, #79870, #61495, #26854, #161138, #194690, #46332, #112447, #30069, #145979, #131870, #115629, #19124, #717, #164329, #15919, #82002, #100388, #85203, #181624, #117778, #51656, #34313, #18050, #200006, #197878, #66782, #84137, #83060, #151287, #183769, #35379, #16980, #1795, #68928, #167526, #149136, #101454, #33253, #2858, #135048, #201061, #214095, #196825, #102524, #65722, #148089, #52702, #132922, #32195, #118833, #150225, #184819, #116695, #67852, #49509, #36449, #168586, #99337, #165386, #20186, #147036, #213058, #134000, #64688, #130833, #198927, #50573, #180573 ) ),
 .UNSPECIFIED., .F., .T., .F.,
 ( 2, 2 ),
 ( 4, 2, 2, 2, 2, 2, 2, 2, 2, 2, 2, 2, 2, 2, 2, 2, 2, 2, 2, 2, 2, 2, 2, 2, 2, 2, 2, 2, 2, 2, 2, 2, 2, 2, 2, 2, 2, 2, 2, 2, 2, 2, 2, 2, 2, 2, 2, 2, 2, 2, 2, 2, 2, 2, 2, 2, 2, 2, 2, 2, 2, 2, 2, 2, 2, 2, 2, 2, 2, 2, 2, 2, 2, 2, 2, 2, 2, 2, 2, 2, 2, 2, 2, 2, 2, 2, 2, 2, 2, 2, 2, 2, 2, 2, 2, 2, 2, 2, 2, 2, 2, 2, 2, 2, 2, 2, 2, 2, 2, 2, 2, 4 ),
 ( 0.000000000000000000, 1.000000000000000000 ),
 ( 0.0003185708494972700616, 0.0004481554763622086794, 0.0005777401032271472971, 0.0007073247300920859149, 0.0008369093569570245326, 0.0009017016703894938957, 0.0009664939838219631504, 0.001031286297254432405, 0.001096078610686901768, 0.001225663237551840277, 0.001290455550984309641, 0.001322851707700544322, 0.001355247864416779004, 0.001420040177849248367, 0.001484832491281717730, 0.001614417118146656239, 0.001679209431579125385, 0.001744001745011594749, 0.001808794058444064112, 0.001873586371876533475, 0.001938378685309002621, 0.002003170998741471767, 0.002067963312173941130, 0.002132755625606410493, 0.002197547939038879856, 0.002229944095755114538, 0.002262340252471349220, 0.002391924879336287946, 0.002521509506201226672, 0.002586301819633696035, 0.002651094133066165398, 0.002715886446498634761, 0.002780678759931104124, 0.002910263386796042417, 0.002975055700228511346, 0.003039848013660980709, 0.003104640327093450072, 0.003169432640525919435, 0.003299017267390858162, 0.003428601894255796888, 0.003493394207688266251, 0.003558186521120735614, 0.003622978834553204977, 0.003687771147985673906, 0.003817355774850612199, 0.003946940401715550925, 0.003979336558431785173, 0.004011732715148020288, 0.004076525028580489651, 0.004141317342012959014, 0.004206109655445428377, 0.004270901968877897741, 0.004335694282310367104, 0.004400486595742836467, 0.004465278909175305830, 0.004594863536040244556, 0.004659655849472713919, 0.004724448162905183282, 0.004789240476337652645, 0.004854032789770122008, 0.004918825103202591371, 0.004983617416635060735, 0.005048409730067530098, 0.005113202043499999461, 0.005177994356932468824, 0.005210390513648703939, 0.005242786670364938187, 0.005372371297229876913, 0.005501955924094814772, 0.005566748237527284135, 0.005631540550959752631, 0.005696332864392221994, 0.005761125177824691357, 0.005890709804689630083, 0.005955502118122099446, 0.006020294431554568809, 0.006085086744987038172, 0.006149879058419507535, 0.006214671371851976898, 0.006279463685284446262, 0.006409048312149384988, 0.006473840625581854351, 0.006506236782298089466, 0.006538632939014323714, 0.006603425252446793077, 0.006668217565879262440, 0.006797802192744201166, 0.006862594506176670529, 0.006927386819609139892, 0.006992179133041609256, 0.007056971446474078619, 0.007121763759906547982, 0.007186556073339017345, 0.007251348386771486708, 0.007316140700203956071, 0.007380933013636425434, 0.007445725327068894797, 0.007510517640501363293, 0.007575309953933832656, 0.007704894580798770515, 0.007769686894231239878, 0.007834479207663709241, 0.007866875364379945224, 0.007899271521096179471, 0.007964063834528647967, 0.008093648461393586693, 0.008158440774826056924, 0.008223233088258525419, 0.008288025401690993915, 0.008352817715123464146, 0.008482402341988402872, 0.008611986968853341598 ),
 .UNSPECIFIED. ) ;
#17423=CARTESIAN_POINT ( 'NONE',  ( 2.943528747942701695, 6.448217615992859919, 0.000000000000000000 ) ) ;
#17428=CARTESIAN_POINT ( 'NONE',  ( 5.727393547130178675, 5.646656991265468939, 0.000000000000000000 ) ) ;
#17434=CARTESIAN_POINT ( 'NONE',  ( -4.434925645001610128, 8.188180662561590495, 0.7216878364870338292 ) ) ;
#17440=CARTESIAN_POINT ( 'NONE',  ( -6.668631453075260396, 8.873432343378178544, -1.599625672291271394 ) ) ;
#17449=CARTESIAN_POINT ( 'NONE',  ( -5.498713818794216834, 8.572860667638675380, -1.199719254218452047 ) ) ;
#17452=CARTESIAN_POINT ( 'NONE',  ( 5.057296774772758852, 7.978757421411086348, 1.172581024337983724 ) ) ;
#17457=CARTESIAN_POINT ( 'NONE',  ( 7.828907357248368726, 8.098423103070084395, 0.7998128361456281477 ) ) ;
#17465=CARTESIAN_POINT ( 'NONE',  ( -4.980641328173854632, 6.904110530993182948, 1.599625672291263179 ) ) ;
#17469=CARTESIAN_POINT ( 'NONE',  ( -5.152980901645737077, 8.169505597632108262, -1.199719254218453823 ) ) ;
#17473=CARTESIAN_POINT ( 'NONE',  ( 7.065207446052794715, 9.336104335185329006, -1.443375672974064550 ) ) ;
#17475=CARTESIAN_POINT ( 'NONE',  ( -6.577113915960836721, 8.766661883411348555, -1.443375672974066548 ) ) ;
#17481=CARTESIAN_POINT ( 'NONE',  ( 5.169401708560450004, 9.252995436621013425, 0.000000000000000000 ) ) ;
#17489=CARTESIAN_POINT ( 'NONE',  ( -5.181866634007240791, 6.340624232048664766, 1.284222742053082733 ) ) ;
#17495=CARTESIAN_POINT ( 'NONE',  ( 6.489313741793890422, 6.842916442627623219, -0.5960428994750706089 ) ) ;
#17509=CARTESIAN_POINT ( 'NONE',  ( 4.851297196472967421, 8.072458764906237150, -0.9094135686919021522 ) ) ;
#17522=CARTESIAN_POINT ( 'NONE',  ( -5.962047440371475382, 7.122956488241998230, -1.095284208787988822 ) ) ;
#17525=ORIENTED_EDGE ( 'NONE', *, *, #5141, .T. ) ;
#17539=CARTESIAN_POINT ( 'NONE',  ( -4.522526758610270647, 7.433975764090723359, -1.199719254218453823 ) ) ;
#17553=CARTESIAN_POINT ( 'NONE',  ( 7.205232291019763480, 7.370802192470005565, -0.7998128361456341429 ) ) ;
#17556=CARTESIAN_POINT ( 'NONE',  ( 5.343321937117211817, 9.247976336696488886, 0.000000000000000000 ) ) ;
#17572=CARTESIAN_POINT ( 'NONE',  ( -4.423703259808839938, 8.383013913077441259, 0.7998128361456352531 ) ) ;
#17573=CARTESIAN_POINT ( 'NONE',  ( 5.388439706788500594, 5.251210844200210559, 0.7998128361456352531 ) ) ;
#17582=CARTESIAN_POINT ( 'NONE',  ( -5.002032328799064231, 4.800402236545811441, -0.7998128361456362523 ) ) ;
#17583=CARTESIAN_POINT ( 'NONE',  ( 6.668631453075247073, 8.873432343378178544, -1.599625672291281386 ) ) ;
#17590=CARTESIAN_POINT ( 'NONE',  ( 3.555981428534177091, 7.370671776590375757, 0.7998128361456271485 ) ) ;
#17598=CARTESIAN_POINT ( 'NONE',  ( -6.617491849531519144, 6.756558277422160863, -0.006230766683231955816 ) ) ;
#17599=CARTESIAN_POINT ( 'NONE',  ( -5.939880696118548187, 6.102484698325975288, 0.000000000000000000 ) ) ;
#17607=CARTESIAN_POINT ( 'NONE',  ( -3.973948422136970748, 6.690004688251493192, -1.082531754730546636 ) ) ;
#17612=CARTESIAN_POINT ( 'NONE',  ( -6.177789192036478916, 5.326704385441258793, 2.499999999999775735 ) ) ;
#17629=FACE_OUTER_BOUND ( 'NONE', #135883, .T. ) ;
#17638=CARTESIAN_POINT ( 'NONE',  ( 5.737035277238070385, 6.722237907313067140, -1.199719254218452047 ) ) ;
#17645=VECTOR ( 'NONE', #125725, 1000.000000000000000 ) ;
#17661=CARTESIAN_POINT ( 'NONE',  ( 4.016958651398847557, 7.908478536599129249, -0.7998128361456362523 ) ) ;
#17686=CARTESIAN_POINT ( 'NONE',  ( -6.607619761813764647, 8.802252036906432764, 1.599625672291269396 ) ) ;
#17699=CARTESIAN_POINT ( 'NONE',  ( -7.598418745816086783, 7.829519723065708092, 0.000000000000000000 ) ) ;
#17710=CARTESIAN_POINT ( 'NONE',  ( -5.906512197408906317, 6.919960980845699439, -1.199719254218453823 ) ) ;
#17714=CARTESIAN_POINT ( 'NONE',  ( -7.431277594066160397, 7.842447745931541370, -0.7216878364870338292 ) ) ;
#17716=CARTESIAN_POINT ( 'NONE',  ( -6.577113915960828727, 9.727031097712693253, -1.082531754730549967 ) ) ;
#17717=CARTESIAN_POINT ( 'NONE',  ( 3.973948422136968084, 5.729635473950147606, -1.443375672974068769 ) ) ;
#17718=CARTESIAN_POINT ( 'NONE',  ( -4.787437638956939523, 5.718337012605431369, -1.082531754730549967 ) ) ;
#17731=CARTESIAN_POINT ( 'NONE',  ( -0.2349500406733201208, 2.568208434401662021, 1.989585655505116568 ) ) ;
#17736=CARTESIAN_POINT ( 'NONE',  ( 6.212391540903618115, 7.031971956796816414, -1.022972206104319826 ) ) ;
#17758=CARTESIAN_POINT ( 'NONE',  ( 6.272547281004660746, 6.891683285556123195, -0.7655605874731727933 ) ) ;
#17759=EDGE_CURVE ( 'NONE', #130236, #56668, #75055, .T. ) ;
#17771=CYLINDRICAL_SURFACE ( 'NONE', #108194, 0.4000000000000001332 ) ;
#17776=CARTESIAN_POINT ( 'NONE',  ( -5.926849427829407269, 6.943687749669614995, -1.199719254218453823 ) ) ;
#17790=CARTESIAN_POINT ( 'NONE',  ( 5.032011289327418702, 5.899709921417326974, 1.199719254218452935 ) ) ;
#17792=CARTESIAN_POINT ( 'NONE',  ( 7.503511670520385479, 7.718794801887437274, 0.7998128361456281477 ) ) ;
#17799=CARTESIAN_POINT ( 'NONE',  ( -5.424670858799220063, 9.342883411992149334, 0.000000000000000000 ) ) ;
#17800=ORIENTED_EDGE ( 'NONE', *, *, #171627, .T. ) ;
#17807=CARTESIAN_POINT ( 'NONE',  ( 7.038618024149998043, 8.240751112043669835, -1.199719254218452047 ) ) ;
#17821=CARTESIAN_POINT ( 'NONE',  ( -7.119440060951841787, 7.478637290631501067, 0.000000000000000000 ) ) ;
#17822=CARTESIAN_POINT ( 'NONE',  ( 5.885648082108199119, 6.999582529615296700, 1.082531754730549967 ) ) ;
#17831=ORIENTED_EDGE ( 'NONE', *, *, #194419, .F. ) ;
#17832=CARTESIAN_POINT ( 'NONE',  ( -3.122120512896910505, 6.864500708346841229, 0.7998128361456352531 ) ) ;
#17833=CARTESIAN_POINT ( 'NONE',  ( -5.614485009834902840, 9.564333254867113610, 0.7216878364870267237 ) ) ;
#17834=CARTESIAN_POINT ( 'NONE',  ( 5.854088466050551887, 10.05179665369283981, 0.7998128361456341429 ) ) ;
#17837=CARTESIAN_POINT ( 'NONE',  ( 5.573810548549551491, 6.635772073796838200, -1.082531754730548412 ) ) ;
#17848=CARTESIAN_POINT ( 'NONE',  ( -6.423141557142870717, 6.808251908967412724, 0.4733936187572094223 ) ) ;
#17852=CARTESIAN_POINT ( 'NONE',  ( 0.000000000000000000, 3.480000000000000426, -2.000000000000000000 ) ) ;
#17853=FACE_OUTER_BOUND ( 'NONE', #68438, .T. ) ;
#17856=CARTESIAN_POINT ( 'NONE',  ( -4.685224601974262271, 7.623789914682047808, -1.199719254218453823 ) ) ;
#17869=CARTESIAN_POINT ( 'NONE',  ( 3.054329744828568227, 6.785411478933790264, 0.000000000000000000 ) ) ;
#17884=AXIS2_PLACEMENT_3D ( 'NONE', #96585, #77096, #30504 ) ;
#17896=VERTEX_POINT ( 'NONE', #168782 ) ;
#17907=CARTESIAN_POINT ( 'NONE',  ( 4.692530564105613422, 7.528350520548263702, -1.082531754730548412 ) ) ;
#17913=CARTESIAN_POINT ( 'NONE',  ( 6.360183458142179447, 6.592837920686898556, -0.7216878364870458196 ) ) ;
#17928=CARTESIAN_POINT ( 'NONE',  ( -5.433785704026946384, 9.561443431331920095, 0.000000000000000000 ) ) ;
#17938=CARTESIAN_POINT ( 'NONE',  ( 6.770317605177710085, 8.992066187497757213, 1.599625672291268286 ) ) ;
#17944=CARTESIAN_POINT ( 'NONE',  ( -5.250750630242457362, 9.347902511916677426, 0.000000000000000000 ) ) ;
#17950=CARTESIAN_POINT ( 'NONE',  ( -4.638297949650955765, 8.425448351319163365, 0.7216878364870267237 ) ) ;
#17954=CARTESIAN_POINT ( 'NONE',  ( -7.259464905474441565, 7.434073576000447048, -0.7998128361456362523 ) ) ;
#17959=AXIS2_PLACEMENT_3D ( 'NONE', #192873, #160394, #110647 ) ;
#17972=CARTESIAN_POINT ( 'NONE',  ( -6.580325463743616154, 6.773331238431972601, 0.4807764197584866728 ) ) ;
#17977=CARTESIAN_POINT ( 'NONE',  ( -7.795011973214244883, 8.058878488363559356, 0.7998128361456341429 ) ) ;
#17979=CARTESIAN_POINT ( 'NONE',  ( -5.666381855868691808, 5.575476684793721383, 0.000000000000000000 ) ) ;
#17980=CARTESIAN_POINT ( 'NONE',  ( -5.550083779947821760, 7.568460058062819407, -1.599625672291271394 ) ) ;
#18001=AXIS2_PLACEMENT_3D ( 'NONE', #25821, #44234, #23691 ) ;
#18019=AXIS2_PLACEMENT_3D ( 'NONE', #395, #38012, #104084 ) ;
#18037=CARTESIAN_POINT ( 'NONE',  ( 4.085803189671889157, 5.860132702740892263, -1.599625672291273171 ) ) ;
#18050=CARTESIAN_POINT ( 'NONE',  ( 4.646267551848549004, 8.309382712783076386, 0.4446711254955729165 ) ) ;
#18053=CARTESIAN_POINT ( 'NONE',  ( 4.927462483923885195, 4.713404084191450849, -0.7998128361456481317 ) ) ;
#18058=CARTESIAN_POINT ( 'NONE',  ( -6.473091995881817162, 6.516638514809040217, 0.7998128361456281477 ) ) ;
#18063=CARTESIAN_POINT ( 'NONE',  ( -6.224601922005509991, 10.27613631906616476, 0.7216878364870267237 ) ) ;
#18065=CARTESIAN_POINT ( 'NONE',  ( -5.639168051347689392, 7.169606540874463363, 1.217459232585948570 ) ) ;
#18071=CARTESIAN_POINT ( 'NONE',  ( 4.584065335196252811, 8.362176967788721882, 0.7216878364870328300 ) ) ;
#18075=CARTESIAN_POINT ( 'NONE',  ( -5.496904935697871863, 5.377753611261092637, 0.7998128361456281477 ) ) ;
#18085=CARTESIAN_POINT ( 'NONE',  ( 3.203469434578891661, 6.959407783642502565, -0.7998128361456362523 ) ) ;
#18086=CARTESIAN_POINT ( 'NONE',  ( 4.655245641445829641, 6.524482229810530498, 1.599625672291269396 ) ) ;
#18092=ORIENTED_EDGE ( 'NONE', *, *, #211296, .F. ) ;
#18094=DIRECTION ( 'NONE',  ( 0.000000000000000000, -1.000000000000000000, 0.000000000000000000 ) ) ;
#18111=CARTESIAN_POINT ( 'NONE',  ( 5.671053392266061977, 9.838255734277600695, 0.7998128361456331437 ) ) ;
#18119=CARTESIAN_POINT ( 'NONE',  ( 5.505492895601038938, 8.580769590579979678, -1.199719254218452047 ) ) ;
#18124=CARTESIAN_POINT ( 'NONE',  ( 4.909461021924254709, 5.860697626067345567, 1.082531754730549078 ) ) ;
#18127=CARTESIAN_POINT ( 'NONE',  ( 5.045042558060919724, 8.899983727797476263, -0.7216878364870458196 ) ) ;
#18140=CARTESIAN_POINT ( 'NONE',  ( 6.467812791377033577, 6.763347601114057639, -0.2696018389747659172 ) ) ;
#18141=CARTESIAN_POINT ( 'NONE',  ( -6.617788377246193399, 8.814115421577600529, -1.443375672974066548 ) ) ;
#18147=AXIS2_PLACEMENT_3D ( 'NONE', #49844, #43737, #149480 ) ;
#18158=DIRECTION ( 'NONE',  ( 0.000000000000000000, 0.000000000000000000, -1.000000000000000000 ) ) ;
#18167=AXIS2_PLACEMENT_3D ( 'NONE', #155773, #125487, #206637 ) ;
#18178=CARTESIAN_POINT ( 'NONE',  ( 5.722423353419669567, 8.833855124701747386, 1.199719254218451159 ) ) ;
#18180=CARTESIAN_POINT ( 'NONE',  ( 7.686546744304875389, 7.932335721302671949, 0.7998128361456291469 ) ) ;
#18194=CARTESIAN_POINT ( 'NONE',  ( -4.285259070371116863, 7.157163461145040095, 1.199719254218452935 ) ) ;
#18196=CARTESIAN_POINT ( 'NONE',  ( 4.706088717274896638, 7.544168365912456764, 1.082531754730548412 ) ) ;
#18201=EDGE_CURVE ( 'NONE', #123242, #196200, #9399, .T. ) ;
#18212=CARTESIAN_POINT ( 'NONE',  ( -6.292392690518202159, 9.394856334696294553, -1.082531754730549967 ) ) ;
#18214=CARTESIAN_POINT ( 'NONE',  ( -4.990809943606273613, 7.876343129965691858, -1.082531754730549967 ) ) ;
#18223=CARTESIAN_POINT ( 'NONE',  ( -0.3617947196724534131, 3.196405949189511819, 2.034416336090804744 ) ) ;
#18226=EDGE_CURVE ( 'NONE', #38381, #22501, #165399, .T. ) ;
#18239=CARTESIAN_POINT ( 'NONE',  ( -5.679940009482361774, 5.591294530676332641, 0.7998128361456281477 ) ) ;
#18242=DIRECTION ( 'NONE',  ( -0.6507913734559641616, -0.7592566023653004592, 0.000000000000000000 ) ) ;
#18251=CARTESIAN_POINT ( 'NONE',  ( -4.603205931398525408, 8.475712490939976362, -0.2800714110085516517 ) ) ;
#18271=CARTESIAN_POINT ( 'NONE',  ( 5.013482942003290255, 9.071090208970993274, -0.7998128361456481317 ) ) ;
#18292=CARTESIAN_POINT ( 'NONE',  ( 7.028976294042106332, 7.165170195996068969, 0.000000000000000000 ) ) ;
#18293=CARTESIAN_POINT ( 'NONE',  ( 4.875038752565570732, 7.845239757038595663, -1.199719254218452047 ) ) ;
#18295=CARTESIAN_POINT ( 'NONE',  ( 4.179656494762836516, 8.098292687190454586, -0.7998128361456362523 ) ) ;
#18299=CARTESIAN_POINT ( 'NONE',  ( -1.848071122224620888, 8.944961669792201420, -0.7749999999999996891 ) ) ;
#18308=CARTESIAN_POINT ( 'NONE',  ( 5.410124943364367667, 7.538760657221164507, -1.247639402986647550 ) ) ;
#18310=CARTESIAN_POINT ( 'NONE',  ( -4.462041952228942954, 8.219816354326809460, -0.7216878364870338292 ) ) ;
#18311=CARTESIAN_POINT ( 'NONE',  ( 4.421367491832268293, 7.211993602896056288, 1.082531754730549078 ) ) ;
#18315=B_SPLINE_CURVE_WITH_KNOTS ( 'NONE', 3,
 ( #411, #131576, #181332, #113216, #179221, #78503, #212760, #130539, #196530, #48173, #81707, #114286, #170409, #119603, #183461, #116395 ),
 .UNSPECIFIED., .F., .F.,
 ( 4, 3, 3, 3, 3, 4 ),
 ( 0.000000000000000000, 3.031394987250921340E-05, 4.925505422167386496E-05, 6.478297760331552379E-05, 8.039662739264234889E-05, 9.445464058994319236E-05 ),
 .UNSPECIFIED. ) ;
#18335=CARTESIAN_POINT ( 'NONE',  ( -4.462041952228957165, 5.338708711422782471, -1.082531754730549967 ) ) ;
#18340=CARTESIAN_POINT ( 'NONE',  ( 6.017840079619279692, 8.114175741012878973, -1.599625672291281386 ) ) ;
#18341=EDGE_CURVE ( 'NONE', #183115, #179040, #70, .T. ) ;
#18365=CIRCLE ( 'NONE', #115391, 0.8300000000000008482 ) ;
#18371=CARTESIAN_POINT ( 'NONE',  ( 5.657495238652423097, 9.822437888394988548, 0.000000000000000000 ) ) ;
#18375=CARTESIAN_POINT ( 'NONE',  ( -5.615968211774352348, 7.384814024763004525, 1.238619054342107839 ) ) ;
#18376=CARTESIAN_POINT ( 'NONE',  ( 6.176621499477501054, 9.363752961769195693, -1.199719254218452047 ) ) ;
#18382=CARTESIAN_POINT ( 'NONE',  ( -1.930226670627066099, 8.999999999999998224, 0.7750000000000013545 ) ) ;
#18392=CARTESIAN_POINT ( 'NONE',  ( 4.082413651490639062, 7.776916670132135501, 0.000000000000000000 ) ) ;
#18400=( BOUNDED_CURVE ( )  B_SPLINE_CURVE ( 2, ( #34627, #117011, #98578 ),
 .UNSPECIFIED., .F., .T. ) 
 B_SPLINE_CURVE_WITH_KNOTS ( ( 3, 3 ),
 ( 0.000000000000000000, 0.004310887476439823583 ),
 .UNSPECIFIED. ) 
 CURVE ( )  GEOMETRIC_REPRESENTATION_ITEM ( )  RATIONAL_B_SPLINE_CURVE ( ( 1.000000000000000000, 0.9306940709215905105, 0.9330929566528951558 ) ) 
 REPRESENTATION_ITEM ( '' )  );
#18402=CARTESIAN_POINT ( 'NONE',  ( 4.312902262922978736, 5.164712407232485702, -1.082531754730548412 ) ) ;
#18407=CARTESIAN_POINT ( 'NONE',  ( -5.824109505522200081, 8.952488968821326054, -1.199719254218452047 ) ) ;
#18409=CARTESIAN_POINT ( 'NONE',  ( 6.339319342841494453, 9.553567112360518365, -1.199719254218452047 ) ) ;
#18417=ORIENTED_EDGE ( 'NONE', *, *, #18478, .F. ) ;
#18433=CARTESIAN_POINT ( 'NONE',  ( 7.503511670520385479, 7.718794801887437274, 0.7998128361456281477 ) ) ;
#18442=CARTESIAN_POINT ( 'NONE',  ( 3.902768115887398803, 5.646591783325653147, -1.599625672291269396 ) ) ;
#18455=CARTESIAN_POINT ( 'NONE',  ( -5.316205630334263965, 7.295602216847000498, -1.443375672974066548 ) ) ;
#18457=CARTESIAN_POINT ( 'NONE',  ( 4.538947565524982686, 8.517465603079630299, 0.000000000000000000 ) ) ;
#18461=CARTESIAN_POINT ( 'NONE',  ( -3.332271893908731464, 7.109677319527304640, -0.7998128361456481317 ) ) ;
#18463=CARTESIAN_POINT ( 'NONE',  ( 3.963590886093793397, 7.315322400670926761, -0.9154733054410202353 ) ) ;
#18478=EDGE_CURVE ( 'NONE', #157271, #9317, #147398, .T. ) ;
#18503=ADVANCED_FACE ( 'NONE', ( #135452 ), #53118, .F. ) ;
#18509=CARTESIAN_POINT ( 'NONE',  ( 3.691562964670865199, 7.528850235416478576, -0.7998128361456362523 ) ) ;
#18512=CARTESIAN_POINT ( 'NONE',  ( -6.459533842268148973, 6.500820668926428958, 0.000000000000000000 ) ) ;
#18516=CARTESIAN_POINT ( 'NONE',  ( -5.817857313595549584, 6.920493299683823096, 1.082531754730549078 ) ) ;
#18517=DIRECTION ( 'NONE',  ( 0.000000000000000000, 0.000000000000000000, 1.000000000000000000 ) ) ;
#18522=CARTESIAN_POINT ( 'NONE',  ( -7.449279056065764237, 7.655523418356991350, 0.7998128361456341429 ) ) ;
#18527=EDGE_LOOP ( 'NONE', ( #115810, #120348, #16272, #37605, #57249, #150496 ) ) ;
#18528=CARTESIAN_POINT ( 'NONE',  ( 4.749309608864116683, 4.887773556708002509, -0.7920672577798372194 ) ) ;
#18530=CARTESIAN_POINT ( 'NONE',  ( -7.117104292530948229, 7.267986194233038155, -0.7998128361456362523 ) ) ;
#18532=CARTESIAN_POINT ( 'NONE',  ( 4.601164721245145195, 8.482418317249249995, 0.1585857521721554253 ) ) ;
#18537=CARTESIAN_POINT ( 'NONE',  ( 5.885121196783658526, 9.023669275293071834, 1.199719254218452047 ) ) ;
#18544=CARTESIAN_POINT ( 'NONE',  ( -6.154475385960665790, 6.144919136567696505, 0.000000000000000000 ) ) ;
#18548=CARTESIAN_POINT ( 'NONE',  ( -6.394605727500880299, 7.489403432619674561, -1.199719254218452047 ) ) ;
#18552=CARTESIAN_POINT ( 'NONE',  ( 7.471952054462754234, 8.850270497362297206, 1.082531754730549078 ) ) ;
#18554=CARTESIAN_POINT ( 'NONE',  ( -8.041394506236766659, 8.554250810130591631, -0.7216878364870338292 ) ) ;
#18561=CARTESIAN_POINT ( 'NONE',  ( 4.681308178468477799, 8.683552984847038303, 0.000000000000000000 ) ) ;
#18575=CARTESIAN_POINT ( 'NONE',  ( 5.316739912341137853, 7.735632174496787528, -1.307268462668280673 ) ) ;
#18583=CARTESIAN_POINT ( 'NONE',  ( -2.974907306228248061, 6.692710208982554754, 0.008677196802416714538 ) ) ;
#18591=CARTESIAN_POINT ( 'NONE',  ( 4.743613802917549194, 8.193193991156523026, -0.7244234545457691743 ) ) ;
#18599=CARTESIAN_POINT ( 'NONE',  ( 6.831329296439236032, 9.063246493969506545, -1.599625672291267398 ) ) ;
#18604=CARTESIAN_POINT ( 'NONE',  ( -6.405493493895330737, 6.819705373682535487, -0.5214928506756879578 ) ) ;
#18619=CARTESIAN_POINT ( 'NONE',  ( -5.346851039111044201, 6.199209027673978412, 7.500000000000000000 ) ) ;
#18623=CARTESIAN_POINT ( 'NONE',  ( -3.983063267364693960, 7.868933921892603323, -0.7998128361456481317 ) ) ;
#18627=CARTESIAN_POINT ( 'NONE',  ( 4.137366913483981889, 8.820714063342464328, -0.7750000000000000222 ) ) ;
#18635=ORIENTED_EDGE ( 'NONE', *, *, #167207, .T. ) ;
#18636=CARTESIAN_POINT ( 'NONE',  ( 5.020262018810099924, 9.078999131912302900, 0.7998128361456331437 ) ) ;
#18639=CARTESIAN_POINT ( 'NONE',  ( 6.495764994278797388, 8.671754808115688107, 1.443375672974063439 ) ) ;
#18646=CARTESIAN_POINT ( 'NONE',  ( 5.289089323106923146, 6.303597310780433283, -1.082531754730548412 ) ) ;
#18653=CARTESIAN_POINT ( 'NONE',  ( -4.437261413422502798, 8.398831758960053406, 0.000000000000000000 ) ) ;
#18654=CARTESIAN_POINT ( 'NONE',  ( 5.041653019435334393, 6.975290837464928728, -1.599625672291269396 ) ) ;
#18663=CARTESIAN_POINT ( 'NONE',  ( -7.370792787684826486, 8.628288336167626582, -1.199719254218452047 ) ) ;
#18664=CARTESIAN_POINT ( 'NONE',  ( 7.289443866002793371, 8.533381260871966134, 1.199719254218452047 ) ) ;
#18672=CARTESIAN_POINT ( 'NONE',  ( 3.379725431556547477, 7.165039780116438273, -1.734723475976807094E-15 ) ) ;
#18674=CARTESIAN_POINT ( 'NONE',  ( 5.224688093219824303, 7.188831756880171397, -1.599625672291283607 ) ) ;
#18679=CARTESIAN_POINT ( 'NONE',  ( -4.912146588114373991, 8.123387011080156483, 1.048141424314027237 ) ) ;
#18687=CARTESIAN_POINT ( 'NONE',  ( -8.093291352714894415, 8.406871097780989288, -0.7998128361456362523 ) ) ;
#18691=CARTESIAN_POINT ( 'NONE',  ( -4.010620668045727477, 3.846206254399771929, 2.500000000000000444 ) ) ;
#18696=CARTESIAN_POINT ( 'NONE',  ( 4.923019175537949543, 4.916146257648610352, 0.000000000000000000 ) ) ;
#18714=CARTESIAN_POINT ( 'NONE',  ( 5.845500506147374153, 6.848780674373954547, 1.199719254218453823 ) ) ;
#18736=CARTESIAN_POINT ( 'NONE',  ( 4.041212305325117882, 6.872442235258051646, -1.199719254218448494 ) ) ;
#18737=CARTESIAN_POINT ( 'NONE',  ( -3.824808732831001201, 7.476377598362539345, 0.7216878364870338292 ) ) ;
#18761=CARTESIAN_POINT ( 'NONE',  ( -5.271087860662956537, 9.371629280740593870, 0.000000000000000000 ) ) ;
#18763=CARTESIAN_POINT ( 'NONE',  ( 7.810905894804431426, 8.285347430126213553, 0.000000000000000000 ) ) ;
#18768=CARTESIAN_POINT ( 'NONE',  ( -4.065465959251405081, 5.836405933916976707, -1.599625672291271394 ) ) ;
#18774=CARTESIAN_POINT ( 'NONE',  ( -7.923814432544069142, 8.209148024248356990, 0.000000000000000000 ) ) ;
#18781=CARTESIAN_POINT ( 'NONE',  ( 4.415115299905642665, 5.179997933758551554, -1.199719254218450271 ) ) ;
#18786=CARTESIAN_POINT ( 'NONE',  ( -5.098748287191073203, 8.106234214101666780, 1.199719254218452935 ) ) ;
#18791=CARTESIAN_POINT ( 'NONE',  ( -5.316205630334251531, 9.216340645449683677, -0.7216878364870338292 ) ) ;
#18795=CARTESIAN_POINT ( 'NONE',  ( 4.217995187182922656, 6.014356699837137832, 1.443375672974058777 ) ) ;
#18796=CARTESIAN_POINT ( 'NONE',  ( -7.553827861469316396, 8.841829255582865699, -1.199719254218452047 ) ) ;
#18813=CARTESIAN_POINT ( 'NONE',  ( 6.509182584184366682, 6.829728176725765820, 0.5468608461018635847 ) ) ;
#18834=CARTESIAN_POINT ( 'NONE',  ( 6.467812791377033577, 6.763347601114057639, -0.2696018389747659172 ) ) ;
#18850=CARTESIAN_POINT ( 'NONE',  ( 8.039058738260216330, 8.343599714250547805, -0.7998128361456341429 ) ) ;
#18853=CARTESIAN_POINT ( 'NONE',  ( -6.981522756394290319, 7.109807735406931783, 0.7998128361456341429 ) ) ;
#18866=CARTESIAN_POINT ( 'NONE',  ( 6.886615681098613884, 6.999082814228660077, 0.000000000000000000 ) ) ;
#18868=CARTESIAN_POINT ( 'NONE',  ( 7.354371980770088690, 7.544798497178720531, 0.000000000000000000 ) ) ;
#18875=CARTESIAN_POINT ( 'NONE',  ( -6.333067150914850174, 8.481940657524365434, 1.443375672974064550 ) ) ;
#18880=CARTESIAN_POINT ( 'NONE',  ( 7.147083253059300922, 8.367293879104554577, 1.199719254218452935 ) ) ;
#18885=LINE ( 'NONE', #21007, #142339 ) ;
#18887=EDGE_CURVE ( 'NONE', #92086, #207114, #85215, .T. ) ;
#18893=CARTESIAN_POINT ( 'NONE',  ( -6.794044374223859428, 7.099008989448849505, 0.000000000000000000 ) ) ;
#18894=CARTESIAN_POINT ( 'NONE',  ( 5.072158865288222351, 8.931619419562697004, 0.7216878364870317197 ) ) ;
#18904=CARTESIAN_POINT ( 'NONE',  ( -5.255720823952942489, 6.160704378480398979, -1.199719254218453823 ) ) ;
#18905=CARTESIAN_POINT ( 'NONE',  ( -7.946487431385463651, 8.443525889470736345, 0.7216878364870317197 ) ) ;
#18908=CARTESIAN_POINT ( 'NONE',  ( 6.333067150914820864, 6.561202228921677815, 0.7216878364870328300 ) ) ;
#18920=CARTESIAN_POINT ( 'NONE',  ( -5.394899524673852476, 7.567224757263017132, 1.245178244268474010 ) ) ;
#18925=CARTESIAN_POINT ( 'NONE',  ( 3.770576118376306241, 6.452737000530752276, 1.082531754730549078 ) ) ;
#18928=CARTESIAN_POINT ( 'NONE',  ( -5.061990249855848667, 6.999017606288844284, -1.599625672291271394 ) ) ;
#18934=VECTOR ( 'NONE', #202463, 1000.000000000000000 ) ;
#18942=CARTESIAN_POINT ( 'NONE',  ( 6.048345925472166762, 10.07050432311064903, 0.7216878364870317197 ) ) ;
#18981=CARTESIAN_POINT ( 'NONE',  ( 5.397554552016216256, 7.390509292142662723, 1.443375672974065660 ) ) ;
#18988=CARTESIAN_POINT ( 'NONE',  ( 6.007671464186834065, 7.141943142040370063, 1.082531754730549967 ) ) ;
#18989=CARTESIAN_POINT ( 'NONE',  ( -3.947104627881229622, 8.980740528189222971, 0.7749999999999996891 ) ) ;
#19003=CARTESIAN_POINT ( 'NONE',  ( -7.632314129850253259, 7.869064337772231355, 0.7998128361456341429 ) ) ;
#19015=CARTESIAN_POINT ( 'NONE',  ( 4.923019175093585886, 5.876515471431535076, -1.082531754730548412 ) ) ;
#19020=CARTESIAN_POINT ( 'NONE',  ( -5.264308783856126439, 9.363720357799287797, -0.7998128361456362523 ) ) ;
#19025=CARTESIAN_POINT ( 'NONE',  ( -6.970300371201519241, 7.304640985922785212, 0.7216878364870317197 ) ) ;
#19028=CARTESIAN_POINT ( 'NONE',  ( -6.261886844665283114, 8.398896966899865646, 1.599625672291269396 ) ) ;
#19051=CARTESIAN_POINT ( 'NONE',  ( -5.438229012412903352, 6.477593614970734492, -1.082531754730549967 ) ) ;
#19054=CARTESIAN_POINT ( 'NONE',  ( 4.712340909201580885, 7.655425606447271214, -1.199719254218452047 ) ) ;
#19055=CARTESIAN_POINT ( 'NONE',  ( -5.490125858891038213, 5.369844688319787451, -0.7998128361456362523 ) ) ;
#19056=CARTESIAN_POINT ( 'NONE',  ( -4.769436176957319695, 8.786368983084006601, 0.7998128361456281477 ) ) ;
#19098=CIRCLE ( 'NONE', #188725, 0.7499999999999997780 ) ;
#19103=CARTESIAN_POINT ( 'NONE',  ( -4.955918092712652268, 4.886086657537050293, 0.4932186882876873901 ) ) ;
#19111=CARTESIAN_POINT ( 'NONE',  ( 3.223806664999388172, 6.983134552466421674, -0.7998128361456362523 ) ) ;
#19112=CARTESIAN_POINT ( 'NONE',  ( 4.094037528094967016, 3.811616672697253350, -2.445516385416635963 ) ) ;
#19121=EDGE_CURVE ( 'NONE', #115058, #96370, #211809, .T. ) ;
#19124=CARTESIAN_POINT ( 'NONE',  ( 4.771497086726927073, 8.161215468402982509, 0.7801120568680236511 ) ) ;
#19127=CARTESIAN_POINT ( 'NONE',  ( 5.415556014015861841, 5.282846535965431300, -0.7998128361456481317 ) ) ;
#19133=CARTESIAN_POINT ( 'NONE',  ( -6.017840079619296567, 8.114175741012878973, -1.599625672291271394 ) ) ;
#19141=CARTESIAN_POINT ( 'NONE',  ( -6.132724857352506831, 6.712246147164017351, 0.7681735678050619631 ) ) ;
#19147=AXIS2_PLACEMENT_3D ( 'NONE', #2693, #15763, #131715 ) ;
#19148=CARTESIAN_POINT ( 'NONE',  ( 5.017926250833595780, 7.907978821730911712, -1.082531754730548412 ) ) ;
#19152=CARTESIAN_POINT ( 'NONE',  ( -4.634908411025374875, 6.500755460986618495, 1.599625672291263179 ) ) ;
#19163=CARTESIAN_POINT ( 'NONE',  ( 5.225741863424510747, 5.061396693608882558, 0.7998128361456352531 ) ) ;
#19164=CARTESIAN_POINT ( 'NONE',  ( 3.898851692381625877, 6.706354853490643642, -1.199719254218452047 ) ) ;
#19170=ORIENTED_EDGE ( 'NONE', *, *, #210167, .T. ) ;
#19183=CARTESIAN_POINT ( 'NONE',  ( -6.326802395788107880, 6.950450678040672514, 0.9045734915664763731 ) ) ;
#19191=CARTESIAN_POINT ( 'NONE',  ( 3.923105346307896202, 5.670318552149568703, -1.599625672291269396 ) ) ;
#19196=CARTESIAN_POINT ( 'NONE',  ( 6.692885107001518286, 7.837396042037102717, -1.199719254218452047 ) ) ;
#19201=CARTESIAN_POINT ( 'NONE',  ( 4.421367491832268293, 7.211993602896056288, 1.082531754730549078 ) ) ;
#19204=CARTESIAN_POINT ( 'NONE',  ( 6.048345925472166762, 10.07050432311064903, 0.7216878364870317197 ) ) ;
#19205=ORIENTED_EDGE ( 'NONE', *, *, #213637, .T. ) ;
#19217=CARTESIAN_POINT ( 'NONE',  ( 6.292946923374557855, 6.878031543426355476, -0.7329977330566839200 ) ) ;
#19218=CARTESIAN_POINT ( 'NONE',  ( -5.587368702607575344, 8.572328348800551723, 1.082531754730550855 ) ) ;
#19246=TOROIDAL_SURFACE ( 'NONE', #168011, 3.970406073902761790, 0.08000000000000000167 ) ;
#19248=VERTEX_POINT ( 'NONE', #67739 ) ;
#19252=CARTESIAN_POINT ( 'NONE',  ( 6.475954649182838807, 7.584310507915338562, 1.199719254218452047 ) ) ;
#19254=CARTESIAN_POINT ( 'NONE',  ( 5.691390622686558487, 9.861982503101517139, 0.7998128361456341429 ) ) ;
#19267=CARTESIAN_POINT ( 'NONE',  ( -3.800028193580205382, 7.655393002477360653, -0.7998128361456481317 ) ) ;
#19269=CARTESIAN_POINT ( 'NONE',  ( 6.007671464186825183, 8.102312356341712984, 1.443375672974064550 ) ) ;
#19278=FACE_OUTER_BOUND ( 'NONE', #13587, .T. ) ;
#19285=CARTESIAN_POINT ( 'NONE',  ( -7.132998214565509087, 7.494455136514109661, 0.7216878364870317197 ) ) ;
#19287=CARTESIAN_POINT ( 'NONE',  ( -6.482206841109545259, 6.735198534148810090, 0.7216878364870257245 ) ) ;
#19295=CARTESIAN_POINT ( 'NONE',  ( -0.3031628594467480897, 3.278079808138081752, 2.050209013101042643 ) ) ;
#19313=CARTESIAN_POINT ( 'NONE',  ( -4.281342646865346602, 8.216926531310035031, 0.7998128361456352531 ) ) ;
#19323=CARTESIAN_POINT ( 'NONE',  ( 2.713058575063114652, 3.002994061098673395, -2.500000000000000444 ) ) ;
#19324=CARTESIAN_POINT ( 'NONE',  ( -5.696549332702473656, 7.414053552612095643, -1.332310987329322183 ) ) ;
#19326=CARTESIAN_POINT ( 'NONE',  ( 4.540391295830774609, 8.311223921862364250, 0.5620231006616300817 ) ) ;
#19332=CARTESIAN_POINT ( 'NONE',  ( -3.811250579217344558, 5.539821323877241355, 0.000000000000000000 ) ) ;
#19340=CARTESIAN_POINT ( 'NONE',  ( 5.091969210384201361, 8.098325291160362482, 1.199719254218452047 ) ) ;
#19361=CARTESIAN_POINT ( 'NONE',  ( 6.367489420273535039, 7.457767740854454708, -1.199719254218452047 ) ) ;
#19362=CARTESIAN_POINT ( 'NONE',  ( 6.737475991348287785, 6.825086509519945999, -0.7998128361456481317 ) ) ;
#19364=CARTESIAN_POINT ( 'NONE',  ( 5.391302360089590628, 6.318882837306503575, -1.199719254218452047 ) ) ;
#19377=CARTESIAN_POINT ( 'NONE',  ( 5.170590401584001405, 7.751911629329717002, -1.182414590771277085 ) ) ;
#19379=CARTESIAN_POINT ( 'NONE',  ( -7.092323753280154186, 7.447001598347859463, 0.7216878364870317197 ) ) ;
#19380=CARTESIAN_POINT ( 'NONE',  ( 3.770576118376296471, 7.413106214832098750, 0.7216878364870257245 ) ) ;
#19401=CARTESIAN_POINT ( 'NONE',  ( -5.614485009390564940, 5.722856397143323726, 0.000000000000000000 ) ) ;
#19407=CARTESIAN_POINT ( 'NONE',  ( 6.180537922983273091, 8.303989891604203422, -1.599625672291281386 ) ) ;
#19429=DIRECTION ( 'NONE',  ( 0.000000000000000000, 1.000000000000000000, 0.000000000000000000 ) ) ;
#19433=CARTESIAN_POINT ( 'NONE',  ( 6.638652492546827766, 7.774124658506663010, 1.199719254218452047 ) ) ;
#19437=CARTESIAN_POINT ( 'NONE',  ( 7.523848900940885542, 7.742521570711348389, 0.7998128361456291469 ) ) ;
#19466=CARTESIAN_POINT ( 'NONE',  ( 4.800995793014950941, 5.734154859006458160, -1.082531754730548412 ) ) ;
#19470=CARTESIAN_POINT ( 'NONE',  ( -7.279802135894939852, 7.457800344824362604, -0.7998128361456362523 ) ) ;
#19472=CARTESIAN_POINT ( 'NONE',  ( 7.198453214212898743, 7.362893269528701268, 0.7998128361456291469 ) ) ;
#19473=CARTESIAN_POINT ( 'NONE',  ( -2.862179826260718762, 6.353310540697199471, 0.000000000000000000 ) ) ;
#19476=B_SPLINE_CURVE_WITH_KNOTS ( 'NONE', 3,
 ( #68737, #184629, #85009, #51457, #34125, #17852 ),
 .UNSPECIFIED., .F., .F.,
 ( 4, 2, 4 ),
 ( 0.002871295844531347036, 0.002933344926395646882, 0.002995394008259946294 ),
 .UNSPECIFIED. ) ;
#19489=CARTESIAN_POINT ( 'NONE',  ( -5.939880696118548187, 6.102484698325975288, 0.000000000000000000 ) ) ;
#19492=CARTESIAN_POINT ( 'NONE',  ( -3.880700980283063650, 7.437752890734468991, 0.4300534088077876405 ) ) ;
#19496=CARTESIAN_POINT ( 'NONE',  ( 5.345657705538078730, 9.458627433094950021, 0.7998128361456331437 ) ) ;
#19505=CARTESIAN_POINT ( 'NONE',  ( 6.048345925472178308, 9.110135108809304327, 1.082531754730549967 ) ) ;
#19518=CARTESIAN_POINT ( 'NONE',  ( -6.807602527837528505, 7.114826835331461652, 0.7216878364870317197 ) ) ;
#19521=CIRCLE ( 'NONE', #47244, 2.000000000000000000 ) ;
#19522=CARTESIAN_POINT ( 'NONE',  ( 5.352436782344940802, 9.466536356036257871, 0.000000000000000000 ) ) ;
#19527=CARTESIAN_POINT ( 'NONE',  ( -5.503684012504701961, 5.385662534202396934, 0.000000000000000000 ) ) ;
#19544=CARTESIAN_POINT ( 'NONE',  ( 3.821228196946160338, 7.349073440743831398, -0.5400038253845617087 ) ) ;
#19573=CARTESIAN_POINT ( 'NONE',  ( 4.909461021924254709, 5.860697626067345567, 1.082531754730549078 ) ) ;
#19578=CARTESIAN_POINT ( 'NONE',  ( 3.932747076415766596, 6.745899468197171345, 1.199719254218451159 ) ) ;
#19581=CARTESIAN_POINT ( 'NONE',  ( -5.960744811863571968, 6.983232364376142698, 1.199719254218452935 ) ) ;
#19582=CARTESIAN_POINT ( 'NONE',  ( -5.978219388983010418, 5.939287140093763462, -0.7998128361456361413 ) ) ;
#19584=ORIENTED_EDGE ( 'NONE', *, *, #68379, .T. ) ;
#19585=CARTESIAN_POINT ( 'NONE',  ( -5.438229012412899799, 7.437962829272074750, -1.443375672974066548 ) ) ;
#19591=CARTESIAN_POINT ( 'NONE',  ( -5.749539660647037032, 8.865490816466966351, 1.199719254218454489 ) ) ;
#19600=CARTESIAN_POINT ( 'NONE',  ( -6.954406449166956605, 7.078172043641714595, -0.7998128361456362523 ) ) ;
#19601=ORIENTED_EDGE ( 'NONE', *, *, #19728, .T. ) ;
#19602=CARTESIAN_POINT ( 'NONE',  ( 5.004104291928844539, 8.031804922028364047, 1.127571413376940335 ) ) ;
#19607=CARTESIAN_POINT ( 'NONE',  ( 6.668631453075247073, 8.873432343378178544, -1.599625672291281386 ) ) ;
#19617=CARTESIAN_POINT ( 'NONE',  ( -5.915100157312088491, 10.12297696016459092, -0.7998128361456362523 ) ) ;
#19619=CARTESIAN_POINT ( 'NONE',  ( 6.360183458142182111, 6.592837920686895004, -0.7216878364870427109 ) ) ;
#19623=CARTESIAN_POINT ( 'NONE',  ( -6.685579144870156476, 9.853573864773576219, 1.082531754730549967 ) ) ;
#19629=CARTESIAN_POINT ( 'NONE',  ( 5.936491157937257235, 8.019268665717216749, 1.599625672291268286 ) ) ;
#19638=ADVANCED_FACE ( 'NONE', ( #186854 ), #103657, .T. ) ;
#19643=CARTESIAN_POINT ( 'NONE',  ( 5.300918301777743480, 7.749796750553542779, -1.302405036909856761 ) ) ;
#19651=CARTESIAN_POINT ( 'NONE',  ( -2.974142338115852269, 6.685868392857900133, 0.1038623869373533903 ) ) ;
#19664=CARTESIAN_POINT ( 'NONE',  ( 3.919715808126649659, 7.587102519540811940, 0.000000000000000000 ) ) ;
#19671=CARTESIAN_POINT ( 'NONE',  ( -6.468510628652166972, 6.779004017053734898, -0.3101152288892006781 ) ) ;
#19690=CARTESIAN_POINT ( 'NONE',  ( -4.956387674247580755, 7.940146832334256111, 1.199719254218452935 ) ) ;
#19706=CARTESIAN_POINT ( 'NONE',  ( 6.475954649182838807, 7.584310507915338562, 1.199719254218452047 ) ) ;
#19709=CARTESIAN_POINT ( 'NONE',  ( 5.831415467209187575, 9.817418788470464008, 0.000000000000000000 ) ) ;
#19712=ADVANCED_FACE ( 'NONE', ( #61695 ), #31341, .F. ) ;
#19718=B_SPLINE_CURVE_WITH_KNOTS ( 'NONE', 3,
 ( #165250, #183624, #197740, #126710, #180444, #143991 ),
 .UNSPECIFIED., .F., .F.,
 ( 4, 2, 4 ),
 ( 9.243101720622088096E-18, 9.928037272730919299E-05, 0.0001985607454546091432 ),
 .UNSPECIFIED. ) ;
#19723=CARTESIAN_POINT ( 'NONE',  ( -4.925354943514475003, 8.968274210734028529, 0.000000000000000000 ) ) ;
#19724=CARTESIAN_POINT ( 'NONE',  ( 6.364626766972446781, 6.390095747748157251, 0.7998128361456352531 ) ) ;
#19728=EDGE_CURVE ( 'NONE', #38781, #22085, #81994, .T. ) ;
#19733=CARTESIAN_POINT ( 'NONE',  ( -5.752402313948099533, 9.933162809573264695, -0.7998128361456362523 ) ) ;
#19734=CARTESIAN_POINT ( 'NONE',  ( 6.156284269057003655, 9.340026192945279249, -1.199719254218452047 ) ) ;
#19740=CARTESIAN_POINT ( 'NONE',  ( 6.873057527484919937, 6.983264968346048818, 0.7998128361456352531 ) ) ;
#19743=CARTESIAN_POINT ( 'NONE',  ( -3.894033820048823813, 8.999999999999998224, 0.7749999999999996891 ) ) ;
#19746=CARTESIAN_POINT ( 'NONE',  ( -4.845071979149651042, 8.194897641035423064, 0.9605101338234197650 ) ) ;
#19756=CARTESIAN_POINT ( 'NONE',  ( -5.139949632912262700, 5.169231791251960750, 0.7216878364870257245 ) ) ;
#19765=CARTESIAN_POINT ( 'NONE',  ( 3.580761967785000888, 7.191656372475549119, -0.7216878364870338292 ) ) ;
#19769=CARTESIAN_POINT ( 'NONE',  ( -5.448397627845328550, 7.449826213943242514, 1.599625672291263179 ) ) ;
#19773=EDGE_CURVE ( 'NONE', #120691, #164262, #96354, .T. ) ;
#19781=CARTESIAN_POINT ( 'NONE',  ( 4.207966135563057541, 7.175396087857926375, 1.156120096431498379 ) ) ;
#19786=CARTESIAN_POINT ( 'NONE',  ( 4.386945222473598527, 7.275797305264619652, -1.199719254218452047 ) ) ;
#19805=CARTESIAN_POINT ( 'NONE',  ( -0.4461809497497637444, 3.122791860410086606, 1.949595486268986821 ) ) ;
#19807=CARTESIAN_POINT ( 'NONE',  ( 5.041653019435334393, 6.975290837464928728, -1.599625672291269396 ) ) ;
#19808=CARTESIAN_POINT ( 'NONE',  ( -4.990809943606286048, 5.955604701363006015, -1.082531754730549967 ) ) ;
#19832=EDGE_CURVE ( 'NONE', #71609, #191915, #188658, .T. ) ;
#19834=CARTESIAN_POINT ( 'NONE',  ( -6.957269102468015554, 8.145844036748005834, 1.199719254218452047 ) ) ;
#19847=CARTESIAN_POINT ( 'NONE',  ( -5.589704470584107909, 9.743348658981940247, -0.7998128361456362523 ) ) ;
#19854=CARTESIAN_POINT ( 'NONE',  ( 3.217027588192558074, 6.975225629525113824, -1.734723475976807094E-15 ) ) ;
#19859=CARTESIAN_POINT ( 'NONE',  ( -4.762657100150483380, 8.778460060142702304, 0.000000000000000000 ) ) ;
#19864=CARTESIAN_POINT ( 'NONE',  ( -7.783789588021474692, 8.253711738879413673, 0.7216878364870317197 ) ) ;
#19867=CARTESIAN_POINT ( 'NONE',  ( -6.902509602688818191, 9.146290184594002781, -1.443375672974066548 ) ) ;
#19868=CARTESIAN_POINT ( 'NONE',  ( 3.892599500454932304, 7.555466827257172113, 0.7216878364870257245 ) ) ;
#19869=CARTESIAN_POINT ( 'NONE',  ( -3.621436428181653788, 7.239109909604962922, 0.7216878364870338292 ) ) ;
#19882=CARTESIAN_POINT ( 'NONE',  ( 0.3857320732078021175, 2.894052512584739834, 1.963429802559124138 ) ) ;
#19886=CARTESIAN_POINT ( 'NONE',  ( 2.977454500823585093, 6.499579965040511276, -0.5808385047149626779 ) ) ;
#19887=CARTESIAN_POINT ( 'NONE',  ( 6.454463653088309272, 6.866155873091829953, 0.6733577401037347254 ) ) ;
#19907=CARTESIAN_POINT ( 'NONE',  ( 6.486339200172205999, 6.751434215916642501, 0.1376000389162572446 ) ) ;
#19924=CARTESIAN_POINT ( 'NONE',  ( -5.607179047703544583, 8.699403434699558346, 1.199719254218454489 ) ) ;
#19936=CARTESIAN_POINT ( 'NONE',  ( 6.873057527484919937, 6.983264968346048818, 0.7998128361456352531 ) ) ;
#19943=CARTESIAN_POINT ( 'NONE',  ( -5.600926855776877211, 9.548515408466085930, -0.7216878364870338292 ) ) ;
#19947=CARTESIAN_POINT ( 'NONE',  ( 7.635176783151273128, 8.936736330878529699, 1.199719254218452935 ) ) ;
#19963=CARTESIAN_POINT ( 'NONE',  ( -5.261973015879593873, 8.192700047617899273, 1.082531754730549967 ) ) ;
#19964=CARTESIAN_POINT ( 'NONE',  ( 5.397554552016212703, 8.350878506444006533, 1.082531754730547524 ) ) ;
#19966=CARTESIAN_POINT ( 'NONE',  ( 0.000000000000000000, 2.999999999999999112, -2.420000000000000373 ) ) ;
#19974=ORIENTED_EDGE ( 'NONE', *, *, #14937, .T. ) ;
#19975=CARTESIAN_POINT ( 'NONE',  ( -5.957882158562513908, 5.915560371269843465, -0.7998128361456362523 ) ) ;
#19976=CARTESIAN_POINT ( 'NONE',  ( -2.986538976760251263, 6.706322249520737522, -0.7998128361456481317 ) ) ;
#19978=CARTESIAN_POINT ( 'NONE',  ( 6.495764994278809823, 6.751016379513001375, 0.7216878364870328300 ) ) ;
#19980=VERTEX_POINT ( 'NONE', #43246 ) ;
#19991=CARTESIAN_POINT ( 'NONE',  ( -4.604461168338175980, 8.383524640989071131, 0.06638267717353450725 ) ) ;
#19999=CARTESIAN_POINT ( 'NONE',  ( -3.983063267364693960, 7.868933921892603323, -0.7998128361456481317 ) ) ;
#20011=CARTESIAN_POINT ( 'NONE',  ( 5.065906673361608270, 5.939254536123854677, -1.199719254218450271 ) ) ;
#20032=VECTOR ( 'NONE', #62486, 1000.000000000000114 ) ;
#20048=CARTESIAN_POINT ( 'NONE',  ( 5.722950238744200391, 7.770137593325314285, 1.443375672974065660 ) ) ;
#20052=CARTESIAN_POINT ( 'NONE',  ( 6.983858524370782916, 7.320458831286981827, 0.7216878364870328300 ) ) ;
#20066=CARTESIAN_POINT ( 'NONE',  ( -7.014364370223741929, 9.276787413384745662, -1.599625672291271394 ) ) ;
#20076=CARTESIAN_POINT ( 'NONE',  ( -2.844178363816758814, 6.540234867753325076, -0.7998128361456481317 ) ) ;
#20078=CARTESIAN_POINT ( 'NONE',  ( 5.207740400980577888, 5.248321020665011716, 0.000000000000000000 ) ) ;
#20085=CARTESIAN_POINT ( 'NONE',  ( -6.400331034103001748, 9.624747418832267698, 1.199719254218452935 ) ) ;
#20091=CARTESIAN_POINT ( 'NONE',  ( -6.631346530859867805, 6.909194838857525944, 0.000000000000000000 ) ) ;
#20094=CARTESIAN_POINT ( 'NONE',  ( -5.427006627220116286, 9.553534508390610469, -0.7998128361456362523 ) ) ;
#20102=CONICAL_SURFACE ( 'NONE', #103153, 3.999999999999998224, 0.8621700546672330656 ) ;
#20114=CARTESIAN_POINT ( 'NONE',  ( -3.350273356352693188, 6.922752992471175482, 0.000000000000000000 ) ) ;
#20116=CARTESIAN_POINT ( 'NONE',  ( -4.787437638956939523, 5.718337012605431369, -1.082531754730549967 ) ) ;
#20118=CARTESIAN_POINT ( 'NONE',  ( 3.576318658954677598, 7.394398545414291313, 0.7998128361456281477 ) ) ;
#20119=CARTESIAN_POINT ( 'NONE',  ( -5.503684012504701961, 5.385662534202396934, 0.000000000000000000 ) ) ;
#20120=CARTESIAN_POINT ( 'NONE',  ( -6.257970421159510188, 9.458660037064859694, 1.199719254218452047 ) ) ;
#20173=CARTESIAN_POINT ( 'NONE',  ( 4.869313445963426190, 5.709895770826003414, 1.199719254218452935 ) ) ;
#20186=CARTESIAN_POINT ( 'NONE',  ( 4.735857411151594754, 8.202189375375613878, -0.7076125000919450958 ) ) ;
#20189=CARTESIAN_POINT ( 'NONE',  ( 4.634908411025333130, 6.500755460986618495, 1.599625672291268286 ) ) ;
#20196=CARTESIAN_POINT ( 'NONE',  ( -5.399890319992785237, 9.521898816625391504, 0.7998128361456291469 ) ) ;
#20199=ORIENTED_EDGE ( 'NONE', *, *, #58752, .T. ) ;
#20208=CARTESIAN_POINT ( 'NONE',  ( 4.041739190205284160, 7.729463131965888856, 0.000000000000000000 ) ) ;
#20211=CARTESIAN_POINT ( 'NONE',  ( 5.478903473698239601, 7.485416367438324059, -1.443375672974078761 ) ) ;
#20214=CARTESIAN_POINT ( 'NONE',  ( -4.288121723672178476, 8.224835454251337552, -0.7998128361456362523 ) ) ;
#20226=CARTESIAN_POINT ( 'NONE',  ( 4.228163802615382494, 6.026220084508304708, -1.599625672291269396 ) ) ;
#20227=CARTESIAN_POINT ( 'NONE',  ( 5.794130544993763898, 7.853181283949808744, 1.599625672291269396 ) ) ;
#20248=CARTESIAN_POINT ( 'NONE',  ( 6.170730229783032428, 7.061345527190763249, -1.063955632616358615 ) ) ;
#20251=AXIS2_PLACEMENT_3D ( 'NONE', #124707, #190666, #42326 ) ;
#20257=CARTESIAN_POINT ( 'NONE',  ( 4.167152111353856547, 5.955039778036558040, 1.599625672291262513 ) ) ;
#20263=CARTESIAN_POINT ( 'NONE',  ( 4.667750024854814050, 8.667735138964429709, -0.7998128361456381397 ) ) ;
#20268=CARTESIAN_POINT ( 'NONE',  ( 4.828112100242277549, 6.726159765073026264, -1.443375672974068769 ) ) ;
#20271=CARTESIAN_POINT ( 'NONE',  ( 7.838022202476093270, 8.316983122409855156, 0.7216878364870267237 ) ) ;
#20284=CARTESIAN_POINT ( 'NONE',  ( 6.450676980830294838, 6.774405823990504949, -0.3487213023658369826 ) ) ;
#20285=CARTESIAN_POINT ( 'NONE',  ( -6.943184063974175757, 9.193743722760251202, -1.443375672974066548 ) ) ;
#20293=CARTESIAN_POINT ( 'NONE',  ( -0.1010051578917390280, 3.387064998577566488, -1.997555336163420181 ) ) ;
#20310=CARTESIAN_POINT ( 'NONE',  ( 3.879041346841291649, 7.539648981374564407, 1.040834085586084257E-14 ) ) ;
#20319=CARTESIAN_POINT ( 'NONE',  ( 4.844006021832467646, 8.873367135438366304, 0.000000000000000000 ) ) ;
#20321=CARTESIAN_POINT ( 'NONE',  ( 6.658989722967328717, 7.797851427330578566, 1.199719254218452935 ) ) ;
#20323=CYLINDRICAL_SURFACE ( 'NONE', #199735, 1.250000000000000000 ) ;
#20334=CARTESIAN_POINT ( 'NONE',  ( -5.743814354044916470, 6.730146830254374990, -1.199719254218453823 ) ) ;
#20336=CARTESIAN_POINT ( 'NONE',  ( 6.333067150914816423, 7.521571443223021625, 1.082531754730549967 ) ) ;
#20339=B_SPLINE_CURVE_WITH_KNOTS ( 'NONE', 3,
 ( #109728, #97692, #113999, #159470, #43610, #195179, #63035, #110788, #7051, #139227 ),
 .UNSPECIFIED., .F., .F.,
 ( 4, 3, 3, 4 ),
 ( 7.620576258561039861E-17, 9.102628012183976516E-05, 0.0001374522152767717893, 0.0001846341747205655518 ),
 .UNSPECIFIED. ) ;
#20346=CARTESIAN_POINT ( 'NONE',  ( -5.307090785106547415, 5.156303768904543894, -0.7998128361456362523 ) ) ;
#20347=CIRCLE ( 'NONE', #141481, 0.07999999999999968248 ) ;
#20353=CARTESIAN_POINT ( 'NONE',  ( -7.160114521792834807, 8.486460042580672436, 1.082531754730549078 ) ) ;
#20355=CARTESIAN_POINT ( 'NONE',  ( -6.644904684473536882, 6.925012684740138980, 0.7216878364870317197 ) ) ;
#20363=CARTESIAN_POINT ( 'NONE',  ( 0.2375137461210129197, 3.335658684549960284, 2.061805365461736983 ) ) ;
#20366=EDGE_CURVE ( 'NONE', #39859, #52099, #159104, .T. ) ;
#20379=CARTESIAN_POINT ( 'NONE',  ( -5.631432701629818460, 7.663367133358481631, 1.599625672291263179 ) ) ;
#20382=CARTESIAN_POINT ( 'NONE',  ( -4.679499295372141709, 5.488445928469455559, 1.199719254218452935 ) ) ;
#20390=CARTESIAN_POINT ( 'NONE',  ( -4.648357846327917819, 8.420182996469929293, -0.5132882116619559287 ) ) ;
#20422=CARTESIAN_POINT ( 'NONE',  ( 5.194709132691408549, 6.089524072008651423, 1.199719254218452935 ) ) ;
#20429=CARTESIAN_POINT ( 'NONE',  ( 5.254667053748194760, 8.288139441751686931, 1.199719254218452047 ) ) ;
#20431=CARTESIAN_POINT ( 'NONE',  ( 5.367048706163317640, 7.354919138647580290, -1.599625672291281386 ) ) ;
#20445=CARTESIAN_POINT ( 'NONE',  ( 5.364009635805341958, 7.578432035813580825, -1.241402483855597039 ) ) ;
#20447=CARTESIAN_POINT ( 'NONE',  ( -6.251718229232857915, 7.426664367927358512, -1.082531754730549967 ) ) ;
#20448=CARTESIAN_POINT ( 'NONE',  ( 4.231553341240963384, 7.950912974840849579, -0.7216878364870357165 ) ) ;
#20456=CARTESIAN_POINT ( 'NONE',  ( -3.634467696915153034, 6.397906858779740524, 1.199719254218452935 ) ) ;
#20465=CARTESIAN_POINT ( 'NONE',  ( -5.492461626867567226, 6.540864998501174199, 1.082531754730549078 ) ) ;
#20470=CARTESIAN_POINT ( 'NONE',  ( 5.668190738965027897, 8.770583741171307679, -1.199719254218452047 ) ) ;
#20499=CARTESIAN_POINT ( 'NONE',  ( 5.830888582329017744, 8.960397891762626799, -1.199719254218452047 ) ) ;
#20503=B_SPLINE_CURVE_WITH_KNOTS ( 'NONE', 3,
 ( #65623, #211896, #164231, #195671, #197776, #49414, #181529, #128623, #45172, #165287 ),
 .UNSPECIFIED., .F., .F.,
 ( 4, 3, 3, 4 ),
 ( 3.263880750628924922E-18, 3.125190611472425774E-05, 6.297331589974846625E-05, 6.656384948891156620E-05 ),
 .UNSPECIFIED. ) ;
#20508=VECTOR ( 'NONE', #40218, 1000.000000000000000 ) ;
#20511=CARTESIAN_POINT ( 'NONE',  ( -3.000121558099561270, 6.395101958814021437, -0.7378544084795432001 ) ) ;
#20513=CARTESIAN_POINT ( 'NONE',  ( 1.854512760316388897, 2.488359591189891251, 2.484105960264901825 ) ) ;
#20517=ADVANCED_FACE ( 'NONE', ( #55265 ), #147730, .T. ) ;
#20521=CARTESIAN_POINT ( 'NONE',  ( -5.181866634007240791, 6.340624232048664766, 1.284222742053082733 ) ) ;
#20523=FACE_OUTER_BOUND ( 'NONE', #146390, .T. ) ;
#20530=ORIENTED_EDGE ( 'NONE', *, *, #114198, .F. ) ;
#20531=CARTESIAN_POINT ( 'NONE',  ( 4.095971805104288599, 5.871996087412059140, 1.443375672974058777 ) ) ;
#20538=CARTESIAN_POINT ( 'NONE',  ( 6.013923656113508542, 9.173938811177871244, -1.199719254218452047 ) ) ;
#20541=CARTESIAN_POINT ( 'NONE',  ( -3.038435823238377687, 6.558942537171132514, -0.7216878364870458196 ) ) ;
#20551=CARTESIAN_POINT ( 'NONE',  ( 3.840479349152599919, 7.346192795665340114, 0.4818892653144311033 ) ) ;
#20554=AXIS2_PLACEMENT_3D ( 'NONE', #197162, #210207, #180915 ) ;
#20560=CARTESIAN_POINT ( 'NONE',  ( 5.996449078994045223, 10.21788403546024782, 0.7998128361456331437 ) ) ;
#20569=CARTESIAN_POINT ( 'NONE',  ( 4.523580528814945545, 5.306540700819438960, 1.199719254218452047 ) ) ;
#20571=DIRECTION ( 'NONE',  ( 0.000000000000000000, 0.000000000000000000, 1.000000000000000000 ) ) ;
#20581=CARTESIAN_POINT ( 'NONE',  ( -5.397554552016258889, 7.390509292142662723, 1.443375672974058777 ) ) ;
#20583=CARTESIAN_POINT ( 'NONE',  ( 6.713222337422018349, 7.861122810861019161, -1.199719254218452047 ) ) ;
#20588=CARTESIAN_POINT ( 'NONE',  ( -3.156015896931072540, 6.904045323053366268, 0.000000000000000000 ) ) ;
#20599=CARTESIAN_POINT ( 'NONE',  ( -5.361443639997861332, 4.701392137926268866, 2.440314829665658714 ) ) ;
#20603=CARTESIAN_POINT ( 'NONE',  ( 3.861425177953237142, 7.342474422772079734, -0.7004879694037218218 ) ) ;
#20629=CARTESIAN_POINT ( 'NONE',  ( -6.469175572376043348, 7.576401584974034265, 1.199719254218452047 ) ) ;
#20633=CARTESIAN_POINT ( 'NONE',  ( -4.447956913735107598, 7.346977611736363656, 1.199719254218452935 ) ) ;
#20637=CARTESIAN_POINT ( 'NONE',  ( -6.089020385868867180, 7.236850217336030511, -1.082531754730549967 ) ) ;
#20643=CARTESIAN_POINT ( 'NONE',  ( -6.936931872047518155, 8.122117267924091166, 1.199719254218452047 ) ) ;
#20651=CARTESIAN_POINT ( 'NONE',  ( -6.607619761813764647, 8.802252036906432764, 1.599625672291269396 ) ) ;
#20653=CARTESIAN_POINT ( 'NONE',  ( 4.595450297557979624, 8.489593704440707711, 0.02661077391274621617 ) ) ;
#20658=CARTESIAN_POINT ( 'NONE',  ( 6.831329296439236032, 9.063246493969506545, -1.599625672291267398 ) ) ;
#20683=CARTESIAN_POINT ( 'NONE',  ( 7.517069824134078537, 7.734612647770044092, 0.000000000000000000 ) ) ;
#20697=CARTESIAN_POINT ( 'NONE',  ( 5.348589505275513467, 7.707351500233518671, -1.315919829448284784 ) ) ;
#20723=CARTESIAN_POINT ( 'NONE',  ( -6.579637281422358264, 6.781222396613637571, 0.3437121870633503828 ) ) ;
#20741=CARTESIAN_POINT ( 'NONE',  ( -5.276058054373441664, 6.184431147304315424, -1.199719254218453823 ) ) ;
#20752=ORIENTED_EDGE ( 'NONE', *, *, #159680, .F. ) ;
#20758=ORIENTED_EDGE ( 'NONE', *, *, #118802, .T. ) ;
#20760=CARTESIAN_POINT ( 'NONE',  ( 3.410758162289653672, 6.136912401716668519, -1.199719254218453823 ) ) ;
#20762=CARTESIAN_POINT ( 'NONE',  ( 6.821160681006781523, 9.051383109298340557, 1.443375672974063439 ) ) ;
#20773=CARTESIAN_POINT ( 'NONE',  ( -5.261446130555064826, 8.296048364692991228, 1.199719254218452935 ) ) ;
#20775=CARTESIAN_POINT ( 'NONE',  ( 6.204791576909545192, 7.267953590263130259, -1.199719254218452047 ) ) ;
#20778=ADVANCED_FACE ( 'NONE', ( #112608 ), #44357, .F. ) ;
#20786=CARTESIAN_POINT ( 'NONE',  ( -3.820365424000704557, 7.679119771301277098, -0.7998128361456481317 ) ) ;
#20787=CARTESIAN_POINT ( 'NONE',  ( 4.598150373690133463, 5.393538853173795111, -1.199719254218452047 ) ) ;
#20794=CARTESIAN_POINT ( 'NONE',  ( 5.742760583840166966, 8.857581893525663830, 1.199719254218452047 ) ) ;
#20799=CARTESIAN_POINT ( 'NONE',  ( -4.636310691425048702, 8.434871236368708836, 0.4628797641644845084 ) ) ;
#20810=CARTESIAN_POINT ( 'NONE',  ( -3.811250578772977349, 7.460559751961507224, -0.7216878364870458196 ) ) ;
#20819=CARTESIAN_POINT ( 'NONE',  ( 3.445180431648323882, 6.073108699348104267, 1.082531754730549078 ) ) ;
#20822=CARTESIAN_POINT ( 'NONE',  ( -6.611536185319534908, 7.742488966741438716, 1.199719254218452047 ) ) ;
#20825=ORIENTED_EDGE ( 'NONE', *, *, #205051, .T. ) ;
#20827=CARTESIAN_POINT ( 'NONE',  ( 4.260029445439558415, 7.236136616047151193, -2.499999999999996891 ) ) ;
#20834=CARTESIAN_POINT ( 'NONE',  ( 3.088225128862704949, 6.824956093640315302, 0.7998128361456281477 ) ) ;
#20838=CARTESIAN_POINT ( 'NONE',  ( 4.766573523656222555, 7.718696989977711809, 1.199719254218452047 ) ) ;
#20859=CARTESIAN_POINT ( 'NONE',  ( 5.716698046817569434, 6.698511138489155137, -1.199719254218452047 ) ) ;
#20860=CARTESIAN_POINT ( 'NONE',  ( -4.665414256878293031, 7.496714828783040296, -1.082531754730549967 ) ) ;
#20882=CARTESIAN_POINT ( 'NONE',  ( -6.038177310039794854, 8.137902509836795417, -1.599625672291271394 ) ) ;
#20884=CARTESIAN_POINT ( 'NONE',  ( 5.817857313595521163, 9.801600942587855414, -0.7216878364870458196 ) ) ;
#20897=CARTESIAN_POINT ( 'NONE',  ( -7.286581212701773502, 7.465709267765667789, 0.7998128361456341429 ) ) ;
#20904=CARTESIAN_POINT ( 'NONE',  ( 5.076602173674213070, 4.887400388900169368, 0.000000000000000000 ) ) ;
#20908=EDGE_CURVE ( 'NONE', #30079, #175863, #158247, .T. ) ;
#20911=CARTESIAN_POINT ( 'NONE',  ( -7.045397100956844127, 8.248660034984974132, -1.199719254218452047 ) ) ;
#20914=CARTESIAN_POINT ( 'NONE',  ( -3.623772196602547346, 7.449761006003425834, 0.000000000000000000 ) ) ;
#20918=CARTESIAN_POINT ( 'NONE',  ( 3.404505970362959655, 6.986024375483197879, 0.7216878364870257245 ) ) ;
#20919=CARTESIAN_POINT ( 'NONE',  ( -5.438229012412903352, 6.477593614970734492, -1.082531754730549967 ) ) ;
#20924=CARTESIAN_POINT ( 'NONE',  ( -3.935609729716867289, 7.813571461303467913, 0.7998128361456350310 ) ) ;
#20938=CARTESIAN_POINT ( 'NONE',  ( 5.214490215732396017, 7.828485850976955263, 1.269369371331245500 ) ) ;
#20942=CARTESIAN_POINT ( 'NONE',  ( 0.4208425991348082040, 2.777615014373102653, 1.955394415493260984 ) ) ;
#20947=CARTESIAN_POINT ( 'NONE',  ( 7.374709211190586089, 7.568525266002632534, 0.000000000000000000 ) ) ;
#20957=CARTESIAN_POINT ( 'NONE',  ( 5.654245663017247736, 7.339362581565530341, 1.229167601055790815 ) ) ;
#20976=CARTESIAN_POINT ( 'NONE',  ( -5.468734858265826837, 7.473552982767158070, 1.599625672291263179 ) ) ;
#20989=CARTESIAN_POINT ( 'NONE',  ( 6.249382461256315580, 6.255644057745969988, -0.7998128361456481317 ) ) ;
#21001=CARTESIAN_POINT ( 'NONE',  ( 4.380693030546913391, 7.164540064729805202, 1.082531754730549078 ) ) ;
#21007=CARTESIAN_POINT ( 'NONE',  ( -8.014278199453791274, 8.522615118883788199, 1.530808498934192557E-16 ) ) ;
#21014=CARTESIAN_POINT ( 'NONE',  ( -6.699137298928187434, 8.909022496873262753, 1.443375672974064550 ) ) ;
#21015=CARTESIAN_POINT ( 'NONE',  ( 6.129694847154206983, 8.244672969803623630, -1.443375672974078761 ) ) ;
#21027=CARTESIAN_POINT ( 'NONE',  ( -5.418418667316934112, 6.350518529071726981, -1.199719254218453823 ) ) ;
#21028=CARTESIAN_POINT ( 'NONE',  ( -3.135678666510573365, 6.880318554229450712, 0.000000000000000000 ) ) ;
#21030=CARTESIAN_POINT ( 'NONE',  ( 5.763624699140868834, 7.817591130454727200, -1.443375672974078761 ) ) ;
#21038=CARTESIAN_POINT ( 'NONE',  ( -4.623560037311160720, 8.450214339770131033, 0.4765305399337668169 ) ) ;
#21043=CARTESIAN_POINT ( 'NONE',  ( -4.617805310829839804, 8.366410568267871994, -0.2388493967704352627 ) ) ;
#21050=CARTESIAN_POINT ( 'NONE',  ( -6.306477729012051725, 7.386587434382707151, 1.199719254218452047 ) ) ;
#21062=CARTESIAN_POINT ( 'NONE',  ( 6.540882763950133238, 6.595727744222092959, 0.000000000000000000 ) ) ;
#21075=DIRECTION ( 'NONE',  ( -0.6507913734559658270, -0.7592566023652989049, 0.000000000000000000 ) ) ;
#21097=CARTESIAN_POINT ( 'NONE',  ( 6.102578539926878598, 7.252668063737060855, -1.082531754730548412 ) ) ;
#21101=CARTESIAN_POINT ( 'NONE',  ( 6.712695452097489301, 7.964471127936110229, -1.082531754730548412 ) ) ;
#21115=CARTESIAN_POINT ( 'NONE',  ( -7.605197822622922210, 7.837428646007010613, -0.7998128361456362523 ) ) ;
#21127=B_SPLINE_CURVE_WITH_KNOTS ( 'NONE', 3,
 ( #86496, #55071, #70218, #5209, #100609, #69150, #199151, #187189, #119059, #151512, #201284, #37749, #185042, #38818, #136329, #85426 ),
 .UNSPECIFIED., .F., .F.,
 ( 4, 3, 3, 3, 3, 4 ),
 ( 0.000000000000000000, 3.083448363908645134E-05, 6.173412828017592617E-05, 9.147751612222104365E-05, 0.0001189036761826361657, 0.0001300740652511593631 ),
 .UNSPECIFIED. ) ;
#21129=CARTESIAN_POINT ( 'NONE',  ( 4.868786560638889149, 6.773613302202437403, 1.443375672974065660 ) ) ;
#21136=CARTESIAN_POINT ( 'NONE',  ( -5.191846479390389568, 5.021852078902356631, 0.7998128361456281477 ) ) ;
#21141=CARTESIAN_POINT ( 'NONE',  ( -6.075462232699549325, 9.141770800574526845, 1.082531754730549967 ) ) ;
#21144=CARTESIAN_POINT ( 'NONE',  ( -7.937372586157736443, 8.224965870130965584, 0.7998128361456341429 ) ) ;
#21164=CARTESIAN_POINT ( 'NONE',  ( -5.831415467653581430, 5.975941931783510519, 0.7216878364870257245 ) ) ;
#21166=CARTESIAN_POINT ( 'NONE',  ( -5.031484404002922517, 6.963427452793760963, 1.443375672974058777 ) ) ;
#21168=CARTESIAN_POINT ( 'NONE',  ( 3.725458348705031231, 7.568394850123006279, -1.734723475976807094E-15 ) ) ;
#21169=CARTESIAN_POINT ( 'NONE',  ( -5.224688093219839402, 7.188831756880171397, -1.599625672291271394 ) ) ;
#21170=CARTESIAN_POINT ( 'NONE',  ( -6.903036488013351679, 8.082572653217566128, -1.199719254218452047 ) ) ;
#21218=DIRECTION ( 'NONE',  ( -0.6292706268317957985, 0.7771862570881697962, 0.000000000000000000 ) ) ;
#21227=CARTESIAN_POINT ( 'NONE',  ( 5.224688093219824303, 7.188831756880171397, -1.599625672291283607 ) ) ;
#21243=CARTESIAN_POINT ( 'NONE',  ( 5.554000203453580475, 6.508696987897830688, -1.199719254218452047 ) ) ;
#21249=CARTESIAN_POINT ( 'NONE',  ( -6.720001414228860881, 7.869031733802326123, -1.199719254218452047 ) ) ;
#21254=CARTESIAN_POINT ( 'NONE',  ( 5.923986774528332333, 5.876015756563318426, -0.7998128361456481317 ) ) ;
#21266=CARTESIAN_POINT ( 'NONE',  ( 5.885648082108199119, 6.999582529615296700, 1.082531754730549967 ) ) ;
#21268=CARTESIAN_POINT ( 'NONE',  ( -4.258669648468323743, 6.061810238003387141, 1.443375672974065660 ) ) ;
#21269=CARTESIAN_POINT ( 'NONE',  ( -4.749098946536820520, 8.762642214260091933, 0.7998128361456281477 ) ) ;
#21276=ORIENTED_EDGE ( 'NONE', *, *, #91128, .T. ) ;
#21281=CARTESIAN_POINT ( 'NONE',  ( 4.203910148689107729, 7.062256385849379647, -1.199719254218448494 ) ) ;
#21282=CARTESIAN_POINT ( 'NONE',  ( 6.900173834712277632, 7.014900660111269559, -0.7998128361456341429 ) ) ;
#21302=CARTESIAN_POINT ( 'NONE',  ( 5.092389439195339484, 7.944299729584391123, -1.199137415704543130 ) ) ;
#21305=DIRECTION ( 'NONE',  ( 0.000000000000000000, 1.000000000000000000, 0.000000000000000000 ) ) ;
#21311=CARTESIAN_POINT ( 'NONE',  ( 5.734172623936983904, 5.654565914206774124, 0.7998128361456352531 ) ) ;
#21315=CARTESIAN_POINT ( 'NONE',  ( 6.156284269057003655, 9.340026192945279249, -1.199719254218452047 ) ) ;
#21320=CARTESIAN_POINT ( 'NONE',  ( 6.427974226654860956, 7.632296364919712417, -1.082531754730548412 ) ) ;
#21323=CARTESIAN_POINT ( 'NONE',  ( 5.076602173674213070, 4.887400388900169368, 0.000000000000000000 ) ) ;
#21335=CARTESIAN_POINT ( 'NONE',  ( 6.477827756726281194, 6.756902019748111776, -0.2091553196570776485 ) ) ;
#21336=CARTESIAN_POINT ( 'NONE',  ( -4.309512724297390740, 6.121127159803966933, 1.599625672291270506 ) ) ;
#21343=CARTESIAN_POINT ( 'NONE',  ( 0.3337279542187601145, 3.354361423484768956, -1.974754334845483905 ) ) ;
#21345=( BOUNDED_CURVE ( )  B_SPLINE_CURVE ( 2, ( #130753, #179444, #196747, #32115, #14777, #180498, #68844 ),
 .UNSPECIFIED., .F., .T. ) 
 B_SPLINE_CURVE_WITH_KNOTS ( ( 3, 2, 2, 3 ),
 ( 0.2749999999999999112, 0.2833333333333333259, 0.2916666666666667962, 0.3000000000000002109 ),
 .UNSPECIFIED. ) 
 CURVE ( )  GEOMETRIC_REPRESENTATION_ITEM ( )  RATIONAL_B_SPLINE_CURVE ( ( 1.000000000000001776, 0.8660254037844369313, 1.000000000000000000, 0.8660254037844387076, 1.000000000000000000, 0.8660254037844351549, 1.000000000000003553 ) ) 
 REPRESENTATION_ITEM ( '' )  );
#21370=CARTESIAN_POINT ( 'NONE',  ( 6.261886844665240481, 8.398896966899865646, 1.599625672291268286 ) ) ;
#21372=CARTESIAN_POINT ( 'NONE',  ( 5.040599249230596435, 9.102725900736217568, 0.7998128361456341429 ) ) ;
#21386=CARTESIAN_POINT ( 'NONE',  ( -5.971440312176176768, 5.931378217152456500, 0.000000000000000000 ) ) ;
#21388=CARTESIAN_POINT ( 'NONE',  ( 5.519577934094851202, 8.493239118869080784, 1.082531754730547524 ) ) ;
#21398=CARTESIAN_POINT ( 'NONE',  ( -3.623772196602547346, 7.449761006003425834, 0.000000000000000000 ) ) ;
#21401=CARTESIAN_POINT ( 'NONE',  ( -3.526529353330355221, 6.168015774643768268, -1.082531754730546636 ) ) ;
#21404=CARTESIAN_POINT ( 'NONE',  ( -3.797165540279144214, 6.587721009371067638, 1.199719254218452935 ) ) ;
#21406=CARTESIAN_POINT ( 'NONE',  ( -6.021229618244897885, 7.157760988441397743, 1.082531754730548412 ) ) ;
#21428=CARTESIAN_POINT ( 'NONE',  ( -5.173318132066234476, 8.193232366456022930, -1.199719254218453823 ) ) ;
#21430=CARTESIAN_POINT ( 'NONE',  ( -3.006876207180748217, 6.730049018344652190, -0.7998128361456481317 ) ) ;
#21439=CARTESIAN_POINT ( 'NONE',  ( -6.265495719280979259, 6.992744598377811371, -0.9808356887253886214 ) ) ;
#21454=EDGE_CURVE ( 'NONE', #78850, #29771, #5245, .T. ) ;
#21469=CARTESIAN_POINT ( 'NONE',  ( 5.598591087800349086, 5.496387455380669529, -0.7998128361456481317 ) ) ;
#21477=CARTESIAN_POINT ( 'NONE',  ( 6.984385409695311964, 8.177479728513226576, 1.199719254218452935 ) ) ;
#21479=CARTESIAN_POINT ( 'NONE',  ( 5.505492895601038938, 8.580769590579979678, -1.199719254218452047 ) ) ;
#21492=CARTESIAN_POINT ( 'NONE',  ( 6.292946923374557855, 6.878031543426355476, -0.7329977330566839200 ) ) ;
#21494=CARTESIAN_POINT ( 'NONE',  ( -6.902509602688830626, 7.225551755991315162, -0.7216878364870338292 ) ) ;
#21495=CARTESIAN_POINT ( 'NONE',  ( 6.048345925472191631, 6.229027465905275562, 0.7216878364870328300 ) ) ;
#21507=CARTESIAN_POINT ( 'NONE',  ( 0.2248163340835918345, 3.434981140918095477, -1.989104691395113367 ) ) ;
#21510=CARTESIAN_POINT ( 'NONE',  ( -5.438229012412899799, 7.437962829272074750, -1.443375672974066548 ) ) ;
#21514=CARTESIAN_POINT ( 'NONE',  ( 5.182959862174088883, 9.268813282503625572, 0.7998128361456331437 ) ) ;
#21541=CARTESIAN_POINT ( 'NONE',  ( -3.791842586888578559, 7.437917094763062842, 0.3113814200439020130 ) ) ;
#21573=CARTESIAN_POINT ( 'NONE',  ( 5.424670859243587273, 5.501406555305196733, -0.7216878364870458196 ) ) ;
#21580=CARTESIAN_POINT ( 'NONE',  ( 7.374709211190586089, 7.568525266002632534, 0.000000000000000000 ) ) ;
#21584=CARTESIAN_POINT ( 'NONE',  ( -4.746763178560296836, 6.631252689777363152, 1.443375672974058777 ) ) ;
#21588=AXIS2_PLACEMENT_3D ( 'NONE', #144020, #157042, #41164 ) ;
#21613=CARTESIAN_POINT ( 'NONE',  ( 7.526184669361807522, 7.953172667109813077, 0.000000000000000000 ) ) ;
#21626=CARTESIAN_POINT ( 'NONE',  ( -4.990809943606273613, 7.876343129965691858, -1.082531754730549967 ) ) ;
#21628=CARTESIAN_POINT ( 'NONE',  ( 7.700104897918568447, 7.948153567185284096, 0.000000000000000000 ) ) ;
#21633=CARTESIAN_POINT ( 'NONE',  ( -5.492988512192097161, 6.437516681426083132, 1.199719254218452935 ) ) ;
#21679=CARTESIAN_POINT ( 'NONE',  ( -6.631873415740034083, 7.766215735565355160, 1.199719254218452047 ) ) ;
#21683=CARTESIAN_POINT ( 'NONE',  ( -5.204350862799341115, 7.165104988056252289, -1.599625672291271394 ) ) ;
#21684=CARTESIAN_POINT ( 'NONE',  ( -3.969505113751027547, 7.853116076009993840, 1.214306433183764966E-14 ) ) ;
#21688=CARTESIAN_POINT ( 'NONE',  ( -5.763624699140868834, 9.738329559057408602, -0.7216878364870338292 ) ) ;
#21693=EDGE_LOOP ( 'NONE', ( #104758, #54905, #191283, #98116 ) ) ;
#21694=CARTESIAN_POINT ( 'NONE',  ( -5.901542003698421190, 10.10715911428198055, 0.000000000000000000 ) ) ;
#21702=CARTESIAN_POINT ( 'NONE',  ( -7.391130018105325661, 8.652015104991543026, -1.199719254218452047 ) ) ;
#21704=CARTESIAN_POINT ( 'NONE',  ( 4.710809438828709617, 8.349644928513606956, 0.6747337923850562635 ) ) ;
#21710=CARTESIAN_POINT ( 'NONE',  ( 5.032011289327418702, 5.899709921417326974, 1.199719254218452935 ) ) ;
#21722=CARTESIAN_POINT ( 'NONE',  ( -6.505933609711270549, 8.683618192786854095, -1.599625672291271394 ) ) ;
#21723=EDGE_CURVE ( 'NONE', #34262, #135468, #169100, .T. ) ;
#21736=CARTESIAN_POINT ( 'NONE',  ( 7.289443866002793371, 8.533381260871966134, 1.199719254218452047 ) ) ;
#21751=CARTESIAN_POINT ( 'NONE',  ( 5.997720278586790243, 7.186234674792547850, 1.197368251494409286 ) ) ;
#21776=CARTESIAN_POINT ( 'NONE',  ( -6.111218785694742195, 7.101581614182197022, 1.130138924470771800 ) ) ;
#21796=CARTESIAN_POINT ( 'NONE',  ( -4.118644803501354978, 8.027112380718707030, 0.7998128361456352531 ) ) ;
#21804=CARTESIAN_POINT ( 'NONE',  ( 4.318600669050608687, 4.999583595936801572, -2.499999999999996891 ) ) ;
#21807=ORIENTED_EDGE ( 'NONE', *, *, #70875, .F. ) ;
#21815=CARTESIAN_POINT ( 'NONE',  ( 4.760848217054122422, 5.583353003765119560, -1.199719254218452047 ) ) ;
#21830=CARTESIAN_POINT ( 'NONE',  ( 6.866278450678116485, 6.975356045404744521, 0.000000000000000000 ) ) ;
#21838=ORIENTED_EDGE ( 'NONE', *, *, #8484, .F. ) ;
#21840=CARTESIAN_POINT ( 'NONE',  ( -4.305596300791617814, 7.180890229968955651, 1.199719254218452935 ) ) ;
#21841=CARTESIAN_POINT ( 'NONE',  ( 7.828907357248368726, 8.098423103070084395, 0.7998128361456281477 ) ) ;
#21845=CARTESIAN_POINT ( 'NONE',  ( -4.911796789900812144, 8.952456364851418158, 0.7998128361456291469 ) ) ;
#21849=CARTESIAN_POINT ( 'NONE',  ( 5.851225812749518695, 8.984124660586543243, -1.199719254218452047 ) ) ;
#21854=CARTESIAN_POINT ( 'NONE',  ( -4.585403371929053229, 8.498043419817562949, 0.04945426522169442396 ) ) ;
#21864=CARTESIAN_POINT ( 'NONE',  ( -5.763624699140894592, 5.896852701852039580, -0.7216878364870338292 ) ) ;
#21875=CARTESIAN_POINT ( 'NONE',  ( 2.957086901556340575, 6.464035461875470290, 0.7216878364870257245 ) ) ;
#21879=CARTESIAN_POINT ( 'NONE',  ( -6.231907884136888676, 7.299589282028351001, -1.199719254218453823 ) ) ;
#21917=CARTESIAN_POINT ( 'NONE',  ( -6.156811154381562012, 6.355570232966157640, 0.7216878364870257245 ) ) ;
#21920=( BOUNDED_CURVE ( )  B_SPLINE_CURVE ( 2, ( #67281, #19619, #151779, #200490, #132359, #101949, #4410 ),
 .UNSPECIFIED., .F., .T. ) 
 B_SPLINE_CURVE_WITH_KNOTS ( ( 3, 2, 2, 3 ),
 ( 0.4499999999999999556, 0.4583333333333331483, 0.4666666666666663965, 0.4749999999999995892 ),
 .UNSPECIFIED. ) 
 CURVE ( )  GEOMETRIC_REPRESENTATION_ITEM ( )  RATIONAL_B_SPLINE_CURVE ( ( 1.000000000000000888, 0.8660254037844378194, 1.000000000000000000, 0.8660254037844387076, 1.000000000000000000, 0.8660254037844449249, 0.9999999999999937828 ) ) 
 REPRESENTATION_ITEM ( '' )  );
#21942=CARTESIAN_POINT ( 'NONE',  ( -5.433785704026946384, 9.561443431331920095, 0.000000000000000000 ) ) ;
#21948=CARTESIAN_POINT ( 'NONE',  ( -5.659602779061863487, 5.567567761852417085, 0.7998128361456281477 ) ) ;
#21959=CARTESIAN_POINT ( 'NONE',  ( -5.029148636026397945, 4.832037928311032182, 0.7998128361456281477 ) ) ;
#21965=CARTESIAN_POINT ( 'NONE',  ( 4.529305835417093640, 7.441884687032027657, -1.199719254218450271 ) ) ;
#21970=CARTESIAN_POINT ( 'NONE',  ( -7.273023059088104425, 7.449891421883056530, 0.000000000000000000 ) ) ;
#21973=CARTESIAN_POINT ( 'NONE',  ( -4.821859908315634158, 5.654533310236863564, 1.199719254218452935 ) ) ;
#21977=CARTESIAN_POINT ( 'NONE',  ( 5.614485009834906393, 6.683225611963085733, -1.082531754730548412 ) ) ;
#21978=CARTESIAN_POINT ( 'NONE',  ( 4.462041952228939401, 6.299077925724123617, -1.443375672974068769 ) ) ;
#21979=CARTESIAN_POINT ( 'NONE',  ( -4.462041952228944730, 7.259447140025469203, -1.082531754730549967 ) ) ;
#21994=CARTESIAN_POINT ( 'NONE',  ( 3.881377115262160782, 7.750300077773022878, 0.7998128361456271485 ) ) ;
#21999=CARTESIAN_POINT ( 'NONE',  ( 5.901825473515108555, 7.257632781371366804, 1.250113620240392631 ) ) ;
#22004=CARTESIAN_POINT ( 'NONE',  ( -5.000000000000013323, 11.39843543023555661, 0.7750000000000004663 ) ) ;
#22009=CARTESIAN_POINT ( 'NONE',  ( 6.363572996767764778, 8.517530811019446091, -1.599625672291283607 ) ) ;
#22019=CARTESIAN_POINT ( 'NONE',  ( 6.400493444083267036, 6.807005473012165631, 0.5116258143813920967 ) ) ;
#22033=CARTESIAN_POINT ( 'NONE',  ( 4.207966135563082410, 7.175396087857922822, -1.043745235818753780 ) ) ;
#22036=CARTESIAN_POINT ( 'NONE',  ( -5.336015975430226099, 8.383046517047350932, -1.199719254218453823 ) ) ;
#22049=CARTESIAN_POINT ( 'NONE',  ( 7.035755370848908896, 7.173079118937375931, 0.7998128361456352531 ) ) ;
#22061=CARTESIAN_POINT ( 'NONE',  ( 5.221298554594243413, 5.264138866547622975, -0.7216878364870458196 ) ) ;
#22067=CARTESIAN_POINT ( 'NONE',  ( 3.179715765502636682, 5.975770656120749535, 2.499999999999999556 ) ) ;
#22071=ORIENTED_EDGE ( 'NONE', *, *, #40535, .T. ) ;
#22075=CARTESIAN_POINT ( 'NONE',  ( -5.966997003790221576, 9.015228033513643879, -1.082531754730549967 ) ) ;
#22076=CARTESIAN_POINT ( 'NONE',  ( 5.885648082108188461, 8.920320958217979879, 1.082531754730549967 ) ) ;
#22085=VERTEX_POINT ( 'NONE', #8419 ) ;
#22086=CARTESIAN_POINT ( 'NONE',  ( -5.743814354044916470, 6.730146830254374990, -1.199719254218453823 ) ) ;
#22087=CARTESIAN_POINT ( 'NONE',  ( -6.861835142292179057, 9.098836647464588978, 1.443375672974064550 ) ) ;
#22089=CARTESIAN_POINT ( 'NONE',  ( 6.983858524370782916, 7.320458831286981827, 0.7216878364870328300 ) ) ;
#22097=CARTESIAN_POINT ( 'NONE',  ( -5.911293591272317904, 7.247452768069575058, 1.263797332732160106 ) ) ;
#22101=CARTESIAN_POINT ( 'NONE',  ( -4.665006653791238911, 8.307176129776033591, 0.4851093158183654719 ) ) ;
#22105=EDGE_CURVE ( 'NONE', #186231, #53161, #20347, .T. ) ;
#22106=CARTESIAN_POINT ( 'NONE',  ( 5.560252395380215873, 6.619954228432645138, 1.082531754730549078 ) ) ;
#22110=CARTESIAN_POINT ( 'NONE',  ( -3.969505113751027547, 7.853116076009993840, 1.214306433183764966E-14 ) ) ;
#22123=CARTESIAN_POINT ( 'NONE',  ( 4.179656494762836516, 8.098292687190454586, -0.7998128361456362523 ) ) ;
#22159=CARTESIAN_POINT ( 'NONE',  ( 6.427974226654860956, 7.632296364919712417, -1.082531754730548412 ) ) ;
#22165=CARTESIAN_POINT ( 'NONE',  ( 6.495764994278809823, 7.711385593814346073, 1.082531754730549967 ) ) ;
#22168=CARTESIAN_POINT ( 'NONE',  ( -3.923301836239767137, 8.994671190470434397, 0.7749999999999996891 ) ) ;
#22182=CARTESIAN_POINT ( 'NONE',  ( -5.932574734431526942, 9.079031735882207244, 1.199719254218454489 ) ) ;
#22196=CARTESIAN_POINT ( 'NONE',  ( 5.383996397958233260, 5.453953017138946535, -0.7216878364870458196 ) ) ;
#22202=CARTESIAN_POINT ( 'NONE',  ( -3.871735385154307263, 6.674719161725423788, -1.199719254218450271 ) ) ;
#22207=CARTESIAN_POINT ( 'NONE',  ( -6.861835142292179057, 9.098836647464588978, 1.443375672974064550 ) ) ;
#22210=CARTESIAN_POINT ( 'NONE',  ( -5.752402313948099533, 9.933162809573264695, -0.7998128361456362523 ) ) ;
#22215=CARTESIAN_POINT ( 'NONE',  ( -4.930325137224961907, 5.781076077297750970, -1.199719254218453823 ) ) ;
#22229=CARTESIAN_POINT ( 'NONE',  ( -5.492461627311929995, 5.580495784718250363, 0.000000000000000000 ) ) ;
#22231=ORIENTED_EDGE ( 'NONE', *, *, #208628, .F. ) ;
#22232=CARTESIAN_POINT ( 'NONE',  ( -3.634994581795317536, 7.254927755487573293, 0.000000000000000000 ) ) ;
#22234=CARTESIAN_POINT ( 'NONE',  ( 5.387385936583818591, 7.378645907471495846, -1.599625672291283607 ) ) ;
#22236=CARTESIAN_POINT ( 'NONE',  ( -6.306477729012051725, 7.386587434382707151, 1.199719254218452047 ) ) ;
#22237=CARTESIAN_POINT ( 'NONE',  ( -7.119966945832006289, 8.335658187339330283, 1.199719254218452047 ) ) ;
#22238=CARTESIAN_POINT ( 'NONE',  ( -6.397211430516217767, 6.896709913541772430, -0.8587214783020010733 ) ) ;
#22239=EDGE_CURVE ( 'NONE', #36876, #213748, #164278, .T. ) ;
#22281=CARTESIAN_POINT ( 'NONE',  ( 7.065207446497155708, 9.336104335703744539, 0.000000000000000000 ) ) ;
#22284=CARTESIAN_POINT ( 'NONE',  ( 3.006787879153326681, 6.373552747333731006, -0.4818892653130519843 ) ) ;
#22292=CARTESIAN_POINT ( 'NONE',  ( 5.468734858265785093, 7.473552982767158070, 1.599625672291269396 ) ) ;
#22311=CARTESIAN_POINT ( 'NONE',  ( 3.881377115262159894, 7.750300077773022878, 0.7998128361456271485 ) ) ;
#22318=CARTESIAN_POINT ( 'NONE',  ( -6.129167961829681488, 9.308390501180058507, -1.199719254218452047 ) ) ;
#22322=VERTEX_POINT ( 'NONE', #163225 ) ;
#22323=CARTESIAN_POINT ( 'NONE',  ( 4.278479993564246797, 7.149254538203735798, 1.199719254218452047 ) ) ;
#22336=CARTESIAN_POINT ( 'NONE',  ( 7.851580356089786328, 8.332800968292465527, 0.000000000000000000 ) ) ;
#22337=CARTESIAN_POINT ( 'NONE',  ( -3.024877669624710386, 6.543124691288523920, 0.000000000000000000 ) ) ;
#22338=CARTESIAN_POINT ( 'NONE',  ( -6.622231685632140596, 6.690634819517756959, 0.000000000000000000 ) ) ;
#22352=CARTESIAN_POINT ( 'NONE',  ( 4.016958651398847557, 7.908478536599129249, -0.7998128361456362523 ) ) ;
#22353=CARTESIAN_POINT ( 'NONE',  ( 6.073126464278658432, 6.050012061272033392, 0.000000000000000000 ) ) ;
#22371=CARTESIAN_POINT ( 'NONE',  ( 5.620636616140949116, 7.477306742562066511, -1.332712173395997013 ) ) ;
#22382=CARTESIAN_POINT ( 'NONE',  ( 5.110497557708379546, 4.926945003606695295, -0.7998128361456481317 ) ) ;
#22387=CARTESIAN_POINT ( 'NONE',  ( 5.494797395288433250, 9.632623737803665875, 0.000000000000000000 ) ) ;
#22392=CARTESIAN_POINT ( 'NONE',  ( 4.556949027968946631, 8.330541276023501140, -0.7216878364870357165 ) ) ;
#22395=CARTESIAN_POINT ( 'NONE',  ( -6.143779885648060102, 7.196773283791382703, 1.199719254218452047 ) ) ;
#22397=CARTESIAN_POINT ( 'NONE',  ( 3.715816618597135523, 6.492813934075403637, -1.199719254218453823 ) ) ;
#22405=CARTESIAN_POINT ( 'NONE',  ( -5.731716152730447433, 6.325271568888634732, -0.8228651010004313093 ) ) ;
#22408=CARTESIAN_POINT ( 'NONE',  ( 6.426609430950597890, 6.789993649951097332, 0.4362094596595481599 ) ) ;
#22409=CARTESIAN_POINT ( 'NONE',  ( -7.322812365156824654, 8.676274193172000437, 1.082531754730549078 ) ) ;
#22443=CARTESIAN_POINT ( 'NONE',  ( 5.027041095616958444, 9.086908054853605421, 0.000000000000000000 ) ) ;
#22445=DIRECTION ( 'NONE',  ( -0.9629532593499512405, -0.2632023826131885680, 0.05869860385091355687 ) ) ;
#22458=CARTESIAN_POINT ( 'NONE',  ( -4.098307573080856692, 8.003385611894792362, 0.7998128361456352531 ) ) ;
#22460=CARTESIAN_POINT ( 'NONE',  ( 5.139949632912227173, 8.050339434155988627, -1.082531754730548412 ) ) ;
#22470=CARTESIAN_POINT ( 'NONE',  ( -6.120580001926503755, 6.105374521861167914, -0.7998128361456362523 ) ) ;
#22473=CARTESIAN_POINT ( 'NONE',  ( -2.862179826260718762, 6.353310540697199471, 0.000000000000000000 ) ) ;
#22477=CARTESIAN_POINT ( 'NONE',  ( -5.320648938720212051, 5.172121614787156929, 0.000000000000000000 ) ) ;
#22501=VERTEX_POINT ( 'NONE', #93976 ) ;
#22502=CARTESIAN_POINT ( 'NONE',  ( -5.061990249855848667, 6.999017606288844284, -1.599625672291271394 ) ) ;
#22528=CARTESIAN_POINT ( 'NONE',  ( -5.173318132066234476, 8.193232366456022930, -1.199719254218453823 ) ) ;
#22529=CARTESIAN_POINT ( 'NONE',  ( 5.345219749365309525, 4.708221922860561293, 2.500000000000000444 ) ) ;
#22537=CARTESIAN_POINT ( 'NONE',  ( 6.278834536460164983, 9.379038488295265097, -1.082531754730548412 ) ) ;
#22550=CARTESIAN_POINT ( 'NONE',  ( 3.223806664999388172, 6.983134552466421674, -0.7998128361456362523 ) ) ;
#22559=CARTESIAN_POINT ( 'NONE',  ( 6.119526231721748033, 8.232809585132461194, 1.599625672291269396 ) ) ;
#22561=CARTESIAN_POINT ( 'NONE',  ( 4.369470645354133431, 8.319742529546998000, 0.7998128361456271485 ) ) ;
#22565=CARTESIAN_POINT ( 'NONE',  ( -2.300257893000399623, 2.674526321726193867, -2.456405337815161793 ) ) ;
#22574=CARTESIAN_POINT ( 'NONE',  ( 6.457572779797339457, 6.769951385671206801, 0.3193968722623799494 ) ) ;
#22576=CARTESIAN_POINT ( 'NONE',  ( 4.746763178560241769, 8.551991118380046331, 0.7216878364870328300 ) ) ;
#22583=CARTESIAN_POINT ( 'NONE',  ( -2.959422669532919326, 6.674686557755516780, 0.7998128361456352531 ) ) ;
#22594=CARTESIAN_POINT ( 'NONE',  ( -4.462041952228942954, 8.219816354326809460, -0.7216878364870338292 ) ) ;
#22599=CARTESIAN_POINT ( 'NONE',  ( 6.855582950365507244, 8.027210192628430718, -1.199719254218452047 ) ) ;
#22614=CARTESIAN_POINT ( 'NONE',  ( -4.094259397040477033, 3.811769539471001167, -2.445515378722424860 ) ) ;
#22637=FACE_OUTER_BOUND ( 'NONE', #98082, .T. ) ;
#22644=CYLINDRICAL_SURFACE ( 'NONE', #73522, 0.08000000000000041800 ) ;
#22649=LINE ( 'NONE', #86610, #18934 ) ;
#22653=CARTESIAN_POINT ( 'NONE',  ( 3.580761967785000888, 7.191656372475549119, -0.7216878364870338292 ) ) ;
#22664=CARTESIAN_POINT ( 'NONE',  ( -4.990809943606281607, 6.915973915664348937, -1.443375672974066548 ) ) ;
#22692=CARTESIAN_POINT ( 'NONE',  ( 7.349928672384119288, 8.707909884937221179, 1.082531754730549967 ) ) ;
#22706=CARTESIAN_POINT ( 'NONE',  ( -5.722950238744243023, 7.770137593325314285, 1.443375672974058777 ) ) ;
#22709=CARTESIAN_POINT ( 'NONE',  ( 5.203297092594585393, 9.292540051327542017, 0.7998128361456341429 ) ) ;
#22715=CARTESIAN_POINT ( 'NONE',  ( -6.303615075710993665, 6.318915441276411471, -0.7998128361456362523 ) ) ;
#22724=FACE_BOUND ( 'NONE', #165825, .T. ) ;
#22729=CARTESIAN_POINT ( 'NONE',  ( -6.441468915117185112, 6.687670953824438769, 0.7183096694902652013 ) ) ;
#22751=CARTESIAN_POINT ( 'NONE',  ( 3.757017964762656703, 7.397288368949487491, -1.734723475976807094E-15 ) ) ;
#22755=CARTESIAN_POINT ( 'NONE',  ( -7.391130018105325661, 8.652015104991543026, -1.199719254218452047 ) ) ;
#22760=CARTESIAN_POINT ( 'NONE',  ( -4.599959256786493533, 8.588645909551377855, 0.000000000000000000 ) ) ;
#22765=CARTESIAN_POINT ( 'NONE',  ( -7.119440060507479018, 8.439006504414422238, 1.082531754730549078 ) ) ;
#22772=CARTESIAN_POINT ( 'NONE',  ( -3.142457743317409680, 6.888227477170756785, 0.7998128361456352531 ) ) ;
#22776=ORIENTED_EDGE ( 'NONE', *, *, #31576, .T. ) ;
#22778=B_SPLINE_CURVE_WITH_KNOTS ( 'NONE', 3,
 ( #154546, #171855, #23450, #89562, #57043, #106918 ),
 .UNSPECIFIED., .F., .F.,
 ( 4, 2, 4 ),
 ( 0.001263516168593488680, 0.001315211845502643750, 0.001366907522411799037 ),
 .UNSPECIFIED. ) ;
#22779=CARTESIAN_POINT ( 'NONE',  ( -5.824109505522200081, 8.952488968821326054, -1.199719254218452047 ) ) ;
#22781=CARTESIAN_POINT ( 'NONE',  ( 5.910429572389825026, 7.145202977605201511, -1.123150837922413547 ) ) ;
#22786=CARTESIAN_POINT ( 'NONE',  ( 4.167152111353856547, 5.955039778036558040, 1.599625672291262513 ) ) ;
#22791=AXIS2_PLACEMENT_3D ( 'NONE', #192194, #65384, #47056 ) ;
#22798=CARTESIAN_POINT ( 'NONE',  ( -5.399890319992785237, 9.521898816625391504, 0.7998128361456291469 ) ) ;
#22799=B_SPLINE_CURVE_WITH_KNOTS ( 'NONE', 3,
 ( #178918, #96613, #99784, #196225 ),
 .UNSPECIFIED., .F., .F.,
 ( 4, 4 ),
 ( 0.0004855182311547751126, 0.001091960318275098660 ),
 .UNSPECIFIED. ) ;
#22802=CARTESIAN_POINT ( 'NONE',  ( -3.719872605471121751, 6.605953636083950364, -2.499999999999998668 ) ) ;
#22811=CARTESIAN_POINT ( 'NONE',  ( 4.598150373690133463, 5.393538853173795111, -1.199719254218452047 ) ) ;
#22825=CARTESIAN_POINT ( 'NONE',  ( -0.1904212755198937679, 3.362625042665647879, -2.069931805936022329 ) ) ;
#22826=CARTESIAN_POINT ( 'NONE',  ( 6.257994703896152089, 7.000112715747270009, 0.9732540237740094913 ) ) ;
#22833=CARTESIAN_POINT ( 'NONE',  ( -5.602498012743508227, 5.726462300312828546, -0.1687859242097844992 ) ) ;
#22839=VERTEX_POINT ( 'NONE', #118781 ) ;
#22849=CARTESIAN_POINT ( 'NONE',  ( -4.505562513083238407, 8.245961809465203629, -0.2033783863445335349 ) ) ;
#22854=CARTESIAN_POINT ( 'NONE',  ( -6.480235040494578769, 6.771487114559836762, -0.2501488059577141598 ) ) ;
#22872=CARTESIAN_POINT ( 'NONE',  ( -6.656127069666307072, 6.730179434224282886, 0.7998128361456341429 ) ) ;
#22880=CARTESIAN_POINT ( 'NONE',  ( 5.733910645827320351, 5.654260273078802079, -0.3844519940494390831 ) ) ;
#22892=DIRECTION ( 'NONE',  ( 0.7592566023653004592, 0.6507913734559639396, -0.000000000000000000 ) ) ;
#22900=CARTESIAN_POINT ( 'NONE',  ( 5.968508390656825036, 7.206245191706623032, 1.226434852180135149 ) ) ;
#22908=CARTESIAN_POINT ( 'NONE',  ( 6.879836604291781121, 6.991173891287354003, -0.7998128361456341429 ) ) ;
#22916=CIRCLE ( 'NONE', #9029, 0.4000000000000001332 ) ;
#22919=CARTESIAN_POINT ( 'NONE',  ( -4.329849954717889915, 6.144853928627882489, 1.599625672291270506 ) ) ;
#22921=CARTESIAN_POINT ( 'NONE',  ( 7.991605200612358573, 8.288237253661408843, 0.7998128361456281477 ) ) ;
#22924=CARTESIAN_POINT ( 'NONE',  ( -6.231907884136888676, 7.299589282028351001, -1.199719254218453823 ) ) ;
#22926=VERTEX_POINT ( 'NONE', #66730 ) ;
#22927=CARTESIAN_POINT ( 'NONE',  ( 7.374709211190586089, 7.568525266002632534, 0.000000000000000000 ) ) ;
#22932=CARTESIAN_POINT ( 'NONE',  ( -4.936046011350697427, 8.098431898006973384, 1.075429046246343612 ) ) ;
#22942=CARTESIAN_POINT ( 'NONE',  ( -5.628043163004235794, 5.738674243025936761, 0.7216878364870257245 ) ) ;
#22943=VECTOR ( 'NONE', #98808, 1000.000000000000227 ) ;
#22953=CARTESIAN_POINT ( 'NONE',  ( 4.421367491832282504, 5.291255174293369556, 1.082531754730549078 ) ) ;
#22957=CARTESIAN_POINT ( 'NONE',  ( -5.250750630242457362, 9.347902511916677426, 0.000000000000000000 ) ) ;
#22996=CARTESIAN_POINT ( 'NONE',  ( -3.526529353330350336, 7.128384988945109413, -0.7216878364870458196 ) ) ;
#23009=CARTESIAN_POINT ( 'NONE',  ( -4.916039773278787273, 4.881957280557857715, 0.5603013081572870702 ) ) ;
#23020=EDGE_LOOP ( 'NONE', ( #22776, #65052, #109177, #14397 ) ) ;
#23021=CARTESIAN_POINT ( 'NONE',  ( -3.648552735408990166, 6.310376387068841630, -1.082531754730546636 ) ) ;
#23022=EDGE_CURVE ( 'NONE', #22085, #61771, #113523, .T. ) ;
#23029=CARTESIAN_POINT ( 'NONE',  ( -3.935609729716867289, 7.813571461303467913, 0.7998128361456352531 ) ) ;
#23032=CARTESIAN_POINT ( 'NONE',  ( 4.407809338218622308, 8.156544971314787063, 0.000000000000000000 ) ) ;
#23037=CARTESIAN_POINT ( 'NONE',  ( -3.169574050544739841, 6.919863168935977527, -0.7998128361456481317 ) ) ;
#23039=CARTESIAN_POINT ( 'NONE',  ( 6.304162555737000240, 6.968127521147626346, -0.9177210060461529206 ) ) ;
#23043=CARTESIAN_POINT ( 'NONE',  ( 5.564695703766185275, 5.456842840674144490, 0.000000000000000000 ) ) ;
#23048=CARTESIAN_POINT ( 'NONE',  ( -6.947627372360122955, 7.070263120700404968, 0.000000000000000000 ) ) ;
#23051=CARTESIAN_POINT ( 'NONE',  ( -3.363304624641834106, 6.081549941127532222, -1.199719254218452047 ) ) ;
#23054=B_SPLINE_CURVE_WITH_KNOTS ( 'NONE', 3,
 ( #59456, #125614, #94123, #60517, #43236, #175364, #10692, #76763, #208886, #126678 ),
 .UNSPECIFIED., .F., .F.,
 ( 4, 3, 3, 4 ),
 ( 8.033417195976369988E-16, 3.125154781590810406E-05, 6.537904841941566522E-05, 9.952318552807673643E-05 ),
 .UNSPECIFIED. ) ;
#23057=CARTESIAN_POINT ( 'NONE',  ( 4.868786560638896255, 5.813244087901094481, 1.082531754730549078 ) ) ;
#23058=CARTESIAN_POINT ( 'NONE',  ( -5.763624699140894592, 5.896852701852039580, -0.7216878364870338292 ) ) ;
#23066=CARTESIAN_POINT ( 'NONE',  ( 3.878514461961128479, 6.682628084666728085, -1.199719254218448494 ) ) ;
#23070=FACE_OUTER_BOUND ( 'NONE', #202158, .T. ) ;
#23078=CARTESIAN_POINT ( 'NONE',  ( 4.842126824027952026, 8.201492973507317430, 0.9351865777775794086 ) ) ;
#23084=ORIENTED_EDGE ( 'NONE', *, *, #82890, .T. ) ;
#23087=CARTESIAN_POINT ( 'NONE',  ( 6.387826650694035990, 7.481494509678370264, -1.199719254218452047 ) ) ;
#23098=CARTESIAN_POINT ( 'NONE',  ( 5.638349000628050334, 7.351887578364292075, 1.232751772250343381 ) ) ;
#23114=CARTESIAN_POINT ( 'NONE',  ( -5.745623237141265882, 9.925253886631958622, 0.7998128361456291469 ) ) ;
#23127=CARTESIAN_POINT ( 'NONE',  ( 4.376249722160992839, 8.327651452488305850, 0.000000000000000000 ) ) ;
#23133=CARTESIAN_POINT ( 'NONE',  ( -8.041394506236766659, 8.554250810130591631, -0.7216878364870338292 ) ) ;
#23135=CARTESIAN_POINT ( 'NONE',  ( 4.309512724297349884, 6.121127159803966933, 1.599625672291261402 ) ) ;
#23139=CARTESIAN_POINT ( 'NONE',  ( 4.217995187182920880, 6.974725914138481642, 1.082531754730549078 ) ) ;
#23156=CARTESIAN_POINT ( 'NONE',  ( -6.238160076063538284, 9.331584951165851294, 1.082531754730549967 ) ) ;
#23158=CARTESIAN_POINT ( 'NONE',  ( 6.536439455564164724, 7.758839131980592718, 1.082531754730549967 ) ) ;
#23167=CARTESIAN_POINT ( 'NONE',  ( -3.949167883330528372, 7.829389307186077396, 1.214306433183764966E-14 ) ) ;
#23168=CARTESIAN_POINT ( 'NONE',  ( -3.959863383643135393, 6.777535159962392086, 1.199719254218452935 ) ) ;
#23171=CARTESIAN_POINT ( 'NONE',  ( 5.302647476276220573, 8.240153584747313076, -1.082531754730548412 ) ) ;
#23178=DIRECTION ( 'NONE',  ( 0.000000000000000000, 0.000000000000000000, -1.000000000000000000 ) ) ;
#23181=CARTESIAN_POINT ( 'NONE',  ( -4.646665375593996394, 8.329970469126573462, 0.4085986083085801912 ) ) ;
#23185=CARTESIAN_POINT ( 'NONE',  ( 3.580761967785000888, 7.191656372475549119, -0.7216878364870338292 ) ) ;
#23189=CARTESIAN_POINT ( 'NONE',  ( -5.257529707049291900, 9.355811434857983500, 0.7998128361456291469 ) ) ;
#23197=ADVANCED_FACE ( 'NONE', ( #164038 ), #208646, .T. ) ;
#23204=CARTESIAN_POINT ( 'NONE',  ( 6.391743074199808916, 6.421731439513382433, -0.7998128361456481317 ) ) ;
#23242=CARTESIAN_POINT ( 'NONE',  ( 6.455090533882185788, 8.624301270986276080, -1.443375672974078761 ) ) ;
#23248=CARTESIAN_POINT ( 'NONE',  ( 5.668717623845194176, 9.627604637879139560, 0.000000000000000000 ) ) ;
#23273=CARTESIAN_POINT ( 'NONE',  ( -5.191846479390389568, 5.021852078902356631, 0.7998128361456281477 ) ) ;
#23275=CARTESIAN_POINT ( 'NONE',  ( 5.411112705185558092, 6.445957923205511086, -1.082531754730548412 ) ) ;
#23281=CARTESIAN_POINT ( 'NONE',  ( -4.167152111353897403, 5.955039778036558040, 1.599625672291270506 ) ) ;
#23286=CARTESIAN_POINT ( 'NONE',  ( -6.780486220610186798, 8.043560357867583832, -1.082531754730549967 ) ) ;
#23291=CARTESIAN_POINT ( 'NONE',  ( -7.208094944320834863, 8.438474185576302133, -1.199719254218452047 ) ) ;
#23296=CARTESIAN_POINT ( 'NONE',  ( -5.472651281771599763, 6.413789912602166687, 1.199719254218452935 ) ) ;
#23310=CARTESIAN_POINT ( 'NONE',  ( -4.611181642423629157, 7.433443445252599702, 1.082531754730549967 ) ) ;
#23313=CARTESIAN_POINT ( 'NONE',  ( -4.706088717274938382, 6.583799151611112954, 1.443375672974058777 ) ) ;
#23315=CARTESIAN_POINT ( 'NONE',  ( 4.278479993564246797, 7.149254538203735798, 1.199719254218452047 ) ) ;
#23316=CARTESIAN_POINT ( 'NONE',  ( -4.633854640820660009, 8.628190524257904670, -0.7998128361456362523 ) ) ;
#23317=CARTESIAN_POINT ( 'NONE',  ( -6.095272577795516789, 9.268845886473535245, 1.199719254218452047 ) ) ;
#23335=CARTESIAN_POINT ( 'NONE',  ( 7.472478939787284169, 8.746922180287201698, 1.199719254218452935 ) ) ;
#23348=ADVANCED_FACE ( 'NONE', ( #137930 ), #148549, .T. ) ;
#23360=DIRECTION ( 'NONE',  ( 2.168404344971003188E-14, -1.000000000000000000, 0.000000000000000000 ) ) ;
#23365=CARTESIAN_POINT ( 'NONE',  ( -1.845237968648473448, 8.937006183319889274, -0.7749999999999996891 ) ) ;
#23367=CARTESIAN_POINT ( 'NONE',  ( 2.982962183914244836, 6.465010346290775978, -0.5414090736701422379 ) ) ;
#23375=CARTESIAN_POINT ( 'NONE',  ( 4.538947565524982686, 8.517465603079630299, 0.000000000000000000 ) ) ;
#23391=CARTESIAN_POINT ( 'NONE',  ( 4.797606254389322089, 6.690569611577942943, 1.599625672291268286 ) ) ;
#23394=VERTEX_POINT ( 'NONE', #24146 ) ;
#23396=CARTESIAN_POINT ( 'NONE',  ( -6.749980374757255319, 8.968339418673846097, 1.599625672291269396 ) ) ;
#23400=VERTEX_POINT ( 'NONE', #90249 ) ;
#23401=CARTESIAN_POINT ( 'NONE',  ( 5.747730777550676073, 5.670383760089384495, 0.000000000000000000 ) ) ;
#23402=ORIENTED_EDGE ( 'NONE', *, *, #51328, .T. ) ;
#23406=FACE_OUTER_BOUND ( 'NONE', #41125, .T. ) ;
#23413=CARTESIAN_POINT ( 'NONE',  ( 7.865138509703455405, 8.348618814175074121, -0.7216878364870317197 ) ) ;
#23414=CARTESIAN_POINT ( 'NONE',  ( -4.855228407469635243, 4.837057028235559386, 0.7216878364870257245 ) ) ;
#23416=CARTESIAN_POINT ( 'NONE',  ( -6.017840079619296567, 8.114175741012878973, -1.599625672291271394 ) ) ;
#23423=ORIENTED_EDGE ( 'NONE', *, *, #61552, .T. ) ;
#23428=CARTESIAN_POINT ( 'NONE',  ( 5.285699784481295183, 7.260012063351913625, 1.599625672291268286 ) ) ;
#23429=CARTESIAN_POINT ( 'NONE',  ( 6.412080304620304538, 6.445458208337293549, -0.7998128361456481317 ) ) ;
#23432=CARTESIAN_POINT ( 'NONE',  ( 7.388267364804250725, 7.584343111885245570, -0.7998128361456341429 ) ) ;
#23440=FACE_OUTER_BOUND ( 'NONE', #124220, .T. ) ;
#23441=EDGE_CURVE ( 'NONE', #52099, #105328, #110574, .T. ) ;
#23448=CARTESIAN_POINT ( 'NONE',  ( 5.396826230253299883, 7.665096674459883630, -1.326205021280580265 ) ) ;
#23450=CARTESIAN_POINT ( 'NONE',  ( 0.3988961525413015075, 2.965604040240178652, 2.024173287229360074 ) ) ;
#23451=CARTESIAN_POINT ( 'NONE',  ( 4.411198876399872404, 6.239761003923544713, -1.599625672291273171 ) ) ;
#23456=CARTESIAN_POINT ( 'NONE',  ( 4.492547798081839794, 6.334668079219206049, 1.599625672291262513 ) ) ;
#23461=CARTESIAN_POINT ( 'NONE',  ( 6.210516883511641772, 9.403297576475722508, 1.199719254218452047 ) ) ;
#23469=CARTESIAN_POINT ( 'NONE',  ( 5.885648082108199119, 6.999582529615296700, 1.082531754730549967 ) ) ;
#23471=CARTESIAN_POINT ( 'NONE',  ( -5.875479466675803231, 7.948088359245467416, -1.599625672291271394 ) ) ;
#23473=CARTESIAN_POINT ( 'NONE',  ( 5.388439706788500594, 5.251210844200210559, 0.7998128361456352531 ) ) ;
#23485=CARTESIAN_POINT ( 'NONE',  ( -7.932929277771797238, 8.427708043588125975, 0.000000000000000000 ) ) ;
#23495=CARTESIAN_POINT ( 'NONE',  ( 0.1975679859324476761, 2.638084932213505152, -1.992869612520775213 ) ) ;
#23515=CARTESIAN_POINT ( 'NONE',  ( 4.312902262922978736, 5.164712407232485702, -1.082531754730548412 ) ) ;
#23520=CARTESIAN_POINT ( 'NONE',  ( 6.481679955784983349, 9.719654494127929922, -1.199719254218452047 ) ) ;
#23522=CARTESIAN_POINT ( 'NONE',  ( 7.014364370223726830, 9.276787413384745662, -1.599625672291269396 ) ) ;
#23532=CARTESIAN_POINT ( 'NONE',  ( -4.599959256786493533, 8.588645909551377855, 0.000000000000000000 ) ) ;
#23534=CARTESIAN_POINT ( 'NONE',  ( 7.160114521348466710, 7.526090827760914870, 0.000000000000000000 ) ) ;
#23543=CARTESIAN_POINT ( 'NONE',  ( -5.418418667316934112, 6.350518529071726981, -1.199719254218453823 ) ) ;
#23548=CARTESIAN_POINT ( 'NONE',  ( -4.014622883422336308, 5.777089012116397804, -1.443375672974066548 ) ) ;
#23553=CARTESIAN_POINT ( 'NONE',  ( -2.972980823146582186, 6.690504403638126263, 0.000000000000000000 ) ) ;
#23579=CARTESIAN_POINT ( 'NONE',  ( -6.629010762438975135, 6.698543742459062145, -0.7998128361456362523 ) ) ;
#23581=CARTESIAN_POINT ( 'NONE',  ( -5.164730172163054966, 4.990216387137135889, -0.7998128361456362523 ) ) ;
#23591=CARTESIAN_POINT ( 'NONE',  ( -5.346851039111045978, 6.199209027673978412, -1.060622344683157747 ) ) ;
#23600=EDGE_CURVE ( 'NONE', #183890, #116379, #24566, .T. ) ;
#23605=AXIS2_PLACEMENT_3D ( 'NONE', #197930, #132979, #116752 ) ;
#23606=CARTESIAN_POINT ( 'NONE',  ( -4.606738333593328072, 8.596554832492683929, 0.7998128361456281477 ) ) ;
#23614=CARTESIAN_POINT ( 'NONE',  ( 6.658462837642789012, 9.821938173008357253, 1.082531754730549078 ) ) ;
#23627=CARTESIAN_POINT ( 'NONE',  ( 3.739016502318667445, 7.584212696005614873, 0.7998128361456271485 ) ) ;
#23635=CARTESIAN_POINT ( 'NONE',  ( 7.361151057576892143, 7.552707420120024828, 0.7998128361456291469 ) ) ;
#23637=CARTESIAN_POINT ( 'NONE',  ( 6.638652492546827766, 7.774124658506663010, 1.199719254218452047 ) ) ;
#23651=CARTESIAN_POINT ( 'NONE',  ( 6.272547281004660746, 6.891683285556123195, -0.7655605874731727933 ) ) ;
#23653=CARTESIAN_POINT ( 'NONE',  ( 4.733205024946604667, 8.536173272497439513, 0.000000000000000000 ) ) ;
#23670=CARTESIAN_POINT ( 'NONE',  ( -4.733205024502264102, 7.575804057677677505, 1.082531754730549967 ) ) ;
#23675=CARTESIAN_POINT ( 'NONE',  ( 5.075973375179646752, 4.911903417823547002, -0.2129554534070592919 ) ) ;
#23691=DIRECTION ( 'NONE',  ( 0.000000000000000000, 0.000000000000000000, 1.000000000000000000 ) ) ;
#23693=CARTESIAN_POINT ( 'NONE',  ( 5.692444392891300886, 7.734547439830227411, -1.599625672291281386 ) ) ;
#23734=CARTESIAN_POINT ( 'NONE',  ( 5.261973015879598314, 5.311592404713873172, -0.7216878364870458196 ) ) ;
#23744=CARTESIAN_POINT ( 'NONE',  ( -5.167065940583949413, 5.200867483535597913, 0.000000000000000000 ) ) ;
#23750=CARTESIAN_POINT ( 'NONE',  ( 7.065207446497155708, 9.336104335703744539, 0.000000000000000000 ) ) ;
#23766=EDGE_CURVE ( 'NONE', #100853, #149695, #34269, .T. ) ;
#23775=CARTESIAN_POINT ( 'NONE',  ( 5.564695703766185275, 5.456842840674144490, 0.000000000000000000 ) ) ;
#23787=CARTESIAN_POINT ( 'NONE',  ( -6.129694847154220305, 8.244672969803623630, -1.443375672974066548 ) ) ;
#23789=CARTESIAN_POINT ( 'NONE',  ( 7.014364370223726830, 9.276787413384745662, -1.599625672291269396 ) ) ;
#23793=VECTOR ( 'NONE', #128143, 1000.000000000000000 ) ;
#23805=CARTESIAN_POINT ( 'NONE',  ( 4.913904330310220558, 4.697586238308844919, 0.000000000000000000 ) ) ;
#23807=CARTESIAN_POINT ( 'NONE',  ( -3.526529353330355221, 6.168015774643768268, -1.082531754730546636 ) ) ;
#23810=LINE ( 'NONE', #89915, #83681 ) ;
#23836=CARTESIAN_POINT ( 'NONE',  ( -7.781453819600577582, 8.043060642480948985, 0.000000000000000000 ) ) ;
#23839=CARTESIAN_POINT ( 'NONE',  ( -6.286140498591554326, 7.362860665558790707, 1.199719254218452047 ) ) ;
#23840=CARTESIAN_POINT ( 'NONE',  ( -5.605310199005481664, 5.702455421404705405, 0.3560189469562446973 ) ) ;
#23844=CARTESIAN_POINT ( 'NONE',  ( -6.170369307550858551, 8.292126506933035657, 1.443375672974058777 ) ) ;
#23845=MANIFOLD_SOLID_BREP ( 'Fillet2', #4953 ) ;
#23851=CARTESIAN_POINT ( 'NONE',  ( -4.329849954717889915, 6.144853928627882489, 1.599625672291270506 ) ) ;
#23858=CARTESIAN_POINT ( 'NONE',  ( -5.610041701004606196, 9.767075427805856691, -0.7998128361456362523 ) ) ;
#23860=CARTESIAN_POINT ( 'NONE',  ( 4.771426152247889796, 8.279957873513081879, -0.8122977234717634332 ) ) ;
#23863=CARTESIAN_POINT ( 'NONE',  ( 6.387350227241329392, 6.552219065289217603, 2.499999999999828582 ) ) ;
#23865=CARTESIAN_POINT ( 'NONE',  ( 8.167861197590044142, 8.493869250135347215, 0.000000000000000000 ) ) ;
#23872=AXIS2_PLACEMENT_3D ( 'NONE', #76220, #192085, #174821 ) ;
#23875=CARTESIAN_POINT ( 'NONE',  ( -6.064239847062411926, 10.29697326487330500, 0.000000000000000000 ) ) ;
#23888=CARTESIAN_POINT ( 'NONE',  ( 7.180978637093494044, 8.406838493811077839, -1.199719254218452047 ) ) ;
#23902=CARTESIAN_POINT ( 'NONE',  ( 6.308853223578811509, 6.964933332891984463, 0.9108697706533327443 ) ) ;
#23904=CARTESIAN_POINT ( 'NONE',  ( -3.757017964318317471, 6.436919154129725484, 1.082531754730549967 ) ) ;
#23911=CARTESIAN_POINT ( 'NONE',  ( -6.116136693540540570, 10.14959355252369910, 0.000000000000000000 ) ) ;
#23927=ORIENTED_EDGE ( 'NONE', *, *, #7268, .T. ) ;
#23931=CARTESIAN_POINT ( 'NONE',  ( 5.551137550152489553, 5.441024994791534120, 0.7998128361456352531 ) ) ;
#23949=AXIS2_PLACEMENT_3D ( 'NONE', #147510, #131310, #1211 ) ;
#23951=CARTESIAN_POINT ( 'NONE',  ( -6.794571259104023930, 7.956029886156682274, 1.199719254218452047 ) ) ;
#23954=CYLINDRICAL_SURFACE ( 'NONE', #5343, 0.08000000000000020983 ) ;
#23968=CARTESIAN_POINT ( 'NONE',  ( 5.923986774528332333, 5.876015756563318426, -0.7998128361456481317 ) ) ;
#23970=CARTESIAN_POINT ( 'NONE',  ( 6.739811759324814133, 8.956476034002680109, -1.443375672974078761 ) ) ;
#23977=CARTESIAN_POINT ( 'NONE',  ( 4.739226852959141034, 8.198292129125304584, 0.7147376406119988479 ) ) ;
#23979=CARTESIAN_POINT ( 'NONE',  ( 6.059270238282111087, 7.038290852966752276, 1.014332888565868229 ) ) ;
#23996=CARTESIAN_POINT ( 'NONE',  ( -5.679940009482361774, 5.591294530676332641, 0.7998128361456281477 ) ) ;
#23998=CARTESIAN_POINT ( 'NONE',  ( 5.574337433874081427, 6.532423756721743580, -1.199719254218452047 ) ) ;
#24002=CARTESIAN_POINT ( 'NONE',  ( -5.315678745009726924, 8.359319748223434487, -1.199719254218453823 ) ) ;
#24006=CARTESIAN_POINT ( 'NONE',  ( 5.013482942003290255, 9.071090208970993274, -0.7998128361456481317 ) ) ;
#24012=CARTESIAN_POINT ( 'NONE',  ( -4.905272163827030241, 8.130510659208837865, -1.040677472382423474 ) ) ;
#24013=DIRECTION ( 'NONE',  ( -1.000000000000000000, 0.000000000000000000, 0.000000000000000000 ) ) ;
#24020=CARTESIAN_POINT ( 'NONE',  ( -6.089020385868876062, 6.276481003034692030, -0.7216878364870338292 ) ) ;
#24029=CARTESIAN_POINT ( 'NONE',  ( 4.692530564105613422, 7.528350520548263702, -1.082531754730548412 ) ) ;
#24033=CARTESIAN_POINT ( 'NONE',  ( -6.291865805193673111, 9.498204651771386509, -1.199719254218452047 ) ) ;
#24035=ORIENTED_EDGE ( 'NONE', *, *, #19121, .F. ) ;
#24047=CARTESIAN_POINT ( 'NONE',  ( 3.061108821635398769, 6.793320401875094561, -0.7998128361456362523 ) ) ;
#24076=CARTESIAN_POINT ( 'NONE',  ( -4.502716413514296079, 8.267269892493059658, -0.7216878364870338292 ) ) ;
#24100=CARTESIAN_POINT ( 'NONE',  ( -4.963693635934603776, 4.963599794778024155, 0.000000000000000000 ) ) ;
#24105=CARTESIAN_POINT ( 'NONE',  ( -3.623772196602547346, 7.449761006003425834, 0.000000000000000000 ) ) ;
#24113=CARTESIAN_POINT ( 'NONE',  ( -8.100070429521727178, 8.414780020722290033, 0.7998128361456341429 ) ) ;
#24115=CARTESIAN_POINT ( 'NONE',  ( 5.845834525830363226, 7.300097092180095615, -1.274846751706928849 ) ) ;
#24119=CARTESIAN_POINT ( 'NONE',  ( 4.553559489343365740, 6.405848385690952718, -1.599625672291269396 ) ) ;
#24125=CARTESIAN_POINT ( 'NONE',  ( -7.422162748838431412, 7.623887726591770608, -0.7998128361456362523 ) ) ;
#24128=CARTESIAN_POINT ( 'NONE',  ( -4.065465959251405081, 5.836405933916976707, -1.599625672291271394 ) ) ;
#24133=CARTESIAN_POINT ( 'NONE',  ( 6.495764994278809823, 6.751016379513001375, 0.7216878364870328300 ) ) ;
#24134=CARTESIAN_POINT ( 'NONE',  ( -5.356880090730904875, 7.343055753976412525, 1.443375672974058777 ) ) ;
#24140=CARTESIAN_POINT ( 'NONE',  ( 5.401997860402196316, 5.267028690082820930, 0.000000000000000000 ) ) ;
#24144=CARTESIAN_POINT ( 'NONE',  ( -4.489403031431899116, 8.251676092768461146, -0.01033961207361998313 ) ) ;
#24146=CARTESIAN_POINT ( 'NONE',  ( -5.608757509019071108, 5.629766575892905855, -0.3787719694710602325 ) ) ;
#24150=CARTESIAN_POINT ( 'NONE',  ( 5.602183562003149042, 7.492195738860313092, 1.335281325244306982 ) ) ;
#24159=CARTESIAN_POINT ( 'NONE',  ( 5.956828388357757298, 8.042995434541133193, 1.599625672291269396 ) ) ;
#24169=CARTESIAN_POINT ( 'NONE',  ( 6.438112759045284683, 6.782534085545247393, 0.3978009605737874432 ) ) ;
#24182=CARTESIAN_POINT ( 'NONE',  ( 4.892484645941061139, 4.880522639849741218, -0.04086785794226917984 ) ) ;
#24185=CARTESIAN_POINT ( 'NONE',  ( -7.767895665986912057, 8.027242796598338614, -0.7998128361456362523 ) ) ;
#24198=CARTESIAN_POINT ( 'NONE',  ( 5.664274315459256748, 9.830346811336296398, -0.7998128361456481317 ) ) ;
#24205=CARTESIAN_POINT ( 'NONE',  ( -5.912764388891193157, 9.912325863766124456, 0.000000000000000000 ) ) ;
#24206=EDGE_LOOP ( 'NONE', ( #94248, #57078, #20752 ) ) ;
#24207=CARTESIAN_POINT ( 'NONE',  ( 2.878073747850912412, 6.579779482459851003, -0.7998128361456362523 ) ) ;
#24210=CARTESIAN_POINT ( 'NONE',  ( 3.404505970362959655, 6.986024375483197879, 0.7216878364870257245 ) ) ;
#24217=DIRECTION ( 'NONE',  ( -1.000000000000000000, 0.000000000000000000, 0.000000000000000000 ) ) ;
#24218=CARTESIAN_POINT ( 'NONE',  ( -6.489499031467138579, 6.765560312407735033, -0.1891594744549245088 ) ) ;
#24222=ORIENTED_EDGE ( 'NONE', *, *, #24434, .T. ) ;
#24225=CARTESIAN_POINT ( 'NONE',  ( -4.496464221587651799, 5.274905009054215554, 1.199719254218452935 ) ) ;
#24226=CARTESIAN_POINT ( 'NONE',  ( 5.063044020060520900, 4.871582543017558109, 0.7998128361456352531 ) ) ;
#24236=ORIENTED_EDGE ( 'NONE', *, *, #61327, .F. ) ;
#24237=CARTESIAN_POINT ( 'NONE',  ( -5.367048706163331850, 7.354919138647580290, -1.599625672291271394 ) ) ;
#24238=CARTESIAN_POINT ( 'NONE',  ( -6.147696309153835692, 6.137010213626392208, 0.7998128361456281477 ) ) ;
#24240=CARTESIAN_POINT ( 'NONE',  ( 4.706088717274885092, 8.504537580213796133, 0.7216878364870317197 ) ) ;
#24252=CARTESIAN_POINT ( 'NONE',  ( -4.683575932806860465, 8.284415941318199472, -0.5487617172068790516 ) ) ;
#24256=CARTESIAN_POINT ( 'NONE',  ( 5.397554552016228691, 5.469770863539975991, 0.7216878364870328300 ) ) ;
#24261=CARTESIAN_POINT ( 'NONE',  ( -7.119966945832006289, 8.335658187339330283, 1.199719254218452047 ) ) ;
#24274=CARTESIAN_POINT ( 'NONE',  ( 4.355912491740495440, 8.303924683664389406, 0.000000000000000000 ) ) ;
#24311=CARTESIAN_POINT ( 'NONE',  ( 7.200788982633824276, 7.573544365927161515, 0.000000000000000000 ) ) ;
#24316=CARTESIAN_POINT ( 'NONE',  ( 6.007671464186812749, 10.02305078494439883, 0.7216878364870317197 ) ) ;
#24340=CARTESIAN_POINT ( 'NONE',  ( -5.327428015527048366, 5.180030537728460338, -0.7998128361456362523 ) ) ;
#24342=CARTESIAN_POINT ( 'NONE',  ( 4.041739190205284160, 7.729463131965888856, 0.000000000000000000 ) ) ;
#24348=CARTESIAN_POINT ( 'NONE',  ( -3.383641855062333281, 6.105276709951447778, -1.199719254218452047 ) ) ;
#24353=CARTESIAN_POINT ( 'NONE',  ( -6.997416678428844072, 8.296645891989347987, 1.082531754730549078 ) ) ;
#24360=CARTESIAN_POINT ( 'NONE',  ( -3.959863383643135393, 6.777535159962392086, 1.199719254218452935 ) ) ;
#24372=CARTESIAN_POINT ( 'NONE',  ( -6.143253000767895600, 6.339752387083549934, 0.000000000000000000 ) ) ;
#24374=CARTESIAN_POINT ( 'NONE',  ( -5.194182247366913252, 7.153241603385088965, 1.443375672974058777 ) ) ;
#24375=CARTESIAN_POINT ( 'NONE',  ( 5.875479466675786355, 7.948088359245467416, -1.599625672291283607 ) ) ;
#24377=CARTESIAN_POINT ( 'NONE',  ( -4.769436176957319695, 8.786368983084006601, 0.7998128361456281477 ) ) ;
#24397=CARTESIAN_POINT ( 'NONE',  ( 6.875920180786008196, 8.050936961452347163, -1.199719254218452047 ) ) ;
#24434=EDGE_CURVE ( 'NONE', #80483, #85779, #53990, .T. ) ;
#24437=CARTESIAN_POINT ( 'NONE',  ( 4.199993725183334803, 8.122019456014369254, -0.7998128361456362523 ) ) ;
#24438=LINE ( 'NONE', #54834, #54907 ) ;
#24440=CARTESIAN_POINT ( 'NONE',  ( -5.340986169140711226, 5.195848383611072485, 0.000000000000000000 ) ) ;
#24455=CARTESIAN_POINT ( 'NONE',  ( 2.911969131885072670, 6.619324097166378706, 0.000000000000000000 ) ) ;
#24456=CARTESIAN_POINT ( 'NONE',  ( 4.420840606507738357, 7.315341919971147355, 1.199719254218451159 ) ) ;
#24464=CARTESIAN_POINT ( 'NONE',  ( -5.264308783856126439, 9.363720357799287797, -0.7998128361456362523 ) ) ;
#24469=CARTESIAN_POINT ( 'NONE',  ( 4.929271367020211514, 7.908511140569038922, 1.199719254218452047 ) ) ;
#24474=CARTESIAN_POINT ( 'NONE',  ( -3.179715765502671321, 5.975770656120749535, 2.419999999999999485 ) ) ;
#24480=CARTESIAN_POINT ( 'NONE',  ( 5.885648082108188461, 8.920320958217979879, 1.082531754730549967 ) ) ;
#24481=CARTESIAN_POINT ( 'NONE',  ( -4.502716413514310290, 6.346531463890372926, -1.443375672974066548 ) ) ;
#24482=CARTESIAN_POINT ( 'NONE',  ( -6.424584688029276514, 8.588711117491191871, 1.599625672291269396 ) ) ;
#24488=( BOUNDED_CURVE ( )  B_SPLINE_CURVE ( 2, ( #153060, #134707, #183421, #367, #118492 ),
 .UNSPECIFIED., .F., .T. ) 
 B_SPLINE_CURVE_WITH_KNOTS ( ( 3, 2, 3 ),
 ( 0.02206790957329452310, 0.02500000000000000139, 0.02750504326964346713 ),
 .UNSPECIFIED. ) 
 CURVE ( )  GEOMETRIC_REPRESENTATION_ITEM ( )  RATIONAL_B_SPLINE_CURVE ( ( 0.9388936963964400473, 0.9528609242817545066, 1.000000000000000000, 0.9597265407336408316, 0.9436659034065904006 ) ) 
 REPRESENTATION_ITEM ( '' )  );
#24494=CARTESIAN_POINT ( 'NONE',  ( 6.180537922983273091, 8.303989891604203422, -1.599625672291281386 ) ) ;
#24495=VERTEX_POINT ( 'NONE', #69699 ) ;
#24496=CARTESIAN_POINT ( 'NONE',  ( 6.391743074199808916, 6.421731439513382433, -0.7998128361456481317 ) ) ;
#24497=CARTESIAN_POINT ( 'NONE',  ( 5.688527969385528849, 8.794310509995222347, -1.199719254218452047 ) ) ;
#24500=CARTESIAN_POINT ( 'NONE',  ( 7.364013710877980401, 8.620379413226322285, -1.199719254218452047 ) ) ;
#24521=CARTESIAN_POINT ( 'NONE',  ( 4.760848217054122422, 5.583353003765119560, -1.199719254218452047 ) ) ;
#24523=FACE_OUTER_BOUND ( 'NONE', #34660, .T. ) ;
#24526=CARTESIAN_POINT ( 'NONE',  ( 4.248501033035879004, 6.049946853332221153, -1.599625672291273171 ) ) ;
#24531=B_SPLINE_CURVE_WITH_KNOTS ( 'NONE', 3,
 ( #205671, #59432, #126650, #41077 ),
 .UNSPECIFIED., .F., .F.,
 ( 4, 4 ),
 ( 1.685346633177199101E-15, 0.0005562209383481761353 ),
 .UNSPECIFIED. ) ;
#24532=CARTESIAN_POINT ( 'NONE',  ( 2.898410978271408922, 6.603506251283770112, -0.7998128361456362523 ) ) ;
#24536=CARTESIAN_POINT ( 'NONE',  ( 5.777182853198898904, 6.873039762554409293, -1.082531754730548412 ) ) ;
#24538=CARTESIAN_POINT ( 'NONE',  ( -5.468734858265826837, 7.473552982767158070, 1.599625672291263179 ) ) ;
#24540=CARTESIAN_POINT ( 'NONE',  ( 3.932747076415766596, 6.745899468197171345, 1.199719254218451159 ) ) ;
#24550=CARTESIAN_POINT ( 'NONE',  ( -2.972980823146582186, 6.690504403638126263, 0.000000000000000000 ) ) ;
#24561=CARTESIAN_POINT ( 'NONE',  ( 0.1009995753616280273, 2.612933547399907130, -1.997555607063249861 ) ) ;
#24566=( BOUNDED_CURVE ( )  B_SPLINE_CURVE ( 2, ( #25226, #91329, #157389, #75056, #105446, #37212, #55599, #103286, #153101, #136862, #139006, #21994, #38283, #4676, #70750, #154175, #71820, #187722, #202887, #39350, #120679, #104360, #170405, #205028, #6822, #72901, #56674, #126020, #160569, #46847, #194130, #59868, #42583, #43647, #208236, #128168, #191980, #124957, #96670, #193057, #45779, #95606, #92405, #111896, #178973, #177900, #161655, #212503, #108687, #60937, #174716, #78249, #29513, #12177, #159503, #195210, #80388 ),
 .UNSPECIFIED., .F., .T. ) 
 B_SPLINE_CURVE_WITH_KNOTS ( ( 3, 2, 2, 2, 2, 2, 2, 2, 2, 2, 2, 2, 2, 2, 2, 2, 2, 2, 2, 2, 2, 2, 2, 2, 2, 2, 2, 2, 3 ),
 ( 0.2844739210328581791, 0.2916666666666666852, 0.2999999999999999889, 0.3083333333333333481, 0.3166666666666666519, 0.3250000000000000111, 0.3333333333333333148, 0.3416666666666666741, 0.3499999999999999778, 0.3583333333333333370, 0.3666666666666666408, 0.3750000000000000000, 0.3833333333333333592, 0.3916666666666666630, 0.4000000000000000222, 0.4083333333333333259, 0.4166666666666666852, 0.4249999999999999889, 0.4333333333333333481, 0.4416666666666666519, 0.4500000000000000111, 0.4583333333333333148, 0.4666666666666666741, 0.4749999999999999778, 0.4833333333333333370, 0.4916666666666666408, 0.5000000000000000000, 0.5083333333333333037, 0.5122792266304363462 ),
 .UNSPECIFIED. ) 
 CURVE ( )  GEOMETRIC_REPRESENTATION_ITEM ( )  RATIONAL_B_SPLINE_CURVE ( ( 0.9683452906431593288, 0.8843625769635120593, 1.000000000000000000, 0.8660254037844387076, 1.000000000000000000, 0.8660254037844387076, 1.000000000000000000, 0.8660254037844387076, 1.000000000000000000, 0.8660254037844387076, 1.000000000000000000, 0.8660254037844387076, 1.000000000000000000, 0.8660254037844387076, 1.000000000000000000, 0.8660254037844387076, 1.000000000000000000, 0.8660254037844387076, 1.000000000000000000, 0.8660254037844387076, 1.000000000000000000, 0.8660254037844387076, 1.000000000000000000, 0.8660254037844387076, 1.000000000000000000, 0.8660254037844387076, 1.000000000000000000, 0.8660254037844387076, 1.000000000000000000, 0.8660254037844387076, 1.000000000000000000, 0.8660254037844387076, 1.000000000000000000, 0.8660254037844387076, 1.000000000000000000, 0.8660254037844387076, 1.000000000000000000, 0.8660254037844387076, 1.000000000000000000, 0.8660254037844387076, 1.000000000000000000, 0.8660254037844387076, 1.000000000000000000, 0.8660254037844387076, 1.000000000000000000, 0.8660254037844387076, 1.000000000000000000, 0.8660254037844387076, 1.000000000000000000, 0.8660254037844387076, 1.000000000000000000, 0.8660254037844387076, 1.000000000000000000, 0.8660254037844387076, 1.000000000000000000, 0.9365620646573122876, 0.9332007670388082765 ) ) 
 REPRESENTATION_ITEM ( '' )  );
#24572=ORIENTED_EDGE ( 'NONE', *, *, #163868, .T. ) ;
#24582=CARTESIAN_POINT ( 'NONE',  ( 4.177320726786311056, 5.966903162707725805, -1.443375672974068769 ) ) ;
#24589=CARTESIAN_POINT ( 'NONE',  ( 3.973948422136968084, 5.729635473950147606, -1.443375672974068769 ) ) ;
#24601=CARTESIAN_POINT ( 'NONE',  ( -5.098748287191073203, 8.106234214101666780, 1.199719254218452935 ) ) ;
#24603=CARTESIAN_POINT ( 'NONE',  ( 7.309254211098760834, 8.660456346770972758, 1.082531754730549967 ) ) ;
#24605=EDGE_CURVE ( 'NONE', #188712, #142732, #149508, .T. ) ;
#24613=CARTESIAN_POINT ( 'NONE',  ( -5.808742468812186033, 5.741564066561132940, 0.000000000000000000 ) ) ;
#24618=CARTESIAN_POINT ( 'NONE',  ( -4.841670253855968831, 4.821239182352949904, 0.000000000000000000 ) ) ;
#24623=CARTESIAN_POINT ( 'NONE',  ( -5.171509248969888617, 4.998125310078441075, 0.7998128361456281477 ) ) ;
#24631=CARTESIAN_POINT ( 'NONE',  ( -5.593777659986292505, 7.397990072842402398, -1.241664499109219166 ) ) ;
#24644=CARTESIAN_POINT ( 'NONE',  ( -7.456058132872594335, 7.663432341298296535, 0.000000000000000000 ) ) ;
#24645=DIRECTION ( 'NONE',  ( -0.7592566023652990159, -0.6507913734559659380, 0.000000000000000000 ) ) ;
#24648=ORIENTED_EDGE ( 'NONE', *, *, #30406, .T. ) ;
#24657=CARTESIAN_POINT ( 'NONE',  ( -6.041797769283476782, 7.151762567314746022, -1.181783516275588752 ) ) ;
#24669=DIRECTION ( 'NONE',  ( -0.000000000000000000, 1.000000000000000000, -0.000000000000000000 ) ) ;
#24672=CARTESIAN_POINT ( 'NONE',  ( -5.818384198920079520, 6.817144982608731141, 1.199719254218452935 ) ) ;
#24673=CARTESIAN_POINT ( 'NONE',  ( 7.005397802120290507, 5.950282834973755541, 2.500000000000000444 ) ) ;
#24688=CARTESIAN_POINT ( 'NONE',  ( -4.271379415251800538, 7.751480557515569636, 0.6337447475577907552 ) ) ;
#24693=CARTESIAN_POINT ( 'NONE',  ( 5.032011289327418702, 5.899709921417326974, 1.199719254218452935 ) ) ;
#24701=CARTESIAN_POINT ( 'NONE',  ( 7.388267364804250725, 7.584343111885245570, -0.7998128361456341429 ) ) ;
#24703=CARTESIAN_POINT ( 'NONE',  ( 7.015418140428412386, 7.149352350113456822, 0.7998128361456331437 ) ) ;
#24716=CARTESIAN_POINT ( 'NONE',  ( 5.910429572389825026, 7.145202977605201511, -1.123150837922413547 ) ) ;
#24719=CARTESIAN_POINT ( 'NONE',  ( 5.234856708652227297, 7.200695141551334721, 1.443375672974065660 ) ) ;
#24738=CARTESIAN_POINT ( 'NONE',  ( -5.926322542504877333, 7.047036066744706950, -1.082531754730549967 ) ) ;
#24742=CARTESIAN_POINT ( 'NONE',  ( 6.831329296439236032, 9.063246493969506545, -1.599625672291267398 ) ) ;
#24743=CARTESIAN_POINT ( 'NONE',  ( 4.835665178762361904, 4.878023855840926792, -0.5635330974447970709 ) ) ;
#24758=CARTESIAN_POINT ( 'NONE',  ( 7.191674137406095291, 7.354984346587396082, 0.000000000000000000 ) ) ;
#24778=CARTESIAN_POINT ( 'NONE',  ( -5.773793314573309132, 7.829454515125894964, 1.599625672291263179 ) ) ;
#24795=CARTESIAN_POINT ( 'NONE',  ( 5.316205630334249754, 7.295602216847000498, -1.443375672974078316 ) ) ;
#24798=CARTESIAN_POINT ( 'NONE',  ( 5.451787166470912993, 6.493411461371761284, -1.082531754730548412 ) ) ;
#24806=CARTESIAN_POINT ( 'NONE',  ( -4.604090349816896577, 8.398638366325423377, -0.2811922690319359486 ) ) ;
#24809=CARTESIAN_POINT ( 'NONE',  ( -5.370438244788932280, 6.398504386076097283, 1.082531754730549078 ) ) ;
#24839=EDGE_LOOP ( 'NONE', ( #3905, #44652, #18092, #198938, #118887, #60968, #157164, #92105, #40960, #162535, #120254, #160899, #4036, #209285, #121765, #135364, #53042, #15205, #212201, #196370 ) ) ;
#24843=CARTESIAN_POINT ( 'NONE',  ( 4.848976215542928792, 5.686169002002086970, 1.199719254218452047 ) ) ;
#24853=CARTESIAN_POINT ( 'NONE',  ( -7.431277594066160397, 7.842447745931541370, -0.7216878364870338292 ) ) ;
#24855=CARTESIAN_POINT ( 'NONE',  ( 3.512971199272317602, 6.152197928242737923, -1.082531754730549967 ) ) ;
#24873=CARTESIAN_POINT ( 'NONE',  ( -4.882344714696960075, 5.829061934302122161, 1.082531754730549078 ) ) ;
#24903=CARTESIAN_POINT ( 'NONE',  ( -7.065734331377342414, 8.272386803808890576, -1.199719254218452047 ) ) ;
#24906=CARTESIAN_POINT ( 'NONE',  ( -5.098748287191073203, 8.106234214101666780, 1.199719254218452935 ) ) ;
#24907=CARTESIAN_POINT ( 'NONE',  ( -5.064290697676250730, 7.960144884870772763, -1.236948567437242907 ) ) ;
#24911=CARTESIAN_POINT ( 'NONE',  ( -7.065207446052813367, 8.375735120883982532, -1.082531754730549967 ) ) ;
#24919=CARTESIAN_POINT ( 'NONE',  ( -5.002032328799064231, 4.800402236545811441, -0.7998128361456362523 ) ) ;
#24929=CARTESIAN_POINT ( 'NONE',  ( -5.420227550413282636, 9.545625585449309725, 0.7998128361456291469 ) ) ;
#24930=VERTEX_POINT ( 'NONE', #200243 ) ;
#24931=CARTESIAN_POINT ( 'NONE',  ( 5.559975706299111309, 7.414571502401146930, -1.245397951563255834 ) ) ;
#24936=CARTESIAN_POINT ( 'NONE',  ( 3.074666975249065626, 6.809138247757705820, 0.000000000000000000 ) ) ;
#24960=CARTESIAN_POINT ( 'NONE',  ( 3.410758162289653672, 6.136912401716668519, -1.199719254218453823 ) ) ;
#24975=CARTESIAN_POINT ( 'NONE',  ( 6.582202237817778467, 6.781708767774706104, 0.2773405359152263383 ) ) ;
#24976=CARTESIAN_POINT ( 'NONE',  ( -5.790741006368224753, 5.928488393617260321, 0.7216878364870257245 ) ) ;
#25005=CARTESIAN_POINT ( 'NONE',  ( 4.686278372178935392, 5.496354851410763409, 1.199719254218452047 ) ) ;
#25019=CARTESIAN_POINT ( 'NONE',  ( 3.588273936444265289, 7.344317902764286643, -0.3372145678562175064 ) ) ;
#25023=CARTESIAN_POINT ( 'NONE',  ( -6.740338644649361832, 7.892758502626242567, -1.199719254218452047 ) ) ;
#25034=VERTEX_POINT ( 'NONE', #34558 ) ;
#25040=CARTESIAN_POINT ( 'NONE',  ( 3.739016502318667445, 7.584212696005614873, 0.7998128361456271485 ) ) ;
#25050=CARTESIAN_POINT ( 'NONE',  ( 4.733245298435761583, 8.205245971696047746, 0.7015191473903161778 ) ) ;
#25051=CARTESIAN_POINT ( 'NONE',  ( -0.1036471877147697312, 3.479999999999997318, 1.999999999999997780 ) ) ;
#25052=CARTESIAN_POINT ( 'NONE',  ( 5.264264421420239870, 7.666326994050936428, 1.218248458220503094 ) ) ;
#25071=CARTESIAN_POINT ( 'NONE',  ( -5.438755897737433287, 6.374245297895642537, -1.199719254218453823 ) ) ;
#25073=CARTESIAN_POINT ( 'NONE',  ( 5.598591087800349086, 5.496387455380669529, -0.7998128361456481317 ) ) ;
#25075=CARTESIAN_POINT ( 'NONE',  ( -6.947627372360122955, 7.070263120700404968, 0.000000000000000000 ) ) ;
#25081=AXIS2_PLACEMENT_3D ( 'NONE', #98723, #108, #128114 ) ;
#25082=CARTESIAN_POINT ( 'NONE',  ( -5.297016005617503076, 7.750740434075895635, -1.313619143682826396 ) ) ;
#25092=CARTESIAN_POINT ( 'NONE',  ( -5.655159470231558849, 6.730679149092498648, 1.082531754730549078 ) ) ;
#25101=CARTESIAN_POINT ( 'NONE',  ( 3.906157654512984134, 7.571284673658201569, -0.7216878364870338292 ) ) ;
#25105=CARTESIAN_POINT ( 'NONE',  ( -7.761116589180078407, 8.019333873657032541, 0.000000000000000000 ) ) ;
#25115=CARTESIAN_POINT ( 'NONE',  ( -3.174017359375036929, 6.717120995997236221, 0.7216878364870338292 ) ) ;
#25120=CARTESIAN_POINT ( 'NONE',  ( 4.167152111353856547, 5.955039778036558040, 1.599625672291262513 ) ) ;
#25136=ORIENTED_EDGE ( 'NONE', *, *, #161571, .F. ) ;
#25148=CARTESIAN_POINT ( 'NONE',  ( -5.804299160426242388, 6.904675454319632699, -1.082531754730549967 ) ) ;
#25168=AXIS2_PLACEMENT_3D ( 'NONE', #102918, #135429, #186283 ) ;
#25175=CARTESIAN_POINT ( 'NONE',  ( -6.420668264523499147, 9.648474187656182366, 1.199719254218452935 ) ) ;
#25181=CARTESIAN_POINT ( 'NONE',  ( 5.777182853198898904, 6.873039762554409293, -1.082531754730548412 ) ) ;
#25182=CARTESIAN_POINT ( 'NONE',  ( -3.959863383643135393, 6.777535159962392086, 1.199719254218452935 ) ) ;
#25189=CARTESIAN_POINT ( 'NONE',  ( -6.454563648557663846, 9.688018802362710957, -1.199719254218452047 ) ) ;
#25191=CARTESIAN_POINT ( 'NONE',  ( 6.038137670975392446, 7.156622065392123311, -1.170913047369964710 ) ) ;
#25195=CARTESIAN_POINT ( 'NONE',  ( 5.174371902270911150, 6.065797303184739420, 1.199719254218452047 ) ) ;
#25199=CARTESIAN_POINT ( 'NONE',  ( -5.002032328799064231, 4.800402236545811441, -0.7998128361456362523 ) ) ;
#25203=CARTESIAN_POINT ( 'NONE',  ( -4.309512724297390740, 6.121127159803966933, 1.599625672291270506 ) ) ;
#25210=CARTESIAN_POINT ( 'NONE',  ( 4.950135482320912494, 6.868520377498098739, -1.443375672974068769 ) ) ;
#25211=CARTESIAN_POINT ( 'NONE',  ( -4.950135482320918712, 7.828889591799445213, -1.082531754730549967 ) ) ;
#25217=CARTESIAN_POINT ( 'NONE',  ( 3.230585741806197841, 6.991043475407723307, 0.7998128361456271485 ) ) ;
#25218=ORIENTED_EDGE ( 'NONE', *, *, #23600, .F. ) ;
#25226=CARTESIAN_POINT ( 'NONE',  ( 4.393008644795362905, 7.016788222801661590, 1.284222742053114041 ) ) ;
#25229=CARTESIAN_POINT ( 'NONE',  ( 4.725438941449205288, 8.332574750205820280, 0.7120043264817934592 ) ) ;
#25239=CARTESIAN_POINT ( 'NONE',  ( 5.712781623311797397, 7.758274208654143855, -1.599625672291283607 ) ) ;
#25250=CARTESIAN_POINT ( 'NONE',  ( 4.637309883081485395, 8.320457421531981979, 0.4059539251603030974 ) ) ;
#25258=CARTESIAN_POINT ( 'NONE',  ( 6.475954649182838807, 7.584310507915338562, 1.199719254218452047 ) ) ;
#25262=CARTESIAN_POINT ( 'NONE',  ( -4.665006653791238911, 8.307176129776033591, 0.4851093158183654719 ) ) ;
#25269=CARTESIAN_POINT ( 'NONE',  ( -5.824109505522200081, 8.952488968821326054, -1.199719254218452047 ) ) ;
#25273=CARTESIAN_POINT ( 'NONE',  ( -3.707465945607718805, 7.355851012256872323, 0.5743249234583160945 ) ) ;
#25282=CARTESIAN_POINT ( 'NONE',  ( 5.515134625708930649, 9.656350506627580543, 0.000000000000000000 ) ) ;
#25292=CARTESIAN_POINT ( 'NONE',  ( 3.542423274920540432, 7.354853930707762721, -1.734723475976807094E-15 ) ) ;
#25294=CARTESIAN_POINT ( 'NONE',  ( 3.838366886000300404, 6.531826229425389485, -1.082531754730548412 ) ) ;
#25300=TOROIDAL_SURFACE ( 'NONE', #49566, 7.374593666277937665, 0.08000000000000000167 ) ;
#25308=CARTESIAN_POINT ( 'NONE',  ( -5.966997003790217136, 9.975597247814986801, -0.7216878364870338292 ) ) ;
#25309=CARTESIAN_POINT ( 'NONE',  ( 5.709392085130549077, 9.675058176045386205, 0.000000000000000000 ) ) ;
#25321=EDGE_LOOP ( 'NONE', ( #138966, #62331, #140605, #88168, #93539, #84687, #155470, #175835 ) ) ;
#25322=CARTESIAN_POINT ( 'NONE',  ( -4.288121723672178476, 8.224835454251337552, -0.7998128361456362523 ) ) ;
#25323=CARTESIAN_POINT ( 'NONE',  ( -4.553559489343377287, 6.405848385690952718, -1.599625672291271394 ) ) ;
#25325=CARTESIAN_POINT ( 'NONE',  ( 7.987161891782087686, 8.490979426600148372, -0.7216878364870317197 ) ) ;
#25336=CARTESIAN_POINT ( 'NONE',  ( -5.221311770390402174, 7.721201550036163042, -1.200461426208466076 ) ) ;
#25341=CARTESIAN_POINT ( 'NONE',  ( 3.933273961740296087, 6.642551151122080277, 1.082531754730549078 ) ) ;
#25346=CARTESIAN_POINT ( 'NONE',  ( -5.121948170912633991, 9.197632976031879792, -0.7998128361456362523 ) ) ;
#25359=CARTESIAN_POINT ( 'NONE',  ( 6.554440917563797875, 6.611545590104705994, -0.7998128361456481317 ) ) ;
#25394=DIRECTION ( 'NONE',  ( 0.000000000000000000, 0.000000000000000000, 1.000000000000000000 ) ) ;
#25397=CARTESIAN_POINT ( 'NONE',  ( 5.885648082108188461, 8.920320958217979879, 1.082531754730549967 ) ) ;
#25401=CARTESIAN_POINT ( 'NONE',  ( 5.844973620822830895, 8.872867420051733234, 1.082531754730549967 ) ) ;
#25423=CARTESIAN_POINT ( 'NONE',  ( -5.167592825464113915, 6.057888380243431570, 1.199719254218452935 ) ) ;
#25425=CARTESIAN_POINT ( 'NONE',  ( 4.678972410047582464, 8.472901888448573615, -0.7216878364870357165 ) ) ;
#25431=CARTESIAN_POINT ( 'NONE',  ( -3.305155586681401303, 7.078041627762083898, 0.7998128361456352531 ) ) ;
#25436=CARTESIAN_POINT ( 'NONE',  ( -3.526002468005825286, 6.271364091718859335, -1.199719254218450271 ) ) ;
#25438=CARTESIAN_POINT ( 'NONE',  ( -1.854512760316423536, 2.488359591189891251, 2.484105960264900936 ) ) ;
#25443=CARTESIAN_POINT ( 'NONE',  ( -5.123001941117347080, 7.070197912760590064, 1.599625672291263179 ) ) ;
#25449=ORIENTED_EDGE ( 'NONE', *, *, #175830, .F. ) ;
#25456=EDGE_CURVE ( 'NONE', #137116, #117552, #127649, .T. ) ;
#25459=CARTESIAN_POINT ( 'NONE',  ( -4.665414256878301025, 6.536345614481700927, -1.443375672974066548 ) ) ;
#25460=CARTESIAN_POINT ( 'NONE',  ( -5.655159470231558849, 6.730679149092498648, 1.082531754730549078 ) ) ;
#25461=CARTESIAN_POINT ( 'NONE',  ( 6.900173834712277632, 7.014900660111269559, -0.7998128361456341429 ) ) ;
#25462=CARTESIAN_POINT ( 'NONE',  ( -6.414942957921379474, 7.513130201443591005, -1.199719254218452047 ) ) ;
#25484=CARTESIAN_POINT ( 'NONE',  ( 6.526270840131753737, 8.707344961610770540, -1.599625672291283607 ) ) ;
#25508=EDGE_CURVE ( 'NONE', #95167, #213971, #63618, .T. ) ;
#25519=CARTESIAN_POINT ( 'NONE',  ( 4.549643065837591038, 7.465611455855944101, -1.199719254218452047 ) ) ;
#25522=CARTESIAN_POINT ( 'NONE',  ( -3.709037541790315640, 6.484905011134099340, -1.199719254218450271 ) ) ;
#25525=CARTESIAN_POINT ( 'NONE',  ( -5.600926855776888758, 7.627776979863398310, -1.443375672974066548 ) ) ;
#25536=CARTESIAN_POINT ( 'NONE',  ( 5.982890925380405456, 10.20206618957764100, 0.000000000000000000 ) ) ;
#25537=CARTESIAN_POINT ( 'NONE',  ( 5.234329823327693809, 8.264412672927770487, 1.199719254218451159 ) ) ;
#25543=ORIENTED_EDGE ( 'NONE', *, *, #130359, .T. ) ;
#25549=CARTESIAN_POINT ( 'NONE',  ( 4.441177836928239309, 7.339068688795062911, 1.199719254218452047 ) ) ;
#25560=CARTESIAN_POINT ( 'NONE',  ( 5.872089928494542477, 9.864872326636710653, 0.000000000000000000 ) ) ;
#25561=CARTESIAN_POINT ( 'NONE',  ( -3.363831509966360489, 6.938570838353784076, -0.7216878364870458196 ) ) ;
#25562=CARTESIAN_POINT ( 'NONE',  ( -7.045397100956844127, 8.248660034984974132, -1.199719254218452047 ) ) ;
#25570=DIRECTION ( 'NONE',  ( 1.000000000000000000, 0.000000000000000000, 0.000000000000000000 ) ) ;
#25573=CARTESIAN_POINT ( 'NONE',  ( 6.150558962454855561, 7.204682206732687000, 1.199719254218452047 ) ) ;
#25574=CARTESIAN_POINT ( 'NONE',  ( 5.417364897112183719, 8.477953592343014932, 1.199719254218451159 ) ) ;
#25577=CARTESIAN_POINT ( 'NONE',  ( 4.217995187182922656, 6.014356699837137832, 1.443375672974058777 ) ) ;
#25579=EDGE_LOOP ( 'NONE', ( #160454, #171920, #134662, #83234 ) ) ;
#25594=CARTESIAN_POINT ( 'NONE',  ( 4.061549535745618833, 6.896169004081968090, -1.199719254218452047 ) ) ;
#25596=DIRECTION ( 'NONE',  ( -1.000000000000000000, 0.000000000000000000, 0.000000000000000000 ) ) ;
#25599=CARTESIAN_POINT ( 'NONE',  ( 4.766573523656222555, 7.718696989977711809, 1.199719254218452047 ) ) ;
#25605=CARTESIAN_POINT ( 'NONE',  ( 7.693325821111733021, 7.940244644243982464, -0.7998128361456341429 ) ) ;
#25610=CARTESIAN_POINT ( 'NONE',  ( 5.641601317062233001, 7.675230518029648508, -1.443375672974078761 ) ) ;
#25612=CARTESIAN_POINT ( 'NONE',  ( -5.818384198920079520, 6.817144982608731141, 1.199719254218452935 ) ) ;
#25613=CARTESIAN_POINT ( 'NONE',  ( 4.030516805012513082, 7.924296382481737844, 0.000000000000000000 ) ) ;
#25620=CARTESIAN_POINT ( 'NONE',  ( -5.674335135020206700, 6.369890614947046892, -0.8991698295912193828 ) ) ;
#25623=CARTESIAN_POINT ( 'NONE',  ( -4.285259070371116863, 7.157163461145040095, 1.199719254218452935 ) ) ;
#25651=CARTESIAN_POINT ( 'NONE',  ( 4.909461021924256485, 4.900328411765999981, 0.7216878364870338292 ) ) ;
#25657=CARTESIAN_POINT ( 'NONE',  ( 5.806634928402749196, 9.996434193103704402, -0.7998128361456481317 ) ) ;
#25659=CARTESIAN_POINT ( 'NONE',  ( 3.838366886000300404, 6.531826229425389485, -1.082531754730548412 ) ) ;
#25672=CARTESIAN_POINT ( 'NONE',  ( -5.315678745009726924, 8.359319748223434487, -1.199719254218453823 ) ) ;
#25674=CARTESIAN_POINT ( 'NONE',  ( 5.668717623845194176, 9.627604637879139560, 0.000000000000000000 ) ) ;
#25684=CARTESIAN_POINT ( 'NONE',  ( -5.472651281771599763, 6.413789912602166687, 1.199719254218452935 ) ) ;
#25689=DIRECTION ( 'NONE',  ( 5.329070518200750605E-15, 0.000000000000000000, 1.000000000000000000 ) ) ;
#25691=CARTESIAN_POINT ( 'NONE',  ( -3.201133666602369310, 6.748756687762456963, -0.7216878364870458196 ) ) ;
#25695=CARTESIAN_POINT ( 'NONE',  ( -4.309512724297390740, 6.121127159803966933, 1.599625672291270506 ) ) ;
#25717=CARTESIAN_POINT ( 'NONE',  ( -6.794571259104023930, 7.956029886156682274, 1.199719254218452047 ) ) ;
#25719=CARTESIAN_POINT ( 'NONE',  ( -5.815521545619021460, 5.749472989502435460, -0.7998128361456362523 ) ) ;
#25727=CARTESIAN_POINT ( 'NONE',  ( -6.238615401616060652, 7.011456692927672485, -1.010807710288418981 ) ) ;
#25743=CARTESIAN_POINT ( 'NONE',  ( -4.471156797456668386, 8.438376373666578445, -0.7998128361456362523 ) ) ;
#25767=ADVANCED_FACE ( 'NONE', ( #28991 ), #155649, .T. ) ;
#25770=CARTESIAN_POINT ( 'NONE',  ( 5.905458427204159477, 9.047396044116986502, 1.199719254218452047 ) ) ;
#25772=CARTESIAN_POINT ( 'NONE',  ( 5.342795052237045539, 8.390955439988655229, -1.199719254218450271 ) ) ;
#25781=CARTESIAN_POINT ( 'NONE',  ( 6.463880482550782958, 6.803305507656864037, -0.5117977836574041373 ) ) ;
#25786=CARTESIAN_POINT ( 'NONE',  ( 6.326190869690321961, 6.855918622363850190, 0.6739092513716876676 ) ) ;
#25788=CARTESIAN_POINT ( 'NONE',  ( 6.753369913382843315, 8.011924666102361314, -1.082531754730548412 ) ) ;
#25797=CARTESIAN_POINT ( 'NONE',  ( -5.659602779061863487, 5.567567761852417085, 0.7998128361456281477 ) ) ;
#25805=CARTESIAN_POINT ( 'NONE',  ( -6.916067756302494374, 7.241369601873926420, 0.000000000000000000 ) ) ;
#25809=CARTESIAN_POINT ( 'NONE',  ( -4.226151626080061341, 7.204621842858783154, -0.9994034082375232719 ) ) ;
#25811=AXIS2_PLACEMENT_3D ( 'NONE', #6429, #103967, #72503 ) ;
#25814=CARTESIAN_POINT ( 'NONE',  ( -3.851398154733808088, 6.650992392901508232, -1.199719254218450271 ) ) ;
#25821=CARTESIAN_POINT ( 'NONE',  ( 0.000000000000000000, 0.000000000000000000, 0.000000000000000000 ) ) ;
#25823=CARTESIAN_POINT ( 'NONE',  ( 6.047819040147648373, 9.213483425884394507, 1.199719254218452047 ) ) ;
#25837=CARTESIAN_POINT ( 'NONE',  ( -4.858757509019083543, 5.629766575900002401, -2.420000000000000373 ) ) ;
#25840=EDGE_CURVE ( 'NONE', #212849, #9659, #156179, .T. ) ;
#25842=ORIENTED_EDGE ( 'NONE', *, *, #173321, .F. ) ;
#25843=CARTESIAN_POINT ( 'NONE',  ( -5.399890319992785237, 9.521898816625391504, 0.7998128361456291469 ) ) ;
#25847=CARTESIAN_POINT ( 'NONE',  ( -6.452141306522730879, 6.789529044577018446, 0.3774816029595753353 ) ) ;
#25859=EDGE_CURVE ( 'NONE', #90338, #89251, #175631, .T. ) ;
#25864=CARTESIAN_POINT ( 'NONE',  ( 6.061904079085887354, 6.244845311787889486, 0.000000000000000000 ) ) ;
#25871=CARTESIAN_POINT ( 'NONE',  ( 8.025500584646550806, 8.327781868367935658, 0.000000000000000000 ) ) ;
#25875=CARTESIAN_POINT ( 'NONE',  ( -5.153507786970285665, 5.185049637652990207, -0.7216878364870338292 ) ) ;
#25885=CYLINDRICAL_SURFACE ( 'NONE', #50193, 0.07999999999999954370 ) ;
#25907=CARTESIAN_POINT ( 'NONE',  ( 3.715816618597135523, 6.492813934075403637, -1.199719254218453823 ) ) ;
#25921=CARTESIAN_POINT ( 'NONE',  ( -5.804299160426229953, 8.825413882922319431, -1.082531754730549967 ) ) ;
#25923=CARTESIAN_POINT ( 'NONE',  ( 4.882344714252594642, 4.868692719482363707, 0.000000000000000000 ) ) ;
#25934=DIRECTION ( 'NONE',  ( 0.6507913734559658270, 0.7592566023652989049, 0.000000000000000000 ) ) ;
#25942=CARTESIAN_POINT ( 'NONE',  ( -3.336715202739028552, 6.906935146588564223, 0.7216878364870338292 ) ) ;
#25968=CARTESIAN_POINT ( 'NONE',  ( 5.579538156164684182, 5.837173214716261604, -0.7738445141641551173 ) ) ;
#25973=CARTESIAN_POINT ( 'NONE',  ( -5.921879234118920365, 10.13088588310589699, 0.000000000000000000 ) ) ;
#25976=CARTESIAN_POINT ( 'NONE',  ( -5.074494633264801990, 9.142270515442742607, 0.7998128361456291469 ) ) ;
#25977=CARTESIAN_POINT ( 'NONE',  ( -5.604063331876898424, 5.713547423438217976, 0.3306394700328639802 ) ) ;
#25981=CARTESIAN_POINT ( 'NONE',  ( -7.227905289416804102, 8.565549271475310533, -1.082531754730549967 ) ) ;
#25982=CARTESIAN_POINT ( 'NONE',  ( 7.526184668917440312, 8.913541880892736913, -1.082531754730548412 ) ) ;
#25988=CARTESIAN_POINT ( 'NONE',  ( -7.923814432544069142, 8.209148024248356990, 0.000000000000000000 ) ) ;
#25997=CARTESIAN_POINT ( 'NONE',  ( 5.364009635805341958, 7.578432035813580825, -1.241402483855597039 ) ) ;
#26001=CARTESIAN_POINT ( 'NONE',  ( 6.994027139803230320, 9.253060644560830994, -1.599625672291267398 ) ) ;
#26024=CARTESIAN_POINT ( 'NONE',  ( 2.911969131885072670, 6.619324097166378706, 0.000000000000000000 ) ) ;
#26038=DIRECTION ( 'NONE',  ( 0.000000000000000000, 0.000000000000000000, 1.000000000000000000 ) ) ;
#26039=CARTESIAN_POINT ( 'NONE',  ( 6.597622414017595638, 6.771646741010207471, 0.1687998040609314243 ) ) ;
#26040=CARTESIAN_POINT ( 'NONE',  ( -5.275531169048911728, 6.287779464379406491, -1.082531754730549967 ) ) ;
#26054=EDGE_LOOP ( 'NONE', ( #71518, #119290, #189482, #171422 ) ) ;
#26071=CARTESIAN_POINT ( 'NONE',  ( 4.390861645979372341, 6.216034235099629157, -1.599625672291269396 ) ) ;
#26075=VERTEX_POINT ( 'NONE', #186953 ) ;
#26090=CARTESIAN_POINT ( 'NONE',  ( -4.633854640820660009, 8.628190524257904670, -0.7998128361456362523 ) ) ;
#26092=EDGE_LOOP ( 'NONE', ( #165046, #143177, #119411, #11303, #21838, #46099, #58383 ) ) ;
#26101=ORIENTED_EDGE ( 'NONE', *, *, #139194, .F. ) ;
#26106=CARTESIAN_POINT ( 'NONE',  ( 3.874598038455354665, 7.742391154831717692, -0.7998128361456362523 ) ) ;
#26114=CARTESIAN_POINT ( 'NONE',  ( 4.716156256285582771, 8.225219390492719995, 0.6619851453327877389 ) ) ;
#26117=CARTESIAN_POINT ( 'NONE',  ( 6.210774601750883583, 6.933448576277219111, 0.8519936491524527922 ) ) ;
#26139=CARTESIAN_POINT ( 'NONE',  ( -6.805266759416629618, 6.904175738932996964, 0.000000000000000000 ) ) ;
#26141=CARTESIAN_POINT ( 'NONE',  ( 5.585032934186686226, 5.480569609498057382, 0.000000000000000000 ) ) ;
#26144=CARTESIAN_POINT ( 'NONE',  ( -6.069210040772897052, 7.109775131437022999, -1.199719254218453823 ) ) ;
#26147=CARTESIAN_POINT ( 'NONE',  ( 6.770317605177710085, 8.992066187497757213, 1.599625672291268286 ) ) ;
#26148=DIRECTION ( 'NONE',  ( 0.6507913734559641616, -0.7592566023653004592, 0.000000000000000000 ) ) ;
#26150=EDGE_CURVE ( 'NONE', #179040, #195055, #200853, .T. ) ;
#26153=CARTESIAN_POINT ( 'NONE',  ( -5.018240346111991990, 8.014652766117364990, -1.155606277404798821 ) ) ;
#26167=CARTESIAN_POINT ( 'NONE',  ( 6.238160076063542725, 6.450477308261824305, -0.7216878364870458196 ) ) ;
#26173=CARTESIAN_POINT ( 'NONE',  ( -7.099629715411508890, 8.311931418515415615, 1.199719254218452047 ) ) ;
#26188=CARTESIAN_POINT ( 'NONE',  ( 5.248941747146098180, 6.152795455539095570, -1.199719254218452047 ) ) ;
#26192=CARTESIAN_POINT ( 'NONE',  ( 5.468734858265785093, 7.473552982767156294, 1.599625672291269396 ) ) ;
#26224=DIRECTION ( 'NONE',  ( 0.000000000000000000, 0.000000000000000000, -1.000000000000000000 ) ) ;
#26237=CARTESIAN_POINT ( 'NONE',  ( -3.594320120954326292, 6.247105003538398371, 1.082531754730549967 ) ) ;
#26242=CARTESIAN_POINT ( 'NONE',  ( -4.878955176071358757, 6.785476686873604280, -1.599625672291271394 ) ) ;
#26245=FACE_OUTER_BOUND ( 'NONE', #107397, .T. ) ;
#26251=CARTESIAN_POINT ( 'NONE',  ( -3.156015896931072540, 6.904045323053366268, 0.000000000000000000 ) ) ;
#26253=CARTESIAN_POINT ( 'NONE',  ( 6.546060204425600659, 6.805396270974036987, -0.4351356575816138772 ) ) ;
#26258=CARTESIAN_POINT ( 'NONE',  ( 4.030516805012513082, 7.924296382481737844, 0.000000000000000000 ) ) ;
#26263=CARTESIAN_POINT ( 'NONE',  ( -6.050681693448748177, 10.28115541899069463, 0.7998128361456291469 ) ) ;
#26269=CARTESIAN_POINT ( 'NONE',  ( -6.296835998904160014, 6.311006518335105397, 0.000000000000000000 ) ) ;
#26273=CARTESIAN_POINT ( 'NONE',  ( 5.519577934094861860, 6.572500690266394940, 1.082531754730549078 ) ) ;
#26275=CARTESIAN_POINT ( 'NONE',  ( -6.414416072596849538, 7.616478518518682073, -1.082531754730549967 ) ) ;
#26278=CARTESIAN_POINT ( 'NONE',  ( -4.450819567036170099, 8.414649604842665553, -0.7998128361456361413 ) ) ;
#26283=CARTESIAN_POINT ( 'NONE',  ( 4.472210567661338843, 6.310941310395290493, 1.599625672291261402 ) ) ;
#26312=CARTESIAN_POINT ( 'NONE',  ( 4.595929827128614420, 8.372548788374160722, -0.07784623617661419470 ) ) ;
#26320=CARTESIAN_POINT ( 'NONE',  ( 6.210516883511641772, 9.403297576475722508, 1.199719254218452047 ) ) ;
#26324=CARTESIAN_POINT ( 'NONE',  ( -4.839221724899702259, 8.104102677821947154, -0.8803655321611182361 ) ) ;
#26329=ADVANCED_FACE ( 'NONE', ( #131130 ), #98566, .F. ) ;
#26333=CARTESIAN_POINT ( 'NONE',  ( -7.445362632559989535, 8.715286488521982733, 1.199719254218452047 ) ) ;
#26337=CARTESIAN_POINT ( 'NONE',  ( -3.752568318859959007, 7.355240624044412812, 0.6449737300090957470 ) ) ;
#26346=CARTESIAN_POINT ( 'NONE',  ( 5.013482942003290255, 9.071090208970993274, -0.7998128361456481317 ) ) ;
#26353=CARTESIAN_POINT ( 'NONE',  ( 3.393283585170187688, 7.180857625999046867, 0.7998128361456271485 ) ) ;
#26356=CARTESIAN_POINT ( 'NONE',  ( 6.007671464186834065, 7.141943142040370063, 1.082531754730549967 ) ) ;
#26373=CARTESIAN_POINT ( 'NONE',  ( -4.659162064951642535, 5.464719159645540003, 1.199719254218452935 ) ) ;
#26374=CARTESIAN_POINT ( 'NONE',  ( 7.187230829020129441, 8.518095734345896730, 1.082531754730549967 ) ) ;
#26387=CARTESIAN_POINT ( 'NONE',  ( -6.310394152517827315, 6.326824364217716656, 0.7998128361456281477 ) ) ;
#26388=CARTESIAN_POINT ( 'NONE',  ( -5.581116510680924847, 6.540332679663050541, -1.199719254218453823 ) ) ;
#26390=CARTESIAN_POINT ( 'NONE',  ( 7.322812364712459221, 7.715904978352238430, 0.000000000000000000 ) ) ;
#26393=CARTESIAN_POINT ( 'NONE',  ( 0.000000000000000000, 0.08000000000000020983, 0.000000000000000000 ) ) ;
#26394=CARTESIAN_POINT ( 'NONE',  ( 2.878073747850912412, 6.579779482459851003, -0.7998128361456362523 ) ) ;
#26403=CARTESIAN_POINT ( 'NONE',  ( -6.074251926901598431, 7.043194046877760961, -1.007762736454496988 ) ) ;
#26407=CARTESIAN_POINT ( 'NONE',  ( 3.607878275012302627, 7.223292064240769861, 0.7216878364870257245 ) ) ;
#26412=CARTESIAN_POINT ( 'NONE',  ( -6.577640801285370209, 7.702944352034914566, -1.199719254218452047 ) ) ;
#26428=CARTESIAN_POINT ( 'NONE',  ( 6.204791576909545192, 7.267953590263130259, -1.199719254218452047 ) ) ;
#26463=EDGE_CURVE ( 'NONE', #186231, #49308, #53569, .T. ) ;
#26464=CARTESIAN_POINT ( 'NONE',  ( 6.156811154381533591, 9.236677875870187293, -1.082531754730548412 ) ) ;
#26469=CARTESIAN_POINT ( 'NONE',  ( 6.495764994278795612, 9.632124022417032805, 1.082531754730549078 ) ) ;
#26494=CARTESIAN_POINT ( 'NONE',  ( -3.820365424000704557, 7.679119771301277098, -0.7998128361456481317 ) ) ;
#26496=CARTESIAN_POINT ( 'NONE',  ( 4.367134876933267407, 8.109091433148536865, 0.000000000000000000 ) ) ;
#26501=CARTESIAN_POINT ( 'NONE',  ( -3.820365424000704557, 7.679119771301277098, -0.7998128361456481317 ) ) ;
#26506=CARTESIAN_POINT ( 'NONE',  ( -3.959863383643135393, 6.777535159962392086, 1.199719254218452935 ) ) ;
#26514=CARTESIAN_POINT ( 'NONE',  ( -4.014095998097799267, 6.840806543492835345, -1.199719254218450271 ) ) ;
#26523=CARTESIAN_POINT ( 'NONE',  ( -5.157951095356222204, 4.982307464195829816, 0.000000000000000000 ) ) ;
#26527=CARTESIAN_POINT ( 'NONE',  ( -6.617788377246196951, 7.853746207276256719, -1.082531754730549967 ) ) ;
#26528=CARTESIAN_POINT ( 'NONE',  ( -4.950135482320918712, 7.828889591799445213, -1.082531754730549967 ) ) ;
#26529=CARTESIAN_POINT ( 'NONE',  ( 5.688527969385528849, 8.794310509995222347, -1.199719254218452047 ) ) ;
#26530=CARTESIAN_POINT ( 'NONE',  ( -6.818824913030298696, 6.919993584815607335, 0.7998128361456341429 ) ) ;
#26548=CARTESIAN_POINT ( 'NONE',  ( 7.523848900940885542, 7.742521570711348389, 0.7998128361456291469 ) ) ;
#26569=CARTESIAN_POINT ( 'NONE',  ( 4.607021725950278146, 8.475092030744066918, 0.2235605714990263060 ) ) ;
#26576=B_SPLINE_CURVE_WITH_KNOTS ( 'NONE', 3,
 ( #165340, #131826, #197835, #34270, #16935, #100342 ),
 .UNSPECIFIED., .F., .F.,
 ( 4, 2, 4 ),
 ( 0.000000000000000000, 0.002403146417856977853, 0.004806292835713955706 ),
 .UNSPECIFIED. ) ;
#26586=CARTESIAN_POINT ( 'NONE',  ( 7.198453214212898743, 7.362893269528701268, 0.7998128361456291469 ) ) ;
#26589=CARTESIAN_POINT ( 'NONE',  ( -3.169574050544739841, 6.919863168935977527, -0.7998128361456481317 ) ) ;
#26592=CARTESIAN_POINT ( 'NONE',  ( -7.729556973122450714, 8.190440354830551328, 0.000000000000000000 ) ) ;
#26593=CARTESIAN_POINT ( 'NONE',  ( 4.882344714252594642, 4.868692719482363707, 0.000000000000000000 ) ) ;
#26603=CARTESIAN_POINT ( 'NONE',  ( 6.210516883511641772, 9.403297576475722508, 1.199719254218452047 ) ) ;
#26604=CARTESIAN_POINT ( 'NONE',  ( 6.042093733545556233, 7.078139439671806699, -1.199719254218452047 ) ) ;
#26619=CARTESIAN_POINT ( 'NONE',  ( 4.538947565524982686, 8.517465603079630299, 0.000000000000000000 ) ) ;
#26620=VERTEX_POINT ( 'NONE', #101756 ) ;
#26629=CARTESIAN_POINT ( 'NONE',  ( 7.349928672384119288, 8.707909884937221179, 1.082531754730549967 ) ) ;
#26630=CARTESIAN_POINT ( 'NONE',  ( -5.478903473698255588, 7.485416367438324059, -1.443375672974066548 ) ) ;
#26631=CARTESIAN_POINT ( 'NONE',  ( -6.261886844665283114, 8.398896966899865646, 1.599625672291269396 ) ) ;
#26645=CARTESIAN_POINT ( 'NONE',  ( 5.716698046817569434, 6.698511138489155137, -1.199719254218452047 ) ) ;
#26646=CARTESIAN_POINT ( 'NONE',  ( 7.225569521440261767, 7.394528961293920233, -0.7998128361456341429 ) ) ;
#26649=CARTESIAN_POINT ( 'NONE',  ( 3.567203813726949058, 7.175838526074521440, 0.7216878364870257245 ) ) ;
#26655=DIRECTION ( 'NONE',  ( -0.7592566023653005702, 0.6507913734559640506, 0.000000000000000000 ) ) ;
#26666=CARTESIAN_POINT ( 'NONE',  ( 4.980641328173811999, 6.904110530993182948, 1.599625672291269396 ) ) ;
#26671=CARTESIAN_POINT ( 'NONE',  ( 6.062430963966053632, 7.101866208495718702, -1.199719254218452047 ) ) ;
#26682=CARTESIAN_POINT ( 'NONE',  ( 5.207740401424913124, 9.089797878388800711, -0.7216878364870458196 ) ) ;
#26684=CARTESIAN_POINT ( 'NONE',  ( -4.308458954092677651, 8.248562223075252220, -0.7998128361456362523 ) ) ;
#26685=CARTESIAN_POINT ( 'NONE',  ( 5.554000203453580475, 6.508696987897830688, -1.199719254218452047 ) ) ;
#26696=CARTESIAN_POINT ( 'NONE',  ( -4.390861645979385663, 6.216034235099629157, -1.599625672291271394 ) ) ;
#26709=AXIS2_PLACEMENT_3D ( 'NONE', #107982, #110116, #92754 ) ;
#26714=VERTEX_POINT ( 'NONE', #84436 ) ;
#26729=CARTESIAN_POINT ( 'NONE',  ( 8.018721507839716267, 8.319872945426633137, -0.7998128361456341429 ) ) ;
#26730=CARTESIAN_POINT ( 'NONE',  ( 5.031484404002891431, 5.042689024191078673, 0.7216878364870328300 ) ) ;
#26741=CARTESIAN_POINT ( 'NONE',  ( -6.140917232347002042, 6.129101290685087911, -0.7998128361456362523 ) ) ;
#26743=CARTESIAN_POINT ( 'NONE',  ( -6.635789839245807897, 6.706452665400368218, 0.7998128361456341429 ) ) ;
#26745=CARTESIAN_POINT ( 'NONE',  ( 6.170369307550806148, 10.21286493553572328, 0.7216878364870317197 ) ) ;
#26747=B_SPLINE_CURVE_WITH_KNOTS ( 'NONE', 3,
 ( #110888, #125027, #108758, #192049, #190984, #79389 ),
 .UNSPECIFIED., .F., .F.,
 ( 4, 2, 4 ),
 ( 0.001373143222731355991, 0.001435267353687973493, 0.001497391484644590995 ),
 .UNSPECIFIED. ) ;
#26749=CARTESIAN_POINT ( 'NONE',  ( -3.771179864959864680, 7.354219769063552015, -0.6724184775293801097 ) ) ;
#26755=CARTESIAN_POINT ( 'NONE',  ( -6.784929528996132220, 6.880448970109080520, 0.000000000000000000 ) ) ;
#26762=CARTESIAN_POINT ( 'NONE',  ( -5.478903473698260029, 6.525047153136981137, -1.082531754730549967 ) ) ;
#26766=CARTESIAN_POINT ( 'NONE',  ( -6.134138155540168391, 6.121192367743780949, 0.000000000000000000 ) ) ;
#26785=CARTESIAN_POINT ( 'NONE',  ( -6.282224075085783177, 8.422623735723785643, 1.599625672291269396 ) ) ;
#26787=CARTESIAN_POINT ( 'NONE',  ( -5.492988512192097161, 6.437516681426083132, 1.199719254218452935 ) ) ;
#26815=CARTESIAN_POINT ( 'NONE',  ( -4.945692173934974178, 8.992000979557944973, 0.000000000000000000 ) ) ;
#26822=CARTESIAN_POINT ( 'NONE',  ( 3.903294069008342415, 8.999999999999998224, 0.7749999999999996891 ) ) ;
#26842=CARTESIAN_POINT ( 'NONE',  ( 5.481239241674765950, 9.616805891921051952, -0.7998128361456481317 ) ) ;
#26854=CARTESIAN_POINT ( 'NONE',  ( 4.909045613421183063, 8.010784895652180992, 0.9812996480243344477 ) ) ;
#26856=CARTESIAN_POINT ( 'NONE',  ( 5.546694241766559230, 9.485244025454063532, 0.000000000000000000 ) ) ;
#26864=CARTESIAN_POINT ( 'NONE',  ( -5.093022980588950865, 5.970890227889075419, -1.199719254218453823 ) ) ;
#26872=CARTESIAN_POINT ( 'NONE',  ( -6.794044373779495771, 8.059378203231773341, 1.082531754730549078 ) ) ;
#26876=CARTESIAN_POINT ( 'NONE',  ( 6.047819040147648373, 9.213483425884394507, 1.199719254218452047 ) ) ;
#26882=CARTESIAN_POINT ( 'NONE',  ( -2.959422669532919326, 6.674686557755516780, 0.7998128361456352531 ) ) ;
#26891=CARTESIAN_POINT ( 'NONE',  ( 6.831329296439236032, 9.063246493969506545, -1.599625672291267398 ) ) ;
#26897=CARTESIAN_POINT ( 'NONE',  ( -3.231779075379149546, 6.036511184309975242, 0.9899555337401846344 ) ) ;
#26908=CARTESIAN_POINT ( 'NONE',  ( -5.074494633264801990, 9.142270515442742607, 0.7998128361456291469 ) ) ;
#26910=CARTESIAN_POINT ( 'NONE',  ( 6.964048179274811012, 8.153752959689313684, 1.199719254218452047 ) ) ;
#26929=CARTESIAN_POINT ( 'NONE',  ( 4.556949027968946631, 8.330541276023501140, -0.7216878364870357165 ) ) ;
#26941=CARTESIAN_POINT ( 'NONE',  ( -6.129694847154222970, 7.284303755502281597, -1.082531754730549967 ) ) ;
#26952=DIRECTION ( 'NONE',  ( 0.000000000000000000, 0.000000000000000000, -1.000000000000000000 ) ) ;
#26974=CARTESIAN_POINT ( 'NONE',  ( 5.713835393516482952, 5.630839145382857680, 0.7998128361456352531 ) ) ;
#26984=CARTESIAN_POINT ( 'NONE',  ( -6.129694847154211423, 9.205042184104968328, -1.082531754730549967 ) ) ;
#26986=CARTESIAN_POINT ( 'NONE',  ( 6.556249800660121529, 9.806652646482286073, 1.199719254218452047 ) ) ;
#26993=CYLINDRICAL_SURFACE ( 'NONE', #183941, 1.250000000000000000 ) ;
#26997=CIRCLE ( 'NONE', #54680, 0.08000000000000020983 ) ;
#27004=CARTESIAN_POINT ( 'NONE',  ( -3.201133666602369310, 6.748756687762456963, -0.7216878364870458196 ) ) ;
#27010=CARTESIAN_POINT ( 'NONE',  ( -6.305925513666572613, 6.529536985466737775, -1.006778644550405474E-06 ) ) ;
#27038=CARTESIAN_POINT ( 'NONE',  ( -5.250750630242457362, 9.347902511916677426, 0.000000000000000000 ) ) ;
#27039=CARTESIAN_POINT ( 'NONE',  ( -4.702355942707336034, 8.355867970554191615, 0.6817663069898479700 ) ) ;
#27040=CARTESIAN_POINT ( 'NONE',  ( -4.308458954092677651, 8.248562223075252220, -0.7998128361456361413 ) ) ;
#27048=CARTESIAN_POINT ( 'NONE',  ( -2.993318053567081360, 6.714231172462041819, 0.000000000000000000 ) ) ;
#27053=CARTESIAN_POINT ( 'NONE',  ( -3.467853430045390706, 7.267855778353407459, 0.7998128361456352531 ) ) ;
#27058=ORIENTED_EDGE ( 'NONE', *, *, #33667, .T. ) ;
#27068=CARTESIAN_POINT ( 'NONE',  ( 4.899292406491845497, 6.809203455697518947, -1.599625672291273171 ) ) ;
#27076=LINE ( 'NONE', #138725, #73386 ) ;
#27093=CARTESIAN_POINT ( 'NONE',  ( 5.662465432362883355, 6.635239754958710989, 1.199719254218451159 ) ) ;
#27094=CARTESIAN_POINT ( 'NONE',  ( 3.400062661977048428, 7.188766548940353829, -1.734723475976807094E-15 ) ) ;
#27107=CARTESIAN_POINT ( 'NONE',  ( 5.043764445095213489, 7.992138250556588552, 1.161813593947092382 ) ) ;
#27108=CARTESIAN_POINT ( 'NONE',  ( -3.323157048681004699, 6.891117300187535655, -0.7216878364870458196 ) ) ;
#27133=EDGE_LOOP ( 'NONE', ( #28143, #191240, #191270, #78171, #165185 ) ) ;
#27138=CARTESIAN_POINT ( 'NONE',  ( 5.174371902270911150, 6.065797303184739420, 1.199719254218452047 ) ) ;
#27143=EDGE_CURVE ( 'NONE', #141262, #79190, #104938, .T. ) ;
#27159=CARTESIAN_POINT ( 'NONE',  ( -6.257970421159510188, 9.458660037064859694, 1.199719254218452047 ) ) ;
#27173=CARTESIAN_POINT ( 'NONE',  ( 5.747730777550676073, 5.670383760089384495, 0.000000000000000000 ) ) ;
#27183=CARTESIAN_POINT ( 'NONE',  ( -6.102578539482539810, 6.292298848917299736, 0.000000000000000000 ) ) ;
#27184=CARTESIAN_POINT ( 'NONE',  ( 5.309622429108474151, 7.625948988765205883, 1.230663689527239812 ) ) ;
#27186=CARTESIAN_POINT ( 'NONE',  ( -6.328551337425281531, 6.876786110265634910, 0.7058904598814246256 ) ) ;
#27204=CARTESIAN_POINT ( 'NONE',  ( -4.945692173934974178, 8.992000979557944973, 0.000000000000000000 ) ) ;
#27206=CARTESIAN_POINT ( 'NONE',  ( 3.898851692381625877, 6.706354853490643642, -1.199719254218452047 ) ) ;
#27210=CARTESIAN_POINT ( 'NONE',  ( -6.774234028683526532, 7.932303117332766718, 1.199719254218452047 ) ) ;
#27213=CARTESIAN_POINT ( 'NONE',  ( 5.826972158823246595, 10.02016096192762085, -0.7998128361456481317 ) ) ;
#27218=CARTESIAN_POINT ( 'NONE',  ( -5.476171693740270463, 7.594609835490887306, -1.347918582746489902 ) ) ;
#27234=CARTESIAN_POINT ( 'NONE',  ( 4.095971805104276164, 7.792734516014745871, 0.7216878364870257245 ) ) ;
#27238=CARTESIAN_POINT ( 'NONE',  ( -5.576146316970437944, 9.727530813099326323, 0.000000000000000000 ) ) ;
#27252=CARTESIAN_POINT ( 'NONE',  ( 5.194709132691408549, 6.089524072008651423, 1.199719254218452935 ) ) ;
#27263=AXIS2_PLACEMENT_3D ( 'NONE', #57880, #107772, #21075 ) ;
#27277=EDGE_CURVE ( 'NONE', #122390, #83476, #63019, .T. ) ;
#27304=CARTESIAN_POINT ( 'NONE',  ( -7.608060475923978494, 8.905100639113307182, 1.199719254218452047 ) ) ;
#27310=EDGE_CURVE ( 'NONE', #127442, #51151, #192197, .T. ) ;
#27312=CARTESIAN_POINT ( 'NONE',  ( -5.773793314573309132, 7.829454515125894964, 1.599625672291263179 ) ) ;
#27323=CARTESIAN_POINT ( 'NONE',  ( -5.224688093219839402, 7.188831756880171397, -1.599625672291271394 ) ) ;
#27325=CARTESIAN_POINT ( 'NONE',  ( 5.561552386509557522, 7.525632394756676113, -1.337405013919689800 ) ) ;
#27330=CARTESIAN_POINT ( 'NONE',  ( 5.020262018810099924, 9.078999131912302900, 0.7998128361456331437 ) ) ;
#27334=AXIS2_PLACEMENT_3D ( 'NONE', #141452, #59078, #105735 ) ;
#27337=CARTESIAN_POINT ( 'NONE',  ( -5.725286006720766707, 9.901527117808042178, 0.7998128361456291469 ) ) ;
#27342=CARTESIAN_POINT ( 'NONE',  ( -5.204350862799341115, 7.165104988056252289, -1.599625672291271394 ) ) ;
#27347=CARTESIAN_POINT ( 'NONE',  ( 5.736508391913541338, 6.825586224388162648, -1.082531754730548412 ) ) ;
#27348=CARTESIAN_POINT ( 'NONE',  ( -6.739811759324840779, 7.035737605399991601, -0.7216878364870338292 ) ) ;
#27357=CARTESIAN_POINT ( 'NONE',  ( 3.718679271898170491, 7.560485927181699317, 0.7998128361456271485 ) ) ;
#27363=CARTESIAN_POINT ( 'NONE',  ( 5.398914348987485567, 6.259949555863199677, 2.419999999999999485 ) ) ;
#27384=CARTESIAN_POINT ( 'NONE',  ( 4.622017735560743468, 8.339529265130579461, 0.3277269337885590494 ) ) ;
#27393=CARTESIAN_POINT ( 'NONE',  ( 7.180978637093494044, 8.406838493811077839, -1.199719254218452047 ) ) ;
#27398=CARTESIAN_POINT ( 'NONE',  ( -4.695470500997839025, 8.269974592382618894, -0.5850018098894956831 ) ) ;
#27406=CARTESIAN_POINT ( 'NONE',  ( -6.851666526859749418, 9.086973262793417661, -1.599625672291271394 ) ) ;
#27412=CARTESIAN_POINT ( 'NONE',  ( -4.683370693966717901, 4.898792820011970583, -0.6382510007943015262 ) ) ;
#27418=CARTESIAN_POINT ( 'NONE',  ( 6.607619761813720238, 8.802252036906432764, 1.599625672291268286 ) ) ;
#27424=STYLED_ITEM ( 'NONE', ( #34451 ), #210156 ) ;
#27425=CARTESIAN_POINT ( 'NONE',  ( -0.1054627972275519465, 3.385846599571567417, -2.076146368081344118 ) ) ;
#27428=CARTESIAN_POINT ( 'NONE',  ( 3.040771591214902259, 6.769593633051179005, -0.7998128361456362523 ) ) ;
#27431=CARTESIAN_POINT ( 'NONE',  ( 5.844973620822844218, 5.991759777147701804, 0.7216878364870328300 ) ) ;
#27438=CARTESIAN_POINT ( 'NONE',  ( -5.536209915801717507, 7.449110030843877794, 1.248366777010925910 ) ) ;
#27441=ORIENTED_EDGE ( 'NONE', *, *, #132097, .F. ) ;
#27444=CARTESIAN_POINT ( 'NONE',  ( -3.474632506852224356, 7.275764701294714420, -0.7998128361456481317 ) ) ;
#27445=CARTESIAN_POINT ( 'NONE',  ( 6.156811154381533591, 9.236677875870187293, -1.082531754730548412 ) ) ;
#27457=CARTESIAN_POINT ( 'NONE',  ( -6.961185525973791144, 7.086080966583015339, 0.7998128361456341429 ) ) ;
#27458=CARTESIAN_POINT ( 'NONE',  ( -6.310394152517827315, 6.326824364217716656, 0.7998128361456281477 ) ) ;
#27460=CARTESIAN_POINT ( 'NONE',  ( 5.831415467209187575, 9.817418788470464008, 0.000000000000000000 ) ) ;
#27464=CARTESIAN_POINT ( 'NONE',  ( 3.390420931869152721, 6.113185632892752075, -1.199719254218452047 ) ) ;
#27473=CARTESIAN_POINT ( 'NONE',  ( -6.329889402343163773, 6.869280899661572626, -0.6830204514151876349 ) ) ;
#27478=CARTESIAN_POINT ( 'NONE',  ( 4.746763178560250651, 7.591621904078704297, 1.082531754730549078 ) ) ;
#27483=CARTESIAN_POINT ( 'NONE',  ( -5.607179047703544583, 8.699403434699558346, 1.199719254218454489 ) ) ;
#27499=CARTESIAN_POINT ( 'NONE',  ( 4.694866332082116678, 8.699370830729650450, 0.7998128361456341429 ) ) ;
#27536=CARTESIAN_POINT ( 'NONE',  ( 7.675324359112103423, 8.127168971818530707, 0.7216878364870267237 ) ) ;
#27565=CARTESIAN_POINT ( 'NONE',  ( -3.806807270387036368, 7.663301925418665839, 0.000000000000000000 ) ) ;
#27567=CARTESIAN_POINT ( 'NONE',  ( 6.034787771414195312, 6.213209619504250547, -0.7216878364870458196 ) ) ;
#27572=CARTESIAN_POINT ( 'NONE',  ( -5.764151584465413869, 6.753873599078290546, -1.199719254218453823 ) ) ;
#27577=CARTESIAN_POINT ( 'NONE',  ( -4.228163802615396705, 6.026220084508304708, -1.599625672291271394 ) ) ;
#27585=CARTESIAN_POINT ( 'NONE',  ( -5.152980901645737077, 8.169505597632108262, -1.199719254218453823 ) ) ;
#27594=CARTESIAN_POINT ( 'NONE',  ( -3.688700311369816909, 6.461178242310183784, -1.199719254218450271 ) ) ;
#27597=CARTESIAN_POINT ( 'NONE',  ( -5.722950238744243023, 7.770137593325314285, 1.443375672974058777 ) ) ;
#27598=CARTESIAN_POINT ( 'NONE',  ( -4.462041952228942954, 8.219816354326809460, -0.7216878364870338292 ) ) ;
#27599=CARTESIAN_POINT ( 'NONE',  ( 6.550524494058025837, 7.671308660269694712, -1.199719254218452047 ) ) ;
#27600=CARTESIAN_POINT ( 'NONE',  ( -6.740338644649361832, 7.892758502626242567, -1.199719254218452047 ) ) ;
#27619=CARTESIAN_POINT ( 'NONE',  ( 8.188198428010544205, 8.517596018959260107, 0.000000000000000000 ) ) ;
#27639=CARTESIAN_POINT ( 'NONE',  ( 4.913571454530422322, 8.125067815752732514, -1.031885869761673069 ) ) ;
#27646=( BOUNDED_CURVE ( )  B_SPLINE_CURVE ( 2, ( #206898, #154970, #171208 ),
 .UNSPECIFIED., .F., .T. ) 
 B_SPLINE_CURVE_WITH_KNOTS ( ( 3, 3 ),
 ( 0.2500000000000002776, 0.2551636414462434277 ),
 .UNSPECIFIED. ) 
 CURVE ( )  GEOMETRIC_REPRESENTATION_ITEM ( )  RATIONAL_B_SPLINE_CURVE ( ( 0.9999999999999955591, 0.9169843866685133404, 0.9368478601411348583 ) ) 
 REPRESENTATION_ITEM ( '' )  );
#27650=B_SPLINE_CURVE_WITH_KNOTS ( 'NONE', 3,
 ( #206665, #176322, #174208, #25781, #160061, #192542, #91893, #157949, #28998, #126581, #109257, #10594 ),
 .UNSPECIFIED., .F., .F.,
 ( 4, 2, 2, 2, 2, 4 ),
 ( 0.000000000000000000, 0.0006161371811066557137, 0.001232274362213311427, 0.001540342952766639338, 0.001848411543319967466, 0.002464548724426622421 ),
 .UNSPECIFIED. ) ;
#27655=ADVANCED_FACE ( 'NONE', ( #110104 ), #173752, .T. ) ;
#27656=CARTESIAN_POINT ( 'NONE',  ( 5.013482942003290255, 9.071090208970993274, -0.7998128361456481317 ) ) ;
#27659=FACE_OUTER_BOUND ( 'NONE', #128417, .T. ) ;
#27663=CARTESIAN_POINT ( 'NONE',  ( -7.119440060507479018, 8.439006504414422238, 1.082531754730549078 ) ) ;
#27664=CARTESIAN_POINT ( 'NONE',  ( 4.779848517908583894, 4.883929213520019630, -0.7538207499340529028 ) ) ;
#27675=CARTESIAN_POINT ( 'NONE',  ( 6.912678218121202534, 9.158153569265168770, 1.599625672291268286 ) ) ;
#27676=CARTESIAN_POINT ( 'NONE',  ( 4.681308178468477799, 8.683552984847038303, 0.000000000000000000 ) ) ;
#27690=CARTESIAN_POINT ( 'NONE',  ( 7.035755370848908896, 7.173079118937375931, 0.7998128361456352531 ) ) ;
#27706=CARTESIAN_POINT ( 'NONE',  ( -4.326460416536637155, 8.061637896019123062, 0.000000000000000000 ) ) ;
#27707=CARTESIAN_POINT ( 'NONE',  ( -5.752402313948099533, 9.933162809573264695, -0.7998128361456362523 ) ) ;
#27720=CARTESIAN_POINT ( 'NONE',  ( 7.523848900940885542, 7.742521570711348389, 0.7998128361456291469 ) ) ;
#27723=CARTESIAN_POINT ( 'NONE',  ( 3.404505970362959655, 6.986024375483197879, 0.7216878364870257245 ) ) ;
#27742=CARTESIAN_POINT ( 'NONE',  ( 3.088225128862704949, 6.824956093640315302, 0.7998128361456281477 ) ) ;
#27744=CARTESIAN_POINT ( 'NONE',  ( -3.546339698426324460, 6.295090860542775779, -1.199719254218450271 ) ) ;
#27747=CARTESIAN_POINT ( 'NONE',  ( 6.059568310664962709, 6.034194215389424798, 0.7998128361456352531 ) ) ;
#27757=CARTESIAN_POINT ( 'NONE',  ( 5.831415467653547680, 8.857049574687536619, -1.082531754730548412 ) ) ;
#27759=CARTESIAN_POINT ( 'NONE',  ( -5.607179047703544583, 8.699403434699558346, 1.199719254218454489 ) ) ;
#27760=CARTESIAN_POINT ( 'NONE',  ( 6.201928923608456046, 6.200281597156833691, 0.7998128361456352531 ) ) ;
#27770=CARTESIAN_POINT ( 'NONE',  ( -3.447516199624892419, 7.244129009529488350, 0.7998128361456352531 ) ) ;
#27788=ORIENTED_EDGE ( 'NONE', *, *, #144165, .F. ) ;
#27804=CARTESIAN_POINT ( 'NONE',  ( 5.045042557616584489, 5.058506870073687267, 0.000000000000000000 ) ) ;
#27816=CARTESIAN_POINT ( 'NONE',  ( -3.657667580636712934, 7.489305620709952649, -0.7998128361456481317 ) ) ;
#27818=CARTESIAN_POINT ( 'NONE',  ( -6.099189001301292379, 8.209082816308541197, 1.599625672291263179 ) ) ;
#27820=CARTESIAN_POINT ( 'NONE',  ( 6.414416072596830887, 8.576847732820027659, -1.443375672974078761 ) ) ;
#27830=CARTESIAN_POINT ( 'NONE',  ( -6.394605727500880299, 7.489403432619674561, -1.199719254218452047 ) ) ;
#27837=CARTESIAN_POINT ( 'NONE',  ( -3.675669043080673770, 7.302381293653823491, 0.000000000000000000 ) ) ;
#27841=CARTESIAN_POINT ( 'NONE',  ( -3.637330350216213759, 7.465578851886037093, -0.7998128361456481317 ) ) ;
#27861=CARTESIAN_POINT ( 'NONE',  ( -7.618755976236585958, 7.853246491889623648, 0.000000000000000000 ) ) ;
#27863=CARTESIAN_POINT ( 'NONE',  ( -5.490125858891038213, 5.369844688319787451, -0.7998128361456362523 ) ) ;
#27873=CARTESIAN_POINT ( 'NONE',  ( 6.007671464186845611, 6.181573927739023588, 0.7216878364870273899 ) ) ;
#27874=CARTESIAN_POINT ( 'NONE',  ( -4.009193028827814587, 7.297902834095492786, -0.7581239365674132813 ) ) ;
#27891=CARTESIAN_POINT ( 'NONE',  ( -6.903036488013351679, 8.082572653217566128, -1.199719254218452047 ) ) ;
#27893=ORIENTED_EDGE ( 'NONE', *, *, #198557, .F. ) ;
#27918=CARTESIAN_POINT ( 'NONE',  ( 5.820193082016415609, 10.01225203898631655, 0.000000000000000000 ) ) ;
#27933=CARTESIAN_POINT ( 'NONE',  ( 5.067666882003905471, 7.850148838107081417, 1.122879199148843377 ) ) ;
#27935=CARTESIAN_POINT ( 'NONE',  ( 5.383996398402570271, 9.295429874862735531, 0.000000000000000000 ) ) ;
#27941=CARTESIAN_POINT ( 'NONE',  ( -5.483346782084204563, 5.361935765378481378, 0.000000000000000000 ) ) ;
#27949=CARTESIAN_POINT ( 'NONE',  ( -6.590672069574513792, 6.861741300691274859, 0.000000000000000000 ) ) ;
#27953=CARTESIAN_POINT ( 'NONE',  ( 8.154303043976348420, 8.478051404252736845, 0.7998128361456281477 ) ) ;
#27954=CARTESIAN_POINT ( 'NONE',  ( -4.698419658905671703, 6.826623453404498498, -1.249972656429306772 ) ) ;
#27966=CARTESIAN_POINT ( 'NONE',  ( -5.823017895876262173, 7.308274721394978357, -1.333157625313810879 ) ) ;
#27968=CARTESIAN_POINT ( 'NONE',  ( 7.343676480457483002, 8.596652644402405841, -1.199719254218452047 ) ) ;
#27972=ORIENTED_EDGE ( 'NONE', *, *, #202320, .F. ) ;
#27983=CARTESIAN_POINT ( 'NONE',  ( -3.895996091634230218, 7.334980739573080832, 0.5863762202383783206 ) ) ;
#27987=CARTESIAN_POINT ( 'NONE',  ( -6.831329296439251131, 9.063246493969506545, -1.599625672291271394 ) ) ;
#27989=CARTESIAN_POINT ( 'NONE',  ( 5.345657705538078730, 9.458627433094950021, 0.7998128361456331437 ) ) ;
#27991=CARTESIAN_POINT ( 'NONE',  ( -5.631831469557842418, 7.372220891417233801, 1.235678285582973546 ) ) ;
#27997=CARTESIAN_POINT ( 'NONE',  ( 5.285699784481295183, 7.260012063351913625, 1.599625672291268286 ) ) ;
#28005=CARTESIAN_POINT ( 'NONE',  ( 2.943528747942701695, 6.448217615992859919, 0.000000000000000000 ) ) ;
#28008=CARTESIAN_POINT ( 'NONE',  ( 6.075462232699553766, 6.260663157670496304, -0.7216878364870458196 ) ) ;
#28019=CARTESIAN_POINT ( 'NONE',  ( -5.980555157403903976, 6.149938236492225485, 0.000000000000000000 ) ) ;
#28041=CARTESIAN_POINT ( 'NONE',  ( -4.207966135563084187, 7.175396087857926375, 2.420000000000000373 ) ) ;
#28043=EDGE_CURVE ( 'NONE', #118869, #207685, #91032, .T. ) ;
#28052=VERTEX_POINT ( 'NONE', #68711 ) ;
#28056=CARTESIAN_POINT ( 'NONE',  ( 5.228604516725597229, 6.129068686715179126, -1.199719254218450271 ) ) ;
#28067=CARTESIAN_POINT ( 'NONE',  ( -7.444835747679825033, 7.858265591814152629, 0.000000000000000000 ) ) ;
#28069=CARTESIAN_POINT ( 'NONE',  ( 5.533136087708556694, 5.627949321847663278, 0.000000000000000000 ) ) ;
#28085=CARTESIAN_POINT ( 'NONE',  ( 4.137367429043227851, 8.820713629714100890, 0.7750000000000002442 ) ) ;
#28089=DIRECTION ( 'NONE',  ( 0.000000000000000000, 0.000000000000000000, 1.000000000000000000 ) ) ;
#28091=CARTESIAN_POINT ( 'NONE',  ( 3.570880328030153539, 7.341005539872356600, 0.2896471194287209006 ) ) ;
#28101=ORIENTED_EDGE ( 'NONE', *, *, #3854, .T. ) ;
#28112=CARTESIAN_POINT ( 'NONE',  ( 5.591005849568446706, 5.791977450266268868, -0.7139200525481930182 ) ) ;
#28121=CARTESIAN_POINT ( 'NONE',  ( -6.291865805193673111, 9.498204651771386509, -1.199719254218452047 ) ) ;
#28122=CARTESIAN_POINT ( 'NONE',  ( -4.651396499164954790, 8.416516698401213858, 0.5247324002638984464 ) ) ;
#28123=CARTESIAN_POINT ( 'NONE',  ( -4.281342646865346602, 8.216926531310035031, 0.7998128361456350310 ) ) ;
#28127=CARTESIAN_POINT ( 'NONE',  ( -8.054952659850432184, 8.570068656013202002, 0.000000000000000000 ) ) ;
#28133=CARTESIAN_POINT ( 'NONE',  ( -5.061990249855848667, 6.999017606288844284, -1.599625672291271394 ) ) ;
#28143=ORIENTED_EDGE ( 'NONE', *, *, #7522, .T. ) ;
#28147=CARTESIAN_POINT ( 'NONE',  ( 4.736594563127852098, 6.619389305106191834, -1.599625672291273171 ) ) ;
#28151=ORIENTED_EDGE ( 'NONE', *, *, #100532, .T. ) ;
#28169=CARTESIAN_POINT ( 'NONE',  ( 5.611095471209277541, 7.639640364534566075, 1.599625672291268286 ) ) ;
#28170=CARTESIAN_POINT ( 'NONE',  ( 3.711900195091365262, 7.552577004240394132, -0.7998128361456362523 ) ) ;
#28172=CARTESIAN_POINT ( 'NONE',  ( 4.686278372178935392, 5.496354851410763409, 1.199719254218452047 ) ) ;
#28177=EDGE_CURVE ( 'NONE', #94850, #103686, #148927, .T. ) ;
#28185=CARTESIAN_POINT ( 'NONE',  ( 5.568688238291347403, 7.519645578322940338, 1.337618216391135428 ) ) ;
#28186=CARTESIAN_POINT ( 'NONE',  ( -5.628043163004235794, 5.738674243025936761, 0.7216878364870257245 ) ) ;
#28212=ORIENTED_EDGE ( 'NONE', *, *, #17058, .F. ) ;
#28217=CARTESIAN_POINT ( 'NONE',  ( 3.607351389687783794, 6.366271167014519783, 1.199719254218451159 ) ) ;
#28235=CARTESIAN_POINT ( 'NONE',  ( -6.095272577795516789, 9.268845886473535245, 1.199719254218452047 ) ) ;
#28246=ORIENTED_EDGE ( 'NONE', *, *, #147535, .F. ) ;
#28252=CARTESIAN_POINT ( 'NONE',  ( 6.222266154028957885, 6.224008365980749247, 0.7998128361456352531 ) ) ;
#28263=CARTESIAN_POINT ( 'NONE',  ( 5.614387949662905442, 7.370906683214474953, 1.237392280610301931 ) ) ;
#28264=CARTESIAN_POINT ( 'NONE',  ( 4.796824973295459316, 8.251456047330133714, 0.8599625132450954279 ) ) ;
#28280=CARTESIAN_POINT ( 'NONE',  ( -4.308458954092677651, 8.248562223075252220, -0.7998128361456362523 ) ) ;
#28282=CARTESIAN_POINT ( 'NONE',  ( 5.899733120602060232, 6.912052057904395141, -1.199719254218452047 ) ) ;
#28286=CARTESIAN_POINT ( 'NONE',  ( -7.449279056065764237, 7.655523418356991350, 0.7998128361456341429 ) ) ;
#28290=CARTESIAN_POINT ( 'NONE',  ( 8.039058738260216330, 8.343599714250547805, -0.7998128361456341429 ) ) ;
#28294=CARTESIAN_POINT ( 'NONE',  ( -5.328968068096138211, 7.722205811214136517, -1.323081262718794893 ) ) ;
#28312=CARTESIAN_POINT ( 'NONE',  ( 5.397554552016226914, 6.430140077841320689, 1.082531754730549078 ) ) ;
#28326=CARTESIAN_POINT ( 'NONE',  ( -3.851925040058345573, 5.587274861525073355, -1.443375672974078761 ) ) ;
#28330=CARTESIAN_POINT ( 'NONE',  ( 4.064412189046650248, 7.963840997188264659, 0.7998128361456271485 ) ) ;
#28342=AXIS2_PLACEMENT_3D ( 'NONE', #155968, #139738, #43298 ) ;
#28350=EDGE_CURVE ( 'NONE', #2366, #111968, #84984, .T. ) ;
#28362=ADVANCED_FACE ( 'NONE', ( #200837 ), #102301, .F. ) ;
#28382=CARTESIAN_POINT ( 'NONE',  ( -5.628043163004235794, 5.738674243025936761, 0.7216878364870257245 ) ) ;
#28389=CARTESIAN_POINT ( 'NONE',  ( -4.098307573080856692, 8.003385611894792362, 0.7998128361456352531 ) ) ;
#28399=CARTESIAN_POINT ( 'NONE',  ( -4.034433228518296666, 6.864533312316751790, -1.199719254218450271 ) ) ;
#28402=CARTESIAN_POINT ( 'NONE',  ( 6.564609147483420060, 6.793222102749934876, 0.3624652974001541517 ) ) ;
#28407=CARTESIAN_POINT ( 'NONE',  ( 4.369470645354133431, 8.319742529546998000, 0.7998128361456271485 ) ) ;
#28414=CARTESIAN_POINT ( 'NONE',  ( -7.937372586157736443, 8.224965870130965584, 0.7998128361456341429 ) ) ;
#28420=CARTESIAN_POINT ( 'NONE',  ( -5.367048706163331850, 7.354919138647580290, -1.599625672291271394 ) ) ;
#28424=CARTESIAN_POINT ( 'NONE',  ( 5.899206235277530297, 7.015400374979486209, -1.082531754730548412 ) ) ;
#28425=CARTESIAN_POINT ( 'NONE',  ( -6.916067756302494374, 7.241369601873926420, 0.000000000000000000 ) ) ;
#28429=CARTESIAN_POINT ( 'NONE',  ( -4.936050443827081580, 7.916420063510339666, 1.199719254218452935 ) ) ;
#28432=CARTESIAN_POINT ( 'NONE',  ( 4.854701522145073334, 7.821512988214679218, -1.199719254218450271 ) ) ;
#28433=EDGE_LOOP ( 'NONE', ( #87024, #72556, #110733, #61974 ) ) ;
#28435=DIRECTION ( 'NONE',  ( 0.000000000000000000, 1.000000000000000000, 0.000000000000000000 ) ) ;
#28460=CARTESIAN_POINT ( 'NONE',  ( 4.635702676548680401, 8.322458603728597026, -0.3981331281527732968 ) ) ;
#28468=CARTESIAN_POINT ( 'NONE',  ( 6.424584688029230328, 8.588711117491191871, 1.599625672291268286 ) ) ;
#28469=EDGE_LOOP ( 'NONE', ( #198400, #85054, #56342, #204712, #100510, #163393, #120446 ) ) ;
#28473=CARTESIAN_POINT ( 'NONE',  ( -4.616709804987970678, 8.367809121204862421, 0.2297300046584915267 ) ) ;
#28480=CARTESIAN_POINT ( 'NONE',  ( -3.485854892044998543, 6.120562236477518070, -1.082531754730546636 ) ) ;
#28491=CARTESIAN_POINT ( 'NONE',  ( -4.516801452008150086, 5.298631777878131111, 1.199719254218452935 ) ) ;
#28493=CARTESIAN_POINT ( 'NONE',  ( 6.363572996767764778, 8.517530811019446091, -1.599625672291283607 ) ) ;
#28503=CARTESIAN_POINT ( 'NONE',  ( 5.071631979963703962, 8.074598522336444262, 1.199719254218451159 ) ) ;
#28506=CARTESIAN_POINT ( 'NONE',  ( 4.706088717274896638, 7.544168365912456764, 1.082531754730548412 ) ) ;
#28515=CARTESIAN_POINT ( 'NONE',  ( -6.394499343358424959, 6.826875778244118287, 0.5478302896938479494 ) ) ;
#28523=CARTESIAN_POINT ( 'NONE',  ( -3.447516199624892419, 7.244129009529488350, 0.7998128361456352531 ) ) ;
#28524=CARTESIAN_POINT ( 'NONE',  ( 3.984117037569365305, 5.741498858621315371, 1.599625672291261402 ) ) ;
#28528=( BOUNDED_CURVE ( )  B_SPLINE_CURVE ( 2, ( #210288, #97642, #61928, #81368, #147448 ),
 .UNSPECIFIED., .F., .T. ) 
 B_SPLINE_CURVE_WITH_KNOTS ( ( 3, 2, 3 ),
 ( 0.2458537933072449944, 0.2500000000000000000, 0.2548141018745767039 ),
 .UNSPECIFIED. ) 
 CURVE ( )  GEOMETRIC_REPRESENTATION_ITEM ( )  RATIONAL_B_SPLINE_CURVE ( ( 0.9330143170877186476, 0.9333416359014268249, 1.000000000000000000, 0.9226039174255613595, 0.9346300651406820315 ) ) 
 REPRESENTATION_ITEM ( '' )  );
#28530=ORIENTED_EDGE ( 'NONE', *, *, #115651, .F. ) ;
#28535=CARTESIAN_POINT ( 'NONE',  ( -5.424143973919053785, 8.485862515284315677, 1.199719254218454489 ) ) ;
#28536=CARTESIAN_POINT ( 'NONE',  ( -4.261005416444848315, 8.193199762486115034, 0.7998128361456352531 ) ) ;
#28538=CARTESIAN_POINT ( 'NONE',  ( 7.309254211098760834, 8.660456346770972758, 1.082531754730549967 ) ) ;
#28544=CARTESIAN_POINT ( 'NONE',  ( 4.577813143269636065, 5.369812084349879555, -1.199719254218450271 ) ) ;
#28545=AXIS2_PLACEMENT_3D ( 'NONE', #119688, #132710, #116483 ) ;
#28551=CARTESIAN_POINT ( 'NONE',  ( -6.405493493895330737, 6.819705373682535487, -0.5214928506756879578 ) ) ;
#28560=CARTESIAN_POINT ( 'NONE',  ( -7.957709816578236506, 8.248692638954882028, 0.7998128361456341429 ) ) ;
#28578=CARTESIAN_POINT ( 'NONE',  ( 6.852720297064418986, 6.959538199522133262, 0.7998128361456331437 ) ) ;
#28612=CARTESIAN_POINT ( 'NONE',  ( 5.252858170651868441, 5.093032385374103299, -0.7998128361456481317 ) ) ;
#28643=CARTESIAN_POINT ( 'NONE',  ( -4.132202957115018727, 8.042930226601317401, 0.000000000000000000 ) ) ;
#28645=CARTESIAN_POINT ( 'NONE',  ( 6.712695452097489301, 7.964471127936110229, -1.082531754730548412 ) ) ;
#28650=CARTESIAN_POINT ( 'NONE',  ( -4.468294144155606773, 7.370704380560280100, 1.199719254218452935 ) ) ;
#28656=CARTESIAN_POINT ( 'NONE',  ( -4.767627293860968507, 5.591261926706423857, -1.199719254218453823 ) ) ;
#28664=CARTESIAN_POINT ( 'NONE',  ( -4.773352600463090845, 7.726605912919016106, 1.199719254218452935 ) ) ;
#28673=CARTESIAN_POINT ( 'NONE',  ( -5.632486471834530661, 5.535932070087196344, -0.7998128361456362523 ) ) ;
#28676=CARTESIAN_POINT ( 'NONE',  ( -5.560252395380252288, 7.580323442733986283, 1.443375672974058777 ) ) ;
#28677=CARTESIAN_POINT ( 'NONE',  ( -4.272227801637618505, 7.998366511970260717, 0.7216878364870338292 ) ) ;
#28678=CARTESIAN_POINT ( 'NONE',  ( 6.282224075085741433, 8.422623735723785643, 1.599625672291268286 ) ) ;
#28679=CARTESIAN_POINT ( 'NONE',  ( -6.200875153403786477, 8.327716660428123419, -1.599625672291271394 ) ) ;
#28716=CARTESIAN_POINT ( 'NONE',  ( 4.636584873806110174, 8.438537862545894441, 0.4145994950837776916 ) ) ;
#28731=CARTESIAN_POINT ( 'NONE',  ( 6.875920180786008196, 8.050936961452347163, -1.199719254218452047 ) ) ;
#28734=CARTESIAN_POINT ( 'NONE',  ( -5.764151584465413869, 6.753873599078290546, -1.199719254218453823 ) ) ;
#28738=CARTESIAN_POINT ( 'NONE',  ( -5.912764388891193157, 9.912325863766124456, 0.000000000000000000 ) ) ;
#28750=CARTESIAN_POINT ( 'NONE',  ( 7.180978637093494044, 8.406838493811077839, -1.199719254218452047 ) ) ;
#28751=CARTESIAN_POINT ( 'NONE',  ( 5.773793314573267388, 7.829454515125894964, 1.599625672291268286 ) ) ;
#28758=ORIENTED_EDGE ( 'NONE', *, *, #71694, .F. ) ;
#28765=CARTESIAN_POINT ( 'NONE',  ( 6.550524494058025837, 7.671308660269694712, -1.199719254218452047 ) ) ;
#28779=CARTESIAN_POINT ( 'NONE',  ( -4.475600106286965918, 8.235634200727838916, 0.7216878364870338292 ) ) ;
#28780=CARTESIAN_POINT ( 'NONE',  ( -5.264308783856126439, 9.363720357799287797, -0.7998128361456362523 ) ) ;
#28793=CARTESIAN_POINT ( 'NONE',  ( 5.905458427204159477, 9.047396044116986502, 1.199719254218452047 ) ) ;
#28796=CARTESIAN_POINT ( 'NONE',  ( 8.025500584646550806, 8.327781868367935658, 0.000000000000000000 ) ) ;
#28812=CARTESIAN_POINT ( 'NONE',  ( 6.076298462418691315, 7.128931413452940014, -1.143247356662546732 ) ) ;
#28814=CARTESIAN_POINT ( 'NONE',  ( 5.631432701629774051, 7.663367133358481631, 1.599625672291269396 ) ) ;
#28816=CARTESIAN_POINT ( 'NONE',  ( -4.329849954717889915, 6.144853928627882489, 1.599625672291270506 ) ) ;
#28819=CARTESIAN_POINT ( 'NONE',  ( 5.143339171537801846, 7.093924681584509173, 1.599625672291269396 ) ) ;
#28827=CARTESIAN_POINT ( 'NONE',  ( 6.455090533882185788, 8.624301270986276080, -1.443375672974078761 ) ) ;
#28830=CARTESIAN_POINT ( 'NONE',  ( -4.959250327548641479, 9.007818825440551791, -0.7998128361456362523 ) ) ;
#28831=CARTESIAN_POINT ( 'NONE',  ( 5.662465432362883355, 6.635239754958710989, 1.199719254218451159 ) ) ;
#28841=CARTESIAN_POINT ( 'NONE',  ( -5.957882158562513908, 5.915560371269843465, -0.7998128361456362523 ) ) ;
#28852=ADVANCED_FACE ( 'NONE', ( #93550 ), #146312, .F. ) ;
#28870=CARTESIAN_POINT ( 'NONE',  ( 5.424670859243587273, 5.501406555305196733, -0.7216878364870458196 ) ) ;
#28871=ORIENTED_EDGE ( 'NONE', *, *, #97685, .T. ) ;
#28876=CARTESIAN_POINT ( 'NONE',  ( 4.543390873910906791, 6.393985001019784953, 1.443375672974065660 ) ) ;
#28879=EDGE_CURVE ( 'NONE', #56474, #79244, #1137, .T. ) ;
#28891=CARTESIAN_POINT ( 'NONE',  ( -5.387385936583832802, 7.378645907471495846, -1.599625672291271394 ) ) ;
#28893=CARTESIAN_POINT ( 'NONE',  ( -5.413448473606448985, 9.537716662508005427, 0.000000000000000000 ) ) ;
#28895=CARTESIAN_POINT ( 'NONE',  ( 7.634649897826744080, 9.040084647953621655, 1.082531754730549078 ) ) ;
#28905=CARTESIAN_POINT ( 'NONE',  ( -5.906512197408906317, 6.919960980845699439, -1.199719254218453823 ) ) ;
#28911=CARTESIAN_POINT ( 'NONE',  ( -3.662110889467009578, 7.286563447771212232, 0.7216878364870338292 ) ) ;
#28915=CARTESIAN_POINT ( 'NONE',  ( -6.283277845290492714, 6.295188672452495915, -0.7998128361456362523 ) ) ;
#28928=( BOUNDED_CURVE ( )  B_SPLINE_CURVE ( 2, ( #128943, #96387, #14014, #192771, #146204 ),
 .UNSPECIFIED., .F., .T. ) 
 B_SPLINE_CURVE_WITH_KNOTS ( ( 3, 2, 3 ),
 ( 0.04818853575335232259, 0.05000000000000000278, 0.05151109858792213281 ),
 .UNSPECIFIED. ) 
 CURVE ( )  GEOMETRIC_REPRESENTATION_ITEM ( )  RATIONAL_B_SPLINE_CURVE ( ( 0.9544155427547809101, 0.9708771770795741052, 1.000000000000000000, 0.9757061412209473428, 0.9602227822089841602 ) ) 
 REPRESENTATION_ITEM ( '' )  );
#28935=CARTESIAN_POINT ( 'NONE',  ( -7.293360289508603600, 7.473618190706972086, 0.000000000000000000 ) ) ;
#28936=DIRECTION ( 'NONE',  ( 0.6507913734559658270, -0.7592566023652989049, 0.000000000000000000 ) ) ;
#28937=CARTESIAN_POINT ( 'NONE',  ( -4.034433228518296666, 6.864533312316751790, -1.199719254218450271 ) ) ;
#28962=CARTESIAN_POINT ( 'NONE',  ( -5.596483547390937119, 9.751257581923240991, 0.000000000000000000 ) ) ;
#28988=CARTESIAN_POINT ( 'NONE',  ( 6.339319342841494453, 9.553567112360518365, -1.199719254218452047 ) ) ;
#28990=CARTESIAN_POINT ( 'NONE',  ( 6.964048179274811012, 8.153752959689313684, 1.199719254218452047 ) ) ;
#28991=FACE_OUTER_BOUND ( 'NONE', #206045, .T. ) ;
#28998=CARTESIAN_POINT ( 'NONE',  ( 6.460097816570166351, 6.783347224138203124, 0.3989550415292943408 ) ) ;
#29003=CARTESIAN_POINT ( 'NONE',  ( 6.244837129360077732, 6.910362811036335096, 0.8058565020967979331 ) ) ;
#29005=CARTESIAN_POINT ( 'NONE',  ( 7.024532985656136930, 8.328281583754568729, 1.082531754730549967 ) ) ;
#29011=CARTESIAN_POINT ( 'NONE',  ( -3.786470039966538970, 7.639575156594750283, 0.000000000000000000 ) ) ;
#29014=ORIENTED_EDGE ( 'NONE', *, *, #85316, .F. ) ;
#29020=CARTESIAN_POINT ( 'NONE',  ( -6.305950843687521790, 7.489935751457798219, 1.082531754730548412 ) ) ;
#29031=FACE_OUTER_BOUND ( 'NONE', #175719, .T. ) ;
#29039=CARTESIAN_POINT ( 'NONE',  ( -6.628729601230480384, 6.698215721049152194, 0.3833203584966006217 ) ) ;
#29041=CARTESIAN_POINT ( 'NONE',  ( 6.535912570239620578, 9.782925877658371405, 1.199719254218452047 ) ) ;
#29055=CARTESIAN_POINT ( 'NONE',  ( -5.599738924909661186, 5.745725798494749625, 0.2540040342395213369 ) ) ;
#29058=CARTESIAN_POINT ( 'NONE',  ( -8.100070429521727178, 8.414780020722290033, 0.7998128361456341429 ) ) ;
#29061=CARTESIAN_POINT ( 'NONE',  ( 5.505492895601038938, 8.580769590579979678, -1.199719254218452047 ) ) ;
#29062=CARTESIAN_POINT ( 'NONE',  ( -6.378792857440260811, 6.837131066116997502, 0.5844455422965456615 ) ) ;
#29069=CARTESIAN_POINT ( 'NONE',  ( 3.854260808034858155, 7.718664386007802136, -0.7998128361456362523 ) ) ;
#29077=CARTESIAN_POINT ( 'NONE',  ( 3.390947817193682656, 6.009837315817661008, -1.082531754730549967 ) ) ;
#29082=CARTESIAN_POINT ( 'NONE',  ( 6.400857919427532572, 6.640291458853147866, -0.7216878364870458196 ) ) ;
#29093=CARTESIAN_POINT ( 'NONE',  ( -5.966997003790240228, 6.134120390609613338, -0.7216878364870338292 ) ) ;
#29114=CARTESIAN_POINT ( 'NONE',  ( 5.573810548549551491, 6.635772073796838200, -1.082531754730548412 ) ) ;
#29123=CARTESIAN_POINT ( 'NONE',  ( 5.662465432362883355, 6.635239754958710989, 1.199719254218451159 ) ) ;
#29135=CARTESIAN_POINT ( 'NONE',  ( -5.496904935697871863, 5.377753611261092637, 0.7998128361456281477 ) ) ;
#29139=CARTESIAN_POINT ( 'NONE',  ( 3.567203813726949058, 7.175838526074521440, 0.7216878364870257245 ) ) ;
#29154=CARTESIAN_POINT ( 'NONE',  ( -4.665414256878287702, 8.457084043084382330, -0.7216878364870338292 ) ) ;
#29155=ORIENTED_EDGE ( 'NONE', *, *, #193063, .T. ) ;
#29156=CARTESIAN_POINT ( 'NONE',  ( -4.746763178560296836, 6.631252689777363152, 1.443375672974058777 ) ) ;
#29165=ADVANCED_FACE ( 'NONE', ( #55700 ), #83396, .F. ) ;
#29195=CARTESIAN_POINT ( 'NONE',  ( -5.562588163356775972, 9.711712967216715953, 0.7998128361456291469 ) ) ;
#29196=CARTESIAN_POINT ( 'NONE',  ( -4.622835856459495574, 8.451390222604121760, 0.3997878540293615113 ) ) ;
#29198=CARTESIAN_POINT ( 'NONE',  ( -5.388983382465591276, 7.615141676677004590, 1.304926139240682348 ) ) ;
#29201=CARTESIAN_POINT ( 'NONE',  ( -7.607533590599451223, 9.008448956188397361, 1.082531754730549078 ) ) ;
#29204=CARTESIAN_POINT ( 'NONE',  ( -4.842197138736131556, 5.678260079060780008, 1.199719254218452935 ) ) ;
#29207=CARTESIAN_POINT ( 'NONE',  ( -4.468294144155606773, 7.370704380560280100, 1.199719254218452935 ) ) ;
#29216=ORIENTED_EDGE ( 'NONE', *, *, #101627, .F. ) ;
#29220=CARTESIAN_POINT ( 'NONE',  ( 5.224688093219824303, 7.188831756880171397, -1.599625672291283607 ) ) ;
#29244=CARTESIAN_POINT ( 'NONE',  ( 4.355912491740495440, 8.303924683664389406, 0.000000000000000000 ) ) ;
#29245=CARTESIAN_POINT ( 'NONE',  ( 5.032011289327418702, 5.899709921417326974, 1.199719254218452935 ) ) ;
#29247=CARTESIAN_POINT ( 'NONE',  ( 3.366167277942881064, 7.149221934233827014, -0.7998128361456362523 ) ) ;
#29259=CARTESIAN_POINT ( 'NONE',  ( 4.595450297557979624, 8.489593704440707711, 0.02661077391274621617 ) ) ;
#29260=CARTESIAN_POINT ( 'NONE',  ( -4.272227801637618505, 7.998366511970260717, 0.7216878364870338292 ) ) ;
#29261=CARTESIAN_POINT ( 'NONE',  ( 4.095971805104288599, 5.871996087412059140, 1.443375672974058777 ) ) ;
#29286=CARTESIAN_POINT ( 'NONE',  ( 4.878955176071345434, 6.785476686873604280, -1.599625672291269396 ) ) ;
#29305=CARTESIAN_POINT ( 'NONE',  ( -5.932574734431526942, 9.079031735882207244, 1.199719254218454489 ) ) ;
#29314=VERTEX_POINT ( 'NONE', #153743 ) ;
#29316=CARTESIAN_POINT ( 'NONE',  ( 5.180097208873055692, 8.201141289397330780, -1.199719254218450271 ) ) ;
#29321=VERTEX_POINT ( 'NONE', #20521 ) ;
#29322=CARTESIAN_POINT ( 'NONE',  ( 5.306037014901791693, 7.283738832175834510, 1.599625672291269396 ) ) ;
#29334=CARTESIAN_POINT ( 'NONE',  ( 4.649081266440608928, 8.305916344280937835, -0.4560373724170601606 ) ) ;
#29343=CARTESIAN_POINT ( 'NONE',  ( 5.346851039111009563, 6.199209027673978412, 1.092492203018504471 ) ) ;
#29356=CARTESIAN_POINT ( 'NONE',  ( -6.791708605802965870, 6.888357893050385705, -0.7998128361456362523 ) ) ;
#29358=CARTESIAN_POINT ( 'NONE',  ( 4.875038752565570732, 7.845239757038595663, -1.199719254218452047 ) ) ;
#29362=CARTESIAN_POINT ( 'NONE',  ( -5.589704470584107909, 9.743348658981940247, -0.7998128361456362523 ) ) ;
#29365=CARTESIAN_POINT ( 'NONE',  ( 5.677832469072920496, 9.846164657218904992, 0.000000000000000000 ) ) ;
#29370=CARTESIAN_POINT ( 'NONE',  ( -6.481153920547079395, 6.846182452143763086, -0.6414432093310319383 ) ) ;
#29371=CARTESIAN_POINT ( 'NONE',  ( -3.947104627881229622, 8.980740528189222971, 0.7749999999999996891 ) ) ;
#29382=ADVANCED_FACE ( 'NONE', ( #55175 ), #22644, .T. ) ;
#29389=CARTESIAN_POINT ( 'NONE',  ( 7.038091139269835317, 7.383730215335837954, 0.000000000000000000 ) ) ;
#29410=CARTESIAN_POINT ( 'NONE',  ( 6.249382461256315580, 6.255644057745969988, -0.7998128361456481317 ) ) ;
#29428=B_SPLINE_CURVE_WITH_KNOTS ( 'NONE', 3,
 ( #87366, #35394, #34330, #101471, #19141, #137197, #70009, #18065, #149153, #100405, #66798, #116711, #121018, #51673, #136125, #169673, #117794, #50588 ),
 .UNSPECIFIED., .F., .F.,
 ( 4, 2, 2, 2, 2, 2, 2, 2, 4 ),
 ( 0.8245435890462745609, 0.8388218094160719840, 0.8531000297858694070, 0.8673782501556668301, 0.8816564705254642531, 0.8959346908952616761, 0.9102129112650590992, 0.9244911316348565222, 0.9387693520046538342 ),
 .UNSPECIFIED. ) ;
#29451=CARTESIAN_POINT ( 'NONE',  ( 4.909461021924256485, 4.900328411765999981, 0.7216878364870338292 ) ) ;
#29456=FACE_OUTER_BOUND ( 'NONE', #193940, .T. ) ;
#29460=CARTESIAN_POINT ( 'NONE',  ( -6.102578539482539810, 6.292298848917299736, 0.000000000000000000 ) ) ;
#29465=CARTESIAN_POINT ( 'NONE',  ( -6.473091995881817162, 6.516638514809040217, 0.7998128361456281477 ) ) ;
#29475=CARTESIAN_POINT ( 'NONE',  ( -3.955946960137363799, 7.837298230127379917, 0.7998128361456352531 ) ) ;
#29477=CARTESIAN_POINT ( 'NONE',  ( 6.589288424369031283, 6.777081280454712697, 0.2339771526987007022 ) ) ;
#29482=CARTESIAN_POINT ( 'NONE',  ( 6.554440917563797875, 6.611545590104705994, -0.7998128361456481317 ) ) ;
#29488=CARTESIAN_POINT ( 'NONE',  ( -4.167152111353897403, 5.955039778036558040, 1.599625672291270506 ) ) ;
#29494=CARTESIAN_POINT ( 'NONE',  ( -4.098307573080856692, 8.003385611894792362, 0.7998128361456352531 ) ) ;
#29498=CARTESIAN_POINT ( 'NONE',  ( 6.387299765369506055, 7.584842826753462219, -1.082531754730548412 ) ) ;
#29500=CARTESIAN_POINT ( 'NONE',  ( -7.241463443030476732, 7.620997903056574430, 0.000000000000000000 ) ) ;
#29507=CARTESIAN_POINT ( 'NONE',  ( 5.890091390494168522, 5.836471141856793388, 0.000000000000000000 ) ) ;
#29513=CARTESIAN_POINT ( 'NONE',  ( 6.540882763950133238, 6.595727744222092959, 0.000000000000000000 ) ) ;
#29515=CARTESIAN_POINT ( 'NONE',  ( -6.141084208779844289, 5.378569653125054195, -2.500000000000000888 ) ) ;
#29536=CARTESIAN_POINT ( 'NONE',  ( 4.612778539632031105, 8.351152097327862123, 0.2683542610703564812 ) ) ;
#29544=CARTESIAN_POINT ( 'NONE',  ( 6.261886844665240481, 8.398896966899865646, 1.599625672291268286 ) ) ;
#29549=CARTESIAN_POINT ( 'NONE',  ( -4.606260857482554982, 8.381206713624141713, 0.1075878075270080697 ) ) ;
#29557=CARTESIAN_POINT ( 'NONE',  ( -3.634994581795317536, 7.254927755487573293, 0.000000000000000000 ) ) ;
#29567=CARTESIAN_POINT ( 'NONE',  ( -4.085803189671902480, 5.860132702740892263, -1.599625672291271394 ) ) ;
#29578=CARTESIAN_POINT ( 'NONE',  ( 6.201928923608456046, 6.200281597156833691, 0.7998128361456352531 ) ) ;
#29582=CARTESIAN_POINT ( 'NONE',  ( 4.543390873910903238, 7.354354215321133204, 1.082531754730548412 ) ) ;
#29598=CARTESIAN_POINT ( 'NONE',  ( -3.298376509874564988, 7.070132704820777825, 0.000000000000000000 ) ) ;
#29599=CARTESIAN_POINT ( 'NONE',  ( 5.391302360089590628, 6.318882837306503575, -1.199719254218452047 ) ) ;
#29610=CARTESIAN_POINT ( 'NONE',  ( -5.912237504011027767, 9.055304967058290799, 1.199719254218454489 ) ) ;
#29611=CARTESIAN_POINT ( 'NONE',  ( 5.505492895601038938, 8.580769590579979678, -1.199719254218452047 ) ) ;
#29613=CARTESIAN_POINT ( 'NONE',  ( 6.658462837642791676, 8.861568958707010779, 1.443375672974063439 ) ) ;
#29618=CARTESIAN_POINT ( 'NONE',  ( 3.553118775233146120, 6.302999783484076524, -1.199719254218453823 ) ) ;
#29626=CARTESIAN_POINT ( 'NONE',  ( -5.495582220874787538, 7.482514367559947033, -1.250084184017367539 ) ) ;
#29634=CARTESIAN_POINT ( 'NONE',  ( -4.977251789548269301, 4.979417640660637190, 0.7216878364870257245 ) ) ;
#29652=CARTESIAN_POINT ( 'NONE',  ( 6.801350335910821165, 7.963938809097990124, 1.199719254218452047 ) ) ;
#29685=CARTESIAN_POINT ( 'NONE',  ( 3.715816618597135523, 6.492813934075403637, -1.199719254218453823 ) ) ;
#29690=CARTESIAN_POINT ( 'NONE',  ( 4.879147978569815969, 4.879180288469956217, -0.1512534140984626019 ) ) ;
#29717=CARTESIAN_POINT ( 'NONE',  ( -6.140917232347002042, 6.129101290685087911, -0.7998128361456362523 ) ) ;
#29719=CARTESIAN_POINT ( 'NONE',  ( 5.031484404002867450, 8.884165881396448583, 0.7216878364870317197 ) ) ;
#29724=CARTESIAN_POINT ( 'NONE',  ( -3.806807270387036368, 7.663301925418665839, 0.000000000000000000 ) ) ;
#29729=CARTESIAN_POINT ( 'NONE',  ( -4.930325137224961907, 5.781076077297750970, -1.199719254218453823 ) ) ;
#29734=CARTESIAN_POINT ( 'NONE',  ( -6.445975688654487001, 6.485002823043819475, -0.7998128361456362523 ) ) ;
#29745=CARTESIAN_POINT ( 'NONE',  ( -5.309953438407606363, 6.223975762010839574, 1.199719254218452935 ) ) ;
#29748=CARTESIAN_POINT ( 'NONE',  ( -5.966997003790228682, 8.054858819212300958, -1.443375672974066548 ) ) ;
#29749=CARTESIAN_POINT ( 'NONE',  ( -5.926322542504860458, 9.928143709648733051, -0.7216878364870338292 ) ) ;
#29750=CARTESIAN_POINT ( 'NONE',  ( 5.501576472095266901, 9.640532660744973725, -0.7998128361456481317 ) ) ;
#29751=CARTESIAN_POINT ( 'NONE',  ( -7.795011973214244883, 8.058878488363559356, 0.7998128361456341429 ) ) ;
#29771=VERTEX_POINT ( 'NONE', #79937 ) ;
#29790=CARTESIAN_POINT ( 'NONE',  ( 4.985841187518467166, 7.931359929992748192, -1.059499378661461710 ) ) ;
#29805=CARTESIAN_POINT ( 'NONE',  ( 4.877901405866606588, 8.912911750144889567, 0.7998128361456341429 ) ) ;
#29808=( BOUNDED_SURFACE ( )  B_SPLINE_SURFACE ( 1, 2, ( 
 ( #42898, #175026, #29834, #13562, #45028, #92714, #10355, #111141, #210694, #9301, #75374, #177142, #142540, #94843, #160894, #62323, #163035, #14616, #146803, #179286, #30911, #195527, #80713, #47166, #212820, #113280, #129545, #96985, #186124, #22550, #138472, #73445, #156860, #8446, #137405, #40979, #172034, #107090, #106012, #173112, #140633, #104910, #202358, #87578, #203424, #169879, #24693, #121228, #54008, #21469, #6297, #139549, #55079, #170951, #168818, #90796, #120147, #7368, #20422, #187198, #74533, #119069, #153649, #155784, #206646, #38826, #88656, #23627, #154716, #205576, #86504, #185050, #71293, #36675, #72372, #152569, #4156, #37758, #102763, #89735, #70227, #204494, #136338, #57213, #122305, #103831, #5218, #56144, #188263, #39903, #123373, #189340, #147156, #79996, #195891, #212111, #211047, #96280, #97342, #182827, #146100, #116825, #114703, #47529, #196947, #181747, #83186, #66913, #162330, #180698, #113642, #148217, #149269, #13915, #64810, #165516, #63748, #129907, #82124, #46450, #214219, #30190, #112571, #65848, #98390, #178582, #179647, #17108, #133054, #32322, #31267, #163399, #14973, #115757, #848, #194814, #164454, #99459, #199055, #81070, #130957, #16041, #131997, #50701, #213181, #48587, #128832, #198006, #49633, #95212, #33378, #161261, #12848, #78922, #145045, #62673, #203325, #72263, #138371, #52832, #170853, #87480, #22443, #21372, #88554, #56044, #20321, #117903, #2991, #118969, #85335, #154615, #36574, #183896, #151417, #136235, #54977, #184947, #86407, #84267, #6194, #35508, #137309, #150352, #102660, #204389, #34442, #69058, #71192, #122200, #168718, #152474, #153546, #4054, #121130, #1923, #100516, #201193, #166591, #70124, #67981, #134124, #101585, #18180, #5115, #200133, #202258, #51786, #187093, #37655, #167653, #19254, #135178, #53909, #120044, #38727, #186018, #103732, #169783, #104808, #7262, #209733, #126456, #61377, #157824, #125386, #43017, #141602, #40878, #205476, #57108, #23522, #156759, #9420, #155680, #106983, #192420, #76546, #188162, #207609, #89628 ),
 ( #173008, #110193, #44074, #24589, #91768, #59228, #142657, #11546, #77616, #206543, #176203, #26730, #27804, #175144, #93902, #39795, #174086, #123277, #8346, #58173, #90696, #159941, #190291, #189239, #74431, #75491, #208667, #124331, #25659, #73339, #143739, #140531, #60298, #139441, #41948, #105902, #171926, #108061, #10472, #191352, #109131, #92832, #158876, #97097, #15793, #28876, #127534, #79745, #165259, #31022, #94961, #12604, #128597, #584, #180454, #161009, #63507, #45147, #98159, #130712, #16852, #194563, #177262, #82935, #46208, #114454, #145862, #111259, #78676, #193506, #144803, #149008, #65596, #210809, #163149, #64569, #196703, #80825, #112324, #62434, #178339, #29948, #96033, #14733, #162084, #99210, #13674, #212933, #211868, #32071, #181502, #129661, #146915, #197750, #195645, #47281, #164206, #113393, #81878, #179402, #48343, #147963, #213976, #131745, #49389, #115507, #33130, #152212, #67716, #17913, #200923, #87205, #137035, #166323, #86141, #120855, #69856, #203061, #18988, #199874, #50447, #37384, #154345, #116565, #83998, #118701, #51517, #167397, #183634, #182559, #133867, #68796, #66650, #117642, #88280, #3782, #85070, #168454, #153269, #54705, #132796, #102387, #35241, #186829, #198799, #4844, #38459, #101316, #104536, #134916, #52571, #184687, #151155, #70924, #22165, #20052, #36308, #135965, #201982, #170582, #1660, #150088, #119771, #53638, #185751, #34182, #2724, #100255, #103459, #169521, #21101, #96580, #139170, #10218, #108864, #5923, #25401, #121926, #206282, #155408, #107799, #91502, #56842, #30496, #138106, #8080, #173824, #171650, #79232, #204117, #62975, #125132, #9156, #187894, #74168, #157563, #156491, #124070, #23248, #75232, #145349, #141342, #73070, #190035, #123015, #41688, #207356, #211350, #140261, #58977, #39522, #92579, #71995, #106714, #90422, #195120, #40609, #57906, #55769, #174890, #191090, #42759, #105622, #24316, #26469, #129144, #158621, #46758, #188967, #112869, #178884, #89360, #6991, #205201, #172740, #133345, #72, #213466, #50997, #65090, #97636 ) ),
 .UNSPECIFIED., .F., .F., .T. ) 
 B_SPLINE_SURFACE_WITH_KNOTS ( ( 2, 2 ),
 ( 3, 2, 2, 2, 2, 2, 2, 2, 2, 2, 2, 2, 2, 2, 2, 2, 2, 2, 2, 2, 2, 2, 2, 2, 2, 2, 2, 2, 2, 2, 2, 2, 2, 2, 2, 2, 2, 2, 2, 2, 2, 2, 2, 2, 2, 2, 2, 2, 2, 2, 2, 2, 2, 2, 2, 2, 2, 2, 2, 2, 2, 2, 2, 2, 2, 2, 2, 2, 2, 2, 2, 2, 2, 2, 2, 2, 2, 2, 2, 2, 2, 2, 2, 2, 2, 2, 2, 2, 2, 2, 2, 2, 2, 2, 2, 2, 2, 2, 2, 2, 2, 2, 2, 2, 2, 2, 2, 2, 2, 2, 2, 2, 2, 2, 2, 2, 2, 2, 2, 2, 3 ),
 ( 0.000000000000000000, 1.000000000000000000 ),
 ( 0.000000000000000000, 0.008333333333333333218, 0.01666666666666666644, 0.02500000000000000139, 0.03333333333333333287, 0.04166666666666666435, 0.05000000000000000278, 0.05833333333333333426, 0.06666666666666666574, 0.07499999999999999722, 0.08333333333333332871, 0.09166666666666666019, 0.1000000000000000056, 0.1083333333333333370, 0.1166666666666666685, 0.1250000000000000000, 0.1333333333333333315, 0.1416666666666666630, 0.1499999999999999944, 0.1583333333333333259, 0.1666666666666666574, 0.1749999999999999889, 0.1833333333333333204, 0.1916666666666666796, 0.2000000000000000111, 0.2083333333333333426, 0.2166666666666666741, 0.2250000000000000056, 0.2333333333333333370, 0.2416666666666666685, 0.2500000000000000000, 0.2583333333333333592, 0.2666666666666666630, 0.2750000000000000222, 0.2833333333333333259, 0.2916666666666666852, 0.2999999999999999889, 0.3083333333333333481, 0.3166666666666666519, 0.3250000000000000111, 0.3333333333333333148, 0.3416666666666666741, 0.3499999999999999778, 0.3583333333333333370, 0.3666666666666666408, 0.3750000000000000000, 0.3833333333333333592, 0.3916666666666666630, 0.4000000000000000222, 0.4083333333333333259, 0.4166666666666666852, 0.4249999999999999889, 0.4333333333333333481, 0.4416666666666666519, 0.4500000000000000111, 0.4583333333333333148, 0.4666666666666666741, 0.4749999999999999778, 0.4833333333333333370, 0.4916666666666666408, 0.5000000000000000000, 0.5083333333333333037, 0.5166666666666667185, 0.5250000000000000222, 0.5333333333333333259, 0.5416666666666666297, 0.5500000000000000444, 0.5583333333333333481, 0.5666666666666666519, 0.5749999999999999556, 0.5833333333333333703, 0.5916666666666666741, 0.5999999999999999778, 0.6083333333333332815, 0.6166666666666666963, 0.6250000000000000000, 0.6333333333333333037, 0.6416666666666667185, 0.6500000000000000222, 0.6583333333333333259, 0.6666666666666666297, 0.6750000000000000444, 0.6833333333333333481, 0.6916666666666666519, 0.6999999999999999556, 0.7083333333333333703, 0.7166666666666666741, 0.7249999999999999778, 0.7333333333333332815, 0.7416666666666666963, 0.7500000000000000000, 0.7583333333333333037, 0.7666666666666667185, 0.7750000000000000222, 0.7833333333333333259, 0.7916666666666666297, 0.8000000000000000444, 0.8083333333333333481, 0.8166666666666666519, 0.8249999999999999556, 0.8333333333333333703, 0.8416666666666666741, 0.8499999999999999778, 0.8583333333333332815, 0.8666666666666666963, 0.8750000000000000000, 0.8833333333333333037, 0.8916666666666667185, 0.9000000000000000222, 0.9083333333333333259, 0.9166666666666666297, 0.9250000000000000444, 0.9333333333333333481, 0.9416666666666666519, 0.9499999999999999556, 0.9583333333333333703, 0.9666666666666666741, 0.9749999999999999778, 0.9833333333333332815, 0.9916666666666666963, 1.000000000000000000 ),
 .UNSPECIFIED. ) 
 GEOMETRIC_REPRESENTATION_ITEM ( )  RATIONAL_B_SPLINE_SURFACE ( (
 ( 1.000000000000000000, 0.8660254037844387076, 1.000000000000000000, 0.8660254037844387076, 1.000000000000000000, 0.8660254037844387076, 1.000000000000000000, 0.8660254037844387076, 1.000000000000000000, 0.8660254037844387076, 1.000000000000000000, 0.8660254037844387076, 1.000000000000000000, 0.8660254037844387076, 1.000000000000000000, 0.8660254037844387076, 1.000000000000000000, 0.8660254037844387076, 1.000000000000000000, 0.8660254037844387076, 1.000000000000000000, 0.8660254037844387076, 1.000000000000000000, 0.8660254037844387076, 1.000000000000000000, 0.8660254037844387076, 1.000000000000000000, 0.8660254037844387076, 1.000000000000000000, 0.8660254037844387076, 1.000000000000000000, 0.8660254037844387076, 1.000000000000000000, 0.8660254037844387076, 1.000000000000000000, 0.8660254037844387076, 1.000000000000000000, 0.8660254037844387076, 1.000000000000000000, 0.8660254037844387076, 1.000000000000000000, 0.8660254037844387076, 1.000000000000000000, 0.8660254037844387076, 1.000000000000000000, 0.8660254037844387076, 1.000000000000000000, 0.8660254037844387076, 1.000000000000000000, 0.8660254037844387076, 1.000000000000000000, 0.8660254037844387076, 1.000000000000000000, 0.8660254037844387076, 1.000000000000000000, 0.8660254037844387076, 1.000000000000000000, 0.8660254037844387076, 1.000000000000000000, 0.8660254037844387076, 1.000000000000000000, 0.8660254037844387076, 1.000000000000000000, 0.8660254037844387076, 1.000000000000000000, 0.8660254037844387076, 1.000000000000000000, 0.8660254037844387076, 1.000000000000000000, 0.8660254037844387076, 1.000000000000000000, 0.8660254037844387076, 1.000000000000000000, 0.8660254037844387076, 1.000000000000000000, 0.8660254037844387076, 1.000000000000000000, 0.8660254037844387076, 1.000000000000000000, 0.8660254037844387076, 1.000000000000000000, 0.8660254037844387076, 1.000000000000000000, 0.8660254037844387076, 1.000000000000000000, 0.8660254037844387076, 1.000000000000000000, 0.8660254037844387076, 1.000000000000000000, 0.8660254037844387076, 1.000000000000000000, 0.8660254037844387076, 1.000000000000000000, 0.8660254037844387076, 1.000000000000000000, 0.8660254037844387076, 1.000000000000000000, 0.8660254037844387076, 1.000000000000000000, 0.8660254037844387076, 1.000000000000000000, 0.8660254037844387076, 1.000000000000000000, 0.8660254037844387076, 1.000000000000000000, 0.8660254037844387076, 1.000000000000000000, 0.8660254037844387076, 1.000000000000000000, 0.8660254037844387076, 1.000000000000000000, 0.8660254037844387076, 1.000000000000000000, 0.8660254037844387076, 1.000000000000000000, 0.8660254037844387076, 1.000000000000000000, 0.8660254037844387076, 1.000000000000000000, 0.8660254037844387076, 1.000000000000000000, 0.8660254037844387076, 1.000000000000000000, 0.8660254037844387076, 1.000000000000000000, 0.8660254037844387076, 1.000000000000000000, 0.8660254037844387076, 1.000000000000000000, 0.8660254037844387076, 1.000000000000000000, 0.8660254037844387076, 1.000000000000000000, 0.8660254037844387076, 1.000000000000000000, 0.8660254037844387076, 1.000000000000000000, 0.8660254037844387076, 1.000000000000000000, 0.8660254037844387076, 1.000000000000000000, 0.8660254037844387076, 1.000000000000000000, 0.8660254037844387076, 1.000000000000000000, 0.8660254037844387076, 1.000000000000000000, 0.8660254037844387076, 1.000000000000000000, 0.8660254037844387076, 1.000000000000000000, 0.8660254037844387076, 1.000000000000000000, 0.8660254037844387076, 1.000000000000000000, 0.8660254037844387076, 1.000000000000000000, 0.8660254037844387076, 1.000000000000000000, 0.8660254037844387076, 1.000000000000000000, 0.8660254037844387076, 1.000000000000000000, 0.8660254037844387076, 1.000000000000000000, 0.8660254037844387076, 1.000000000000000000, 0.8660254037844387076, 1.000000000000000000, 0.8660254037844387076, 1.000000000000000000, 0.8660254037844387076, 1.000000000000000000, 0.8660254037844387076, 1.000000000000000000, 0.8660254037844387076, 1.000000000000000000, 0.8660254037844387076, 1.000000000000000000, 0.8660254037844387076, 1.000000000000000000, 0.8660254037844387076, 1.000000000000000000, 0.8660254037844387076, 1.000000000000000000, 0.8660254037844387076, 1.000000000000000000, 0.8660254037844387076, 1.000000000000000000, 0.8660254037844387076, 1.000000000000000000, 0.8660254037844387076, 1.000000000000000000, 0.8660254037844387076, 1.000000000000000000, 0.8660254037844387076, 1.000000000000000000, 0.8660254037844387076, 1.000000000000000000, 0.8660254037844387076, 1.000000000000000000, 0.8660254037844387076, 1.000000000000000000, 0.8660254037844387076, 1.000000000000000000, 0.8660254037844387076, 1.000000000000000000, 0.8660254037844387076, 1.000000000000000000, 0.8660254037844387076, 1.000000000000000000, 0.8660254037844387076, 1.000000000000000000, 0.8660254037844387076, 1.000000000000000000, 0.8660254037844387076, 1.000000000000000000, 0.8660254037844387076, 1.000000000000000000, 0.8660254037844387076, 1.000000000000000000, 0.8660254037844387076, 1.000000000000000000, 0.8660254037844387076, 1.000000000000000000, 0.8660254037844387076, 1.000000000000000000, 0.8660254037844387076, 1.000000000000000000, 0.8660254037844387076, 1.000000000000000000, 0.8660254037844387076, 1.000000000000000000, 0.8660254037844387076, 1.000000000000000000, 0.8660254037844387076, 1.000000000000000000, 0.8660254037844387076, 1.000000000000000000, 0.8660254037844387076, 1.000000000000000000),
 ( 1.000000000000000000, 0.8660254037844387076, 1.000000000000000000, 0.8660254037844387076, 1.000000000000000000, 0.8660254037844387076, 1.000000000000000000, 0.8660254037844387076, 1.000000000000000000, 0.8660254037844387076, 1.000000000000000000, 0.8660254037844387076, 1.000000000000000000, 0.8660254037844387076, 1.000000000000000000, 0.8660254037844387076, 1.000000000000000000, 0.8660254037844387076, 1.000000000000000000, 0.8660254037844387076, 1.000000000000000000, 0.8660254037844387076, 1.000000000000000000, 0.8660254037844387076, 1.000000000000000000, 0.8660254037844387076, 1.000000000000000000, 0.8660254037844387076, 1.000000000000000000, 0.8660254037844387076, 1.000000000000000000, 0.8660254037844387076, 1.000000000000000000, 0.8660254037844387076, 1.000000000000000000, 0.8660254037844387076, 1.000000000000000000, 0.8660254037844387076, 1.000000000000000000, 0.8660254037844387076, 1.000000000000000000, 0.8660254037844387076, 1.000000000000000000, 0.8660254037844387076, 1.000000000000000000, 0.8660254037844387076, 1.000000000000000000, 0.8660254037844387076, 1.000000000000000000, 0.8660254037844387076, 1.000000000000000000, 0.8660254037844387076, 1.000000000000000000, 0.8660254037844387076, 1.000000000000000000, 0.8660254037844387076, 1.000000000000000000, 0.8660254037844387076, 1.000000000000000000, 0.8660254037844387076, 1.000000000000000000, 0.8660254037844387076, 1.000000000000000000, 0.8660254037844387076, 1.000000000000000000, 0.8660254037844387076, 1.000000000000000000, 0.8660254037844387076, 1.000000000000000000, 0.8660254037844387076, 1.000000000000000000, 0.8660254037844387076, 1.000000000000000000, 0.8660254037844387076, 1.000000000000000000, 0.8660254037844387076, 1.000000000000000000, 0.8660254037844387076, 1.000000000000000000, 0.8660254037844387076, 1.000000000000000000, 0.8660254037844387076, 1.000000000000000000, 0.8660254037844387076, 1.000000000000000000, 0.8660254037844387076, 1.000000000000000000, 0.8660254037844387076, 1.000000000000000000, 0.8660254037844387076, 1.000000000000000000, 0.8660254037844387076, 1.000000000000000000, 0.8660254037844387076, 1.000000000000000000, 0.8660254037844387076, 1.000000000000000000, 0.8660254037844387076, 1.000000000000000000, 0.8660254037844387076, 1.000000000000000000, 0.8660254037844387076, 1.000000000000000000, 0.8660254037844387076, 1.000000000000000000, 0.8660254037844387076, 1.000000000000000000, 0.8660254037844387076, 1.000000000000000000, 0.8660254037844387076, 1.000000000000000000, 0.8660254037844387076, 1.000000000000000000, 0.8660254037844387076, 1.000000000000000000, 0.8660254037844387076, 1.000000000000000000, 0.8660254037844387076, 1.000000000000000000, 0.8660254037844387076, 1.000000000000000000, 0.8660254037844387076, 1.000000000000000000, 0.8660254037844387076, 1.000000000000000000, 0.8660254037844387076, 1.000000000000000000, 0.8660254037844387076, 1.000000000000000000, 0.8660254037844387076, 1.000000000000000000, 0.8660254037844387076, 1.000000000000000000, 0.8660254037844387076, 1.000000000000000000, 0.8660254037844387076, 1.000000000000000000, 0.8660254037844387076, 1.000000000000000000, 0.8660254037844387076, 1.000000000000000000, 0.8660254037844387076, 1.000000000000000000, 0.8660254037844387076, 1.000000000000000000, 0.8660254037844387076, 1.000000000000000000, 0.8660254037844387076, 1.000000000000000000, 0.8660254037844387076, 1.000000000000000000, 0.8660254037844387076, 1.000000000000000000, 0.8660254037844387076, 1.000000000000000000, 0.8660254037844387076, 1.000000000000000000, 0.8660254037844387076, 1.000000000000000000, 0.8660254037844387076, 1.000000000000000000, 0.8660254037844387076, 1.000000000000000000, 0.8660254037844387076, 1.000000000000000000, 0.8660254037844387076, 1.000000000000000000, 0.8660254037844387076, 1.000000000000000000, 0.8660254037844387076, 1.000000000000000000, 0.8660254037844387076, 1.000000000000000000, 0.8660254037844387076, 1.000000000000000000, 0.8660254037844387076, 1.000000000000000000, 0.8660254037844387076, 1.000000000000000000, 0.8660254037844387076, 1.000000000000000000, 0.8660254037844387076, 1.000000000000000000, 0.8660254037844387076, 1.000000000000000000, 0.8660254037844387076, 1.000000000000000000, 0.8660254037844387076, 1.000000000000000000, 0.8660254037844387076, 1.000000000000000000, 0.8660254037844387076, 1.000000000000000000, 0.8660254037844387076, 1.000000000000000000, 0.8660254037844387076, 1.000000000000000000, 0.8660254037844387076, 1.000000000000000000, 0.8660254037844387076, 1.000000000000000000, 0.8660254037844387076, 1.000000000000000000, 0.8660254037844387076, 1.000000000000000000, 0.8660254037844387076, 1.000000000000000000, 0.8660254037844387076, 1.000000000000000000, 0.8660254037844387076, 1.000000000000000000, 0.8660254037844387076, 1.000000000000000000, 0.8660254037844387076, 1.000000000000000000, 0.8660254037844387076, 1.000000000000000000, 0.8660254037844387076, 1.000000000000000000, 0.8660254037844387076, 1.000000000000000000, 0.8660254037844387076, 1.000000000000000000, 0.8660254037844387076, 1.000000000000000000, 0.8660254037844387076, 1.000000000000000000, 0.8660254037844387076, 1.000000000000000000, 0.8660254037844387076, 1.000000000000000000, 0.8660254037844387076, 1.000000000000000000, 0.8660254037844387076, 1.000000000000000000, 0.8660254037844387076, 1.000000000000000000, 0.8660254037844387076, 1.000000000000000000, 0.8660254037844387076, 1.000000000000000000) ) ) 
 REPRESENTATION_ITEM ( '' )  SURFACE ( )  );
#29809=CARTESIAN_POINT ( 'NONE',  ( -4.118644803501354978, 8.027112380718707030, 0.7998128361456352531 ) ) ;
#29813=CARTESIAN_POINT ( 'NONE',  ( -7.282137903871469753, 8.628820655005750240, 1.082531754730549078 ) ) ;
#29825=CARTESIAN_POINT ( 'NONE',  ( 5.422335090822693715, 5.290755458906732933, 0.000000000000000000 ) ) ;
#29826=CARTESIAN_POINT ( 'NONE',  ( 5.006703865196457492, 9.063181286029688977, 0.000000000000000000 ) ) ;
#29833=EDGE_LOOP ( 'NONE', ( #127743, #137722, #96028, #197817 ) ) ;
#29834=CARTESIAN_POINT ( 'NONE',  ( 4.435452530326143616, 5.203724702582467998, -1.199719254218452047 ) ) ;
#29840=CARTESIAN_POINT ( 'NONE',  ( 7.062871678076271920, 7.204714810702593120, -0.7998128361456341429 ) ) ;
#29841=ORIENTED_EDGE ( 'NONE', *, *, #47045, .F. ) ;
#29855=CARTESIAN_POINT ( 'NONE',  ( -4.340018570150309785, 7.117086527600392287, -1.082531754730551743 ) ) ;
#29856=CARTESIAN_POINT ( 'NONE',  ( 4.828112100242277549, 6.726159765073026264, -1.443375672974068769 ) ) ;
#29864=ORIENTED_EDGE ( 'NONE', *, *, #58107, .F. ) ;
#29866=CARTESIAN_POINT ( 'NONE',  ( -5.316205630334251531, 9.216340645449683677, -0.7216878364870338292 ) ) ;
#29867=CARTESIAN_POINT ( 'NONE',  ( 1.886825320689258012, 2.480000000000016858, -2.459652456995881753 ) ) ;
#29870=CARTESIAN_POINT ( 'NONE',  ( 6.556249800660121529, 9.806652646482286073, 1.199719254218452047 ) ) ;
#29883=CARTESIAN_POINT ( 'NONE',  ( -5.943394452344507251, 6.548109163587250592, 0.8056209499170760013 ) ) ;
#29886=CARTESIAN_POINT ( 'NONE',  ( 4.199993725183334803, 8.122019456014369254, -0.7998128361456362523 ) ) ;
#29888=CARTESIAN_POINT ( 'NONE',  ( -4.359828915246279024, 7.244161613499399799, -1.199719254218455378 ) ) ;
#29900=CARTESIAN_POINT ( 'NONE',  ( 6.292392690518195941, 8.434487120394948079, -1.443375672974078761 ) ) ;
#29902=CARTESIAN_POINT ( 'NONE',  ( -5.661411662158206681, 8.762674818229999829, -1.199719254218452047 ) ) ;
#29903=CARTESIAN_POINT ( 'NONE',  ( 5.692444392891300886, 7.734547439830227411, -1.599625672291281386 ) ) ;
#29910=AXIS2_PLACEMENT_3D ( 'NONE', #37276, #36196, #168347 ) ;
#29914=CARTESIAN_POINT ( 'NONE',  ( -3.800028193580205382, 7.655393002477360653, -0.7998128361456481317 ) ) ;
#29941=CARTESIAN_POINT ( 'NONE',  ( 3.743459811148990291, 7.381470523066878009, -0.7216878364870338292 ) ) ;
#29948=CARTESIAN_POINT ( 'NONE',  ( 5.031484404002879884, 6.963427452793765404, 1.443375672974065660 ) ) ;
#29959=CARTESIAN_POINT ( 'NONE',  ( -4.457598643843001973, 8.422558527783969851, 0.000000000000000000 ) ) ;
#29961=CARTESIAN_POINT ( 'NONE',  ( -7.774674742793745708, 8.035151719539642912, 0.7998128361456341429 ) ) ;
#29967=CARTESIAN_POINT ( 'NONE',  ( 8.025500584646550806, 8.327781868367935658, 0.000000000000000000 ) ) ;
#29973=CARTESIAN_POINT ( 'NONE',  ( -5.692444392891315097, 7.734547439830227411, -1.599625672291271394 ) ) ;
#29979=CARTESIAN_POINT ( 'NONE',  ( -5.478903473698268023, 5.564677938835638216, -0.7216878364870338292 ) ) ;
#29980=CIRCLE ( 'NONE', #185645, 0.08000000000000020983 ) ;
#29983=CARTESIAN_POINT ( 'NONE',  ( -4.447956913735107598, 7.346977611736363656, 1.199719254218452935 ) ) ;
#30005=CARTESIAN_POINT ( 'NONE',  ( -3.160459205317013076, 6.701303149596211206, -0.7216878364870458196 ) ) ;
#30007=CARTESIAN_POINT ( 'NONE',  ( -4.522526758610270647, 7.433975764090723359, -1.199719254218453823 ) ) ;
#30030=CARTESIAN_POINT ( 'NONE',  ( -7.605197822622922210, 7.837428646007010613, -0.7998128361456362523 ) ) ;
#30052=ADVANCED_FACE ( 'NONE', ( #164399 ), #15982, .F. ) ;
#30054=CARTESIAN_POINT ( 'NONE',  ( 7.876360894896227371, 8.153785563659219804, -0.7998128361456341429 ) ) ;
#30055=CARTESIAN_POINT ( 'NONE',  ( 4.934241560730721510, 4.721313007132757811, 0.000000000000000000 ) ) ;
#30069=CARTESIAN_POINT ( 'NONE',  ( 4.802738015080052492, 8.126035781178083894, 0.8349615142884360131 ) ) ;
#30071=CARTESIAN_POINT ( 'NONE',  ( 5.831415467653547680, 8.857049574687536619, -1.082531754730548412 ) ) ;
#30077=CARTESIAN_POINT ( 'NONE',  ( -3.800028193580205382, 7.655393002477360653, -0.7998128361456481317 ) ) ;
#30079=VERTEX_POINT ( 'NONE', #167598 ) ;
#30082=CARTESIAN_POINT ( 'NONE',  ( -5.763624699140874164, 8.777960344756069233, -1.082531754730549967 ) ) ;
#30101=CARTESIAN_POINT ( 'NONE',  ( 7.180978637093494044, 8.406838493811077839, -1.199719254218452047 ) ) ;
#30124=CARTESIAN_POINT ( 'NONE',  ( 6.801350335910821165, 7.963938809097990124, 1.199719254218452047 ) ) ;
#30126=CARTESIAN_POINT ( 'NONE',  ( -6.027110718723775129, 7.076430883291389584, 1.047497865993127553 ) ) ;
#30132=CARTESIAN_POINT ( 'NONE',  ( 4.193214648376505593, 8.114110533073061404, 0.000000000000000000 ) ) ;
#30133=DIRECTION ( 'NONE',  ( -1.000000000000000000, 0.000000000000000000, 0.000000000000000000 ) ) ;
#30138=CARTESIAN_POINT ( 'NONE',  ( 4.934241560730721510, 4.721313007132757811, 0.000000000000000000 ) ) ;
#30140=CARTESIAN_POINT ( 'NONE',  ( 3.716343503921665459, 6.389465617000312569, -1.082531754730549967 ) ) ;
#30143=CARTESIAN_POINT ( 'NONE',  ( 6.875393295905841917, 7.193916064744513506, 0.000000000000000000 ) ) ;
#30151=LINE ( 'NONE', #95174, #77765 ) ;
#30154=CARTESIAN_POINT ( 'NONE',  ( -5.234856708652269042, 7.200695141551334721, 1.443375672974058777 ) ) ;
#30176=CARTESIAN_POINT ( 'NONE',  ( 5.600441157405738224, 5.741305760636564059, 0.6425381723618078800 ) ) ;
#30178=( BOUNDED_SURFACE ( )  B_SPLINE_SURFACE ( 3, 2, ( 
 ( #117386, #51261, #148760 ),
 ( #186582, #16594, #3538 ),
 ( #183382, #34988, #167147 ),
 ( #166072, #84817, #198546 ),
 ( #116312, #184440, #150906 ),
 ( #103209, #153024, #100007 ),
 ( #200675, #70673, #52324 ),
 ( #86957, #118453, #136783 ),
 ( #36057, #102138, #168206 ),
 ( #4599, #202812, #19805 ) ),
 .UNSPECIFIED., .F., .F., .T. ) 
 B_SPLINE_SURFACE_WITH_KNOTS ( ( 4, 2, 2, 2, 4 ),
 ( 3, 3 ),
 ( 0.001504965851240676507, 0.001881207314050846718, 0.002257448776861016929, 0.002633690239671187573, 0.003009931702481357784 ),
 ( 0.000000000000000000, 1.000000000000000000 ),
 .UNSPECIFIED. ) 
 GEOMETRIC_REPRESENTATION_ITEM ( )  RATIONAL_B_SPLINE_SURFACE ( (
 ( 1.000000000000000000, 0.7796377409682132553, 1.000000000000000000),
 ( 1.000000000000000000, 0.7901490482358394241, 1.000000000000000000),
 ( 1.000000000000000000, 0.7828211856522472312, 1.000000000000000000),
 ( 1.000000000000000000, 0.7482553577056408889, 1.000000000000000000),
 ( 1.000000000000000000, 0.7228574685501613084, 1.000000000000000000),
 ( 1.000000000000000000, 0.7019526649397319629, 1.000000000000000000),
 ( 1.000000000000000000, 0.7095376569258128319, 1.000000000000000000),
 ( 1.000000000000000000, 0.7455209376246204611, 1.000000000000000000),
 ( 1.000000000000000000, 0.7705606446023164358, 1.000000000000000000),
 ( 1.000000000000000000, 0.7796368470575135712, 1.000000000000000000) ) ) 
 REPRESENTATION_ITEM ( '' )  SURFACE ( )  );
#30188=CARTESIAN_POINT ( 'NONE',  ( 5.611095471209277541, 7.639640364534566075, 1.599625672291268286 ) ) ;
#30190=CARTESIAN_POINT ( 'NONE',  ( 6.574778147984297938, 6.635272358928617997, -0.7998128361456481317 ) ) ;
#30203=CARTESIAN_POINT ( 'NONE',  ( -5.320648938720212051, 5.172121614787156929, 0.000000000000000000 ) ) ;
#30207=CARTESIAN_POINT ( 'NONE',  ( 4.977251789548238214, 7.860525283564661514, -1.082531754730548412 ) ) ;
#30216=( BOUNDED_SURFACE ( )  B_SPLINE_SURFACE ( 3, 2, ( 
 ( #165587, #99527, #4123 ),
 ( #133126, #202326, #182897 ),
 ( #198076, #135247, #69125 ),
 ( #17180, #50768, #149340 ),
 ( #65918, #33450, #166660 ),
 ( #117970, #85400, #19323 ),
 ( #101654, #185017, #199124 ),
 ( #87546, #132065, #102727 ) ),
 .UNSPECIFIED., .F., .F., .F. ) 
 B_SPLINE_SURFACE_WITH_KNOTS ( ( 4, 2, 2, 4 ),
 ( 3, 3 ),
 ( 0.000000000000000000, 0.003124175592871729877, 0.004686263389307594382, 0.006248351185743459754 ),
 ( 0.000000000000000000, 1.000000000000000000 ),
 .UNSPECIFIED. ) 
 GEOMETRIC_REPRESENTATION_ITEM ( )  RATIONAL_B_SPLINE_SURFACE ( (
 ( 1.000000000000000000, 0.7762074382822415908, 1.000000000000000000),
 ( 1.000000000000000000, 0.7833327836897199248, 1.000000000000000000),
 ( 1.000000000000000000, 0.7920843231447862731, 1.000000000000000000),
 ( 1.000000000000000000, 0.8126254522527567303, 1.000000000000000000),
 ( 1.000000000000000000, 0.8207499603065130378, 1.000000000000000000),
 ( 1.000000000000000000, 0.8408200424460848810, 1.000000000000000000),
 ( 1.000000000000000000, 0.8529123454023501694, 1.000000000000000000),
 ( 1.000000000000000000, 0.8665634049582059406, 1.000000000000000000) ) ) 
 REPRESENTATION_ITEM ( '' )  SURFACE ( )  );
#30223=CARTESIAN_POINT ( 'NONE',  ( -6.129694847154222970, 7.284303755502281597, -1.082531754730549967 ) ) ;
#30225=CARTESIAN_POINT ( 'NONE',  ( -5.980555157403903976, 6.149938236492225485, 0.000000000000000000 ) ) ;
#30238=EDGE_CURVE ( 'NONE', #22926, #71404, #200077, .T. ) ;
#30253=CARTESIAN_POINT ( 'NONE',  ( -4.787964524281469458, 5.614988695530339413, -1.199719254218453823 ) ) ;
#30262=CARTESIAN_POINT ( 'NONE',  ( -5.725286006720766707, 9.901527117808042178, 0.7998128361456291469 ) ) ;
#30263=CARTESIAN_POINT ( 'NONE',  ( -4.592595068035599581, 8.488991103336598343, 0.1827531742817755656 ) ) ;
#30265=CARTESIAN_POINT ( 'NONE',  ( -5.233772384569284064, 7.755300245267345183, 1.265081041508690607 ) ) ;
#30272=CARTESIAN_POINT ( 'NONE',  ( -3.644109427023046521, 7.473487774827342278, 0.000000000000000000 ) ) ;
#30275=CARTESIAN_POINT ( 'NONE',  ( -5.503684012504701961, 5.385662534202396934, 0.000000000000000000 ) ) ;
#30288=CARTESIAN_POINT ( 'NONE',  ( 4.224247379109608680, 7.085983154673295203, -1.199719254218452047 ) ) ;
#30313=CARTESIAN_POINT ( 'NONE',  ( 6.703580607314123085, 6.785541894813420072, 0.000000000000000000 ) ) ;
#30314=CARTESIAN_POINT ( 'NONE',  ( 3.725458348705031231, 7.568394850123006279, -1.734723475976807094E-15 ) ) ;
#30316=CARTESIAN_POINT ( 'NONE',  ( 4.913904330310220558, 4.697586238308844919, 0.000000000000000000 ) ) ;
#30324=B_SPLINE_CURVE_WITH_KNOTS ( 'NONE', 3,
 ( #47517, #194802, #30176, #96266, #214206, #146087, #212099, #64798, #130942, #196935 ),
 .UNSPECIFIED., .F., .F.,
 ( 4, 3, 3, 4 ),
 ( 4.424023162370599995E-18, 3.125149536070166581E-05, 5.486596421586658484E-05, 7.848575944736516173E-05 ),
 .UNSPECIFIED. ) ;
#30326=CARTESIAN_POINT ( 'NONE',  ( 0.4106005709051863128, 3.230891568747374265, 1.957863677979522654 ) ) ;
#30328=ORIENTED_EDGE ( 'NONE', *, *, #162643, .T. ) ;
#30330=CARTESIAN_POINT ( 'NONE',  ( 4.802592184731321545, 8.245026257381830703, 0.8702854636597904259 ) ) ;
#30331=CARTESIAN_POINT ( 'NONE',  ( -5.817857313595549584, 6.920493299683823096, 1.082531754730549078 ) ) ;
#30353=DIRECTION ( 'NONE',  ( -0.000000000000000000, -1.000000000000000000, -0.000000000000000000 ) ) ;
#30358=CARTESIAN_POINT ( 'NONE',  ( 4.960304097753311936, 6.880383762169266504, 1.599625672291268286 ) ) ;
#30360=CARTESIAN_POINT ( 'NONE',  ( 3.923105346307896202, 5.670318552149568703, -1.599625672291269396 ) ) ;
#30368=DIRECTION ( 'NONE',  ( 0.7592566023653005702, 0.6507913734559639396, 0.000000000000000000 ) ) ;
#30379=CARTESIAN_POINT ( 'NONE',  ( -6.071018923869249129, 10.30488218781460574, 0.7998128361456291469 ) ) ;
#30388=ORIENTED_EDGE ( 'NONE', *, *, #91128, .F. ) ;
#30390=CARTESIAN_POINT ( 'NONE',  ( 6.367489420273535039, 7.457767740854454708, -1.199719254218452047 ) ) ;
#30394=ORIENTED_EDGE ( 'NONE', *, *, #144483, .T. ) ;
#30397=CARTESIAN_POINT ( 'NONE',  ( 6.170896192875352959, 7.228408975556602556, 1.199719254218453823 ) ) ;
#30406=EDGE_CURVE ( 'NONE', #79641, #131991, #208613, .T. ) ;
#30409=CARTESIAN_POINT ( 'NONE',  ( 4.746850994788568201, 8.189453717816405742, 0.7312505120831546135 ) ) ;
#30421=CARTESIAN_POINT ( 'NONE',  ( -6.137446956630687289, 6.999240388318681561, 0.9466904651086446298 ) ) ;
#30428=CARTESIAN_POINT ( 'NONE',  ( -4.685224601974262271, 7.623789914682047808, -1.199719254218453823 ) ) ;
#30430=CARTESIAN_POINT ( 'NONE',  ( 6.547661840756936691, 6.603636667163397256, 0.7998128361456352531 ) ) ;
#30431=CARTESIAN_POINT ( 'NONE',  ( -3.599035817516879288, 3.565494897539134733, 2.500000000000000444 ) ) ;
#30434=CARTESIAN_POINT ( 'NONE',  ( -7.425025402139490360, 8.691559719698066289, 1.199719254218452047 ) ) ;
#30439=DIRECTION ( 'NONE',  ( -0.7592566023653004592, -0.6507913734559639396, 0.000000000000000000 ) ) ;
#30443=CARTESIAN_POINT ( 'NONE',  ( -6.238615401616060652, 7.011456692927672485, -1.010807710288418981 ) ) ;
#30459=CARTESIAN_POINT ( 'NONE',  ( 5.722950238744200391, 7.770137593325314285, 1.443375672974065660 ) ) ;
#30464=ORIENTED_EDGE ( 'NONE', *, *, #173168, .F. ) ;
#30465=CARTESIAN_POINT ( 'NONE',  ( -5.398914348987532641, 6.259949555863199677, -2.500000000000000444 ) ) ;
#30474=CARTESIAN_POINT ( 'NONE',  ( -4.001064729808656573, 7.682009594836471500, 1.214306433183764966E-14 ) ) ;
#30477=CARTESIAN_POINT ( 'NONE',  ( 5.032011289327418702, 5.899709921417326974, 1.199719254218452935 ) ) ;
#30496=CARTESIAN_POINT ( 'NONE',  ( 6.414416072596830887, 8.576847732820027659, -1.443375672974078761 ) ) ;
#30501=EDGE_CURVE ( 'NONE', #7055, #122390, #52955, .T. ) ;
#30504=DIRECTION ( 'NONE',  ( 0.000000000000000000, 0.000000000000000000, -1.000000000000000000 ) ) ;
#30521=CARTESIAN_POINT ( 'NONE',  ( 3.092668437693027794, 6.622213920701574885, -0.7216878364870338292 ) ) ;
#30532=CARTESIAN_POINT ( 'NONE',  ( -3.919715807682309094, 6.626733304721049933, 1.082531754730549967 ) ) ;
#30538=CARTESIAN_POINT ( 'NONE',  ( -4.274563570058511175, 8.209017608368725405, 0.000000000000000000 ) ) ;
#30548=CARTESIAN_POINT ( 'NONE',  ( -4.630991987519598396, 7.560518531151607213, 1.199719254218452935 ) ) ;
#30550=CARTESIAN_POINT ( 'NONE',  ( 6.177100234330334061, 7.056796855232915888, 1.058592334412721936 ) ) ;
#30555=CARTESIAN_POINT ( 'NONE',  ( 5.397027666691686321, 8.454226823519094935, 1.199719254218451159 ) ) ;
#30563=CARTESIAN_POINT ( 'NONE',  ( -4.736594563127865420, 6.619389305106191834, -1.599625672291271394 ) ) ;
#30568=CARTESIAN_POINT ( 'NONE',  ( -5.285699784481336927, 7.260012063351913625, 1.599625672291263179 ) ) ;
#30571=CARTESIAN_POINT ( 'NONE',  ( -3.765305043611756552, 7.354576300424669810, -0.6638232778202641793 ) ) ;
#30572=CARTESIAN_POINT ( 'NONE',  ( 6.875393295461478260, 8.154285278527437342, -1.082531754730548412 ) ) ;
#30574=CARTESIAN_POINT ( 'NONE',  ( -6.794044373779495771, 8.059378203231773341, 1.082531754730549078 ) ) ;
#30580=CARTESIAN_POINT ( 'NONE',  ( 5.123001941117305336, 7.070197912760590064, 1.599625672291268286 ) ) ;
#30587=DIRECTION ( 'NONE',  ( -0.7592566023652989049, 0.6507913734559658270, -1.175982368226367737E-15 ) ) ;
#30618=ORIENTED_EDGE ( 'NONE', *, *, #122876, .T. ) ;
#30622=CARTESIAN_POINT ( 'NONE',  ( -6.348239482750515528, 6.857177101084271698, -0.6483580952693357435 ) ) ;
#30625=EDGE_CURVE ( 'NONE', #158833, #40807, #138669, .T. ) ;
#30630=CARTESIAN_POINT ( 'NONE',  ( -4.462041952228954500, 6.299077925724123617, -1.443375672974066548 ) ) ;
#30642=CARTESIAN_POINT ( 'NONE',  ( -3.467853430045390706, 7.267855778353407459, 0.7998128361456352531 ) ) ;
#30644=CARTESIAN_POINT ( 'NONE',  ( 5.840530312436913007, 10.03597880781023299, 0.000000000000000000 ) ) ;
#30652=CARTESIAN_POINT ( 'NONE',  ( 6.066347387471824781, 6.042103138330730872, -0.7998128361456481317 ) ) ;
#30655=CARTESIAN_POINT ( 'NONE',  ( 6.495764994278809823, 6.751016379513001375, 0.7216878364870328300 ) ) ;
#30670=CARTESIAN_POINT ( 'NONE',  ( -4.285259070371116863, 7.157163461145040095, 1.199719254218452935 ) ) ;
#30671=CARTESIAN_POINT ( 'NONE',  ( 3.881377115262159894, 7.750300077773022878, 0.7998128361456271485 ) ) ;
#30677=ORIENTED_EDGE ( 'NONE', *, *, #33908, .F. ) ;
#30682=CARTESIAN_POINT ( 'NONE',  ( -6.074935347375019390, 9.245119117649618801, 1.199719254218452047 ) ) ;
#30683=CARTESIAN_POINT ( 'NONE',  ( 6.855582950365507244, 8.027210192628430718, -1.199719254218452047 ) ) ;
#30685=CARTESIAN_POINT ( 'NONE',  ( -7.015401035077384329, 6.062865449010540253, -2.437084766375293476 ) ) ;
#30699=CARTESIAN_POINT ( 'NONE',  ( -6.477282242306868554, 6.848760321534919093, 0.6499626829332164624 ) ) ;
#30707=CARTESIAN_POINT ( 'NONE',  ( -5.772739544368596043, 9.956889578397179363, -0.7998128361456362523 ) ) ;
#30709=AXIS2_PLACEMENT_3D ( 'NONE', #96625, #33719, #99796 ) ;
#30722=CARTESIAN_POINT ( 'NONE',  ( 6.530187263637528439, 7.647581891445782709, -1.199719254218452047 ) ) ;
#30754=EDGE_CURVE ( 'NONE', #75032, #186231, #132482, .T. ) ;
#30758=CARTESIAN_POINT ( 'NONE',  ( 5.401997860402196316, 5.267028690082820930, 0.000000000000000000 ) ) ;
#30759=CARTESIAN_POINT ( 'NONE',  ( -5.153507786970285665, 5.185049637652990207, -0.7216878364870338292 ) ) ;
#30762=FACE_OUTER_BOUND ( 'NONE', #179004, .T. ) ;
#30789=CARTESIAN_POINT ( 'NONE',  ( -6.466312919074983512, 6.508729591867735031, -0.7998128361456362523 ) ) ;
#30791=CARTESIAN_POINT ( 'NONE',  ( 4.868786560638878491, 8.694351730805124134, 0.7216878364870317197 ) ) ;
#30796=CARTESIAN_POINT ( 'NONE',  ( -3.983063267364693960, 7.868933921892603323, -0.7998128361456481317 ) ) ;
#30801=CARTESIAN_POINT ( 'NONE',  ( -5.957882158562513908, 5.915560371269843465, -0.7998128361456362523 ) ) ;
#30806=CARTESIAN_POINT ( 'NONE',  ( -5.261446130555064826, 8.296048364692991228, 1.199719254218452935 ) ) ;
#30819=CARTESIAN_POINT ( 'NONE',  ( -3.135678666510573365, 6.880318554229450712, 0.000000000000000000 ) ) ;
#30823=CARTESIAN_POINT ( 'NONE',  ( -6.970300371201519241, 7.304640985922785212, 0.7216878364870317197 ) ) ;
#30825=CARTESIAN_POINT ( 'NONE',  ( -7.404161286394468355, 7.810812053647902431, 0.000000000000000000 ) ) ;
#30826=CARTESIAN_POINT ( 'NONE',  ( 6.013923656113508542, 9.173938811177871244, -1.199719254218452047 ) ) ;
#30827=CARTESIAN_POINT ( 'NONE',  ( -7.279802135894939852, 7.457800344824362604, -0.7998128361456362523 ) ) ;
#30865=CARTESIAN_POINT ( 'NONE',  ( 4.641000714467984345, 8.433135692799648808, 0.4354600853693716411 ) ) ;
#30879=CARTESIAN_POINT ( 'NONE',  ( 6.710359684120930091, 6.793450817754725257, 0.7998128361456352531 ) ) ;
#30882=CARTESIAN_POINT ( 'NONE',  ( -4.197131071882288289, 7.054347462908075350, -1.199719254218455378 ) ) ;
#30887=CARTESIAN_POINT ( 'NONE',  ( -6.061904078641520144, 10.08632216847484031, 0.7216878364870267237 ) ) ;
#30891=CARTESIAN_POINT ( 'NONE',  ( 5.346851039111033543, 6.199209027673978412, -1.009771797811720884 ) ) ;
#30898=CARTESIAN_POINT ( 'NONE',  ( 4.655245641445829641, 6.524482229810530498, 1.599625672291269396 ) ) ;
#30900=CARTESIAN_POINT ( 'NONE',  ( 7.506374323821472849, 8.786466794993730289, -1.199719254218452047 ) ) ;
#30908=B_SPLINE_CURVE_WITH_KNOTS ( 'NONE', 3,
 ( #171793, #122066, #185888, #105768, #90566, #156626 ),
 .UNSPECIFIED., .F., .F.,
 ( 4, 2, 4 ),
 ( 0.000000000000000000, 0.002403146417856977853, 0.004806292835713955706 ),
 .UNSPECIFIED. ) ;
#30911=CARTESIAN_POINT ( 'NONE',  ( 3.627688620108284745, 6.389997935838436227, 1.199719254218452047 ) ) ;
#30916=CARTESIAN_POINT ( 'NONE',  ( 6.900173834712277632, 7.014900660111269559, -0.7998128361456341429 ) ) ;
#30924=CARTESIAN_POINT ( 'NONE',  ( -3.096514578442687515, 6.188910745953249304, -0.7944190528704382359 ) ) ;
#30927=CARTESIAN_POINT ( 'NONE',  ( -5.641601317062248988, 6.714861303728305586, -1.082531754730549967 ) ) ;
#30928=CARTESIAN_POINT ( 'NONE',  ( 4.367134877377630175, 7.148722219365612141, -1.082531754730548412 ) ) ;
#30940=CARTESIAN_POINT ( 'NONE',  ( -7.756673280794142755, 8.222076047114187602, -0.7216878364870338292 ) ) ;
#30941=CARTESIAN_POINT ( 'NONE',  ( 8.011942431032855083, 8.311964022485323511, 0.7998128361456291469 ) ) ;
#30944=CARTESIAN_POINT ( 'NONE',  ( 6.034787771414195312, 6.213209619504250547, -0.7216878364870458196 ) ) ;
#30963=CARTESIAN_POINT ( 'NONE',  ( 6.561219994370630637, 6.619454513046008515, 0.000000000000000000 ) ) ;
#30965=CARTESIAN_POINT ( 'NONE',  ( -3.817502770699643388, 6.611447778194983194, 1.199719254218452935 ) ) ;
#30972=CARTESIAN_POINT ( 'NONE',  ( 4.796824973295459316, 8.251456047330133714, 0.8599625132450954279 ) ) ;
#30976=CARTESIAN_POINT ( 'NONE',  ( 5.872089928494542477, 9.864872326636710653, 0.000000000000000000 ) ) ;
#30978=CARTESIAN_POINT ( 'NONE',  ( -7.293360289508603600, 7.473618190706972086, 0.000000000000000000 ) ) ;
#30979=CARTESIAN_POINT ( 'NONE',  ( 4.667750024854814050, 8.667735138964429709, -0.7998128361456381397 ) ) ;
#30988=CARTESIAN_POINT ( 'NONE',  ( -5.855142236255304944, 7.924361590421551860, -1.599625672291271394 ) ) ;
#31006=ORIENTED_EDGE ( 'NONE', *, *, #141509, .F. ) ;
#31016=CARTESIAN_POINT ( 'NONE',  ( 4.082413651490639062, 7.776916670132135501, 0.000000000000000000 ) ) ;
#31022=CARTESIAN_POINT ( 'NONE',  ( 5.546694241322223107, 5.643767167730274537, -0.7216878364870458196 ) ) ;
#31028=EDGE_CURVE ( 'NONE', #22839, #9659, #133301, .T. ) ;
#31035=CARTESIAN_POINT ( 'NONE',  ( -6.577640801285370209, 7.702944352034914566, -1.199719254218452047 ) ) ;
#31037=CARTESIAN_POINT ( 'NONE',  ( -6.291865805193673111, 9.498204651771386509, -1.199719254218452047 ) ) ;
#31043=CARTESIAN_POINT ( 'NONE',  ( 8.174640274396848483, 8.501778173076651512, 0.7998128361456291469 ) ) ;
#31049=CARTESIAN_POINT ( 'NONE',  ( -7.096767062110449942, 7.244259425409119046, -0.7998128361456362523 ) ) ;
#31055=CARTESIAN_POINT ( 'NONE',  ( -3.824808732831001201, 7.476377598362539345, 0.7216878364870338292 ) ) ;
#31058=CARTESIAN_POINT ( 'NONE',  ( -5.960744811863571968, 6.983232364376142698, 1.199719254218452935 ) ) ;
#31080=CARTESIAN_POINT ( 'NONE',  ( -3.296040741453672318, 6.859481608422314025, 0.7216878364870338292 ) ) ;
#31082=CARTESIAN_POINT ( 'NONE',  ( 4.004454267989866700, 5.765225627445230927, 1.599625672291262513 ) ) ;
#31083=CARTESIAN_POINT ( 'NONE',  ( -4.606738333593328072, 8.596554832492683929, 0.7998128361456281477 ) ) ;
#31103=CARTESIAN_POINT ( 'NONE',  ( 5.451787166470912993, 6.493411461371761284, -1.082531754730548412 ) ) ;
#31108=CARTESIAN_POINT ( 'NONE',  ( -6.770317605177755382, 8.992066187497757213, 1.599625672291269396 ) ) ;
#31133=CARTESIAN_POINT ( 'NONE',  ( 7.367930134383754215, 7.560616343061329125, -0.7998128361456341429 ) ) ;
#31146=CARTESIAN_POINT ( 'NONE',  ( 6.210774601750883583, 6.933448576277219111, 0.8519936491524527922 ) ) ;
#31148=CARTESIAN_POINT ( 'NONE',  ( 5.858531774880875176, 9.849054480754103835, -0.7216878364870458196 ) ) ;
#31153=CARTESIAN_POINT ( 'NONE',  ( -6.231907884136888676, 7.299589282028351001, -1.199719254218453823 ) ) ;
#31159=CARTESIAN_POINT ( 'NONE',  ( -6.658462837642833421, 8.861568958707010779, 1.443375672974064550 ) ) ;
#31162=CARTESIAN_POINT ( 'NONE',  ( -4.009374317532317100, 7.667071904143438310, 0.2036989888780231517 ) ) ;
#31167=CARTESIAN_POINT ( 'NONE',  ( -4.716257332707368910, 6.595662536282280719, -1.599625672291271394 ) ) ;
#31177=CARTESIAN_POINT ( 'NONE',  ( 5.734172623936983904, 5.654565914206774124, 0.7998128361456352531 ) ) ;
#31181=ORIENTED_EDGE ( 'NONE', *, *, #159414, .T. ) ;
#31196=CARTESIAN_POINT ( 'NONE',  ( -6.668631453075260396, 8.873432343378178544, -1.599625672291271394 ) ) ;
#31198=EDGE_CURVE ( 'NONE', #99015, #96867, #180973, .T. ) ;
#31200=CARTESIAN_POINT ( 'NONE',  ( -3.638309248663660345, 7.466720900074724554, 0.3421599456651515103 ) ) ;
#31203=CARTESIAN_POINT ( 'NONE',  ( -5.116488771863230589, 7.819496687688390679, 1.149033069458482270 ) ) ;
#31209=CARTESIAN_POINT ( 'NONE',  ( 4.342354338126830804, 8.288106837781779035, -0.7998128361456381397 ) ) ;
#31218=CARTESIAN_POINT ( 'NONE',  ( 6.536439455564155843, 8.719208346281938304, 1.443375672974065660 ) ) ;
#31229=CARTESIAN_POINT ( 'NONE',  ( -5.397554552016258889, 7.390509292142662723, 1.443375672974058777 ) ) ;
#31246=B_SPLINE_CURVE_WITH_KNOTS ( 'NONE', 3,
 ( #15493, #147664, #66362, #213681 ),
 .UNSPECIFIED., .F., .F.,
 ( 4, 4 ),
 ( 0.001636132410657741747, 0.002375893410536020125 ),
 .UNSPECIFIED. ) ;
#31247=EDGE_CURVE ( 'NONE', #188712, #7055, #194259, .T. ) ;
#31265=CARTESIAN_POINT ( 'NONE',  ( 4.369470645354133431, 8.319742529546998000, 0.7998128361456271485 ) ) ;
#31267=CARTESIAN_POINT ( 'NONE',  ( 6.170896192875352959, 7.228408975556602556, 1.199719254218453823 ) ) ;
#31279=CARTESIAN_POINT ( 'NONE',  ( -6.861835142292179057, 9.098836647464588978, 1.443375672974064550 ) ) ;
#31282=CARTESIAN_POINT ( 'NONE',  ( 6.197485614778188712, 6.403023770095574108, -0.7216878364870458196 ) ) ;
#31289=EDGE_CURVE ( 'NONE', #8487, #201520, #73810, .T. ) ;
#31295=CARTESIAN_POINT ( 'NONE',  ( -5.478903473698247595, 8.445785581739666981, -1.082531754730549967 ) ) ;
#31297=CARTESIAN_POINT ( 'NONE',  ( -5.641601317062259646, 5.754492089426966217, -0.7216878364870338292 ) ) ;
#31301=CARTESIAN_POINT ( 'NONE',  ( -5.612892248198118494, 5.720998175752135317, -0.08478118863167052877 ) ) ;
#31302=DIRECTION ( 'NONE',  ( -0.000000000000000000, -1.000000000000000000, -0.000000000000000000 ) ) ;
#31305=CARTESIAN_POINT ( 'NONE',  ( -4.329838433221154581, 8.065578932188461891, -0.1632719438462266193 ) ) ;
#31320=B_SPLINE_CURVE_WITH_KNOTS ( 'NONE', 3,
 ( #202898, #72911, #36143, #88115 ),
 .UNSPECIFIED., .F., .F.,
 ( 4, 4 ),
 ( 0.000000000000000000, 0.0002661342691797352611 ),
 .UNSPECIFIED. ) ;
#31324=CARTESIAN_POINT ( 'NONE',  ( -4.034433228518296666, 6.864533312316751790, -1.199719254218450271 ) ) ;
#31334=CARTESIAN_POINT ( 'NONE',  ( -7.045397100956844127, 8.248660034984974132, -1.199719254218452047 ) ) ;
#31335=CARTESIAN_POINT ( 'NONE',  ( -5.569768141569340969, 7.516503378918355516, 1.348759926630802131 ) ) ;
#31341=PLANE ( 'NONE',  #12861 ) ;
#31345=CARTESIAN_POINT ( 'NONE',  ( -4.034433228518296666, 6.864533312316751790, -1.199719254218450271 ) ) ;
#31356=CARTESIAN_POINT ( 'NONE',  ( 6.384963997392946844, 6.413822516572072807, 0.7998128361456352531 ) ) ;
#31379=CARTESIAN_POINT ( 'NONE',  ( 5.554000203453580475, 6.508696987897830688, -1.199719254218452047 ) ) ;
#31380=CARTESIAN_POINT ( 'NONE',  ( 4.411198876399872404, 6.239761003923544713, -1.599625672291273171 ) ) ;
#31382=CARTESIAN_POINT ( 'NONE',  ( 3.203469434578891661, 6.959407783642502565, -0.7998128361456362523 ) ) ;
#31385=CYLINDRICAL_SURFACE ( 'NONE', #96269, 1.250000000000000000 ) ;
#31393=CARTESIAN_POINT ( 'NONE',  ( 4.684384365712907616, 8.380862967975740929, 0.5977175665230231028 ) ) ;
#31395=CARTESIAN_POINT ( 'NONE',  ( -6.265276382846530545, 6.482112999508623297, 0.000000000000000000 ) ) ;
#31396=CARTESIAN_POINT ( 'NONE',  ( 2.943528747942701695, 6.448217615992859919, 0.000000000000000000 ) ) ;
#31422=CARTESIAN_POINT ( 'NONE',  ( 5.740951700743842423, 5.662474837148078421, -0.7998128361456481317 ) ) ;
#31424=CARTESIAN_POINT ( 'NONE',  ( 4.706615602599436343, 5.520081620234675412, 1.199719254218452935 ) ) ;
#31426=ORIENTED_EDGE ( 'NONE', *, *, #203130, .T. ) ;
#31442=CARTESIAN_POINT ( 'NONE',  ( -6.903036488013351679, 8.082572653217566128, -1.199719254218452047 ) ) ;
#31455=CARTESIAN_POINT ( 'NONE',  ( 6.475954649182838807, 7.584310507915338562, 1.199719254218452047 ) ) ;
#31459=CARTESIAN_POINT ( 'NONE',  ( 6.873057527484919937, 6.983264968346048818, 0.7998128361456352531 ) ) ;
#31473=CARTESIAN_POINT ( 'NONE',  ( 4.713861384769566953, 8.227931952640012980, -0.6562286284988675389 ) ) ;
#31490=CARTESIAN_POINT ( 'NONE',  ( 3.106226591306694651, 6.638031766584184368, 0.000000000000000000 ) ) ;
#31496=CARTESIAN_POINT ( 'NONE',  ( -6.119526231721793330, 8.232809585132461194, 1.599625672291263179 ) ) ;
#31498=CARTESIAN_POINT ( 'NONE',  ( 5.875479466675786355, 7.948088359245467416, -1.599625672291283607 ) ) ;
#31502=CARTESIAN_POINT ( 'NONE',  ( -7.937372586157736443, 8.224965870130965584, 0.7998128361456341429 ) ) ;
#31509=CARTESIAN_POINT ( 'NONE',  ( -0.3407659764052391460, 3.347064181880099021, -1.971699800770186695 ) ) ;
#31520=CARTESIAN_POINT ( 'NONE',  ( 6.137203345855459347, 5.375636887024366928, 2.500000000000000888 ) ) ;
#31525=CARTESIAN_POINT ( 'NONE',  ( 4.733205024946604667, 8.536173272497439513, 0.000000000000000000 ) ) ;
#31540=CARTESIAN_POINT ( 'NONE',  ( -5.370438244788932280, 6.398504386076097283, 1.082531754730549078 ) ) ;
#31542=CARTESIAN_POINT ( 'NONE',  ( 4.877901405866606588, 8.912911750144889567, 0.7998128361456341429 ) ) ;
#31545=AXIS2_PLACEMENT_3D ( 'NONE', #36469, #152365, #100407 ) ;
#31576=EDGE_CURVE ( 'NONE', #53708, #134461, #96734, .T. ) ;
#31586=DIRECTION ( 'NONE',  ( 0.000000000000000000, 0.000000000000000000, 1.000000000000000000 ) ) ;
#31587=FACE_OUTER_BOUND ( 'NONE', #26054, .T. ) ;
#31591=CARTESIAN_POINT ( 'NONE',  ( 4.927462483923885195, 4.713404084191450849, -0.7998128361456481317 ) ) ;
#31595=CARTESIAN_POINT ( 'NONE',  ( -5.194182247366913252, 7.153241603385088965, 1.443375672974058777 ) ) ;
#31596=CYLINDRICAL_SURFACE ( 'NONE', #25081, 0.7500000000000006661 ) ;
#31601=CARTESIAN_POINT ( 'NONE',  ( -4.423703259808839938, 8.383013913077441259, 0.7998128361456352531 ) ) ;
#31611=CARTESIAN_POINT ( 'NONE',  ( -5.306037014901836990, 7.283738832175834510, 1.599625672291263179 ) ) ;
#31614=CARTESIAN_POINT ( 'NONE',  ( 5.403926048761924505, 7.658933883257522446, 1.327442161737320436 ) ) ;
#31617=CIRCLE ( 'NONE', #145753, 0.08000000000000020983 ) ;
#31620=CARTESIAN_POINT ( 'NONE',  ( 6.530187263637528439, 7.647581891445782709, -1.199719254218452047 ) ) ;
#31627=CARTESIAN_POINT ( 'NONE',  ( -3.332271893908731464, 7.109677319527304640, -0.7998128361456481317 ) ) ;
#31631=CARTESIAN_POINT ( 'NONE',  ( -5.611095471209320174, 7.639640364534566075, 1.599625672291263179 ) ) ;
#31635=CARTESIAN_POINT ( 'NONE',  ( 5.506019780481205217, 9.437790487287811558, 0.000000000000000000 ) ) ;
#31637=CARTESIAN_POINT ( 'NONE',  ( -6.902509602688821744, 8.185920970292658083, -1.082531754730549967 ) ) ;
#31643=CARTESIAN_POINT ( 'NONE',  ( 5.337069745634900997, 6.255611453776062980, 1.199719254218452047 ) ) ;
#31661=ADVANCED_FACE ( 'NONE', ( #198502 ), #163128, .T. ) ;
#31673=CARTESIAN_POINT ( 'NONE',  ( 4.871809496981259535, 8.050285353323946680, -0.9368363805376724862 ) ) ;
#31682=CARTESIAN_POINT ( 'NONE',  ( 5.806634928402749196, 9.996434193103704402, -0.7998128361456481317 ) ) ;
#31687=CARTESIAN_POINT ( 'NONE',  ( -5.310352258326699548, 7.640991054048470232, -1.228972953101372223 ) ) ;
#31705=CARTESIAN_POINT ( 'NONE',  ( -3.546339698426324460, 6.295090860542775779, -1.199719254218450271 ) ) ;
#31709=AXIS2_PLACEMENT_3D ( 'NONE', #44141, #175214, #163220 ) ;
#31710=LINE ( 'NONE', #159561, #119708 ) ;
#31717=CARTESIAN_POINT ( 'NONE',  ( 4.342354338126830804, 8.288106837781779035, -0.7998128361456381397 ) ) ;
#31720=CARTESIAN_POINT ( 'NONE',  ( 6.495764994278809823, 7.711385593814346073, 1.082531754730549967 ) ) ;
#31735=CARTESIAN_POINT ( 'NONE',  ( -6.069210040772897052, 7.109775131437022999, -1.199719254218453823 ) ) ;
#31736=CARTESIAN_POINT ( 'NONE',  ( 3.203469434578891661, 6.959407783642502565, -0.7998128361456362523 ) ) ;
#31747=CARTESIAN_POINT ( 'NONE',  ( -6.424584688029276514, 8.588711117491191871, 1.599625672291269396 ) ) ;
#31748=CARTESIAN_POINT ( 'NONE',  ( 5.155843554946782703, 9.237177590738404831, -0.7998128361456481317 ) ) ;
#31751=DIRECTION ( 'NONE',  ( 0.000000000000000000, 0.000000000000000000, -1.000000000000000000 ) ) ;
#31754=CARTESIAN_POINT ( 'NONE',  ( -1.833030277982346634, 0.000000000000000000, -2.499999999999998668 ) ) ;
#31756=CARTESIAN_POINT ( 'NONE',  ( 5.401997860402196316, 5.267028690082820930, 0.000000000000000000 ) ) ;
#31764=CARTESIAN_POINT ( 'NONE',  ( -6.601093878019091754, 6.767222581227101408, 0.2246719935465150975 ) ) ;
#31772=CARTESIAN_POINT ( 'NONE',  ( -2.997761361953021009, 6.511488999004883205, -0.7216878364870458196 ) ) ;
#31773=CARTESIAN_POINT ( 'NONE',  ( -3.296040741453672318, 6.859481608422314025, 0.7216878364870338292 ) ) ;
#31785=CARTESIAN_POINT ( 'NONE',  ( -3.177206141917641613, 8.963489737286122860, 2.499999999999999556 ) ) ;
#31797=DIRECTION ( 'NONE',  ( -0.6507913734559640506, -0.7592566023653003482, 0.000000000000000000 ) ) ;
#31821=CARTESIAN_POINT ( 'NONE',  ( 7.851580356089786328, 8.332800968292465527, 0.000000000000000000 ) ) ;
#31822=CARTESIAN_POINT ( 'NONE',  ( -3.038435823238377687, 6.558942537171132514, -0.7216878364870458196 ) ) ;
#31851=CARTESIAN_POINT ( 'NONE',  ( -6.089547271193396227, 7.133501900260939443, -1.199719254218453823 ) ) ;
#31853=CARTESIAN_POINT ( 'NONE',  ( 6.170369307550815030, 8.292126506933040986, 1.443375672974064550 ) ) ;
#31858=AXIS2_PLACEMENT_3D ( 'NONE', #188285, #87601, #35630 ) ;
#31859=CARTESIAN_POINT ( 'NONE',  ( -6.282224075085783177, 8.422623735723785643, 1.599625672291269396 ) ) ;
#31867=CARTESIAN_POINT ( 'NONE',  ( -5.315678745009726924, 8.359319748223434487, -1.199719254218453823 ) ) ;
#31879=CARTESIAN_POINT ( 'NONE',  ( -6.134138155540168391, 6.121192367743780949, 0.000000000000000000 ) ) ;
#31883=CARTESIAN_POINT ( 'NONE',  ( -7.024532985656169792, 9.288650798055913427, 1.443375672974064550 ) ) ;
#31885=CARTESIAN_POINT ( 'NONE',  ( -6.794044373779495771, 8.059378203231773341, 1.082531754730549078 ) ) ;
#31886=CARTESIAN_POINT ( 'NONE',  ( 6.851666526859736983, 9.086973262793417661, -1.599625672291269396 ) ) ;
#31887=CARTESIAN_POINT ( 'NONE',  ( -7.767895665986912057, 8.027242796598338614, -0.7998128361456362523 ) ) ;
#31895=VERTEX_POINT ( 'NONE', #173521 ) ;
#31902=CARTESIAN_POINT ( 'NONE',  ( -0.4461809497497637444, 3.122791860410086606, 1.949595486268986821 ) ) ;
#31907=CARTESIAN_POINT ( 'NONE',  ( 6.308853223578811509, 6.964933332891984463, 0.9108697706533327443 ) ) ;
#31924=CARTESIAN_POINT ( 'NONE',  ( 6.455362170788604637, 6.771378801287749383, -0.3290997004737963860 ) ) ;
#31938=CARTESIAN_POINT ( 'NONE',  ( -3.644109427023046521, 7.473487774827342278, 0.000000000000000000 ) ) ;
#31946=CARTESIAN_POINT ( 'NONE',  ( 0.000000000000000000, 2.480000000000016858, 0.000000000000000000 ) ) ;
#31952=CARTESIAN_POINT ( 'NONE',  ( 4.869313445963426190, 5.709895770826003414, 1.199719254218452935 ) ) ;
#31955=CARTESIAN_POINT ( 'NONE',  ( 5.993586425693011144, 9.150212042353954800, -1.199719254218452047 ) ) ;
#31961=CARTESIAN_POINT ( 'NONE',  ( -5.763624699140874164, 8.777960344756069233, -1.082531754730549967 ) ) ;
#31968=CARTESIAN_POINT ( 'NONE',  ( 5.677832469072920496, 9.846164657218904992, 0.000000000000000000 ) ) ;
#31978=B_SPLINE_CURVE_WITH_KNOTS ( 'NONE', 3,
 ( #54573, #103325, #120721, #22033 ),
 .UNSPECIFIED., .F., .F.,
 ( 4, 4 ),
 ( 0.000000000000000000, 0.0002852742075882630057 ),
 .UNSPECIFIED. ) ;
#31984=CARTESIAN_POINT ( 'NONE',  ( -6.780486220610186798, 8.043560357867583832, -1.082531754730549967 ) ) ;
#31985=CARTESIAN_POINT ( 'NONE',  ( 5.234856708652227297, 7.200695141551334721, 1.443375672974065660 ) ) ;
#31994=CARTESIAN_POINT ( 'NONE',  ( -7.282137904315833410, 7.668451441222825515, 0.000000000000000000 ) ) ;
#31995=CARTESIAN_POINT ( 'NONE',  ( 6.339319342841494453, 9.553567112360518365, -1.199719254218452047 ) ) ;
#31999=CARTESIAN_POINT ( 'NONE',  ( 4.977251789548238214, 7.860525283564661514, -1.082531754730548412 ) ) ;
#32016=CARTESIAN_POINT ( 'NONE',  ( -4.573896719763875574, 6.429575154514868274, -1.599625672291271394 ) ) ;
#32026=CARTESIAN_POINT ( 'NONE',  ( 3.366167277942881064, 7.149221934233827014, -0.7998128361456362523 ) ) ;
#32028=CARTESIAN_POINT ( 'NONE',  ( -5.444481204339554736, 8.509589284108232121, 1.199719254218454489 ) ) ;
#32029=CARTESIAN_POINT ( 'NONE',  ( 6.150558962454855561, 7.204682206732687000, 1.199719254218452047 ) ) ;
#32037=CARTESIAN_POINT ( 'NONE',  ( -4.288121723672178476, 8.224835454251337552, -0.7998128361456362523 ) ) ;
#32064=CARTESIAN_POINT ( 'NONE',  ( 5.261973015879598314, 5.311592404713873172, -0.7216878364870458196 ) ) ;
#32071=CARTESIAN_POINT ( 'NONE',  ( 4.190878879955609371, 7.903459436674603822, -0.7216878364870338292 ) ) ;
#32082=CARTESIAN_POINT ( 'NONE',  ( -4.471156797456668386, 8.438376373666578445, -0.7998128361456362523 ) ) ;
#32084=CARTESIAN_POINT ( 'NONE',  ( -7.747558435566414659, 8.003516027774422170, -0.7998128361456362523 ) ) ;
#32092=CARTESIAN_POINT ( 'NONE',  ( 6.607619761813720238, 8.802252036906432764, 1.599625672291268286 ) ) ;
#32098=CARTESIAN_POINT ( 'NONE',  ( 5.038060948978250408, 7.997685013099862239, -1.157798351953726490 ) ) ;
#32099=CARTESIAN_POINT ( 'NONE',  ( -7.370792787684826486, 8.628288336167626582, -1.199719254218452047 ) ) ;
#32105=CARTESIAN_POINT ( 'NONE',  ( -5.316205630334263965, 7.295602216847000498, -1.443375672974066548 ) ) ;
#32108=CARTESIAN_POINT ( 'NONE',  ( -6.608673532018475960, 6.674816973635147477, -0.7998128361456362523 ) ) ;
#32115=CARTESIAN_POINT ( 'NONE',  ( -4.868786560638931782, 6.773613302202437403, 1.443375672974058777 ) ) ;
#32131=CARTESIAN_POINT ( 'NONE',  ( -3.133342898089680695, 6.669667457830990465, 0.7216878364870338292 ) ) ;
#32132=CARTESIAN_POINT ( 'NONE',  ( 3.953084306836263995, 6.769626237021087789, 1.199719254218452047 ) ) ;
#32133=CARTESIAN_POINT ( 'NONE',  ( -5.764151584465413869, 6.753873599078290546, -1.199719254218453823 ) ) ;
#32158=CARTESIAN_POINT ( 'NONE',  ( -5.420227550413282636, 9.545625585449309725, 0.7998128361456291469 ) ) ;
#32182=CARTESIAN_POINT ( 'NONE',  ( 4.573896719763862251, 6.429575154514868274, -1.599625672291273171 ) ) ;
#32195=CARTESIAN_POINT ( 'NONE',  ( 4.631618433768171172, 8.327536854573105884, -0.3785340233409782984 ) ) ;
#32197=CARTESIAN_POINT ( 'NONE',  ( 7.512626515748109135, 8.897724035528543851, 1.082531754730549967 ) ) ;
#32203=CARTESIAN_POINT ( 'NONE',  ( -5.611095471209320174, 7.639640364534566075, 1.599625672291263179 ) ) ;
#32210=CARTESIAN_POINT ( 'NONE',  ( -6.360183458142173230, 9.473945563590925545, 1.082531754730549967 ) ) ;
#32214=CARTESIAN_POINT ( 'NONE',  ( -5.477447344779489136, 6.303105555648046199, 0.9994663861491676071 ) ) ;
#32221=CARTESIAN_POINT ( 'NONE',  ( -3.949167883330528372, 7.829389307186077396, 1.214306433183764966E-14 ) ) ;
#32231=CARTESIAN_POINT ( 'NONE',  ( 4.869313445963426190, 5.709895770826003414, 1.199719254218452935 ) ) ;
#32249=CARTESIAN_POINT ( 'NONE',  ( -6.328223859912621485, 6.936542968411253618, 0.8711560941448781570 ) ) ;
#32252=CARTESIAN_POINT ( 'NONE',  ( -7.533490631048818109, 8.818102486758951031, -1.199719254218452047 ) ) ;
#32265=CARTESIAN_POINT ( 'NONE',  ( 4.532168488718122390, 8.509556680138327778, 0.7998128361456271485 ) ) ;
#32272=CARTESIAN_POINT ( 'NONE',  ( 4.638297949650961982, 5.544340708415133712, -1.082531754730548412 ) ) ;
#32276=CARTESIAN_POINT ( 'NONE',  ( 5.370438244788902971, 9.279612028980123384, -0.7216878364870458196 ) ) ;
#32281=DIRECTION ( 'NONE',  ( 0.000000000000000000, -1.000000000000000000, 0.000000000000000000 ) ) ;
#32287=CARTESIAN_POINT ( 'NONE',  ( -5.885648082108231982, 7.959951743916638733, 1.443375672974058777 ) ) ;
#32320=CARTESIAN_POINT ( 'NONE',  ( 5.825163275726873202, 6.825053905550038991, 1.199719254218452047 ) ) ;
#32322=CARTESIAN_POINT ( 'NONE',  ( 5.631432701629774051, 7.663367133358481631, 1.599625672291269396 ) ) ;
#32324=DIRECTION ( 'NONE',  ( 0.7592566023653005702, 0.6507913734559639396, 0.000000000000000000 ) ) ;
#32334=CARTESIAN_POINT ( 'NONE',  ( -3.634467696915153034, 6.397906858779740524, 1.199719254218452935 ) ) ;
#32337=CARTESIAN_POINT ( 'NONE',  ( 4.380693030546913391, 7.164540064729805202, 1.082531754730549078 ) ) ;
#32348=VECTOR ( 'NONE', #148885, 1000.000000000000114 ) ;
#32353=CARTESIAN_POINT ( 'NONE',  ( -5.316205630334251531, 9.216340645449683677, -0.7216878364870338292 ) ) ;
#32354=ORIENTED_EDGE ( 'NONE', *, *, #6983, .F. ) ;
#32355=CARTESIAN_POINT ( 'NONE',  ( -5.153507786970276783, 6.145418851954329575, -1.082531754730549967 ) ) ;
#32384=CARTESIAN_POINT ( 'NONE',  ( -5.842637852846353397, 5.781108681267656202, 0.7998128361456281477 ) ) ;
#32393=CARTESIAN_POINT ( 'NONE',  ( -5.589704470584107909, 9.743348658981940247, -0.7998128361456362523 ) ) ;
#32394=CARTESIAN_POINT ( 'NONE',  ( -5.628650723579520232, 7.468463085569896798, -1.343613510788654875 ) ) ;
#32411=CARTESIAN_POINT ( 'NONE',  ( 4.701645408888975197, 8.707279753670952971, 0.000000000000000000 ) ) ;
#32436=CARTESIAN_POINT ( 'NONE',  ( 7.503511670520385479, 7.718794801887437274, 0.7998128361456281477 ) ) ;
#32437=CARTESIAN_POINT ( 'NONE',  ( 4.362691568547328202, 8.311833606605697256, -0.7998128361456381397 ) ) ;
#32439=CARTESIAN_POINT ( 'NONE',  ( 5.876533236880477240, 5.820653295974182129, 0.7998128361456352531 ) ) ;
#32450=CARTESIAN_POINT ( 'NONE',  ( 4.632842592818133376, 8.443130954262043630, -0.3954830847591808696 ) ) ;
#32451=CARTESIAN_POINT ( 'NONE',  ( -4.950135482320914271, 8.789258806100786359, -0.7216878364870338292 ) ) ;
#32452=CARTESIAN_POINT ( 'NONE',  ( 3.255366281057017197, 6.812028071292901998, -0.7216878364870338292 ) ) ;
#32474=CARTESIAN_POINT ( 'NONE',  ( 6.527324610336440180, 6.579909898339485252, 0.7998128361456331437 ) ) ;
#32476=CARTESIAN_POINT ( 'NONE',  ( 4.492547798081839794, 6.334668079219206049, 1.599625672291262513 ) ) ;
#32495=CARTESIAN_POINT ( 'NONE',  ( -4.167236710886554896, 7.875866928964825320, -0.1619875888596494506 ) ) ;
#32505=CARTESIAN_POINT ( 'NONE',  ( 5.017399365509065845, 8.011327138806002779, -1.199719254218450271 ) ) ;
#32509=CARTESIAN_POINT ( 'NONE',  ( -5.955741603288206676, 7.127506980570093020, 1.099513196254948699 ) ) ;
#32510=CARTESIAN_POINT ( 'NONE',  ( 5.224688093219824303, 7.188831756880171397, -1.599625672291283607 ) ) ;
#32515=ORIENTED_EDGE ( 'NONE', *, *, #118802, .F. ) ;
#32521=CARTESIAN_POINT ( 'NONE',  ( 4.622017735560743468, 8.339529265130579461, 0.3277269337885590494 ) ) ;
#32530=CARTESIAN_POINT ( 'NONE',  ( 4.584065335196261692, 7.401807753487379848, 1.082531754730549078 ) ) ;
#32543=CARTESIAN_POINT ( 'NONE',  ( -6.688968683495758683, 8.897159112202094988, -1.599625672291271394 ) ) ;
#32545=CARTESIAN_POINT ( 'NONE',  ( 4.362691568547328202, 8.311833606605697256, -0.7998128361456381397 ) ) ;
#32548=FACE_OUTER_BOUND ( 'NONE', #42243, .T. ) ;
#32556=CARTESIAN_POINT ( 'NONE',  ( -6.462985781203115287, 6.858296038324478872, -0.6802466501308057634 ) ) ;
#32571=VECTOR ( 'NONE', #6899, 1000.000000000000114 ) ;
#32575=CARTESIAN_POINT ( 'NONE',  ( 5.641601317062233001, 7.675230518029648508, -1.443375672974078761 ) ) ;
#32589=CARTESIAN_POINT ( 'NONE',  ( -5.994113311017573054, 6.165756082374834079, 0.7216878364870257245 ) ) ;
#32591=CARTESIAN_POINT ( 'NONE',  ( 6.658989722967328717, 7.797851427330578566, 1.199719254218452935 ) ) ;
#32593=B_SPLINE_CURVE_WITH_KNOTS ( 'NONE', 3,
 ( #158107, #56327, #157040, #172218 ),
 .UNSPECIFIED., .F., .F.,
 ( 4, 4 ),
 ( 0.000000000000000000, 0.0005811582027346231649 ),
 .UNSPECIFIED. ) ;
#32595=CARTESIAN_POINT ( 'NONE',  ( -7.014364370223741929, 9.276787413384745662, -1.599625672291271394 ) ) ;
#32597=CARTESIAN_POINT ( 'NONE',  ( -6.563028877466991595, 9.814561569423593923, 1.199719254218452935 ) ) ;
#32607=CARTESIAN_POINT ( 'NONE',  ( -4.094037528094973233, 3.811616672697257346, 2.445516385416635963 ) ) ;
#32640=CARTESIAN_POINT ( 'NONE',  ( 3.067887898442204442, 6.801229324816399746, 0.7998128361456271485 ) ) ;
#32645=CARTESIAN_POINT ( 'NONE',  ( -5.600926855776894975, 6.667407765562058053, -1.082531754730549967 ) ) ;
#32650=ORIENTED_EDGE ( 'NONE', *, *, #27143, .F. ) ;
#32651=CARTESIAN_POINT ( 'NONE',  ( -4.925354943514475003, 8.968274210734028529, 0.000000000000000000 ) ) ;
#32657=CARTESIAN_POINT ( 'NONE',  ( 6.481679955784983349, 9.719654494127929922, -1.199719254218452047 ) ) ;
#32658=CARTESIAN_POINT ( 'NONE',  ( -4.956387674247580755, 7.940146832334256111, 1.199719254218452935 ) ) ;
#32661=CARTESIAN_POINT ( 'NONE',  ( 6.493754380866193721, 6.839952184459461293, 0.5864284347954504817 ) ) ;
#32666=CARTESIAN_POINT ( 'NONE',  ( 6.261886844665240481, 8.398896966899865646, 1.599625672291268286 ) ) ;
#32673=EDGE_CURVE ( 'NONE', #77529, #123242, #174766, .T. ) ;
#32675=CARTESIAN_POINT ( 'NONE',  ( -4.842197138736131556, 5.678260079060780008, 1.199719254218452935 ) ) ;
#32680=CARTESIAN_POINT ( 'NONE',  ( -4.925354943514475003, 8.968274210734028529, 0.000000000000000000 ) ) ;
#32684=CARTESIAN_POINT ( 'NONE',  ( 6.848276988234151652, 7.162280372460873679, -0.7216878364870317197 ) ) ;
#32686=CARTESIAN_POINT ( 'NONE',  ( -5.763624699140868834, 9.738329559057408602, -0.7216878364870338292 ) ) ;
#32692=CARTESIAN_POINT ( 'NONE',  ( 5.855142236255289845, 7.924361590421551860, -1.599625672291281386 ) ) ;
#32706=EDGE_CURVE ( 'NONE', #94850, #156724, #213031, .T. ) ;
#32725=VECTOR ( 'NONE', #62122, 1000.000000000000114 ) ;
#32727=LINE ( 'NONE', #180056, #22943 ) ;
#32731=ORIENTED_EDGE ( 'NONE', *, *, #61327, .T. ) ;
#32736=CARTESIAN_POINT ( 'NONE',  ( -6.127277117991962285, 7.006264510460848527, -0.9572512136472415278 ) ) ;
#32740=EDGE_CURVE ( 'NONE', #36910, #71609, #60755, .T. ) ;
#32755=CARTESIAN_POINT ( 'NONE',  ( -8.100070429521727178, 8.414780020722290033, 0.7998128361456341429 ) ) ;
#32765=EDGE_LOOP ( 'NONE', ( #67711, #147045, #158950, #208148, #37988, #202252 ) ) ;
#32770=CARTESIAN_POINT ( 'NONE',  ( 6.042093733545556233, 7.078139439671806699, -1.199719254218452047 ) ) ;
#32773=CARTESIAN_POINT ( 'NONE',  ( 6.848276988234151652, 7.162280372460873679, -0.7216878364870317197 ) ) ;
#32789=CARTESIAN_POINT ( 'NONE',  ( -5.906512197408906317, 6.919960980845699439, -1.199719254218453823 ) ) ;
#32791=CARTESIAN_POINT ( 'NONE',  ( 3.607351389687783794, 6.366271167014519783, 1.199719254218451159 ) ) ;
#32801=CARTESIAN_POINT ( 'NONE',  ( -5.901542003698421190, 10.10715911428198055, 0.000000000000000000 ) ) ;
#32802=CARTESIAN_POINT ( 'NONE',  ( 5.169401708560450004, 9.252995436621013425, 0.000000000000000000 ) ) ;
#32808=CARTESIAN_POINT ( 'NONE',  ( 5.239300017038202917, 5.077214539491492928, 0.000000000000000000 ) ) ;
#32816=CARTESIAN_POINT ( 'NONE',  ( -6.387810837761664473, 6.908839790476999809, 0.8166356711787735589 ) ) ;
#32824=CARTESIAN_POINT ( 'NONE',  ( -7.014364370223741929, 9.276787413384745662, -1.599625672291271394 ) ) ;
#32829=CARTESIAN_POINT ( 'NONE',  ( -5.514013019825418915, 5.994650414344389056, -0.9619886414689113874 ) ) ;
#32836=CARTESIAN_POINT ( 'NONE',  ( -6.387350227228854038, 6.552219065274637266, 2.500000000000690559 ) ) ;
#32855=CARTESIAN_POINT ( 'NONE',  ( 5.923986774528332333, 5.876015756563318426, -0.7998128361456481317 ) ) ;
#32874=CARTESIAN_POINT ( 'NONE',  ( 3.607351389687783794, 6.366271167014519783, 1.199719254218451159 ) ) ;
#32875=CARTESIAN_POINT ( 'NONE',  ( -3.933273961740340496, 5.682181936820735579, 1.443375672974065660 ) ) ;
#32889=CARTESIAN_POINT ( 'NONE',  ( -3.147653791585856009, 8.920000000000001705, -2.419999999999835616 ) ) ;
#32901=CARTESIAN_POINT ( 'NONE',  ( -6.642568916052639771, 6.714361588341672515, 0.000000000000000000 ) ) ;
#32903=CARTESIAN_POINT ( 'NONE',  ( 6.983858524370782916, 7.320458831286981827, 0.7216878364870328300 ) ) ;
#32908=CARTESIAN_POINT ( 'NONE',  ( -7.144220599758281054, 7.299621885998258897, 0.7998128361456341429 ) ) ;
#32918=CARTESIAN_POINT ( 'NONE',  ( -7.045397100956844127, 8.248660034984974132, -1.199719254218452047 ) ) ;
#32931=CARTESIAN_POINT ( 'NONE',  ( -4.261005416444848315, 8.193199762486115034, 0.7998128361456352531 ) ) ;
#32935=CARTESIAN_POINT ( 'NONE',  ( -6.672020991700860826, 7.917017590806697314, 1.082531754730549078 ) ) ;
#32937=CARTESIAN_POINT ( 'NONE',  ( -5.587368702163209910, 9.532697562583475559, 0.000000000000000000 ) ) ;
#32938=CARTESIAN_POINT ( 'NONE',  ( 6.444921918449731280, 8.612437886315108315, 1.599625672291268286 ) ) ;
#32940=CARTESIAN_POINT ( 'NONE',  ( -3.973948422136981407, 5.729635473950147606, -1.443375672974066548 ) ) ;
#32960=CARTESIAN_POINT ( 'NONE',  ( 6.587573780899039555, 6.778200402807202707, -0.2451836268814889253 ) ) ;
#32978=CARTESIAN_POINT ( 'NONE',  ( 5.410124943364367667, 7.538760657221164507, -1.247639402986647550 ) ) ;
#32991=B_SPLINE_SURFACE_WITH_KNOTS ( 'NONE', 1, 3, ( 
 ( #69655, #88069, #119563, #1448, #135763, #70715, #169315, #153068, #4645, #202854, #154142, #5710, #55569, #39317, #149883, #67513, #10007, #158407, #189827, #174680, #27325, #125985, #41476, #208199, #140046, #191942, #59832, #43607, #172531, #155208, #60900, #24115, #124921, #76083, #173619, #106504, #91295, #188762, #90218, #25191, #109725, #11065, #207144, #107586, #190883, #56639, #157353, #175732, #93427, #204995, #42549, #159466, #77144, #23039, #138972, #156282, #142184, #127059, #122803, #73954, #40402, #171450, #108652, #89155, #8942, #143265, #26253, #209255, #75022, #7866, #141134, #206071, #58767, #57705, #193021, #123862, #92370, #105412, #6789, #72866, #12140, #66192, #29477, #65141, #213518, #95568, #28402, #161618, #45742, #179991, #32661, #46809, #211402, #13211, #79284, #131297, #112923, #162683, #181045, #80348, #94496, #145402, #163747, #178936, #210336, #146448, #130249, #97689, #63032, #30550, #196240, #195176, #197288, #15326, #81416, #129199, #113996, #98740, #48928, #96629, #147497, #14257, #115047, #164798, #16390, #111860, #160534, #125, #177865, #128129, #82469, #212462, #144336, #78212, #44673, #64107, #148559, #47883, #31614, #132337, #110785, #176787, #61975, #194092, #153888, #152813, #53179, #70462, #104071, #1200, #150698, #17452, #183176, #2260, #19602, #119307, #166939, #116101, #198343, #83536, #185293, #49983, #149618, #68336, #120389, #200471, #170118, #133401, #199405, #136579, #5457, #186364, #21704, #51051, #84609, #34780, #36917, #67262, #37999, #117174, #54252, #71537, #103000, #86743, #100854, #169056, #85674, #134468, #18532, #182092, #118246, #33723, #20653, #4391, #52118, #87816, #184228, #35852, #202599, #99801, #101930, #165866, #167996, #201531, #151762, #3331, #69401, #135508, #122544, #88898, #203667, #107325, #55316, #172273, #58513, #189572, #42285, #23860, #154952, #73691, #72615, #7607, #204731, #108397 ),
 ( #138714, #124668, #206881, #56381, #121467, #188505, #6537, #91035, #174421, #89967, #40136, #106249, #156019, #190625, #139789, #205816, #25997, #57448, #187437, #123609, #8684, #41219, #171191, #173349, #24931, #157095, #74766, #140869, #92106, #158161, #9752, #75828, #141935, #207948, #137647, #39065, #105151, #22781, #5079, #151381, #137271, #71154, #54938, #183858, #166552, #72225, #35471, #200095, #121090, #52794, #1882, #84228, #116789, #167618, #88517, #53873, #19217, #85295, #117867, #37616, #104768, #118933, #69022, #101549, #2950, #203291, #184913, #20284, #38689, #152438, #18140, #135139, #21335, #36537, #67942, #4017, #202219, #169746, #201155, #102624, #120006, #168680, #187057, #87441, #153510, #86368, #185982, #170817, #22408, #70086, #154579, #136201, #6156, #138332, #204348, #103696, #150316, #182786, #34404, #51744, #100476, #134086, #90082, #26117, #125850, #56501, #42408, #189688, #142046, #138831, #23979, #157209, #209119, #74884, #192876, #7727, #73811, #159326, #94355, #60757, #44531, #139905, #173475, #123726, #191806, #172391, #126918, #156145, #143125, #28263, #43471, #175595, #205936, #109589, #108514, #8806, #57568, #160397, #207000, #122662, #27184, #93290, #25052, #110649, #140992, #41339, #10923, #72734, #107448, #76998, #204848, #174541, #188625, #91155, #58631, #124784, #190744, #40256, #92228, #106368, #176650, #158279, #9869, #75945, #208062, #59687, #66050, #48785, #14114, #30409, #144198, #112783, #78074, #97547, #196103, #62884, #145255, #80204, #45599, #128477, #95428, #177724, #32521, #197147, #193951, #33580, #211260, #98596, #180899, #129053, #210194, #195028, #13060, #147353, #132194, #146306, #178793, #46662, #96494, #164658, #212319, #130112, #148418, #47738, #61830, #162543, #131156, #63956, #29334, #113854, #163604, #65004, #179849, #31473, #15186, #81276, #16241, #114902, #82326, #213380, #198202, #49836, #115962, #181952 ) ),
 .UNSPECIFIED., .F., .T., .F.,
 ( 2, 2 ),
 ( 4, 2, 2, 2, 2, 2, 2, 2, 2, 2, 2, 2, 2, 2, 2, 2, 2, 2, 2, 2, 2, 2, 2, 2, 2, 2, 2, 2, 2, 2, 2, 2, 2, 2, 2, 2, 2, 2, 2, 2, 2, 2, 2, 2, 2, 2, 2, 2, 2, 2, 2, 2, 2, 2, 2, 2, 2, 2, 2, 2, 2, 2, 2, 2, 2, 2, 2, 2, 2, 2, 2, 2, 2, 2, 2, 2, 2, 2, 2, 2, 2, 2, 2, 2, 2, 2, 2, 2, 2, 2, 2, 2, 2, 2, 2, 2, 2, 2, 2, 2, 2, 2, 2, 2, 2, 2, 2, 2, 2, 2, 2, 4 ),
 ( 0.000000000000000000, 1.000000000000000000 ),
 ( 0.0003185708494972700616, 0.0004481554763622086794, 0.0005777401032271472971, 0.0007073247300920859149, 0.0008369093569570245326, 0.0009017016703894938957, 0.0009664939838219631504, 0.001031286297254432405, 0.001096078610686901768, 0.001225663237551840277, 0.001290455550984309641, 0.001322851707700544322, 0.001355247864416779004, 0.001420040177849248367, 0.001484832491281717730, 0.001614417118146656239, 0.001679209431579125385, 0.001744001745011594749, 0.001808794058444064112, 0.001873586371876533475, 0.001938378685309002621, 0.002003170998741471767, 0.002067963312173941130, 0.002132755625606410493, 0.002197547939038879856, 0.002229944095755114538, 0.002262340252471349220, 0.002391924879336287946, 0.002521509506201226672, 0.002586301819633696035, 0.002651094133066165398, 0.002715886446498634761, 0.002780678759931104124, 0.002910263386796042417, 0.002975055700228511346, 0.003039848013660980709, 0.003104640327093450072, 0.003169432640525919435, 0.003299017267390858162, 0.003428601894255796888, 0.003493394207688266251, 0.003558186521120735614, 0.003622978834553204977, 0.003687771147985673906, 0.003817355774850612199, 0.003946940401715550925, 0.003979336558431785173, 0.004011732715148020288, 0.004076525028580489651, 0.004141317342012959014, 0.004206109655445428377, 0.004270901968877897741, 0.004335694282310367104, 0.004400486595742836467, 0.004465278909175305830, 0.004594863536040244556, 0.004659655849472713919, 0.004724448162905183282, 0.004789240476337652645, 0.004854032789770122008, 0.004918825103202591371, 0.004983617416635060735, 0.005048409730067530098, 0.005113202043499999461, 0.005177994356932468824, 0.005210390513648703939, 0.005242786670364938187, 0.005372371297229876913, 0.005501955924094814772, 0.005566748237527284135, 0.005631540550959752631, 0.005696332864392221994, 0.005761125177824691357, 0.005890709804689630083, 0.005955502118122099446, 0.006020294431554568809, 0.006085086744987038172, 0.006149879058419507535, 0.006214671371851976898, 0.006279463685284446262, 0.006409048312149384988, 0.006473840625581854351, 0.006506236782298089466, 0.006538632939014323714, 0.006603425252446793077, 0.006668217565879262440, 0.006797802192744201166, 0.006862594506176670529, 0.006927386819609139892, 0.006992179133041609256, 0.007056971446474078619, 0.007121763759906547982, 0.007186556073339017345, 0.007251348386771486708, 0.007316140700203956071, 0.007380933013636425434, 0.007445725327068894797, 0.007510517640501363293, 0.007575309953933832656, 0.007704894580798770515, 0.007769686894231239878, 0.007834479207663709241, 0.007866875364379945224, 0.007899271521096179471, 0.007964063834528647967, 0.008093648461393586693, 0.008158440774826056924, 0.008223233088258525419, 0.008288025401690993915, 0.008352817715123464146, 0.008482402341988402872, 0.008611986968853341598 ),
 .UNSPECIFIED. ) ;
#32993=CARTESIAN_POINT ( 'NONE',  ( 6.003228155800906407, 10.22579295840155744, 0.000000000000000000 ) ) ;
#32996=CARTESIAN_POINT ( 'NONE',  ( -4.980641328173854632, 6.904110530993182948, 1.599625672291263179 ) ) ;
#33009=CARTESIAN_POINT ( 'NONE',  ( 3.386504508363381571, 7.172948703057747011, -0.7998128361456362523 ) ) ;
#33011=CARTESIAN_POINT ( 'NONE',  ( 7.289443866002793371, 8.533381260871966134, 1.199719254218452047 ) ) ;
#33018=CARTESIAN_POINT ( 'NONE',  ( -6.577113915960836721, 8.766661883411348555, -1.443375672974066548 ) ) ;
#33024=CARTESIAN_POINT ( 'NONE',  ( 5.528692779322568640, 9.672168352510192690, 0.7998128361456341429 ) ) ;
#33034=CARTESIAN_POINT ( 'NONE',  ( -2.868184766391971952, 6.360316304183658787, -0.2869589966386392743 ) ) ;
#33038=CARTESIAN_POINT ( 'NONE',  ( -6.373741612200205076, 8.529394195690610303, 1.443375672974064550 ) ) ;
#33039=CARTESIAN_POINT ( 'NONE',  ( 5.939880696562888751, 7.062853913145737295, -1.082531754730548412 ) ) ;
#33050=CARTESIAN_POINT ( 'NONE',  ( -4.122561227007127016, 6.967349310553715647, 1.199719254218452935 ) ) ;
#33051=CARTESIAN_POINT ( 'NONE',  ( -7.593975437430151132, 8.032261896522864930, -0.7216878364870338292 ) ) ;
#33052=CARTESIAN_POINT ( 'NONE',  ( 1.833628573703703912, 2.520495649928286674, -2.499561746654547889 ) ) ;
#33056=CARTESIAN_POINT ( 'NONE',  ( 5.411112705185558092, 6.445957923205511086, -1.082531754730548412 ) ) ;
#33061=CARTESIAN_POINT ( 'NONE',  ( -7.065207446497166366, 9.336104335703744539, 0.000000000000000000 ) ) ;
#33070=CARTESIAN_POINT ( 'NONE',  ( -4.320273482414311417, 8.054419775615775379, 0.2990372400716989065 ) ) ;
#33071=CARTESIAN_POINT ( 'NONE',  ( 3.851925040058331806, 5.587274861525073355, -1.443375672974066548 ) ) ;
#33074=CARTESIAN_POINT ( 'NONE',  ( -5.354544322754380303, 5.211666229493680191, 0.7998128361456281477 ) ) ;
#33088=CARTESIAN_POINT ( 'NONE',  ( 6.536439455564150514, 9.679577560583279450, 1.082531754730549078 ) ) ;
#33091=CARTESIAN_POINT ( 'NONE',  ( 6.554440917563797875, 6.611545590104705994, -0.7998128361456481317 ) ) ;
#33124=CARTESIAN_POINT ( 'NONE',  ( 5.126391479742934187, 6.113783160189109722, -1.082531754730548412 ) ) ;
#33129=CARTESIAN_POINT ( 'NONE',  ( 4.465904445180872706, 4.989870290919971474, 0.9171369020453674636 ) ) ;
#33130=CARTESIAN_POINT ( 'NONE',  ( 5.844973620822844218, 6.952128991449046502, 1.082531754730549967 ) ) ;
#33143=CARTESIAN_POINT ( 'NONE',  ( -6.200875153403786477, 8.327716660428123419, -1.599625672291271394 ) ) ;
#33145=CARTESIAN_POINT ( 'NONE',  ( -6.912678218121246942, 9.158153569265168770, 1.599625672291269396 ) ) ;
#33152=CARTESIAN_POINT ( 'NONE',  ( 7.014364370223726830, 9.276787413384745662, -1.599625672291269396 ) ) ;
#33158=CARTESIAN_POINT ( 'NONE',  ( -7.533490631048818109, 8.818102486758951031, -1.199719254218452047 ) ) ;
#33164=CARTESIAN_POINT ( 'NONE',  ( -6.021229618244897885, 7.157760988441397743, 1.082531754730548412 ) ) ;
#33167=CARTESIAN_POINT ( 'NONE',  ( -5.692444392891315097, 7.734547439830227411, -1.599625672291271394 ) ) ;
#33175=CARTESIAN_POINT ( 'NONE',  ( 4.929342268689171469, 7.989555622611471897, -1.003472558803005565 ) ) ;
#33187=CARTESIAN_POINT ( 'NONE',  ( -4.421367491832313590, 6.251624388594711590, 1.443375672974065660 ) ) ;
#33189=CARTESIAN_POINT ( 'NONE',  ( -4.950135482320939140, 4.947781948895412008, -0.7216878364870338292 ) ) ;
#33190=CARTESIAN_POINT ( 'NONE',  ( 3.061108821635398769, 6.793320401875094561, -0.7998128361456362523 ) ) ;
#33191=CARTESIAN_POINT ( 'NONE',  ( -5.631432701629818460, 7.663367133358481631, 1.599625672291263179 ) ) ;
#33209=CARTESIAN_POINT ( 'NONE',  ( 4.068855497876980643, 7.761098824249519801, -0.7216878364870392693 ) ) ;
#33241=CARTESIAN_POINT ( 'NONE',  ( 3.237364818613055473, 6.998952398349030268, -1.734723475976807094E-15 ) ) ;
#33253=CARTESIAN_POINT ( 'NONE',  ( 4.594471896879979589, 8.374412622790375238, -0.01639726577711345112 ) ) ;
#33255=CARTESIAN_POINT ( 'NONE',  ( 3.040771591214902259, 6.769593633051179005, -0.7998128361456362523 ) ) ;
#33261=CARTESIAN_POINT ( 'NONE',  ( -5.692444392891315097, 7.734547439830227411, -1.599625672291271394 ) ) ;
#33266=CARTESIAN_POINT ( 'NONE',  ( -6.522881301506166629, 9.663759714182251770, 1.082531754730549967 ) ) ;
#33273=CARTESIAN_POINT ( 'NONE',  ( 5.180624094197585627, 8.097792972322238825, -1.082531754730548412 ) ) ;
#33276=CARTESIAN_POINT ( 'NONE',  ( -6.283277845290492714, 6.295188672452495915, -0.7998128361456362523 ) ) ;
#33287=CARTESIAN_POINT ( 'NONE',  ( 4.573896719763862251, 6.429575154514868274, -1.599625672291273171 ) ) ;
#33312=( BOUNDED_SURFACE ( )  B_SPLINE_SURFACE ( 1, 2, ( 
 ( #8205, #159793, #176063, #9280, #141465, #58029, #140385, #75352, #207473, #7122, #124193, #111113, #209585, #40732, #205330, #175003, #11396, #125252, #61231, #126314, #191213, #107924, #139301, #190156, #155543, #26589, #25522, #158736, #106838, #43935, #24440, #127386, #89488, #42876, #193359, #60159, #177117, #108984, #92690, #76405, #208523, #56968, #189099, #123141, #116432, #79609, #196566, #197613, #16717, #64432, #82802, #178192, #179260, #160870, #63366, #180318, #94819, #148878, #95894, #98022, #31938, #14592, #30882, #47138, #66519, #12464, #212794, #194426, #165126, #128458, #78539, #210671, #48208, #49257, #195502, #161947, #144656, #213845, #164077, #132662, #451, #32996, #46067, #114320, #81744, #62299, #130576, #145728, #15657, #112188, #211728, #80688, #198667, #96961, #50314, #29809, #13539, #115378, #65463, #147826, #28734, #131614, #181372, #129522, #99073, #113255, #163009, #146779, #38326, #137972, #154214, #51386, #17776, #87073, #70793, #86010, #117507, #20976, #102255, #83864, #153143, #4718, #133733, #149955, #35108, #53507, #101179, #1524, #203991, #167268, #183500, #186697, #118572, #67588, #104402, #185625, #136906, #152084, #119642, #84937, #202933, #54576, #170451, #120724, #168329, #36179, #22036, #37258, #88147, #5786, #199740, #18853, #71863, #151026, #52446, #2595, #55639, #182425, #100125, #34052, #68664, #201861, #166187, #134788, #200795, #184558, #19924, #103328, #3654, #69732, #135836, #169391, #57778, #207220, #159545, #92447, #58843, #91371, #6864, #141209, #126061, #192024, #25269, #56714, #43687, #157431, #77219, #72943, #90289, #205072, #187763, #125000, #105488, #206150, #39393, #7943, #190957, #74033, #122883, #173693, #188841, #107665, #106581, #109804, #172609, #139046, #40477, #175813, #171521, #24185, #42622, #41552, #10085, #174760, #156358, #23114, #140124, #123939, #108732, #27406, #189907, #9024, #75099, #143338, #26333, #158486, #76159, #142264, #208275, #59907, #93504, #155283, #11142, #209332, #121795, #89231, #12216, #194175, #129280, #146532, #211479 ),
 ( #160615, #127134, #28480, #14343, #18335, #60980, #13292, #84415, #34595, #68137, #46890, #95648, #62058, #128213, #134270, #78287, #79365, #151567, #111941, #80432, #150505, #51929, #96716, #118053, #210416, #63115, #193105, #161699, #212549, #44755, #184038, #45820, #130331, #64190, #113003, #195254, #145483, #101733, #110862, #30630, #144414, #200278, #177943, #176868, #94571, #196320, #2065, #179014, #29557, #162765, #100663, #47964, #167803, #35655, #19401, #114080, #180071, #166741, #85481, #187244, #120192, #72415, #69204, #186168, #203469, #123418, #5261, #189381, #152616, #4202, #89780, #188306, #38870, #57257, #106054, #104955, #70270, #155827, #169926, #41024, #20465, #73493, #173157, #107133, #86551, #52978, #122350, #172078, #121269, #136385, #56189, #137454, #119113, #39948, #23670, #168863, #185093, #202402, #88700, #7411, #90839, #54056, #139594, #205617, #71337, #55123, #37802, #103877, #170996, #22594, #135324, #21510, #24738, #3134, #87622, #36720, #154759, #201338, #6343, #102806, #153692, #138516, #204540, #74574, #43164, #8490, #27949, #109277, #11685, #174231, #45280, #91914, #111401, #59381, #142806, #62569, #159021, #128732, #157973, #9563, #29020, #127677, #126599, #210943, #177404, #192562, #75640, #95104, #175286, #194705, #25805, #12740, #112462, #46346, #141747, #206692, #61512, #161152, #60440, #207755, #209873, #76690, #58320, #193637, #78814, #108208, #124477, #125537, #94043, #144938, #30082, #191498, #178472, #156902, #10615, #208809, #26872, #92975, #44217, #110338, #140676, #176341, #190434, #42093, #160082, #77758, #143880, #116709, #15932, #150238, #132936, #98284, #114596, #13812, #196839, #162225, #181638, #48479, #165401, #113533, #198942, #31159, #50586, #96174, #180587, #182710, #66796, #100403, #82015, #130845, #97232, #163285, #166471, #195781, #32210, #183784, #147050, #49521, #34328, #84151, #131884, #1807, #14868, #164343, #79884, #148106, #33266, #145993, #67865, #80957, #16997, #99350, #214109, #65736, #197892, #134012, #212005, #115643, #47418, #18063, #179539 ) ),
 .UNSPECIFIED., .F., .F., .T. ) 
 B_SPLINE_SURFACE_WITH_KNOTS ( ( 2, 2 ),
 ( 3, 2, 2, 2, 2, 2, 2, 2, 2, 2, 2, 2, 2, 2, 2, 2, 2, 2, 2, 2, 2, 2, 2, 2, 2, 2, 2, 2, 2, 2, 2, 2, 2, 2, 2, 2, 2, 2, 2, 2, 2, 2, 2, 2, 2, 2, 2, 2, 2, 2, 2, 2, 2, 2, 2, 2, 2, 2, 2, 2, 2, 2, 2, 2, 2, 2, 2, 2, 2, 2, 2, 2, 2, 2, 2, 2, 2, 2, 2, 2, 2, 2, 2, 2, 2, 2, 2, 2, 2, 2, 2, 2, 2, 2, 2, 2, 2, 2, 2, 2, 2, 2, 2, 2, 2, 2, 2, 2, 2, 2, 2, 2, 2, 2, 2, 2, 2, 2, 2, 2, 3 ),
 ( 0.000000000000000000, 1.000000000000000000 ),
 ( 0.000000000000000000, 0.008333333333333333218, 0.01666666666666666644, 0.02500000000000000139, 0.03333333333333333287, 0.04166666666666666435, 0.05000000000000000278, 0.05833333333333333426, 0.06666666666666666574, 0.07499999999999999722, 0.08333333333333332871, 0.09166666666666666019, 0.1000000000000000056, 0.1083333333333333370, 0.1166666666666666685, 0.1250000000000000000, 0.1333333333333333315, 0.1416666666666666630, 0.1499999999999999944, 0.1583333333333333259, 0.1666666666666666574, 0.1749999999999999889, 0.1833333333333333204, 0.1916666666666666796, 0.2000000000000000111, 0.2083333333333333426, 0.2166666666666666741, 0.2250000000000000056, 0.2333333333333333370, 0.2416666666666666685, 0.2500000000000000000, 0.2583333333333333592, 0.2666666666666666630, 0.2750000000000000222, 0.2833333333333333259, 0.2916666666666666852, 0.2999999999999999889, 0.3083333333333333481, 0.3166666666666666519, 0.3250000000000000111, 0.3333333333333333148, 0.3416666666666666741, 0.3499999999999999778, 0.3583333333333333370, 0.3666666666666666408, 0.3750000000000000000, 0.3833333333333333592, 0.3916666666666666630, 0.4000000000000000222, 0.4083333333333333259, 0.4166666666666666852, 0.4249999999999999889, 0.4333333333333333481, 0.4416666666666666519, 0.4500000000000000111, 0.4583333333333333148, 0.4666666666666666741, 0.4749999999999999778, 0.4833333333333333370, 0.4916666666666666408, 0.5000000000000000000, 0.5083333333333333037, 0.5166666666666667185, 0.5250000000000000222, 0.5333333333333333259, 0.5416666666666666297, 0.5500000000000000444, 0.5583333333333333481, 0.5666666666666666519, 0.5749999999999999556, 0.5833333333333333703, 0.5916666666666666741, 0.5999999999999999778, 0.6083333333333332815, 0.6166666666666666963, 0.6250000000000000000, 0.6333333333333333037, 0.6416666666666667185, 0.6500000000000000222, 0.6583333333333333259, 0.6666666666666666297, 0.6750000000000000444, 0.6833333333333333481, 0.6916666666666666519, 0.6999999999999999556, 0.7083333333333333703, 0.7166666666666666741, 0.7249999999999999778, 0.7333333333333332815, 0.7416666666666666963, 0.7500000000000000000, 0.7583333333333333037, 0.7666666666666667185, 0.7750000000000000222, 0.7833333333333333259, 0.7916666666666666297, 0.8000000000000000444, 0.8083333333333333481, 0.8166666666666666519, 0.8249999999999999556, 0.8333333333333333703, 0.8416666666666666741, 0.8499999999999999778, 0.8583333333333332815, 0.8666666666666666963, 0.8750000000000000000, 0.8833333333333333037, 0.8916666666666667185, 0.9000000000000000222, 0.9083333333333333259, 0.9166666666666666297, 0.9250000000000000444, 0.9333333333333333481, 0.9416666666666666519, 0.9499999999999999556, 0.9583333333333333703, 0.9666666666666666741, 0.9749999999999999778, 0.9833333333333332815, 0.9916666666666666963, 1.000000000000000000 ),
 .UNSPECIFIED. ) 
 GEOMETRIC_REPRESENTATION_ITEM ( )  RATIONAL_B_SPLINE_SURFACE ( (
 ( 1.000000000000000000, 0.8660254037844387076, 1.000000000000000000, 0.8660254037844387076, 1.000000000000000000, 0.8660254037844387076, 1.000000000000000000, 0.8660254037844387076, 1.000000000000000000, 0.8660254037844387076, 1.000000000000000000, 0.8660254037844387076, 1.000000000000000000, 0.8660254037844387076, 1.000000000000000000, 0.8660254037844387076, 1.000000000000000000, 0.8660254037844387076, 1.000000000000000000, 0.8660254037844387076, 1.000000000000000000, 0.8660254037844387076, 1.000000000000000000, 0.8660254037844387076, 1.000000000000000000, 0.8660254037844387076, 1.000000000000000000, 0.8660254037844387076, 1.000000000000000000, 0.8660254037844387076, 1.000000000000000000, 0.8660254037844387076, 1.000000000000000000, 0.8660254037844387076, 1.000000000000000000, 0.8660254037844387076, 1.000000000000000000, 0.8660254037844387076, 1.000000000000000000, 0.8660254037844387076, 1.000000000000000000, 0.8660254037844387076, 1.000000000000000000, 0.8660254037844387076, 1.000000000000000000, 0.8660254037844387076, 1.000000000000000000, 0.8660254037844387076, 1.000000000000000000, 0.8660254037844387076, 1.000000000000000000, 0.8660254037844387076, 1.000000000000000000, 0.8660254037844387076, 1.000000000000000000, 0.8660254037844387076, 1.000000000000000000, 0.8660254037844387076, 1.000000000000000000, 0.8660254037844387076, 1.000000000000000000, 0.8660254037844387076, 1.000000000000000000, 0.8660254037844387076, 1.000000000000000000, 0.8660254037844387076, 1.000000000000000000, 0.8660254037844387076, 1.000000000000000000, 0.8660254037844387076, 1.000000000000000000, 0.8660254037844387076, 1.000000000000000000, 0.8660254037844387076, 1.000000000000000000, 0.8660254037844387076, 1.000000000000000000, 0.8660254037844387076, 1.000000000000000000, 0.8660254037844387076, 1.000000000000000000, 0.8660254037844387076, 1.000000000000000000, 0.8660254037844387076, 1.000000000000000000, 0.8660254037844387076, 1.000000000000000000, 0.8660254037844387076, 1.000000000000000000, 0.8660254037844387076, 1.000000000000000000, 0.8660254037844387076, 1.000000000000000000, 0.8660254037844387076, 1.000000000000000000, 0.8660254037844387076, 1.000000000000000000, 0.8660254037844387076, 1.000000000000000000, 0.8660254037844387076, 1.000000000000000000, 0.8660254037844387076, 1.000000000000000000, 0.8660254037844387076, 1.000000000000000000, 0.8660254037844387076, 1.000000000000000000, 0.8660254037844387076, 1.000000000000000000, 0.8660254037844387076, 1.000000000000000000, 0.8660254037844387076, 1.000000000000000000, 0.8660254037844387076, 1.000000000000000000, 0.8660254037844387076, 1.000000000000000000, 0.8660254037844387076, 1.000000000000000000, 0.8660254037844387076, 1.000000000000000000, 0.8660254037844387076, 1.000000000000000000, 0.8660254037844387076, 1.000000000000000000, 0.8660254037844387076, 1.000000000000000000, 0.8660254037844387076, 1.000000000000000000, 0.8660254037844387076, 1.000000000000000000, 0.8660254037844387076, 1.000000000000000000, 0.8660254037844387076, 1.000000000000000000, 0.8660254037844387076, 1.000000000000000000, 0.8660254037844387076, 1.000000000000000000, 0.8660254037844387076, 1.000000000000000000, 0.8660254037844387076, 1.000000000000000000, 0.8660254037844387076, 1.000000000000000000, 0.8660254037844387076, 1.000000000000000000, 0.8660254037844387076, 1.000000000000000000, 0.8660254037844387076, 1.000000000000000000, 0.8660254037844387076, 1.000000000000000000, 0.8660254037844387076, 1.000000000000000000, 0.8660254037844387076, 1.000000000000000000, 0.8660254037844387076, 1.000000000000000000, 0.8660254037844387076, 1.000000000000000000, 0.8660254037844387076, 1.000000000000000000, 0.8660254037844387076, 1.000000000000000000, 0.8660254037844387076, 1.000000000000000000, 0.8660254037844387076, 1.000000000000000000, 0.8660254037844387076, 1.000000000000000000, 0.8660254037844387076, 1.000000000000000000, 0.8660254037844387076, 1.000000000000000000, 0.8660254037844387076, 1.000000000000000000, 0.8660254037844387076, 1.000000000000000000, 0.8660254037844387076, 1.000000000000000000, 0.8660254037844387076, 1.000000000000000000, 0.8660254037844387076, 1.000000000000000000, 0.8660254037844387076, 1.000000000000000000, 0.8660254037844387076, 1.000000000000000000, 0.8660254037844387076, 1.000000000000000000, 0.8660254037844387076, 1.000000000000000000, 0.8660254037844387076, 1.000000000000000000, 0.8660254037844387076, 1.000000000000000000, 0.8660254037844387076, 1.000000000000000000, 0.8660254037844387076, 1.000000000000000000, 0.8660254037844387076, 1.000000000000000000, 0.8660254037844387076, 1.000000000000000000, 0.8660254037844387076, 1.000000000000000000, 0.8660254037844387076, 1.000000000000000000, 0.8660254037844387076, 1.000000000000000000, 0.8660254037844387076, 1.000000000000000000, 0.8660254037844387076, 1.000000000000000000, 0.8660254037844387076, 1.000000000000000000, 0.8660254037844387076, 1.000000000000000000, 0.8660254037844387076, 1.000000000000000000, 0.8660254037844387076, 1.000000000000000000, 0.8660254037844387076, 1.000000000000000000, 0.8660254037844387076, 1.000000000000000000, 0.8660254037844387076, 1.000000000000000000, 0.8660254037844387076, 1.000000000000000000, 0.8660254037844387076, 1.000000000000000000, 0.8660254037844387076, 1.000000000000000000, 0.8660254037844387076, 1.000000000000000000, 0.8660254037844387076, 1.000000000000000000, 0.8660254037844387076, 1.000000000000000000),
 ( 1.000000000000000000, 0.8660254037844387076, 1.000000000000000000, 0.8660254037844387076, 1.000000000000000000, 0.8660254037844387076, 1.000000000000000000, 0.8660254037844387076, 1.000000000000000000, 0.8660254037844387076, 1.000000000000000000, 0.8660254037844387076, 1.000000000000000000, 0.8660254037844387076, 1.000000000000000000, 0.8660254037844387076, 1.000000000000000000, 0.8660254037844387076, 1.000000000000000000, 0.8660254037844387076, 1.000000000000000000, 0.8660254037844387076, 1.000000000000000000, 0.8660254037844387076, 1.000000000000000000, 0.8660254037844387076, 1.000000000000000000, 0.8660254037844387076, 1.000000000000000000, 0.8660254037844387076, 1.000000000000000000, 0.8660254037844387076, 1.000000000000000000, 0.8660254037844387076, 1.000000000000000000, 0.8660254037844387076, 1.000000000000000000, 0.8660254037844387076, 1.000000000000000000, 0.8660254037844387076, 1.000000000000000000, 0.8660254037844387076, 1.000000000000000000, 0.8660254037844387076, 1.000000000000000000, 0.8660254037844387076, 1.000000000000000000, 0.8660254037844387076, 1.000000000000000000, 0.8660254037844387076, 1.000000000000000000, 0.8660254037844387076, 1.000000000000000000, 0.8660254037844387076, 1.000000000000000000, 0.8660254037844387076, 1.000000000000000000, 0.8660254037844387076, 1.000000000000000000, 0.8660254037844387076, 1.000000000000000000, 0.8660254037844387076, 1.000000000000000000, 0.8660254037844387076, 1.000000000000000000, 0.8660254037844387076, 1.000000000000000000, 0.8660254037844387076, 1.000000000000000000, 0.8660254037844387076, 1.000000000000000000, 0.8660254037844387076, 1.000000000000000000, 0.8660254037844387076, 1.000000000000000000, 0.8660254037844387076, 1.000000000000000000, 0.8660254037844387076, 1.000000000000000000, 0.8660254037844387076, 1.000000000000000000, 0.8660254037844387076, 1.000000000000000000, 0.8660254037844387076, 1.000000000000000000, 0.8660254037844387076, 1.000000000000000000, 0.8660254037844387076, 1.000000000000000000, 0.8660254037844387076, 1.000000000000000000, 0.8660254037844387076, 1.000000000000000000, 0.8660254037844387076, 1.000000000000000000, 0.8660254037844387076, 1.000000000000000000, 0.8660254037844387076, 1.000000000000000000, 0.8660254037844387076, 1.000000000000000000, 0.8660254037844387076, 1.000000000000000000, 0.8660254037844387076, 1.000000000000000000, 0.8660254037844387076, 1.000000000000000000, 0.8660254037844387076, 1.000000000000000000, 0.8660254037844387076, 1.000000000000000000, 0.8660254037844387076, 1.000000000000000000, 0.8660254037844387076, 1.000000000000000000, 0.8660254037844387076, 1.000000000000000000, 0.8660254037844387076, 1.000000000000000000, 0.8660254037844387076, 1.000000000000000000, 0.8660254037844387076, 1.000000000000000000, 0.8660254037844387076, 1.000000000000000000, 0.8660254037844387076, 1.000000000000000000, 0.8660254037844387076, 1.000000000000000000, 0.8660254037844387076, 1.000000000000000000, 0.8660254037844387076, 1.000000000000000000, 0.8660254037844387076, 1.000000000000000000, 0.8660254037844387076, 1.000000000000000000, 0.8660254037844387076, 1.000000000000000000, 0.8660254037844387076, 1.000000000000000000, 0.8660254037844387076, 1.000000000000000000, 0.8660254037844387076, 1.000000000000000000, 0.8660254037844387076, 1.000000000000000000, 0.8660254037844387076, 1.000000000000000000, 0.8660254037844387076, 1.000000000000000000, 0.8660254037844387076, 1.000000000000000000, 0.8660254037844387076, 1.000000000000000000, 0.8660254037844387076, 1.000000000000000000, 0.8660254037844387076, 1.000000000000000000, 0.8660254037844387076, 1.000000000000000000, 0.8660254037844387076, 1.000000000000000000, 0.8660254037844387076, 1.000000000000000000, 0.8660254037844387076, 1.000000000000000000, 0.8660254037844387076, 1.000000000000000000, 0.8660254037844387076, 1.000000000000000000, 0.8660254037844387076, 1.000000000000000000, 0.8660254037844387076, 1.000000000000000000, 0.8660254037844387076, 1.000000000000000000, 0.8660254037844387076, 1.000000000000000000, 0.8660254037844387076, 1.000000000000000000, 0.8660254037844387076, 1.000000000000000000, 0.8660254037844387076, 1.000000000000000000, 0.8660254037844387076, 1.000000000000000000, 0.8660254037844387076, 1.000000000000000000, 0.8660254037844387076, 1.000000000000000000, 0.8660254037844387076, 1.000000000000000000, 0.8660254037844387076, 1.000000000000000000, 0.8660254037844387076, 1.000000000000000000, 0.8660254037844387076, 1.000000000000000000, 0.8660254037844387076, 1.000000000000000000, 0.8660254037844387076, 1.000000000000000000, 0.8660254037844387076, 1.000000000000000000, 0.8660254037844387076, 1.000000000000000000, 0.8660254037844387076, 1.000000000000000000, 0.8660254037844387076, 1.000000000000000000, 0.8660254037844387076, 1.000000000000000000, 0.8660254037844387076, 1.000000000000000000, 0.8660254037844387076, 1.000000000000000000, 0.8660254037844387076, 1.000000000000000000, 0.8660254037844387076, 1.000000000000000000, 0.8660254037844387076, 1.000000000000000000, 0.8660254037844387076, 1.000000000000000000, 0.8660254037844387076, 1.000000000000000000, 0.8660254037844387076, 1.000000000000000000, 0.8660254037844387076, 1.000000000000000000, 0.8660254037844387076, 1.000000000000000000, 0.8660254037844387076, 1.000000000000000000, 0.8660254037844387076, 1.000000000000000000, 0.8660254037844387076, 1.000000000000000000, 0.8660254037844387076, 1.000000000000000000) ) ) 
 REPRESENTATION_ITEM ( '' )  SURFACE ( )  );
#33320=CARTESIAN_POINT ( 'NONE',  ( 5.936491157937257235, 8.019268665717216749, 1.599625672291268286 ) ) ;
#33326=CARTESIAN_POINT ( 'NONE',  ( 4.204437034013637664, 6.958908068774287692, -1.082531754730548412 ) ) ;
#33329=CARTESIAN_POINT ( 'NONE',  ( 7.078765600110826561, 8.391552967285011988, -1.082531754730548412 ) ) ;
#33338=CARTESIAN_POINT ( 'NONE',  ( 4.207966135563082410, 7.175396087857926375, -2.420000000000000373 ) ) ;
#33341=CARTESIAN_POINT ( 'NONE',  ( -5.628043163448566588, 9.580151100749725757, 0.000000000000000000 ) ) ;
#33366=CARTESIAN_POINT ( 'NONE',  ( -3.960390268523300339, 7.634556056670224855, 1.214306433183764966E-14 ) ) ;
#33376=CARTESIAN_POINT ( 'NONE',  ( 4.692003678781083487, 7.631698837623355658, -1.199719254218450271 ) ) ;
#33378=CARTESIAN_POINT ( 'NONE',  ( 4.864343252252968597, 8.897093904262280972, 0.000000000000000000 ) ) ;
#33386=( NAMED_UNIT ( * ) SI_UNIT ( $, .STERADIAN. ) SOLID_ANGLE_UNIT ( ) );
#33393=CARTESIAN_POINT ( 'NONE',  ( -4.930325137224961907, 5.781076077297750970, -1.199719254218453823 ) ) ;
#33396=CARTESIAN_POINT ( 'NONE',  ( 5.194182247366869731, 7.153241603385088965, 1.443375672974064550 ) ) ;
#33404=CARTESIAN_POINT ( 'NONE',  ( -3.149236820124241110, 6.896136400112061970, -0.7998128361456481317 ) ) ;
#33411=CARTESIAN_POINT ( 'NONE',  ( -6.672020991700860826, 7.917017590806697314, 1.082531754730549078 ) ) ;
#33413=CARTESIAN_POINT ( 'NONE',  ( -4.665414256878301025, 6.536345614481700927, -1.443375672974066548 ) ) ;
#33430=CARTESIAN_POINT ( 'NONE',  ( -5.334207092333882017, 5.187939460669764635, 0.7998128361456281477 ) ) ;
#33431=ORIENTED_EDGE ( 'NONE', *, *, #105631, .T. ) ;
#33441=CARTESIAN_POINT ( 'NONE',  ( -4.359828915246279024, 7.244161613499399799, -1.199719254218455378 ) ) ;
#33450=CARTESIAN_POINT ( 'NONE',  ( 3.627755783104286813, 3.517448670773187125, -2.500000000000000444 ) ) ;
#33451=CARTESIAN_POINT ( 'NONE',  ( -5.203215198707511036, 7.836405505866204102, -1.276579466623083858 ) ) ;
#33468=EDGE_CURVE ( 'NONE', #180652, #213748, #140991, .T. ) ;
#33470=CARTESIAN_POINT ( 'NONE',  ( 7.198453214212898743, 7.362893269528701268, 0.7998128361456291469 ) ) ;
#33476=DIRECTION ( 'NONE',  ( 2.439454888092378666E-14, 0.000000000000000000, 1.000000000000000000 ) ) ;
#33495=CARTESIAN_POINT ( 'NONE',  ( 7.126746022638799971, 8.343567110280638133, 1.199719254218452047 ) ) ;
#33496=CARTESIAN_POINT ( 'NONE',  ( 4.929271367020211514, 7.908511140569038922, 1.199719254218452047 ) ) ;
#33498=CARTESIAN_POINT ( 'NONE',  ( 6.215487077222150880, 6.216099443039444949, 0.000000000000000000 ) ) ;
#33502=CARTESIAN_POINT ( 'NONE',  ( 0.000000000000000000, 0.000000000000000000, 0.000000000000000000 ) ) ;
#33510=CARTESIAN_POINT ( 'NONE',  ( 5.504185490526544378, 7.460110003252303557, -1.249659907641489820 ) ) ;
#33511=CARTESIAN_POINT ( 'NONE',  ( -6.251718229232867685, 6.466295153626015590, -0.7216878364870338292 ) ) ;
#33512=CARTESIAN_POINT ( 'NONE',  ( 5.411112705629925301, 5.485588709422586362, 0.000000000000000000 ) ) ;
#33536=CARTESIAN_POINT ( 'NONE',  ( 5.662465432362883355, 6.635239754958710989, 1.199719254218451159 ) ) ;
#33538=CARTESIAN_POINT ( 'NONE',  ( 4.923546060418115822, 5.773167154356443120, -1.199719254218452047 ) ) ;
#33562=CARTESIAN_POINT ( 'NONE',  ( 0.1216811705908975721, 2.536982183874236352, -1.996294991408742003 ) ) ;
#33566=CARTESIAN_POINT ( 'NONE',  ( 6.530187263637528439, 7.647581891445782709, -1.199719254218452047 ) ) ;
#33570=CARTESIAN_POINT ( 'NONE',  ( -5.984664909832329904, 7.106694798503815136, 1.079546468792412783 ) ) ;
#33571=CARTESIAN_POINT ( 'NONE',  ( 5.027041095616958444, 9.086908054853605421, 0.000000000000000000 ) ) ;
#33579=CARTESIAN_POINT ( 'NONE',  ( -1.843739406749240750, 8.923774302061360686, 0.7750000000000013545 ) ) ;
#33580=CARTESIAN_POINT ( 'NONE',  ( 4.607663176575717223, 8.357619647684677133, 0.2284409323990380658 ) ) ;
#33605=CARTESIAN_POINT ( 'NONE',  ( -7.065734331377342414, 8.272386803808890576, -1.199719254218452047 ) ) ;
#33607=CARTESIAN_POINT ( 'NONE',  ( 5.338878628731272613, 9.450718510153643948, -0.7998128361456481317 ) ) ;
#33609=CARTESIAN_POINT ( 'NONE',  ( 3.757017964762656703, 7.397288368949487491, -1.734723475976807094E-15 ) ) ;
#33620=CARTESIAN_POINT ( 'NONE',  ( -6.041797769283476782, 7.151762567314746022, -1.181783516275588752 ) ) ;
#33635=CARTESIAN_POINT ( 'NONE',  ( 6.699137298928153683, 7.948653282571920720, 1.082531754730549967 ) ) ;
#33647=CARTESIAN_POINT ( 'NONE',  ( -3.336715202739028552, 6.906935146588564223, 0.7216878364870338292 ) ) ;
#33649=CARTESIAN_POINT ( 'NONE',  ( 4.525389411911321602, 8.501647757197021704, -0.7998128361456381397 ) ) ;
#33652=CARTESIAN_POINT ( 'NONE',  ( -6.084577077482911101, 10.32070003369722144, 0.000000000000000000 ) ) ;
#33654=CARTESIAN_POINT ( 'NONE',  ( -4.411198876399886615, 6.239761003923544713, -1.599625672291271394 ) ) ;
#33667=EDGE_CURVE ( 'NONE', #90832, #169159, #179693, .T. ) ;
#33700=CARTESIAN_POINT ( 'NONE',  ( 4.903208829997618423, 5.749440385532527564, -1.199719254218450271 ) ) ;
#33706=CARTESIAN_POINT ( 'NONE',  ( -6.414416072596857532, 6.656109304217339151, -0.7216878364870338292 ) ) ;
#33712=CARTESIAN_POINT ( 'NONE',  ( -7.598418745816086783, 7.829519723065708092, 0.000000000000000000 ) ) ;
#33719=DIRECTION ( 'NONE',  ( 0.7978120914393174168, 0.6029061840396252592, -6.536721945407052908E-15 ) ) ;
#33720=CARTESIAN_POINT ( 'NONE',  ( -4.606738333593328072, 8.596554832492683929, 0.7998128361456281477 ) ) ;
#33722=ORIENTED_EDGE ( 'NONE', *, *, #93445, .F. ) ;
#33723=CARTESIAN_POINT ( 'NONE',  ( 4.595841027163160675, 8.489102040997540399, 0.04885061651019838302 ) ) ;
#33728=CARTESIAN_POINT ( 'NONE',  ( 7.180978637093494044, 8.406838493811077839, -1.199719254218452047 ) ) ;
#33735=CARTESIAN_POINT ( 'NONE',  ( -5.991777542596674166, 5.955104985976372944, 0.000000000000000000 ) ) ;
#33739=CARTESIAN_POINT ( 'NONE',  ( -6.774234028683526532, 7.932303117332766718, 1.199719254218452047 ) ) ;
#33742=CARTESIAN_POINT ( 'NONE',  ( 0.000000000000000000, 8.920000000000001705, 0.000000000000000000 ) ) ;
#33744=CARTESIAN_POINT ( 'NONE',  ( 4.868786560638878491, 8.694351730805124134, 0.7216878364870317197 ) ) ;
#33746=CARTESIAN_POINT ( 'NONE',  ( -6.414416072596837104, 9.537216947121368804, -1.082531754730549967 ) ) ;
#33753=CARTESIAN_POINT ( 'NONE',  ( 5.006703865196457492, 9.063181286029688977, 0.000000000000000000 ) ) ;
#33762=CARTESIAN_POINT ( 'NONE',  ( -4.505605203626008581, 6.920276886661140381, 1.305342265584524375 ) ) ;
#33763=CARTESIAN_POINT ( 'NONE',  ( 4.529832720297257254, 8.298905583739861314, 0.000000000000000000 ) ) ;
#33768=CARTESIAN_POINT ( 'NONE',  ( 6.463557619869761517, 6.860074278669063830, -0.6545079704341187909 ) ) ;
#33778=CARTESIAN_POINT ( 'NONE',  ( 1.806654366501771136, 2.518449987798942136, 2.499999999999998668 ) ) ;
#33796=CARTESIAN_POINT ( 'NONE',  ( -5.811016664379555330, 7.234075022110222797, -1.179019473189359068 ) ) ;
#33810=DIRECTION ( 'NONE',  ( 0.000000000000000000, 0.000000000000000000, -1.000000000000000000 ) ) ;
#33813=B_SPLINE_CURVE_WITH_KNOTS ( 'NONE', 3,
 ( #11858, #73670, #77936, #172253, #127860, #23840, #25977, #92083, #158140, #207926 ),
 .UNSPECIFIED., .F., .F.,
 ( 4, 3, 3, 4 ),
 ( 4.665953388357896293E-15, 8.735091161667903135E-05, 0.0001705277764939987001, 0.0002537626642914739207 ),
 .UNSPECIFIED. ) ;
#33815=CARTESIAN_POINT ( 'NONE',  ( -4.793689830883590020, 7.750332681742931662, 1.199719254218452935 ) ) ;
#33817=CARTESIAN_POINT ( 'NONE',  ( 7.095713291905693332, 9.371694488680407886, 1.599625672291268286 ) ) ;
#33819=CARTESIAN_POINT ( 'NONE',  ( 4.327421600515347855, 8.660439283198849481, -0.7750000000000001332 ) ) ;
#33829=CARTESIAN_POINT ( 'NONE',  ( 5.885121196783658526, 9.023669275293071834, 1.199719254218452047 ) ) ;
#33831=CARTESIAN_POINT ( 'NONE',  ( 6.007671464186823407, 9.062681570643055906, 1.082531754730549967 ) ) ;
#33834=VECTOR ( 'NONE', #121567, 1000.000000000000000 ) ;
#33844=CARTESIAN_POINT ( 'NONE',  ( -5.971440312176176768, 5.931378217152456500, 0.000000000000000000 ) ) ;
#33845=CARTESIAN_POINT ( 'NONE',  ( 5.065906673361608270, 5.939254536123854677, -1.199719254218450271 ) ) ;
#33854=CARTESIAN_POINT ( 'NONE',  ( -7.425025402139490360, 8.691559719698066289, 1.199719254218452047 ) ) ;
#33855=CARTESIAN_POINT ( 'NONE',  ( 7.693325821111733021, 7.940244644243982464, -0.7998128361456341429 ) ) ;
#33863=CARTESIAN_POINT ( 'NONE',  ( 3.932747076415766596, 6.745899468197171345, 1.199719254218451159 ) ) ;
#33870=CARTESIAN_POINT ( 'NONE',  ( -6.480235040494578769, 6.771487114559836762, -0.2501488059577141598 ) ) ;
#33875=AXIS2_PLACEMENT_3D ( 'NONE', #39104, #207982, #139825 ) ;
#33880=CARTESIAN_POINT ( 'NONE',  ( -7.957709816578236506, 8.248692638954882028, 0.7998128361456341429 ) ) ;
#33895=ORIENTED_EDGE ( 'NONE', *, *, #131734, .T. ) ;
#33908=EDGE_CURVE ( 'NONE', #67360, #94475, #40040, .T. ) ;
#33911=CARTESIAN_POINT ( 'NONE',  ( 4.064412189046650248, 7.963840997188265547, 0.7998128361456271485 ) ) ;
#33932=CARTESIAN_POINT ( 'NONE',  ( 5.903649544107831382, 5.852288987739402870, -0.7998128361456481317 ) ) ;
#33935=CARTESIAN_POINT ( 'NONE',  ( -4.340018570150322219, 5.196348098997705556, -1.082531754730551743 ) ) ;
#33948=EDGE_CURVE ( 'NONE', #160372, #70814, #89409, .T. ) ;
#33951=CARTESIAN_POINT ( 'NONE',  ( 4.858757509019037357, 5.629766575900002401, 2.499999999999999556 ) ) ;
#33960=CARTESIAN_POINT ( 'NONE',  ( -7.228432174741334038, 8.462200954400218578, -1.199719254218452047 ) ) ;
#33970=CARTESIAN_POINT ( 'NONE',  ( -5.570361349191150779, 5.866663122702686195, 0.5491554309224304653 ) ) ;
#33975=CARTESIAN_POINT ( 'NONE',  ( -7.747558435566414659, 8.003516027774422170, -0.7998128361456362523 ) ) ;
#33987=CARTESIAN_POINT ( 'NONE',  ( -4.586401103172829785, 8.572828063668767484, 0.7998128361456281477 ) ) ;
#33990=CARTESIAN_POINT ( 'NONE',  ( -6.780486220610186798, 8.043560357867583832, -1.082531754730549967 ) ) ;
#33994=CARTESIAN_POINT ( 'NONE',  ( 6.016786309414542622, 10.24161080428416426, 0.7998128361456341429 ) ) ;
#33995=CARTESIAN_POINT ( 'NONE',  ( -3.309598895067336510, 6.875299454304925284, 0.000000000000000000 ) ) ;
#34003=ORIENTED_EDGE ( 'NONE', *, *, #106606, .T. ) ;
#34009=CARTESIAN_POINT ( 'NONE',  ( -0.3380487832185405384, 2.650106715013329950, 1.972192952016705636 ) ) ;
#34014=CARTESIAN_POINT ( 'NONE',  ( 6.304162555737000240, 6.968127521147626346, -0.9177210060461529206 ) ) ;
#34036=CARTESIAN_POINT ( 'NONE',  ( 6.011645680221167076, 7.072102904328817274, -1.053258377668888857 ) ) ;
#34052=CARTESIAN_POINT ( 'NONE',  ( -6.038177310039794854, 8.137902509836795417, -1.599625672291271394 ) ) ;
#34066=CARTESIAN_POINT ( 'NONE',  ( 3.725458348705031231, 7.568394850123006279, -1.734723475976807094E-15 ) ) ;
#34068=CARTESIAN_POINT ( 'NONE',  ( 6.855582950365507244, 8.027210192628430718, -1.199719254218452047 ) ) ;
#34075=CARTESIAN_POINT ( 'NONE',  ( -7.553300976144794454, 7.984808358356614733, -0.7216878364870338292 ) ) ;
#34081=CARTESIAN_POINT ( 'NONE',  ( 4.882344714252594642, 4.868692719482363707, 0.000000000000000000 ) ) ;
#34095=CARTESIAN_POINT ( 'NONE',  ( -6.509323148336870091, 7.727203440215372865, 1.082531754730549078 ) ) ;
#34096=CARTESIAN_POINT ( 'NONE',  ( 6.061904079085887354, 6.244845311787889486, 0.000000000000000000 ) ) ;
#34098=DIRECTION ( 'NONE',  ( -1.000000000000000000, -0.000000000000000000, -2.168404344971003504E-14 ) ) ;
#34102=CARTESIAN_POINT ( 'NONE',  ( 4.353576723319602770, 8.093273587265924718, -0.7216878364870386031 ) ) ;
#34105=CARTESIAN_POINT ( 'NONE',  ( -3.284818356260900796, 7.054314858938165678, 0.7998128361456352531 ) ) ;
#34106=CARTESIAN_POINT ( 'NONE',  ( -5.804299160426229953, 8.825413882922319431, -1.082531754730549967 ) ) ;
#34107=CARTESIAN_POINT ( 'NONE',  ( 6.556249800660121529, 9.806652646482286073, 1.199719254218452047 ) ) ;
#34110=CARTESIAN_POINT ( 'NONE',  ( 5.872089928050205465, 6.023395468912922546, -0.7216878364870458196 ) ) ;
#34112=EDGE_LOOP ( 'NONE', ( #54891, #14267, #203242, #137159, #153887, #182733, #201335, #50629, #122930, #129270, #193938, #152659, #206365, #100989, #191491, #83168, #90606, #160927, #184296, #196475, #98774 ) ) ;
#34125=CARTESIAN_POINT ( 'NONE',  ( -0.02069724287496089998, 3.480000000000000426, -2.000000000000000000 ) ) ;
#34130=CARTESIAN_POINT ( 'NONE',  ( -6.493429226302317225, 6.540365283632955773, 0.7998128361456341429 ) ) ;
#34142=CARTESIAN_POINT ( 'NONE',  ( 4.848976215542928792, 5.686169002002086970, 1.199719254218452047 ) ) ;
#34177=CARTESIAN_POINT ( 'NONE',  ( 6.712695452541852070, 7.004101914153185504, 0.000000000000000000 ) ) ;
#34182=CARTESIAN_POINT ( 'NONE',  ( 6.170369307550815030, 8.292126506933040986, 1.443375672974064550 ) ) ;
#34196=CARTESIAN_POINT ( 'NONE',  ( -5.824109505522200081, 8.952488968821326054, -1.199719254218452047 ) ) ;
#34208=CARTESIAN_POINT ( 'NONE',  ( 5.515134625708930649, 9.656350506627580543, 0.000000000000000000 ) ) ;
#34214=CARTESIAN_POINT ( 'NONE',  ( -7.099629715411508890, 8.311931418515415615, 1.199719254218452047 ) ) ;
#34220=CARTESIAN_POINT ( 'NONE',  ( -5.153507786970267013, 8.066157280557016307, -1.082531754730549967 ) ) ;
#34224=CARTESIAN_POINT ( 'NONE',  ( -5.152980901645737077, 8.169505597632108262, -1.199719254218453823 ) ) ;
#34245=CARTESIAN_POINT ( 'NONE',  ( -4.502716413514313842, 5.386162249589033557, -1.082531754730549967 ) ) ;
#34248=CARTESIAN_POINT ( 'NONE',  ( -4.963693635934603776, 4.963599794778024155, 0.000000000000000000 ) ) ;
#34249=CARTESIAN_POINT ( 'NONE',  ( -4.782994330570982555, 8.802186828966616972, 0.000000000000000000 ) ) ;
#34251=EDGE_CURVE ( 'NONE', #7055, #26620, #51361, .T. ) ;
#34262=VERTEX_POINT ( 'NONE', #158204 ) ;
#34269=CIRCLE ( 'NONE', #155339, 0.08000000000000041800 ) ;
#34270=CARTESIAN_POINT ( 'NONE',  ( -4.450808633097269151, 7.987047222781179734, -2.500000000000000444 ) ) ;
#34302=CARTESIAN_POINT ( 'NONE',  ( 4.706615602599436343, 5.520081620234675412, 1.199719254218452935 ) ) ;
#34313=CARTESIAN_POINT ( 'NONE',  ( 4.651083699394226834, 8.303454393088664176, 0.4639335724816190942 ) ) ;
#34315=CARTESIAN_POINT ( 'NONE',  ( 3.607351389687783794, 6.366271167014519783, 1.199719254218451159 ) ) ;
#34322=CARTESIAN_POINT ( 'NONE',  ( -4.450819567036169211, 8.414649604842665553, -0.7998128361456362523 ) ) ;
#34328=CARTESIAN_POINT ( 'NONE',  ( -6.414416072596837104, 9.537216947121368804, -1.082531754730549967 ) ) ;
#34330=CARTESIAN_POINT ( 'NONE',  ( -6.287978406667054543, 6.558588919770907744, 0.3271801204444577671 ) ) ;
#34335=CARTESIAN_POINT ( 'NONE',  ( 4.909461021924240498, 7.781436054670031410, 1.082531754730549078 ) ) ;
#34338=CARTESIAN_POINT ( 'NONE',  ( -5.581116510680924847, 6.540332679663050541, -1.199719254218453823 ) ) ;
#34350=CARTESIAN_POINT ( 'NONE',  ( 4.553559489343365740, 6.405848385690952718, -1.599625672291269396 ) ) ;
#34351=CARTESIAN_POINT ( 'NONE',  ( 4.817943484809818600, 6.714296380401858499, 1.599625672291269396 ) ) ;
#34359=CARTESIAN_POINT ( 'NONE',  ( -2.889872605471121236, 6.605953636083950364, 2.420000000000000373 ) ) ;
#34369=CARTESIAN_POINT ( 'NONE',  ( 4.495411241332118557, 8.048790631822491548, -2.444653990452267944 ) ) ;
#34375=CARTESIAN_POINT ( 'NONE',  ( 6.210516883511641772, 9.403297576475722508, 1.199719254218452047 ) ) ;
#34382=CARTESIAN_POINT ( 'NONE',  ( 5.318541398310776103, 9.426991741329731056, -0.7998128361456481317 ) ) ;
#34388=CARTESIAN_POINT ( 'NONE',  ( 5.899206235721897507, 6.055031161196562373, 0.000000000000000000 ) ) ;
#34392=CARTESIAN_POINT ( 'NONE',  ( 4.895902868310594513, 8.725987423088758632, 0.000000000000000000 ) ) ;
#34404=CARTESIAN_POINT ( 'NONE',  ( 6.297309100973213170, 6.875137029808006339, 0.7249047842670247599 ) ) ;
#34405=CARTESIAN_POINT ( 'NONE',  ( -6.943184063974186415, 7.273005294157565359, -0.7216878364870338292 ) ) ;
#34441=CARTESIAN_POINT ( 'NONE',  ( 5.155843554946782703, 9.237177590738404831, -0.7998128361456481317 ) ) ;
#34442=CARTESIAN_POINT ( 'NONE',  ( 5.352436782344940802, 9.466536356036257871, 0.000000000000000000 ) ) ;
#34451=PRESENTATION_STYLE_ASSIGNMENT (( #67989 ) ) ;
#34458=CARTESIAN_POINT ( 'NONE',  ( -3.949167883330528372, 7.829389307186077396, 1.214306433183764966E-14 ) ) ;
#34461=CARTESIAN_POINT ( 'NONE',  ( 4.041739190205284160, 7.729463131965888856, 0.000000000000000000 ) ) ;
#34475=CARTESIAN_POINT ( 'NONE',  ( -5.628043163448566588, 9.580151100749725757, 0.000000000000000000 ) ) ;
#34477=CARTESIAN_POINT ( 'NONE',  ( -6.292392690518223475, 6.513748691792265788, -0.7216878364870338292 ) ) ;
#34502=CARTESIAN_POINT ( 'NONE',  ( -3.305155586681401303, 7.078041627762083898, 0.7998128361456352531 ) ) ;
#34514=CARTESIAN_POINT ( 'NONE',  ( -5.847422642759834588, 7.296647196851402839, -1.286413008881746256 ) ) ;
#34516=ORIENTED_EDGE ( 'NONE', *, *, #106606, .F. ) ;
#34519=EDGE_CURVE ( 'NONE', #45181, #40348, #116353, .T. ) ;
#34532=CARTESIAN_POINT ( 'NONE',  ( 6.008198349511364000, 7.038594824965278995, 1.199719254218453823 ) ) ;
#34539=EDGE_CURVE ( 'NONE', #158833, #65494, #24438, .T. ) ;
#34554=CARTESIAN_POINT ( 'NONE',  ( 5.332099551924443404, 9.442809587212341427, 0.000000000000000000 ) ) ;
#34555=CARTESIAN_POINT ( 'NONE',  ( 6.412080304620304538, 6.445458208337293549, -0.7998128361456481317 ) ) ;
#34557=CARTESIAN_POINT ( 'NONE',  ( 6.066347387471824781, 6.042103138330730872, -0.7998128361456481317 ) ) ;
#34558=CARTESIAN_POINT ( 'NONE',  ( -4.787437654953777155, 6.678706214094487947, -1.250000000000001110 ) ) ;
#34570=CARTESIAN_POINT ( 'NONE',  ( 4.771426152247889796, 8.279957873513081879, -0.8122977234717634332 ) ) ;
#34571=CARTESIAN_POINT ( 'NONE',  ( -6.441532379824190357, 6.687744995982559892, 0.7216878364870257245 ) ) ;
#34572=CARTESIAN_POINT ( 'NONE',  ( 4.584065335196260804, 6.441438539186039591, 1.443375672974065660 ) ) ;
#34595=CARTESIAN_POINT ( 'NONE',  ( -4.516274566683622815, 5.401980094953223066, 1.082531754730549078 ) ) ;
#34600=CARTESIAN_POINT ( 'NONE',  ( 5.155843554946782703, 9.237177590738404831, -0.7998128361456481317 ) ) ;
#34618=CARTESIAN_POINT ( 'NONE',  ( -4.395760127892912372, 7.709923763356872684, -0.8030953006082339751 ) ) ;
#34620=EDGE_LOOP ( 'NONE', ( #27788, #93409, #67636, #153809 ) ) ;
#34627=CARTESIAN_POINT ( 'NONE',  ( -2.830620210203090181, 6.524417021870718258, 0.000000000000000000 ) ) ;
#34628=CARTESIAN_POINT ( 'NONE',  ( 7.180978637093494044, 8.406838493811077839, -1.199719254218452047 ) ) ;
#34632=CARTESIAN_POINT ( 'NONE',  ( -5.757633847399098670, 7.274473465504208036, 1.200491007486852002 ) ) ;
#34633=CARTESIAN_POINT ( 'NONE',  ( 5.176180785367283654, 9.260904359562321275, -0.7998128361456481317 ) ) ;
#34660=EDGE_LOOP ( 'NONE', ( #102847, #30618, #4481 ) ) ;
#34664=CARTESIAN_POINT ( 'NONE',  ( -5.986807348886189040, 9.142303119412650503, -1.199719254218452047 ) ) ;
#34666=CARTESIAN_POINT ( 'NONE',  ( 6.526270840131753737, 8.707344961610770540, -1.599625672291283607 ) ) ;
#34669=CARTESIAN_POINT ( 'NONE',  ( -4.394251184604987870, 5.259619482528146150, 1.082531754730549078 ) ) ;
#34686=CARTESIAN_POINT ( 'NONE',  ( 5.481239241674765950, 9.616805891921051952, -0.7998128361456481317 ) ) ;
#34695=CARTESIAN_POINT ( 'NONE',  ( 7.838022202476093270, 8.316983122409855156, 0.7216878364870267237 ) ) ;
#34708=CARTESIAN_POINT ( 'NONE',  ( -4.584065335196305213, 6.441438539186039591, 1.443375672974058777 ) ) ;
#34710=CARTESIAN_POINT ( 'NONE',  ( 6.062430963966053632, 7.101866208495718702, -1.199719254218452047 ) ) ;
#34714=CARTESIAN_POINT ( 'NONE',  ( -3.492107083971660586, 6.231819477012331632, 1.199719254218452935 ) ) ;
#34756=CARTESIAN_POINT ( 'NONE',  ( 4.203910148689107729, 7.062256385849379647, -1.199719254218448494 ) ) ;
#34759=CARTESIAN_POINT ( 'NONE',  ( -4.261005416444848315, 8.193199762486115034, 0.7998128361456352531 ) ) ;
#34763=CARTESIAN_POINT ( 'NONE',  ( -5.682275777458886346, 7.722684055159061423, 1.443375672974058777 ) ) ;
#34770=CARTESIAN_POINT ( 'NONE',  ( -7.774674742793745708, 8.035151719539642912, 0.7998128361456341429 ) ) ;
#34772=CIRCLE ( 'NONE', #211183, 0.08000000000000004330 ) ;
#34777=CARTESIAN_POINT ( 'NONE',  ( 7.075376061485196821, 9.347967719856493218, 1.599625672291268286 ) ) ;
#34778=CARTESIAN_POINT ( 'NONE',  ( -7.279802135894939852, 7.457800344824362604, -0.7998128361456362523 ) ) ;
#34780=CARTESIAN_POINT ( 'NONE',  ( 4.672271667806711548, 8.395315985019093930, 0.5582388282892002396 ) ) ;
#34785=CARTESIAN_POINT ( 'NONE',  ( 7.289443866002793371, 8.533381260871966134, 1.199719254218452047 ) ) ;
#34792=CARTESIAN_POINT ( 'NONE',  ( -6.140917232347002042, 6.129101290685087911, -0.7998128361456362523 ) ) ;
#34797=CARTESIAN_POINT ( 'NONE',  ( -6.947627372360122955, 7.070263120700404968, 0.000000000000000000 ) ) ;
#34800=CARTESIAN_POINT ( 'NONE',  ( 6.658462837642791676, 8.861568958707010779, 1.443375672974063439 ) ) ;
#34802=CARTESIAN_POINT ( 'NONE',  ( -7.553300976144794454, 7.984808358356614733, -0.7216878364870338292 ) ) ;
#34808=CARTESIAN_POINT ( 'NONE',  ( 5.332099551924443404, 9.442809587212341427, 0.000000000000000000 ) ) ;
#34817=CARTESIAN_POINT ( 'NONE',  ( -4.343764581222149701, 7.058997420150165070, 1.213430737042743957 ) ) ;
#34821=CARTESIAN_POINT ( 'NONE',  ( 6.265786130652515773, 6.994708711910199384, -0.9640221254198673151 ) ) ;
#34837=CARTESIAN_POINT ( 'NONE',  ( -5.031484404002922517, 6.963427452793760963, 1.443375672974058777 ) ) ;
#34849=CARTESIAN_POINT ( 'NONE',  ( -5.043389779576542331, 7.890798448915884222, -1.099773784605091009 ) ) ;
#34867=CARTESIAN_POINT ( 'NONE',  ( -4.142898457427624415, 6.991076079377632091, 1.199719254218452935 ) ) ;
#34877=LINE ( 'NONE', #204833, #33834 ) ;
#34881=CARTESIAN_POINT ( 'NONE',  ( 6.964048179274811012, 8.153752959689313684, 1.199719254218452047 ) ) ;
#34884=CARTESIAN_POINT ( 'NONE',  ( 6.658462837642799670, 7.901199744405670522, 1.082531754730549967 ) ) ;
#34899=CARTESIAN_POINT ( 'NONE',  ( -4.502189528189771472, 7.410248995266807803, -1.199719254218453823 ) ) ;
#34901=CARTESIAN_POINT ( 'NONE',  ( 5.071631979963703962, 8.074598522336444262, 1.199719254218451159 ) ) ;
#34910=CARTESIAN_POINT ( 'NONE',  ( -4.004454267989906668, 5.765225627445230927, 1.599625672291270506 ) ) ;
#34911=CARTESIAN_POINT ( 'NONE',  ( 4.543917759235442944, 5.330267469643351852, 1.199719254218452935 ) ) ;
#34917=CARTESIAN_POINT ( 'NONE',  ( -2.995508107964761191, 6.411541510041463887, -0.7147908198718248007 ) ) ;
#34918=CARTESIAN_POINT ( 'NONE',  ( 4.258142763143749399, 7.125527769379820242, 1.199719254218451159 ) ) ;
#34920=CARTESIAN_POINT ( 'NONE',  ( 4.688087255275310561, 8.691461907788344377, -0.7998128361456381397 ) ) ;
#34925=CARTESIAN_POINT ( 'NONE',  ( -6.510788175286835511, 6.826513026331759271, 0.5708727117093035375 ) ) ;
#34937=CARTESIAN_POINT ( 'NONE',  ( -4.787437638956939523, 5.718337012605431369, -1.082531754730549967 ) ) ;
#34940=CARTESIAN_POINT ( 'NONE',  ( -6.132223229318823243, 5.371873414713975947, 2.500000000000000444 ) ) ;
#34946=CARTESIAN_POINT ( 'NONE',  ( 4.312902262922978736, 5.164712407232485702, -1.082531754730548412 ) ) ;
#34967=CARTESIAN_POINT ( 'NONE',  ( 6.086684617892325733, 6.065829907154645539, -0.7998128361456481317 ) ) ;
#34988=CARTESIAN_POINT ( 'NONE',  ( 0.3965938887841921612, 3.117564169212590830, 1.962087417844435189 ) ) ;
#34990=CARTESIAN_POINT ( 'NONE',  ( 4.634908411025333130, 6.500755460986618495, 1.599625672291268286 ) ) ;
#34991=CARTESIAN_POINT ( 'NONE',  ( -3.960390268967665328, 6.674186842887300131, 1.082531754730549967 ) ) ;
#35014=CARTESIAN_POINT ( 'NONE',  ( -4.932134020321308654, 8.976183133675331050, 0.7998128361456291469 ) ) ;
#35021=CARTESIAN_POINT ( 'NONE',  ( -3.984117037569407938, 5.741498858621315371, 1.599625672291270506 ) ) ;
#35027=CARTESIAN_POINT ( 'NONE',  ( -6.720001414228860881, 7.869031733802326123, -1.199719254218452047 ) ) ;
#35034=CARTESIAN_POINT ( 'NONE',  ( 5.252858170651868441, 5.093032385374103299, -0.7998128361456481317 ) ) ;
#35040=CARTESIAN_POINT ( 'NONE',  ( -4.437261413422502798, 8.398831758960053406, 0.000000000000000000 ) ) ;
#35044=CARTESIAN_POINT ( 'NONE',  ( -6.780486220610184134, 9.003929572168926754, -1.443375672974066548 ) ) ;
#35048=CARTESIAN_POINT ( 'NONE',  ( 3.567203813726958828, 6.215469311773181182, 1.082531754730549078 ) ) ;
#35049=CARTESIAN_POINT ( 'NONE',  ( -4.055297343818976330, 5.824542549245813383, 1.443375672974065660 ) ) ;
#35057=ORIENTED_EDGE ( 'NONE', *, *, #106262, .F. ) ;
#35063=CARTESIAN_POINT ( 'NONE',  ( 0.1107184056071714995, 2.601508666554186444, 2.078650322257169503 ) ) ;
#35068=CARTESIAN_POINT ( 'NONE',  ( 6.480989489388473856, 6.848452138476523565, -0.6157061703677743081 ) ) ;
#35090=CARTESIAN_POINT ( 'NONE',  ( 6.292946923374557855, 6.878031543426355476, -0.7329977330566839200 ) ) ;
#35105=CARTESIAN_POINT ( 'NONE',  ( 8.025500584646550806, 8.327781868367935658, 0.000000000000000000 ) ) ;
#35108=CARTESIAN_POINT ( 'NONE',  ( -6.089547271193396227, 7.133501900260939443, -1.199719254218453823 ) ) ;
#35121=CARTESIAN_POINT ( 'NONE',  ( 5.845500506147374153, 6.848780674373954547, 1.199719254218453823 ) ) ;
#35123=CARTESIAN_POINT ( 'NONE',  ( 7.856023664475727308, 8.130058794835305136, -0.7998128361456341429 ) ) ;
#35128=AXIS2_PLACEMENT_3D ( 'NONE', #208849, #107174, #158014 ) ;
#35129=CARTESIAN_POINT ( 'NONE',  ( -7.255021596644144921, 7.636815748939187465, 0.7216878364870317197 ) ) ;
#35134=CARTESIAN_POINT ( 'NONE',  ( 5.905458427204159477, 9.047396044116986502, 1.199719254218452047 ) ) ;
#35146=CARTESIAN_POINT ( 'NONE',  ( -6.468648687495877958, 6.719380688266201496, 0.000000000000000000 ) ) ;
#35148=CARTESIAN_POINT ( 'NONE',  ( 4.895902868310594513, 8.725987423088758632, 0.000000000000000000 ) ) ;
#35158=CARTESIAN_POINT ( 'NONE',  ( -5.632486471834530661, 5.535932070087196344, -0.7998128361456362523 ) ) ;
#35159=CARTESIAN_POINT ( 'NONE',  ( -4.981695098378565945, 4.776675467721892332, -0.7998128361456362523 ) ) ;
#35163=CARTESIAN_POINT ( 'NONE',  ( 4.814553946184248368, 7.670711132973337065, -1.082531754730548412 ) ) ;
#35174=CARTESIAN_POINT ( 'NONE',  ( -5.911423380092099222, 7.159701334921778404, 1.127351979631958434 ) ) ;
#35179=CARTESIAN_POINT ( 'NONE',  ( 2.929970594329034395, 6.432399770110250437, -0.7216878364870338292 ) ) ;
#35182=CARTESIAN_POINT ( 'NONE',  ( -6.330731382938325602, 6.350551133041632212, 0.7998128361456281477 ) ) ;
#35196=CARTESIAN_POINT ( 'NONE',  ( 4.913904330310220558, 4.697586238308844919, 0.000000000000000000 ) ) ;
#35232=CARTESIAN_POINT ( 'NONE',  ( 7.065207446497155708, 9.336104335703744539, 0.000000000000000000 ) ) ;
#35235=CARTESIAN_POINT ( 'NONE',  ( 6.536439455564168277, 6.798469917679251573, 0.7216878364870328300 ) ) ;
#35241=CARTESIAN_POINT ( 'NONE',  ( 6.333067150914816423, 7.521571443223021625, 1.082531754730549967 ) ) ;
#35263=CARTESIAN_POINT ( 'NONE',  ( -5.164730172163054966, 4.990216387137135889, -0.7998128361456362523 ) ) ;
#35265=CARTESIAN_POINT ( 'NONE',  ( 5.695833931072550094, 5.817763472438987726, 0.000000000000000000 ) ) ;
#35271=CARTESIAN_POINT ( 'NONE',  ( -7.923814432544069142, 8.209148024248356990, 0.000000000000000000 ) ) ;
#35278=CARTESIAN_POINT ( 'NONE',  ( -6.183927461608886844, 7.347575139032721303, 1.082531754730548412 ) ) ;
#35280=AXIS2_PLACEMENT_3D ( 'NONE', #64845, #62708, #28089 ) ;
#35282=CARTESIAN_POINT ( 'NONE',  ( -4.762657100150483380, 8.778460060142702304, 0.000000000000000000 ) ) ;
#35305=CARTESIAN_POINT ( 'NONE',  ( -3.960390268523300339, 7.634556056670224855, 1.214306433183764966E-14 ) ) ;
#35307=CARTESIAN_POINT ( 'NONE',  ( 3.888156192069020634, 7.758209000714329839, 1.040834085586084257E-14 ) ) ;
#35308=CARTESIAN_POINT ( 'NONE',  ( -5.438755897737433287, 6.374245297895642537, -1.199719254218453823 ) ) ;
#35309=CARTESIAN_POINT ( 'NONE',  ( -6.805266759416629618, 6.904175738932996964, 0.000000000000000000 ) ) ;
#35365=CARTESIAN_POINT ( 'NONE',  ( 4.543917759235442944, 5.330267469643351852, 1.199719254218452935 ) ) ;
#35367=CARTESIAN_POINT ( 'NONE',  ( 1.886825320689258012, 2.480000000000016858, -2.459652456995881753 ) ) ;
#35379=CARTESIAN_POINT ( 'NONE',  ( 4.605417112443645600, 8.360468292628990383, 0.2083848827989076002 ) ) ;
#35383=CARTESIAN_POINT ( 'NONE',  ( 3.054329744828568227, 6.785411478933790264, 0.000000000000000000 ) ) ;
#35388=CARTESIAN_POINT ( 'NONE',  ( -4.938913097128142304, 8.984092056616635347, -0.7998128361456362523 ) ) ;
#35394=CARTESIAN_POINT ( 'NONE',  ( -6.309289698153002668, 6.533461890506125691, 0.1636223065131766075 ) ) ;
#35399=CARTESIAN_POINT ( 'NONE',  ( 6.427974226654860956, 7.632296364919712417, -1.082531754730548412 ) ) ;
#35403=CARTESIAN_POINT ( 'NONE',  ( -3.474632506852224356, 7.275764701294714420, -0.7998128361456481317 ) ) ;
#35415=CARTESIAN_POINT ( 'NONE',  ( 5.740951700743842423, 5.662474837148078421, -0.7998128361456481317 ) ) ;
#35416=CARTESIAN_POINT ( 'NONE',  ( 3.400062661977048428, 7.188766548940353829, -1.734723475976807094E-15 ) ) ;
#35424=CARTESIAN_POINT ( 'NONE',  ( 1.843739406749228538, 8.499999999999996447, -0.7750000000000013545 ) ) ;
#35448=CARTESIAN_POINT ( 'NONE',  ( 5.855142236255289845, 7.924361590421551860, -1.599625672291281386 ) ) ;
#35455=CARTESIAN_POINT ( 'NONE',  ( 4.367134877377630175, 7.148722219365612141, -1.082531754730548412 ) ) ;
#35459=CARTESIAN_POINT ( 'NONE',  ( 6.780486220610169035, 9.003929572168926754, -1.443375672974078761 ) ) ;
#35471=CARTESIAN_POINT ( 'NONE',  ( 6.093313910611117379, 7.014445836765536235, -0.9825430356366869900 ) ) ;
#35472=CARTESIAN_POINT ( 'NONE',  ( -6.346625304972878467, 7.537389289624049304, 1.082531754730548412 ) ) ;
#35506=CARTESIAN_POINT ( 'NONE',  ( 5.505492895601038938, 8.580769590579979678, -1.199719254218452047 ) ) ;
#35508=CARTESIAN_POINT ( 'NONE',  ( 7.388267364804250725, 7.584343111885245570, -0.7998128361456341429 ) ) ;
#35521=CARTESIAN_POINT ( 'NONE',  ( -4.261005416444848315, 8.193199762486115034, 0.7998128361456352531 ) ) ;
#35523=CARTESIAN_POINT ( 'NONE',  ( 5.167065940139554669, 9.042344340222555843, -0.7216878364870458196 ) ) ;
#35540=CARTESIAN_POINT ( 'NONE',  ( -6.943184063974175757, 9.193743722760251202, -1.443375672974066548 ) ) ;
#35542=CARTESIAN_POINT ( 'NONE',  ( -6.780486220610195680, 7.083191143566240910, -0.7216878364870338292 ) ) ;
#35563=CARTESIAN_POINT ( 'NONE',  ( -6.168033539574333979, 6.160736982450306876, 0.7998128361456281477 ) ) ;
#35575=CARTESIAN_POINT ( 'NONE',  ( -4.953783236630994402, 8.080086878320878796, -1.094444140625696837 ) ) ;
#35593=CARTESIAN_POINT ( 'NONE',  ( 6.387826650694035990, 7.481494509678370264, -1.199719254218452047 ) ) ;
#35597=EDGE_CURVE ( 'NONE', #170847, #100853, #55062, .T. ) ;
#35616=CARTESIAN_POINT ( 'NONE',  ( 4.830447868218803897, 8.857549289555754157, -0.7998128361456481317 ) ) ;
#35617=CARTESIAN_POINT ( 'NONE',  ( 6.710359684120930091, 6.793450817754725257, 0.7998128361456352531 ) ) ;
#35619=CARTESIAN_POINT ( 'NONE',  ( 5.740951700743842423, 5.662474837148078421, -0.7998128361456481317 ) ) ;
#35630=DIRECTION ( 'NONE',  ( 0.000000000000000000, 0.000000000000000000, -1.000000000000000000 ) ) ;
#35631=CARTESIAN_POINT ( 'NONE',  ( 4.730098472736550264, 8.327237590489470875, -0.7222317683119976461 ) ) ;
#35633=CARTESIAN_POINT ( 'NONE',  ( -6.929625909916163451, 7.257187447756535903, 0.7216878364870317197 ) ) ;
#35634=CARTESIAN_POINT ( 'NONE',  ( 4.421367491832270957, 6.251624388594711590, 1.443375672974058777 ) ) ;
#35655=CARTESIAN_POINT ( 'NONE',  ( -5.600926855776901192, 5.707038551260711579, -0.7216878364870338292 ) ) ;
#35660=CARTESIAN_POINT ( 'NONE',  ( 4.667750024854814050, 8.667735138964429709, -0.7998128361456381397 ) ) ;
#35662=VERTEX_POINT ( 'NONE', #33562 ) ;
#35667=ADVANCED_FACE ( 'NONE', ( #1033 ), #82303, .T. ) ;
#35681=CARTESIAN_POINT ( 'NONE',  ( -6.138551946455282682, 6.334268068046505107, -0.2462770601040304153 ) ) ;
#35691=CARTESIAN_POINT ( 'NONE',  ( 6.318982112420993502, 9.529840343536603697, -1.199719254218452047 ) ) ;
#35695=CARTESIAN_POINT ( 'NONE',  ( -5.200254360346833415, 7.740598053885397789, 1.191768289972208628 ) ) ;
#35696=CARTESIAN_POINT ( 'NONE',  ( 5.905458427204159477, 9.047396044116986502, 1.199719254218452047 ) ) ;
#35703=CARTESIAN_POINT ( 'NONE',  ( -3.009160446454586690, 6.366307309526169966, -0.7771143261618658205 ) ) ;
#35704=PRODUCT_DEFINITION_CONTEXT ( 'detailed design', #63005, 'design' ) ;
#35723=CARTESIAN_POINT ( 'NONE',  ( 4.014622883422321209, 5.777089012116397804, -1.443375672974068769 ) ) ;
#35727=CARTESIAN_POINT ( 'NONE',  ( -6.577640801285370209, 7.702944352034914566, -1.199719254218452047 ) ) ;
#35729=CARTESIAN_POINT ( 'NONE',  ( 6.038177310039780643, 8.137902509836795417, -1.599625672291283607 ) ) ;
#35742=VECTOR ( 'NONE', #149309, 1000.000000000000000 ) ;
#35746=CARTESIAN_POINT ( 'NONE',  ( -3.973948422136983183, 7.650373902552822791, -0.7216878364870569218 ) ) ;
#35754=CARTESIAN_POINT ( 'NONE',  ( 8.005163354226054295, 8.304055099544019214, 0.000000000000000000 ) ) ;
#35756=ADVANCED_FACE ( 'NONE', ( #98574 ), #103444, .T. ) ;
#35764=CARTESIAN_POINT ( 'NONE',  ( 6.699137298928145690, 8.909022496873262753, 1.443375672974065660 ) ) ;
#35777=CARTESIAN_POINT ( 'NONE',  ( -6.482206841109545259, 6.735198534148810090, 0.7216878364870257245 ) ) ;
#35779=CARTESIAN_POINT ( 'NONE',  ( 6.496291879603339758, 7.608037276739255006, 1.199719254218452935 ) ) ;
#35782=CARTESIAN_POINT ( 'NONE',  ( -7.391130018105325661, 8.652015104991543026, -1.199719254218452047 ) ) ;
#35784=CARTESIAN_POINT ( 'NONE',  ( -5.164730172163054966, 4.990216387137135889, -0.7998128361456362523 ) ) ;
#35799=DIRECTION ( 'NONE',  ( 0.000000000000000000, 0.000000000000000000, 1.000000000000000000 ) ) ;
#35829=CARTESIAN_POINT ( 'NONE',  ( 5.415556014015861841, 5.282846535965431300, -0.7998128361456481317 ) ) ;
#35832=CARTESIAN_POINT ( 'NONE',  ( -4.773352600463090845, 7.726605912919016106, 1.199719254218452935 ) ) ;
#35833=CARTESIAN_POINT ( 'NONE',  ( -4.817943484809862120, 6.714296380401858499, 1.599625672291263401 ) ) ;
#35836=CARTESIAN_POINT ( 'NONE',  ( -5.112833325684908559, 8.018703742390766109, -1.082531754730549967 ) ) ;
#35841=CARTESIAN_POINT ( 'NONE',  ( -6.261886844665283114, 8.398896966899865646, 1.599625672291269396 ) ) ;
#35850=CARTESIAN_POINT ( 'NONE',  ( -4.620296487206990932, 8.612372678375294299, 0.000000000000000000 ) ) ;
#35852=CARTESIAN_POINT ( 'NONE',  ( 4.601768607255383614, 8.481659704624913587, -0.1707596084408805059 ) ) ;
#35857=CARTESIAN_POINT ( 'NONE',  ( 6.424584688029230328, 8.588711117491191871, 1.599625672291268286 ) ) ;
#35867=CARTESIAN_POINT ( 'NONE',  ( -6.642568916052639771, 6.714361588341672515, 0.000000000000000000 ) ) ;
#35872=CARTESIAN_POINT ( 'NONE',  ( -6.448838341955544173, 7.552674816150118708, 1.199719254218452047 ) ) ;
#35877=CARTESIAN_POINT ( 'NONE',  ( -7.743115126736118015, 8.206258200713163475, 0.7216878364870317197 ) ) ;
#35883=CARTESIAN_POINT ( 'NONE',  ( 6.261886844665240481, 8.398896966899865646, 1.599625672291268286 ) ) ;
#35887=CARTESIAN_POINT ( 'NONE',  ( -4.955918092712652268, 4.886086657537050293, 0.4932186882876873901 ) ) ;
#35896=CARTESIAN_POINT ( 'NONE',  ( 6.567098404289990476, 6.791591158854626720, -0.3517435911668670423 ) ) ;
#35911=VERTEX_POINT ( 'NONE', #53008 ) ;
#35925=CARTESIAN_POINT ( 'NONE',  ( -6.239605170154193026, 7.010755437975583426, 1.009914170685573875 ) ) ;
#35943=CARTESIAN_POINT ( 'NONE',  ( -3.793249116773374396, 7.647484079536056356, 0.7998128361456352531 ) ) ;
#35960=CARTESIAN_POINT ( 'NONE',  ( 6.204791576909545192, 7.267953590263130259, -1.199719254218452047 ) ) ;
#35963=CARTESIAN_POINT ( 'NONE',  ( 6.834718834620487016, 7.146462526578263308, 0.000000000000000000 ) ) ;
#35976=CARTESIAN_POINT ( 'NONE',  ( -6.934069218746458318, 7.054445274817795486, -0.7998128361456362523 ) ) ;
#35977=CARTESIAN_POINT ( 'NONE',  ( 6.378184920586140727, 6.405913593630768510, 0.000000000000000000 ) ) ;
#35985=CARTESIAN_POINT ( 'NONE',  ( -4.462568837553487100, 5.235360394347691404, -1.199719254218453823 ) ) ;
#35986=CARTESIAN_POINT ( 'NONE',  ( 5.820193082016415609, 10.01225203898631655, 0.000000000000000000 ) ) ;
#35992=CARTESIAN_POINT ( 'NONE',  ( 5.794130544993763898, 7.853181283949808744, 1.599625672291269396 ) ) ;
#35997=CARTESIAN_POINT ( 'NONE',  ( -5.519007765018521638, 7.558588572879005874, 1.349693927849420438 ) ) ;
#36007=CARTESIAN_POINT ( 'NONE',  ( -3.160459205317013076, 6.701303149596211206, -0.7216878364870458196 ) ) ;
#36018=CARTESIAN_POINT ( 'NONE',  ( 5.248414862265931902, 5.295774558831261913, 0.000000000000000000 ) ) ;
#36021=CARTESIAN_POINT ( 'NONE',  ( -3.188928480291558287, 8.980740528189064875, 2.451733079074509547 ) ) ;
#36022=CARTESIAN_POINT ( 'NONE',  ( -4.437261413422502798, 8.398831758960053406, 0.000000000000000000 ) ) ;
#36057=CARTESIAN_POINT ( 'NONE',  ( -0.3598541952674910727, 3.203739155314830445, 2.034949316489486737 ) ) ;
#36060=CARTESIAN_POINT ( 'NONE',  ( 4.529305835417093640, 7.441884687032027657, -1.199719254218450271 ) ) ;
#36061=CARTESIAN_POINT ( 'NONE',  ( -4.990809943606281607, 6.915973915664348937, -1.443375672974066548 ) ) ;
#36084=CARTESIAN_POINT ( 'NONE',  ( -5.607179047703544583, 8.699403434699558346, 1.199719254218454489 ) ) ;
#36096=CARTESIAN_POINT ( 'NONE',  ( -5.966470118465691641, 9.118576350588734059, -1.199719254218452047 ) ) ;
#36103=CARTESIAN_POINT ( 'NONE',  ( 4.848976215542928792, 5.686169002002086970, 1.199719254218452047 ) ) ;
#36109=CARTESIAN_POINT ( 'NONE',  ( -3.949167883330528372, 7.829389307186077396, 1.214306433183764966E-14 ) ) ;
#36114=CARTESIAN_POINT ( 'NONE',  ( -5.750066545971566079, 8.762142499391876171, 1.082531754730550855 ) ) ;
#36117=CARTESIAN_POINT ( 'NONE',  ( -6.983858524370814003, 9.241197259889665006, 1.443375672974064550 ) ) ;
#36118=CARTESIAN_POINT ( 'NONE',  ( 5.248414861821569133, 6.256143772614186638, -1.082531754730548412 ) ) ;
#36119=CARTESIAN_POINT ( 'NONE',  ( -3.296040741453672318, 6.859481608422314025, 0.7216878364870338292 ) ) ;
#36128=( BOUNDED_CURVE ( )  B_SPLINE_CURVE ( 2, ( #65244, #96739, #131395 ),
 .UNSPECIFIED., .F., .T. ) 
 B_SPLINE_CURVE_WITH_KNOTS ( ( 3, 3 ),
 ( 0.2458097188974980585, 0.2499999999999997502 ),
 .UNSPECIFIED. ) 
 CURVE ( )  GEOMETRIC_REPRESENTATION_ITEM ( )  RATIONAL_B_SPLINE_CURVE ( ( 0.9330148535346174388, 0.9326330537515126196, 0.9999999999999960032 ) ) 
 REPRESENTATION_ITEM ( '' )  );
#36133=CARTESIAN_POINT ( 'NONE',  ( 0.1277519899680359672, 2.521810436023053992, 1.998702265207899620 ) ) ;
#36138=CARTESIAN_POINT ( 'NONE',  ( 6.425920342564602983, 6.885296541689900351, -0.7293792964763821107 ) ) ;
#36143=CARTESIAN_POINT ( 'NONE',  ( 6.021701820789710169, 7.165471523702656498, -1.202873050745705275 ) ) ;
#36145=ORIENTED_EDGE ( 'NONE', *, *, #14726, .F. ) ;
#36159=CARTESIAN_POINT ( 'NONE',  ( 6.483128551184942800, 6.753495492978965231, -0.1682882784904728146 ) ) ;
#36179=CARTESIAN_POINT ( 'NONE',  ( -4.796552484184649856, 8.818004674849227342, -0.7998128361456362523 ) ) ;
#36190=CARTESIAN_POINT ( 'NONE',  ( 4.227110032410640095, 8.153655147779589996, 0.7998128361456271485 ) ) ;
#36196=DIRECTION ( 'NONE',  ( 0.000000000000000000, 0.000000000000000000, -1.000000000000000000 ) ) ;
#36197=CARTESIAN_POINT ( 'NONE',  ( -7.390603132780803719, 7.794994207765291172, -0.7216878364870338292 ) ) ;
#36202=CARTESIAN_POINT ( 'NONE',  ( 3.051993976407674225, 6.574760382535328240, -0.7216878364870338292 ) ) ;
#36215=CARTESIAN_POINT ( 'NONE',  ( -5.750066545971566079, 8.762142499391876171, 1.082531754730550855 ) ) ;
#36216=CARTESIAN_POINT ( 'NONE',  ( 5.234856708652222856, 8.161064355852680308, 1.082531754730549078 ) ) ;
#36226=CARTESIAN_POINT ( 'NONE',  ( -3.772911886352873445, 7.623757310712140800, 0.7998128361456352531 ) ) ;
#36227=CARTESIAN_POINT ( 'NONE',  ( -5.334207092333882017, 5.187939460669764635, 0.7998128361456281477 ) ) ;
#36229=CARTESIAN_POINT ( 'NONE',  ( 6.387299765369506055, 7.584842826753462219, -1.082531754730548412 ) ) ;
#36242=CARTESIAN_POINT ( 'NONE',  ( -4.619186966818853435, 8.364647258818639131, 0.2498820228645174391 ) ) ;
#36250=CARTESIAN_POINT ( 'NONE',  ( -4.630991987519598396, 7.560518531151607213, 1.199719254218452935 ) ) ;
#36265=CARTESIAN_POINT ( 'NONE',  ( 4.927462483923885195, 4.713404084191450849, -0.7998128361456481317 ) ) ;
#36303=CARTESIAN_POINT ( 'NONE',  ( 6.563555762791525972, 6.830105609444471426, -0.7216878364870458196 ) ) ;
#36308=CARTESIAN_POINT ( 'NONE',  ( 6.997416677984476863, 7.336276677169590421, 0.000000000000000000 ) ) ;
#36322=CARTESIAN_POINT ( 'NONE',  ( -6.526270840131767059, 8.707344961610770540, -1.599625672291271394 ) ) ;
#36334=CARTESIAN_POINT ( 'NONE',  ( 4.055297343818931033, 6.784911763547157193, 1.082531754730549078 ) ) ;
#36340=CARTESIAN_POINT ( 'NONE',  ( -7.422162748838431412, 7.623887726591770608, -0.7998128361456362523 ) ) ;
#36345=CARTESIAN_POINT ( 'NONE',  ( -5.234856708652269042, 7.200695141551334721, 1.443375672974058777 ) ) ;
#36348=CARTESIAN_POINT ( 'NONE',  ( -5.749539660647037032, 8.865490816466966351, 1.199719254218454489 ) ) ;
#36363=AXIS2_PLACEMENT_3D ( 'NONE', #152565, #4152, #55075 ) ;
#36371=FACE_OUTER_BOUND ( 'NONE', #113988, .T. ) ;
#36373=CARTESIAN_POINT ( 'NONE',  ( -4.624739795592943459, 6.488892076315448065, -1.443375672974066548 ) ) ;
#36375=CARTESIAN_POINT ( 'NONE',  ( 5.734172623936983904, 5.654565914206774124, 0.7998128361456352531 ) ) ;
#36377=CARTESIAN_POINT ( 'NONE',  ( -6.154475385960665790, 6.144919136567696505, 0.000000000000000000 ) ) ;
#36378=CARTESIAN_POINT ( 'NONE',  ( -7.632314129850253259, 7.869064337772231355, 0.7998128361456341429 ) ) ;
#36391=ORIENTED_EDGE ( 'NONE', *, *, #84368, .T. ) ;
#36402=CARTESIAN_POINT ( 'NONE',  ( -6.337068562759858636, 6.936200024879327408, -0.9492287992594623525 ) ) ;
#36420=VECTOR ( 'NONE', #209927, 1000.000000000000000 ) ;
#36435=CARTESIAN_POINT ( 'NONE',  ( 5.273195401072370281, 5.116759154198018855, -0.7998128361456481317 ) ) ;
#36449=CARTESIAN_POINT ( 'NONE',  ( 4.693755526227673336, 8.251780594207492214, -0.6034641085399840010 ) ) ;
#36452=CARTESIAN_POINT ( 'NONE',  ( 5.011674058906918638, 5.875983152593414971, 1.199719254218452047 ) ) ;
#36456=ORIENTED_EDGE ( 'NONE', *, *, #3651, .T. ) ;
#36458=CARTESIAN_POINT ( 'NONE',  ( -6.261886844665283114, 8.398896966899865646, 1.599625672291269396 ) ) ;
#36469=CARTESIAN_POINT ( 'NONE',  ( 3.147653791585693028, 8.920000000000001705, 2.419999999999999485 ) ) ;
#36473=CARTESIAN_POINT ( 'NONE',  ( 5.397554552016216256, 7.390509292142662723, 1.443375672974065660 ) ) ;
#36476=CARTESIAN_POINT ( 'NONE',  ( -5.074494633264801990, 9.142270515442742607, 0.7998128361456291469 ) ) ;
#36486=CARTESIAN_POINT ( 'NONE',  ( 4.309512724297349884, 6.121127159803966933, 1.599625672291261402 ) ) ;
#36487=CARTESIAN_POINT ( 'NONE',  ( 5.306037014901791693, 7.283738832175834510, 1.599625672291269396 ) ) ;
#36506=CARTESIAN_POINT ( 'NONE',  ( 6.098455030413784783, 7.112933956528650015, -1.126327413477963502 ) ) ;
#36512=CARTESIAN_POINT ( 'NONE',  ( 5.422335090822693715, 5.290755458906732933, 0.000000000000000000 ) ) ;
#36517=CARTESIAN_POINT ( 'NONE',  ( 5.885121196783658526, 9.023669275293071834, 1.199719254218452047 ) ) ;
#36522=CARTESIAN_POINT ( 'NONE',  ( 4.665414256878284149, 6.536345614481700927, -1.443375672974068769 ) ) ;
#36525=CARTESIAN_POINT ( 'NONE',  ( 3.902768115887398803, 5.646591783325653147, -1.599625672291269396 ) ) ;
#36537=CARTESIAN_POINT ( 'NONE',  ( 6.483128551184942800, 6.753495492978965231, -0.1682882784904728146 ) ) ;
#36538=CARTESIAN_POINT ( 'NONE',  ( -5.641601317062239218, 8.635599732330991429, -1.082531754730549967 ) ) ;
#36545=CARTESIAN_POINT ( 'NONE',  ( -5.507549045659300369, 6.008722659170706137, 0.9225295215002001781 ) ) ;
#36572=CARTESIAN_POINT ( 'NONE',  ( 6.047819040147648373, 9.213483425884394507, 1.199719254218452047 ) ) ;
#36574=CARTESIAN_POINT ( 'NONE',  ( 5.688527969385528849, 8.794310509995222347, -1.199719254218452047 ) ) ;
#36587=CARTESIAN_POINT ( 'NONE',  ( -5.646044625448194410, 5.551749915969804938, 0.000000000000000000 ) ) ;
#36589=CARTESIAN_POINT ( 'NONE',  ( 4.706088717274885092, 8.504537580213796133, 0.7216878364870317197 ) ) ;
#36598=CARTESIAN_POINT ( 'NONE',  ( -3.122120512896910505, 6.864500708346841229, 0.7998128361456352531 ) ) ;
#36606=CARTESIAN_POINT ( 'NONE',  ( -5.451787166470911217, 9.374519104275787384, 0.7216878364870267237 ) ) ;
#36608=CARTESIAN_POINT ( 'NONE',  ( -5.478903473698255588, 7.485416367438324059, -1.443375672974066548 ) ) ;
#36633=CARTESIAN_POINT ( 'NONE',  ( -4.793689830883590020, 7.750332681742931662, 1.199719254218452935 ) ) ;
#36644=CARTESIAN_POINT ( 'NONE',  ( -4.905272163827030241, 8.130510659208837865, -1.040677472382423474 ) ) ;
#36659=CARTESIAN_POINT ( 'NONE',  ( 5.339680242214618566, 4.685059543140487115, 2.440369273555429874 ) ) ;
#36675=CARTESIAN_POINT ( 'NONE',  ( 5.923986774528332333, 5.876015756563318426, -0.7998128361456481317 ) ) ;
#36683=CARTESIAN_POINT ( 'NONE',  ( 6.008198349511364000, 7.038594824965278995, 1.199719254218453823 ) ) ;
#36685=CARTESIAN_POINT ( 'NONE',  ( 4.030516805012513082, 7.924296382481737844, 0.000000000000000000 ) ) ;
#36699=CARTESIAN_POINT ( 'NONE',  ( 4.641544345285703699, 8.432478572106539616, -0.4375188090333537727 ) ) ;
#36701=CARTESIAN_POINT ( 'NONE',  ( -5.356880090730904875, 7.343055753976412525, 1.443375672974058777 ) ) ;
#36702=CARTESIAN_POINT ( 'NONE',  ( 4.529832720741620022, 7.338536369956936589, -1.082531754730548412 ) ) ;
#36720=CARTESIAN_POINT ( 'NONE',  ( -6.441532379824190357, 6.687744995982559892, 0.7216878364870257245 ) ) ;
#36725=CARTESIAN_POINT ( 'NONE',  ( 6.703580607314123085, 6.785541894813420072, 0.000000000000000000 ) ) ;
#36753=CARTESIAN_POINT ( 'NONE',  ( 5.495418255317095380, 6.026204583819558813, -0.7979391942483996525 ) ) ;
#36754=CARTESIAN_POINT ( 'NONE',  ( 8.005163354226054295, 8.304055099544019214, 0.000000000000000000 ) ) ;
#36766=CARTESIAN_POINT ( 'NONE',  ( -3.003428079110303184, 6.384049572106303749, -0.7531072163598397928 ) ) ;
#36785=CARTESIAN_POINT ( 'NONE',  ( 3.879041347285658414, 6.579279767591636130, -1.082531754730548412 ) ) ;
#36792=CARTESIAN_POINT ( 'NONE',  ( 5.840530312436913007, 10.03597880781023299, 0.000000000000000000 ) ) ;
#36815=CARTESIAN_POINT ( 'NONE',  ( 7.679767667498067496, 7.924426798361372093, 0.000000000000000000 ) ) ;
#36816=EDGE_CURVE ( 'NONE', #142253, #204026, #164684, .T. ) ;
#36825=CARTESIAN_POINT ( 'NONE',  ( 6.048345925472166762, 10.07050432311064903, 0.7216878364870317197 ) ) ;
#36837=CARTESIAN_POINT ( 'NONE',  ( -5.424670859243583720, 8.382514198209223721, 1.082531754730550855 ) ) ;
#36840=CARTESIAN_POINT ( 'NONE',  ( 7.862802741282558294, 8.137967717776607657, 0.000000000000000000 ) ) ;
#36845=CARTESIAN_POINT ( 'NONE',  ( -4.004454267989906668, 5.765225627445230927, 1.599625672291270506 ) ) ;
#36847=CARTESIAN_POINT ( 'NONE',  ( 6.966220764712121927, 6.002124920821316323, 2.420000000000000373 ) ) ;
#36855=ORIENTED_EDGE ( 'NONE', *, *, #131734, .F. ) ;
#36858=DIRECTION ( 'NONE',  ( -0.6507913734559641616, -0.7592566023653004592, 0.000000000000000000 ) ) ;
#36876=VERTEX_POINT ( 'NONE', #97563 ) ;
#36888=CARTESIAN_POINT ( 'NONE',  ( 3.445180431648313224, 7.033477913649446300, 0.7216878364870257245 ) ) ;
#36892=CARTESIAN_POINT ( 'NONE',  ( -6.252245114557387851, 7.323316050852266557, -1.199719254218453823 ) ) ;
#36896=CARTESIAN_POINT ( 'NONE',  ( -3.610214042988883598, 7.433943160120816351, 0.7998128361456352531 ) ) ;
#36900=CARTESIAN_POINT ( 'NONE',  ( -5.275531169048909952, 7.248148678680751189, -1.443375672974066548 ) ) ;
#36905=ORIENTED_EDGE ( 'NONE', *, *, #136243, .T. ) ;
#36906=CARTESIAN_POINT ( 'NONE',  ( -4.938913097128142304, 8.984092056616635347, -0.7998128361456362523 ) ) ;
#36910=VERTEX_POINT ( 'NONE', #147369 ) ;
#36912=CARTESIAN_POINT ( 'NONE',  ( 3.602603900285803462, 7.346728939927271718, 0.3723553007324384989 ) ) ;
#36915=CARTESIAN_POINT ( 'NONE',  ( -5.981082042284069367, 7.006959133200059142, 1.199719254218452935 ) ) ;
#36917=CARTESIAN_POINT ( 'NONE',  ( 4.666526410304530970, 8.402211131567142388, 0.5382107299411863499 ) ) ;
#36922=CARTESIAN_POINT ( 'NONE',  ( 6.156284269057003655, 9.340026192945279249, -1.199719254218452047 ) ) ;
#36932=B_SPLINE_CURVE_WITH_KNOTS ( 'NONE', 3,
 ( #143296, #187720, #6820, #58799 ),
 .UNSPECIFIED., .F., .F.,
 ( 4, 4 ),
 ( 0.000000000000000000, 0.0004304244924211256284 ),
 .UNSPECIFIED. ) ;
#36934=CARTESIAN_POINT ( 'NONE',  ( -8.100070429521727178, 8.414780020722290033, 0.7998128361456341429 ) ) ;
#36937=EDGE_CURVE ( 'NONE', #61771, #90338, #200367, .T. ) ;
#36949=CARTESIAN_POINT ( 'NONE',  ( 7.340813827156391191, 7.528980651296110160, 0.7998128361456281477 ) ) ;
#36963=CARTESIAN_POINT ( 'NONE',  ( 5.620636616140949116, 7.477306742562066511, -1.332712173395997013 ) ) ;
#36991=CARTESIAN_POINT ( 'NONE',  ( -6.546709703855362328, 6.802806841334552601, 0.4695730141109008549 ) ) ;
#37004=DIRECTION ( 'NONE',  ( 0.000000000000000000, -1.000000000000000000, 0.000000000000000000 ) ) ;
#37008=CARTESIAN_POINT ( 'NONE',  ( -6.005335696210345020, 5.970922831858983315, 0.7998128361456281477 ) ) ;
#37025=CARTESIAN_POINT ( 'NONE',  ( 6.156811153937166381, 10.19704708965311468, 0.000000000000000000 ) ) ;
#37039=CARTESIAN_POINT ( 'NONE',  ( -5.101610940492132151, 9.173906207207963348, -0.7998128361456362523 ) ) ;
#37041=CARTESIAN_POINT ( 'NONE',  ( 4.518610335104485287, 8.493738834255713854, 0.000000000000000000 ) ) ;
#37052=CARTESIAN_POINT ( 'NONE',  ( -5.191846479390389568, 5.021852078902356631, 0.7998128361456281477 ) ) ;
#37053=CARTESIAN_POINT ( 'NONE',  ( 3.923105346307896202, 5.670318552149568703, -1.599625672291269396 ) ) ;
#37060=CARTESIAN_POINT ( 'NONE',  ( 6.282224075085741433, 8.422623735723785643, 1.599625672291268286 ) ) ;
#37066=CARTESIAN_POINT ( 'NONE',  ( -4.631600894319110040, 8.440630447364583233, 0.4419995416731822280 ) ) ;
#37078=CARTESIAN_POINT ( 'NONE',  ( -4.272227801637618505, 7.998366511970260717, 0.7216878364870338292 ) ) ;
#37087=CARTESIAN_POINT ( 'NONE',  ( 4.502716413514295191, 6.346531463890372926, -1.443375672974068769 ) ) ;
#37091=VECTOR ( 'NONE', #123524, 1000.000000000000000 ) ;
#37092=CARTESIAN_POINT ( 'NONE',  ( -5.478376588373717659, 8.549133898814758936, -1.199719254218452047 ) ) ;
#37107=CARTESIAN_POINT ( 'NONE',  ( 5.422335090822693715, 5.290755458906732933, 0.000000000000000000 ) ) ;
#37111=CARTESIAN_POINT ( 'NONE',  ( 4.050854035433010480, 7.948023151305657841, 0.000000000000000000 ) ) ;
#37121=ORIENTED_EDGE ( 'NONE', *, *, #134227, .F. ) ;
#37131=CARTESIAN_POINT ( 'NONE',  ( 6.229045230835819069, 6.231917288922055320, -0.7998128361456481317 ) ) ;
#37132=CARTESIAN_POINT ( 'NONE',  ( -5.668717624289589807, 5.786127781192186958, 0.7216878364870257245 ) ) ;
#37155=AXIS2_PLACEMENT_3D ( 'NONE', #190575, #42231, #74713 ) ;
#37160=CARTESIAN_POINT ( 'NONE',  ( -5.498713818794216834, 8.572860667638675380, -1.199719254218452047 ) ) ;
#37162=CARTESIAN_POINT ( 'NONE',  ( 7.634649897826745857, 8.079715433652276957, 0.7216878364870267237 ) ) ;
#37171=CARTESIAN_POINT ( 'NONE',  ( 4.207966135563057541, 7.175396087857926375, 2.420000000000000373 ) ) ;
#37172=ORIENTED_EDGE ( 'NONE', *, *, #176059, .T. ) ;
#37177=CARTESIAN_POINT ( 'NONE',  ( -7.123883369337781879, 7.275895117174344229, 0.7998128361456341429 ) ) ;
#37188=CARTESIAN_POINT ( 'NONE',  ( -5.966470118465691641, 9.118576350588734059, -1.199719254218452047 ) ) ;
#37192=CARTESIAN_POINT ( 'NONE',  ( -2.959422669532919326, 6.674686557755516780, 0.7998128361456352531 ) ) ;
#37196=CARTESIAN_POINT ( 'NONE',  ( -8.041394506236766659, 8.554250810130591631, -0.7216878364870338292 ) ) ;
#37197=CARTESIAN_POINT ( 'NONE',  ( 3.377389663135653031, 6.954388683717978026, -0.7216878364870338292 ) ) ;
#37198=CARTESIAN_POINT ( 'NONE',  ( -5.275531169048922386, 5.327410250078064458, -0.7216878364870338292 ) ) ;
#37203=CARTESIAN_POINT ( 'NONE',  ( -5.204350862799341115, 7.165104988056252289, -1.599625672291271394 ) ) ;
#37212=CARTESIAN_POINT ( 'NONE',  ( 5.903649544107831382, 5.852288987739401982, -0.7998128361456481317 ) ) ;
#37217=CARTESIAN_POINT ( 'NONE',  ( 1.857254922381494255, 2.486639013987944402, 2.482058795360528869 ) ) ;
#37218=CARTESIAN_POINT ( 'NONE',  ( 6.104935607482663507, 7.108274908414393245, 1.121150977946131722 ) ) ;
#37221=CARTESIAN_POINT ( 'NONE',  ( 0.1023730323140637083, 2.520000000000004903, 1.999999999999999556 ) ) ;
#37229=CARTESIAN_POINT ( 'NONE',  ( 6.282224075085741433, 8.422623735723785643, 1.599625672291268286 ) ) ;
#37240=CARTESIAN_POINT ( 'NONE',  ( 5.701630405109389343, 7.302376724489803905, 1.216486997566777584 ) ) ;
#37258=CARTESIAN_POINT ( 'NONE',  ( -5.875479466675803231, 7.948088359245467416, -1.599625672291271394 ) ) ;
#37262=B_SPLINE_CURVE_WITH_KNOTS ( 'NONE', 3,
 ( #83712, #164973, #133582, #184408 ),
 .UNSPECIFIED., .F., .F.,
 ( 4, 4 ),
 ( 0.000000000000000000, 0.0007521701867342633907 ),
 .UNSPECIFIED. ) ;
#37270=CARTESIAN_POINT ( 'NONE',  ( 4.525389411911321602, 8.501647757197021704, -0.7998128361456381397 ) ) ;
#37276=CARTESIAN_POINT ( 'NONE',  ( -2.428612866367529932E-14, 2.999999999999999112, 7.500000000000000000 ) ) ;
#37282=CARTESIAN_POINT ( 'NONE',  ( 3.567203813726949058, 7.175838526074521440, 0.7216878364870257245 ) ) ;
#37283=CARTESIAN_POINT ( 'NONE',  ( 5.591005849568446706, 5.791977450266268868, -0.7139200525481930182 ) ) ;
#37288=CARTESIAN_POINT ( 'NONE',  ( 1.896098101912840894, 8.993996023093842496, 0.7750000000000004663 ) ) ;
#37290=CARTESIAN_POINT ( 'NONE',  ( -6.116136693540540570, 10.14959355252369910, 0.000000000000000000 ) ) ;
#37295=CARTESIAN_POINT ( 'NONE',  ( -2.823841133396259639, 6.516508098929413961, -0.7998128361456481317 ) ) ;
#37296=CARTESIAN_POINT ( 'NONE',  ( 4.882344714696929877, 8.710169577206153591, -0.7216878364870458196 ) ) ;
#37301=ORIENTED_EDGE ( 'NONE', *, *, #105692, .T. ) ;
#37306=CARTESIAN_POINT ( 'NONE',  ( -3.634467696915153034, 6.397906858779740524, 1.199719254218452935 ) ) ;
#37307=CARTESIAN_POINT ( 'NONE',  ( -3.363304624641834106, 6.081549941127532222, -1.199719254218452047 ) ) ;
#37309=CARTESIAN_POINT ( 'NONE',  ( 6.333067150914808430, 8.481940657524365434, 1.443375672974063439 ) ) ;
#37321=CARTESIAN_POINT ( 'NONE',  ( -4.610539993796915148, 8.375707290415371986, 0.1689211187793551172 ) ) ;
#37330=CARTESIAN_POINT ( 'NONE',  ( -5.794130544993808307, 7.853181283949808744, 1.599625672291263179 ) ) ;
#37343=CARTESIAN_POINT ( 'NONE',  ( 5.713835393516482952, 5.630839145382857680, 0.7998128361456352531 ) ) ;
#37379=CARTESIAN_POINT ( 'NONE',  ( 6.211043768836181478, 7.379210830797944709, 1.082531754730549967 ) ) ;
#37384=CARTESIAN_POINT ( 'NONE',  ( 6.522881301506172846, 6.782652071278222117, -0.7216878364870458196 ) ) ;
#37398=CARTESIAN_POINT ( 'NONE',  ( -7.228432174741334038, 8.462200954400218578, -1.199719254218452047 ) ) ;
#37409=CARTESIAN_POINT ( 'NONE',  ( -5.015590482412729756, 4.816220082428420923, 0.000000000000000000 ) ) ;
#37411=CARTESIAN_POINT ( 'NONE',  ( 4.760321331729593375, 5.686701320840210627, -1.082531754730548412 ) ) ;
#37417=CARTESIAN_POINT ( 'NONE',  ( -4.655245641445871385, 6.524482229810530498, 1.599625672291263179 ) ) ;
#37422=CARTESIAN_POINT ( 'NONE',  ( -6.373741612200205076, 8.529394195690610303, 1.443375672974064550 ) ) ;
#37425=DIRECTION ( 'NONE',  ( 0.000000000000000000, 0.000000000000000000, -1.000000000000000000 ) ) ;
#37430=CARTESIAN_POINT ( 'NONE',  ( -2.810282979782591006, 6.500690253046801814, 0.000000000000000000 ) ) ;
#37439=CARTESIAN_POINT ( 'NONE',  ( 5.346851039111029991, 6.199209027673978412, 7.500000000000000000 ) ) ;
#37440=CARTESIAN_POINT ( 'NONE',  ( -3.902768115887413014, 5.646591783325653147, -1.599625672291283607 ) ) ;
#37445=CARTESIAN_POINT ( 'NONE',  ( -5.316205630334276400, 5.374863788244313767, -0.7216878364870338292 ) ) ;
#37447=CARTESIAN_POINT ( 'NONE',  ( -5.763624699140894592, 5.896852701852039580, -0.7216878364870338292 ) ) ;
#37448=CARTESIAN_POINT ( 'NONE',  ( 5.747730777550676073, 5.670383760089384495, 0.000000000000000000 ) ) ;
#37449=CARTESIAN_POINT ( 'NONE',  ( -3.657667580636712934, 7.489305620709952649, -0.7998128361456481317 ) ) ;
#37450=CARTESIAN_POINT ( 'NONE',  ( -7.456058132872594335, 7.663432341298296535, 0.000000000000000000 ) ) ;
#37491=VECTOR ( 'NONE', #37512, 1000.000000000000114 ) ;
#37509=CARTESIAN_POINT ( 'NONE',  ( 6.235824307642648279, 6.239826211863360506, 0.000000000000000000 ) ) ;
#37511=CARTESIAN_POINT ( 'NONE',  ( -3.921423297084331239, 8.995353878514519508, -0.7749999999999979128 ) ) ;
#37512=DIRECTION ( 'NONE',  ( 0.7592566023653004592, -0.6507913734559639396, 0.000000000000000000 ) ) ;
#37525=CARTESIAN_POINT ( 'NONE',  ( 4.179656494762836516, 8.098292687190454586, -0.7998128361456362523 ) ) ;
#37531=CARTESIAN_POINT ( 'NONE',  ( -7.774674742793745708, 8.035151719539642912, 0.7998128361456341429 ) ) ;
#37535=CARTESIAN_POINT ( 'NONE',  ( 5.083381250481017410, 4.895309311841474553, 0.7998128361456352531 ) ) ;
#37546=CARTESIAN_POINT ( 'NONE',  ( 4.394251184604957672, 8.140727125432173139, -0.7216878364870357165 ) ) ;
#37548=CARTESIAN_POINT ( 'NONE',  ( -5.180624094197616714, 5.216685329418210948, 0.7216878364870257245 ) ) ;
#37549=CARTESIAN_POINT ( 'NONE',  ( -5.448397627845328550, 7.449826213943242514, 1.599625672291263179 ) ) ;
#37556=ORIENTED_EDGE ( 'NONE', *, *, #158769, .F. ) ;
#37561=CARTESIAN_POINT ( 'NONE',  ( 4.634908411025333130, 6.500755460986618495, 1.599625672291268286 ) ) ;
#37562=CARTESIAN_POINT ( 'NONE',  ( 5.682802662783380754, 6.658966523782627434, 1.199719254218452935 ) ) ;
#37574=ORIENTED_EDGE ( 'NONE', *, *, #48686, .T. ) ;
#37580=CARTESIAN_POINT ( 'NONE',  ( 6.007156502879952953, 7.179297369210805080, -1.191424252104013037 ) ) ;
#37585=CARTESIAN_POINT ( 'NONE',  ( 4.871153761480781164, 8.051123856976298399, 0.9350251597124116243 ) ) ;
#37591=CARTESIAN_POINT ( 'NONE',  ( 4.655245641445829641, 6.524482229810530498, 1.599625672291269396 ) ) ;
#37595=CARTESIAN_POINT ( 'NONE',  ( 6.367489420273535039, 7.457767740854454708, -1.199719254218452047 ) ) ;
#37601=CARTESIAN_POINT ( 'NONE',  ( 4.502716413514295191, 6.346531463890372926, -1.443375672974068769 ) ) ;
#37604=CARTESIAN_POINT ( 'NONE',  ( 8.000720045840086669, 8.506797273001177828, 0.7216878364870267237 ) ) ;
#37605=ORIENTED_EDGE ( 'NONE', *, *, #149120, .T. ) ;
#37616=CARTESIAN_POINT ( 'NONE',  ( 6.348694402744908594, 6.841026321354189754, -0.6301123915167846645 ) ) ;
#37617=CARTESIAN_POINT ( 'NONE',  ( -4.146814880933400005, 5.931313009212638931, 1.599625672291270506 ) ) ;
#37625=CARTESIAN_POINT ( 'NONE',  ( -0.002066265982046951426, 3.412835225567954378, -2.002356613009339981 ) ) ;
#37633=CARTESIAN_POINT ( 'NONE',  ( -5.000000000000013323, 8.499999999999996447, -0.7750000000000013545 ) ) ;
#37645=AXIS2_PLACEMENT_3D ( 'NONE', #57837, #77290, #123999 ) ;
#37652=CARTESIAN_POINT ( 'NONE',  ( 7.042534447655770080, 7.180988041878682004, -0.7998128361456341429 ) ) ;
#37654=ADVANCED_FACE ( 'NONE', ( #63701 ), #211798, .T. ) ;
#37655=CARTESIAN_POINT ( 'NONE',  ( 5.664274315459256748, 9.830346811336296398, -0.7998128361456481317 ) ) ;
#37657=DIRECTION ( 'NONE',  ( -0.000000000000000000, -0.000000000000000000, 1.000000000000000000 ) ) ;
#37670=CARTESIAN_POINT ( 'NONE',  ( -5.632486471834530661, 5.535932070087196344, -0.7998128361456362523 ) ) ;
#37672=CARTESIAN_POINT ( 'NONE',  ( 6.061904078641523697, 7.205214525570814210, -1.082531754730548412 ) ) ;
#37682=CARTESIAN_POINT ( 'NONE',  ( -3.284818356260900796, 7.054314858938165678, 0.7998128361456352531 ) ) ;
#37685=CARTESIAN_POINT ( 'NONE',  ( -5.153507786970285665, 5.185049637652990207, -0.7216878364870338292 ) ) ;
#37689=CARTESIAN_POINT ( 'NONE',  ( -6.116136693540540570, 10.14959355252370266, 0.000000000000000000 ) ) ;
#37691=CARTESIAN_POINT ( 'NONE',  ( -5.966997003790232235, 7.094489604910957148, -1.082531754730549967 ) ) ;
#37695=UNCERTAINTY_MEASURE_WITH_UNIT (LENGTH_MEASURE( 1.000000000000000082E-05 ), #169790, 'distance_accuracy_value', 'NONE');
#37715=CARTESIAN_POINT ( 'NONE',  ( -5.764151584465413869, 6.753873599078290546, -1.199719254218453823 ) ) ;
#37723=CARTESIAN_POINT ( 'NONE',  ( -6.087900257701670981, 7.118292344597175081, -1.149031449265491167 ) ) ;
#37733=AXIS2_PLACEMENT_3D ( 'NONE', #177876, #63043, #112936 ) ;
#37749=CARTESIAN_POINT ( 'NONE',  ( 1.846004154127491415, 8.940320519588478732, -0.7749999999999996891 ) ) ;
#37758=CARTESIAN_POINT ( 'NONE',  ( 3.874598038455354665, 7.742391154831717692, -0.7998128361456362523 ) ) ;
#37767=CARTESIAN_POINT ( 'NONE',  ( 4.864343252252968597, 8.897093904262280972, 0.000000000000000000 ) ) ;
#37769=CARTESIAN_POINT ( 'NONE',  ( 4.694866332082116678, 8.699370830729650450, 0.7998128361456341429 ) ) ;
#37781=CARTESIAN_POINT ( 'NONE',  ( 6.485343392949857844, 6.752073445700102816, -0.1478272009810890908 ) ) ;
#37783=CARTESIAN_POINT ( 'NONE',  ( -5.817857313595549584, 6.920493299683823096, 1.082531754730549078 ) ) ;
#37784=CARTESIAN_POINT ( 'NONE',  ( 4.692530564105613422, 7.528350520548263702, -1.082531754730548412 ) ) ;
#37786=COLOUR_RGB ( '', 0.09019608, 0.27058824, 0.51372549) ;
#37802=CARTESIAN_POINT ( 'NONE',  ( -4.895902867866254837, 7.765618208269001066, 1.082531754730549967 ) ) ;
#37807=CARTESIAN_POINT ( 'NONE',  ( 5.936491157937257235, 8.019268665717216749, 1.599625672291268286 ) ) ;
#37848=CARTESIAN_POINT ( 'NONE',  ( 1.806654366501771136, 2.518449987798942136, 2.499999999999998668 ) ) ;
#37865=CARTESIAN_POINT ( 'NONE',  ( 3.743459811148990291, 7.381470523066878009, -0.7216878364870338292 ) ) ;
#37872=CARTESIAN_POINT ( 'NONE',  ( -7.553827861469316396, 8.841829255582865699, -1.199719254218452047 ) ) ;
#37874=CARTESIAN_POINT ( 'NONE',  ( 5.501576472095266901, 9.640532660744973725, -0.7998128361456481317 ) ) ;
#37878=CARTESIAN_POINT ( 'NONE',  ( -5.655159470675923394, 5.770309935309573923, 0.000000000000000000 ) ) ;
#37882=DIRECTION ( 'NONE',  ( 0.6507913734559688246, 0.7592566023652963514, 0.000000000000000000 ) ) ;
#37886=CARTESIAN_POINT ( 'NONE',  ( -4.950135482320918712, 7.828889591799445213, -1.082531754730549967 ) ) ;
#37898=CARTESIAN_POINT ( 'NONE',  ( 6.994027139803230320, 9.253060644560830994, -1.599625672291267398 ) ) ;
#37908=CARTESIAN_POINT ( 'NONE',  ( 8.000720045840086669, 8.506797273001177828, 0.7216878364870267237 ) ) ;
#37922=CARTESIAN_POINT ( 'NONE',  ( -4.163762573172648196, 7.871823745427799501, 0.000000000000000000 ) ) ;
#37925=CARTESIAN_POINT ( 'NONE',  ( 5.365994935958575240, 9.482354201918870018, 0.7998128361456341429 ) ) ;
#37930=CARTESIAN_POINT ( 'NONE',  ( -5.468734858265826837, 7.473552982767158070, 1.599625672291263179 ) ) ;
#37939=FACE_OUTER_BOUND ( 'NONE', #34112, .T. ) ;
#37959=VERTEX_POINT ( 'NONE', #171088 ) ;
#37970=CARTESIAN_POINT ( 'NONE',  ( 4.638297949650961982, 5.544340708415133712, -1.082531754730548412 ) ) ;
#37974=CARTESIAN_POINT ( 'NONE',  ( -4.633854640820660009, 8.628190524257904670, -0.7998128361456362523 ) ) ;
#37978=CARTESIAN_POINT ( 'NONE',  ( -4.634908411025374875, 6.500755460986618495, 1.599625672291263179 ) ) ;
#37983=CARTESIAN_POINT ( 'NONE',  ( -6.577113915960841162, 7.806292669110006521, -1.082531754730549967 ) ) ;
#37988=ORIENTED_EDGE ( 'NONE', *, *, #15314, .T. ) ;
#37989=CARTESIAN_POINT ( 'NONE',  ( -3.492107083971660586, 6.231819477012331632, 1.199719254218452935 ) ) ;
#37997=CARTESIAN_POINT ( 'NONE',  ( -5.271087860662956537, 9.371629280740593870, 0.000000000000000000 ) ) ;
#37999=CARTESIAN_POINT ( 'NONE',  ( 4.650542599771462449, 8.421518672640367242, 0.4769741307986720136 ) ) ;
#38004=CARTESIAN_POINT ( 'NONE',  ( 5.435893244436359240, 5.306573304789342416, -0.7998128361456481317 ) ) ;
#38012=DIRECTION ( 'NONE',  ( -0.6507913734559650498, 0.7592566023652995710, 0.000000000000000000 ) ) ;
#38020=CARTESIAN_POINT ( 'NONE',  ( 3.923301836239755147, 8.994671190470434397, -0.7749999999999996891 ) ) ;
#38029=CARTESIAN_POINT ( 'NONE',  ( 3.464990776744291345, 6.200183785247111778, 1.199719254218452047 ) ) ;
#38030=( BOUNDED_CURVE ( )  B_SPLINE_CURVE ( 2, ( #13815, #209877, #48482, #80960, #115647 ),
 .UNSPECIFIED., .F., .T. ) 
 B_SPLINE_CURVE_WITH_KNOTS ( ( 3, 2, 3 ),
 ( 0.02117536257016233020, 0.02500000000000000139, 0.02833227121364267215 ),
 .UNSPECIFIED. ) 
 CURVE ( )  GEOMETRIC_REPRESENTATION_ITEM ( )  RATIONAL_B_SPLINE_CURVE ( ( 0.9334640809516798754, 0.9385114893599890706, 1.000000000000000000, 0.9464272371605781942, 0.9356990284279831371 ) ) 
 REPRESENTATION_ITEM ( '' )  );
#38044=CARTESIAN_POINT ( 'NONE',  ( -0.4000000000000243916, 3.000000000000566214, -2.023857702507757317 ) ) ;
#38045=CARTESIAN_POINT ( 'NONE',  ( 5.713240515264599750, 7.403118591225121392, -1.316831503761767719 ) ) ;
#38054=EDGE_CURVE ( 'NONE', #31895, #129718, #118327, .T. ) ;
#38067=DIRECTION ( 'NONE',  ( 0.000000000000000000, 0.000000000000000000, -1.000000000000000000 ) ) ;
#38073=CARTESIAN_POINT ( 'NONE',  ( -6.065932567686177279, 7.134227558401057934, 1.164772332933713184 ) ) ;
#38088=CARTESIAN_POINT ( 'NONE',  ( 3.558982665580148641, 7.338500189690928543, -0.2527556040902705359 ) ) ;
#38092=CARTESIAN_POINT ( 'NONE',  ( -4.655245641445871385, 6.524482229810530498, 1.599625672291263179 ) ) ;
#38094=ORIENTED_EDGE ( 'NONE', *, *, #179894, .T. ) ;
#38109=CARTESIAN_POINT ( 'NONE',  ( 5.246079093845007257, 5.085123462432798114, 0.7998128361456352531 ) ) ;
#38111=CARTESIAN_POINT ( 'NONE',  ( 5.682275777458829502, 9.643422483761748154, 0.7216878364870317197 ) ) ;
#38125=CARTESIAN_POINT ( 'NONE',  ( 6.554440917563797875, 6.611545590104705994, -0.7998128361456481317 ) ) ;
#38136=CARTESIAN_POINT ( 'NONE',  ( -4.142898457427624415, 6.991076079377632091, 1.199719254218452935 ) ) ;
#38137=CARTESIAN_POINT ( 'NONE',  ( 3.736153849017632922, 6.516540702899320081, -1.199719254218453823 ) ) ;
#38141=CARTESIAN_POINT ( 'NONE',  ( -5.936491157937300756, 8.019268665717216749, 1.599625672291263179 ) ) ;
#38143=CARTESIAN_POINT ( 'NONE',  ( 5.417364897112183719, 8.477953592343014932, 1.199719254218451159 ) ) ;
#38147=EDGE_CURVE ( 'NONE', #138513, #156724, #208790, .T. ) ;
#38150=CARTESIAN_POINT ( 'NONE',  ( -4.589286827423546100, 8.493149336607261901, 0.1385767598228414277 ) ) ;
#38159=CARTESIAN_POINT ( 'NONE',  ( -4.082413651046300274, 6.816547455312373494, 1.082531754730549967 ) ) ;
#38168=CARTESIAN_POINT ( 'NONE',  ( 4.177320726786311056, 5.966903162707725805, -1.443375672974068769 ) ) ;
#38173=CARTESIAN_POINT ( 'NONE',  ( -6.099189001301292379, 8.209082816308541197, 1.599625672291263179 ) ) ;
#38186=CARTESIAN_POINT ( 'NONE',  ( 4.411198876399872404, 6.239761003923544713, -1.599625672291273171 ) ) ;
#38200=VERTEX_POINT ( 'NONE', #79004 ) ;
#38207=CIRCLE ( 'NONE', #72675, 0.8299999999999999600 ) ;
#38212=CARTESIAN_POINT ( 'NONE',  ( -4.150204419558982671, 7.856005899545188242, 0.7216878364870338292 ) ) ;
#38233=ADVANCED_FACE ( 'NONE', ( #59555 ), #177041, .T. ) ;
#38235=CARTESIAN_POINT ( 'NONE',  ( -5.447343857640614573, 9.577261277214532242, -0.7998128361456362523 ) ) ;
#38241=CARTESIAN_POINT ( 'NONE',  ( -3.526002468005825286, 6.271364091718859335, -1.199719254218450271 ) ) ;
#38250=CARTESIAN_POINT ( 'NONE',  ( -3.332271893908731464, 7.109677319527304640, -0.7998128361456481317 ) ) ;
#38256=CARTESIAN_POINT ( 'NONE',  ( 6.039231080244466199, 6.010467446565510130, 0.7998128361456352531 ) ) ;
#38261=CARTESIAN_POINT ( 'NONE',  ( -5.478376588373717659, 8.549133898814758936, -1.199719254218452047 ) ) ;
#38264=CARTESIAN_POINT ( 'NONE',  ( -6.102578539926875933, 10.13377570664109051, 0.7216878364870267237 ) ) ;
#38267=CARTESIAN_POINT ( 'NONE',  ( -6.089020385868850305, 10.11795786024005572, -0.7216878364870338292 ) ) ;
#38268=CARTESIAN_POINT ( 'NONE',  ( 3.729901657090948230, 6.405283462364505631, 1.082531754730549078 ) ) ;
#38269=CARTESIAN_POINT ( 'NONE',  ( -6.251718229232867685, 6.466295153626015590, -0.7216878364870338292 ) ) ;
#38271=ORIENTED_EDGE ( 'NONE', *, *, #13673, .T. ) ;
#38274=CARTESIAN_POINT ( 'NONE',  ( -4.285259070371116863, 7.157163461145040095, 1.199719254218452935 ) ) ;
#38283=CARTESIAN_POINT ( 'NONE',  ( 4.420840606507738357, 7.315341919971147355, 1.199719254218451159 ) ) ;
#38288=CARTESIAN_POINT ( 'NONE',  ( 5.260375520412221562, 7.786458765878076171, 1.288147692060326532 ) ) ;
#38297=CARTESIAN_POINT ( 'NONE',  ( 5.875479466675786355, 7.948088359245467416, -1.599625672291283607 ) ) ;
#38308=CARTESIAN_POINT ( 'NONE',  ( 6.365646016822680942, 6.829858545691475769, 0.5939985411197836740 ) ) ;
#38326=CARTESIAN_POINT ( 'NONE',  ( -4.294900800479008574, 8.232744377192641849, 0.000000000000000000 ) ) ;
#38339=CARTESIAN_POINT ( 'NONE',  ( 6.225128807330042591, 7.291680359087043151, -1.199719254218452047 ) ) ;
#38350=CARTESIAN_POINT ( 'NONE',  ( 4.597623488365603528, 5.496887170248887067, -1.082531754730548412 ) ) ;
#38363=CARTESIAN_POINT ( 'NONE',  ( -3.984117037569407938, 5.741498858621315371, 1.599625672291270506 ) ) ;
#38364=CARTESIAN_POINT ( 'NONE',  ( 7.200788982633824276, 7.573544365927161515, 0.000000000000000000 ) ) ;
#38375=CARTESIAN_POINT ( 'NONE',  ( -4.990283058281743678, 7.979691447040783814, -1.199719254218453823 ) ) ;
#38376=CARTESIAN_POINT ( 'NONE',  ( -4.390861645979385663, 6.216034235099629157, -1.599625672291271394 ) ) ;
#38379=CARTESIAN_POINT ( 'NONE',  ( 6.509323147892504657, 6.766834225395614411, 0.000000000000000000 ) ) ;
#38381=VERTEX_POINT ( 'NONE', #138735 ) ;
#38392=CARTESIAN_POINT ( 'NONE',  ( -4.675522092136524144, 8.294237829558845476, 0.5223692772225538850 ) ) ;
#38397=CARTESIAN_POINT ( 'NONE',  ( 5.736508392357904107, 5.865217010605237924, 0.000000000000000000 ) ) ;
#38401=CARTESIAN_POINT ( 'NONE',  ( -5.281783360975562225, 8.319775133516907673, 1.199719254218452935 ) ) ;
#38414=CARTESIAN_POINT ( 'NONE',  ( 4.016958651398847557, 7.908478536599129249, -0.7998128361456362523 ) ) ;
#38453=CARTESIAN_POINT ( 'NONE',  ( 5.234856708652222856, 8.161064355852680308, 1.082531754730549078 ) ) ;
#38459=CARTESIAN_POINT ( 'NONE',  ( 6.387299765369506055, 7.584842826753462219, -1.082531754730548412 ) ) ;
#38461=CARTESIAN_POINT ( 'NONE',  ( -3.894033820048823813, 8.999999999999998224, 0.7749999999999996891 ) ) ;
#38463=B_SPLINE_CURVE_WITH_KNOTS ( 'NONE', 3,
 ( #132217, #80231, #115989, #95453, #30431, #161503, #195049, #13083 ),
 .UNSPECIFIED., .F., .F.,
 ( 4, 2, 2, 4 ),
 ( 0.000000000000000000, 0.003117338238615241595, 0.004676007357922863476, 0.006234676477230485792 ),
 .UNSPECIFIED. ) ;
#38475=CARTESIAN_POINT ( 'NONE',  ( -7.781453819600577582, 8.043060642480948985, 0.000000000000000000 ) ) ;
#38485=CARTESIAN_POINT ( 'NONE',  ( -2.830620210203090181, 6.524417021870718258, 0.000000000000000000 ) ) ;
#38487=CARTESIAN_POINT ( 'NONE',  ( 5.858531774436539052, 6.007577623030311287, 0.000000000000000000 ) ) ;
#38492=CARTESIAN_POINT ( 'NONE',  ( -4.625266680917477835, 5.425174544939014964, -1.199719254218453823 ) ) ;
#38497=CARTESIAN_POINT ( 'NONE',  ( -7.458393901293492334, 7.874083437696761223, 0.7216878364870317197 ) ) ;
#38501=CARTESIAN_POINT ( 'NONE',  ( -7.449279056065764237, 7.655523418356991350, 0.7998128361456341429 ) ) ;
#38506=CARTESIAN_POINT ( 'NONE',  ( -5.147255595043616516, 6.034161611419515125, 1.199719254218452935 ) ) ;
#38520=CARTESIAN_POINT ( 'NONE',  ( -4.340018570150309785, 7.117086527600392287, -1.082531754730551743 ) ) ;
#38522=CARTESIAN_POINT ( 'NONE',  ( -4.841670253411603397, 5.781608396135871075, 1.082531754730549078 ) ) ;
#38524=CARTESIAN_POINT ( 'NONE',  ( 4.875038752565570732, 7.845239757038595663, -1.199719254218452047 ) ) ;
#38525=CARTESIAN_POINT ( 'NONE',  ( -5.712781623311813384, 7.758274208654143855, -1.599625672291271394 ) ) ;
#38526=CARTESIAN_POINT ( 'NONE',  ( -7.605197822622922210, 7.837428646007010613, -0.7998128361456362523 ) ) ;
#38527=CARTESIAN_POINT ( 'NONE',  ( -6.448443555175264130, 6.863647322328955802, -0.7618168508180013232 ) ) ;
#38529=CARTESIAN_POINT ( 'NONE',  ( 0.000000000000000000, 8.999999999999998224, 0.000000000000000000 ) ) ;
#38541=CARTESIAN_POINT ( 'NONE',  ( 5.361566827843168070, 4.701484413405860430, 2.440314516401218548 ) ) ;
#38576=CARTESIAN_POINT ( 'NONE',  ( 6.392116398764381202, 6.567141947923786027, -2.438447736780795072 ) ) ;
#38583=CARTESIAN_POINT ( 'NONE',  ( 5.306037014901791693, 7.283738832175834510, 1.599625672291269396 ) ) ;
#38596=CARTESIAN_POINT ( 'NONE',  ( 3.982994815507484354, 7.308283119008860851, -0.9368446653362592080 ) ) ;
#38599=CARTESIAN_POINT ( 'NONE',  ( 4.878955176071345434, 6.785476686873604280, -1.599625672291269396 ) ) ;
#38603=ORIENTED_EDGE ( 'NONE', *, *, #156207, .T. ) ;
#38605=CARTESIAN_POINT ( 'NONE',  ( -5.803772275101700906, 8.928762199997411386, -1.199719254218452047 ) ) ;
#38610=CARTESIAN_POINT ( 'NONE',  ( 4.213551878797002992, 8.137837301896977849, 0.000000000000000000 ) ) ;
#38622=CARTESIAN_POINT ( 'NONE',  ( 7.214347136247488912, 7.589362211809770997, -0.7216878364870317197 ) ) ;
#38624=CARTESIAN_POINT ( 'NONE',  ( -4.394251184604987870, 5.259619482528146150, 1.082531754730549078 ) ) ;
#38625=CARTESIAN_POINT ( 'NONE',  ( -5.152980901645737077, 8.169505597632108262, -1.199719254218453823 ) ) ;
#38636=CARTESIAN_POINT ( 'NONE',  ( 3.854260808034858155, 7.718664386007802136, -0.7998128361456362523 ) ) ;
#38637=CARTESIAN_POINT ( 'NONE',  ( 5.845500506147374153, 6.848780674373954547, 1.199719254218453823 ) ) ;
#38643=ORIENTED_EDGE ( 'NONE', *, *, #161384, .T. ) ;
#38655=CARTESIAN_POINT ( 'NONE',  ( 5.120401779693986910, 7.917229619699595489, -1.217862772375446712 ) ) ;
#38663=CARTESIAN_POINT ( 'NONE',  ( 6.211043768836151280, 6.418841616496627545, 0.7216878364870578100 ) ) ;
#38665=CARTESIAN_POINT ( 'NONE',  ( 3.413620815590684199, 7.204584394822967752, 0.7998128361456281477 ) ) ;
#38669=CARTESIAN_POINT ( 'NONE',  ( 4.435452530326143616, 5.203724702582467998, -1.199719254218452047 ) ) ;
#38674=CARTESIAN_POINT ( 'NONE',  ( 6.400857919427532572, 6.640291458853147866, -0.7216878364870458196 ) ) ;
#38676=CARTESIAN_POINT ( 'NONE',  ( -5.306037014901836990, 7.283738832175834510, 1.599625672291263179 ) ) ;
#38678=CARTESIAN_POINT ( 'NONE',  ( 5.239300017038202917, 5.077214539491492928, 0.000000000000000000 ) ) ;
#38689=CARTESIAN_POINT ( 'NONE',  ( 6.455362170788604637, 6.771378801287749383, -0.3290997004737963860 ) ) ;
#38691=CARTESIAN_POINT ( 'NONE',  ( -3.797165540279144214, 6.587721009371067638, 1.199719254218452935 ) ) ;
#38725=CARTESIAN_POINT ( 'NONE',  ( 7.614839552730775729, 8.913009562054615031, 1.199719254218452047 ) ) ;
#38727=CARTESIAN_POINT ( 'NONE',  ( 7.849244587668864348, 8.122149871893999062, 0.7998128361456291469 ) ) ;
#38740=CARTESIAN_POINT ( 'NONE',  ( -4.553559489343377287, 6.405848385690952718, -1.599625672291271394 ) ) ;
#38742=CARTESIAN_POINT ( 'NONE',  ( 5.628043163004202931, 8.619781885929965526, -1.082531754730548412 ) ) ;
#38752=CARTESIAN_POINT ( 'NONE',  ( -4.122561227007127016, 6.967349310553715647, 1.199719254218452935 ) ) ;
#38758=CARTESIAN_POINT ( 'NONE',  ( -3.149236820124241110, 6.896136400112061970, -0.7998128361456481317 ) ) ;
#38781=VERTEX_POINT ( 'NONE', #65952 ) ;
#38782=CARTESIAN_POINT ( 'NONE',  ( -4.145761110728687804, 8.058748072483927771, -0.7998128361456481317 ) ) ;
#38784=CARTESIAN_POINT ( 'NONE',  ( -4.462568837553487100, 5.235360394347691404, -1.199719254218453823 ) ) ;
#38812=CARTESIAN_POINT ( 'NONE',  ( 6.821160681006781523, 9.051383109298340557, 1.443375672974063439 ) ) ;
#38818=CARTESIAN_POINT ( 'NONE',  ( 1.844031106778964535, 8.927559574663328945, -0.7749999999999996891 ) ) ;
#38826=CARTESIAN_POINT ( 'NONE',  ( 3.711900195091365262, 7.552577004240394132, -0.7998128361456362523 ) ) ;
#38835=CARTESIAN_POINT ( 'NONE',  ( 5.956828388357757298, 8.042995434541133193, 1.599625672291269396 ) ) ;
#38837=CARTESIAN_POINT ( 'NONE',  ( 4.830447868218803897, 8.857549289555754157, -0.7998128361456481317 ) ) ;
#38850=CARTESIAN_POINT ( 'NONE',  ( 5.969043672405669909, 7.102642550806028687, -1.084880274121432064 ) ) ;
#38852=CARTESIAN_POINT ( 'NONE',  ( 6.726253606155519371, 7.019919760035800316, -0.7216878364870458196 ) ) ;
#38861=CARTESIAN_POINT ( 'NONE',  ( -3.135678666510573365, 6.880318554229450712, 0.000000000000000000 ) ) ;
#38870=CARTESIAN_POINT ( 'NONE',  ( -3.960390268523300339, 7.634556056670224855, 1.214306433183764966E-14 ) ) ;
#38875=CARTESIAN_POINT ( 'NONE',  ( 7.354371980770088690, 7.544798497178720531, 0.000000000000000000 ) ) ;
#38876=EDGE_CURVE ( 'NONE', #84144, #157271, #68715, .T. ) ;
#38933=CARTESIAN_POINT ( 'NONE',  ( 5.560252395380222090, 5.659585014131299552, 0.7216878364870328300 ) ) ;
#38940=CARTESIAN_POINT ( 'NONE',  ( -6.084577077482911101, 10.32070003369722144, 0.000000000000000000 ) ) ;
#38946=CARTESIAN_POINT ( 'NONE',  ( -4.502716413514301408, 7.306900678191715848, -1.082531754730549967 ) ) ;
#38952=CARTESIAN_POINT ( 'NONE',  ( 4.713352964544355039, 8.277509442901161307, 0.6665495596407186030 ) ) ;
#38977=CARTESIAN_POINT ( 'NONE',  ( 6.780486220610169035, 9.003929572168926754, -1.443375672974078761 ) ) ;
#38990=CARTESIAN_POINT ( 'NONE',  ( -5.478903473698255588, 7.485416367438324059, -1.443375672974066548 ) ) ;
#38993=CARTESIAN_POINT ( 'NONE',  ( 7.472478939787284169, 8.746922180287201698, 1.199719254218452935 ) ) ;
#38998=CARTESIAN_POINT ( 'NONE',  ( -4.132202957115018727, 8.042930226601317401, 0.000000000000000000 ) ) ;
#39014=FACE_OUTER_BOUND ( 'NONE', #176919, .T. ) ;
#39036=DIRECTION ( 'NONE',  ( 0.000000000000000000, 0.000000000000000000, 1.000000000000000000 ) ) ;
#39037=CARTESIAN_POINT ( 'NONE',  ( 5.126391479742934187, 6.113783160189109722, -1.082531754730548412 ) ) ;
#39041=CARTESIAN_POINT ( 'NONE',  ( -4.945692173934974178, 8.992000979557944973, 0.000000000000000000 ) ) ;
#39045=CARTESIAN_POINT ( 'NONE',  ( -6.261886844665283114, 8.398896966899865646, 1.599625672291269396 ) ) ;
#39050=CARTESIAN_POINT ( 'NONE',  ( -7.566859129758459979, 8.000626204239226880, 0.000000000000000000 ) ) ;
#39052=DIRECTION ( 'NONE',  ( -0.000000000000000000, -1.000000000000000000, -0.000000000000000000 ) ) ;
#39056=CARTESIAN_POINT ( 'NONE',  ( -3.006876207180748217, 6.730049018344652190, -0.7998128361456481317 ) ) ;
#39063=CARTESIAN_POINT ( 'NONE',  ( -7.930593509350902792, 8.217056947189661287, -0.7998128361456362523 ) ) ;
#39065=CARTESIAN_POINT ( 'NONE',  ( 5.865087380380676230, 7.178575736046542310, -1.148900262672468475 ) ) ;
#39068=CARTESIAN_POINT ( 'NONE',  ( 5.763039058787838620, 7.049721345481010815, 2.500000000000351719 ) ) ;
#39070=CARTESIAN_POINT ( 'NONE',  ( 5.422335090822693715, 5.290755458906732933, 0.000000000000000000 ) ) ;
#39081=CARTESIAN_POINT ( 'NONE',  ( -5.738844160334429567, 9.917344963690652548, 0.000000000000000000 ) ) ;
#39095=AXIS2_PLACEMENT_3D ( 'NONE', #147197, #13955, #193784 ) ;
#39096=CARTESIAN_POINT ( 'NONE',  ( 5.643937085038755797, 9.806620042512378177, -0.7998128361456481317 ) ) ;
#39104=CARTESIAN_POINT ( 'NONE',  ( 7.065207446497155708, 9.336104335703744539, 0.000000000000000000 ) ) ;
#39107=CIRCLE ( 'NONE', #87503, 0.07999999999999998779 ) ;
#39110=CARTESIAN_POINT ( 'NONE',  ( 6.468016842275610578, 6.857101109195174793, 0.6445861549769070775 ) ) ;
#39112=( BOUNDED_CURVE ( )  B_SPLINE_CURVE ( 2, ( #210015, #31301, #46484, #15013, #130991 ),
 .UNSPECIFIED., .F., .T. ) 
 B_SPLINE_CURVE_WITH_KNOTS ( ( 3, 2, 3 ),
 ( 0.2238897612321706643, 0.2250000000000000056, 0.2266653943240793667 ),
 .UNSPECIFIED. ) 
 CURVE ( )  GEOMETRIC_REPRESENTATION_ITEM ( )  RATIONAL_B_SPLINE_CURVE ( ( 0.9690575545878401531, 0.9821507451252642351, 1.000000000000000000, 0.9732255361470136812, 0.9571526819254749796 ) ) 
 REPRESENTATION_ITEM ( '' )  );
#39117=CARTESIAN_POINT ( 'NONE',  ( -2.974934349810927525, 6.692942428052418791, -0.01217162047775656973 ) ) ;
#39137=CARTESIAN_POINT ( 'NONE',  ( -6.616720264197946122, 6.757059058146986708, -0.05018984082068300712 ) ) ;
#39157=CARTESIAN_POINT ( 'NONE',  ( -6.252245114557387851, 7.323316050852266557, -1.199719254218453823 ) ) ;
#39174=CARTESIAN_POINT ( 'NONE',  ( 5.273195401072370281, 5.116759154198018855, -0.7998128361456481317 ) ) ;
#39176=CARTESIAN_POINT ( 'NONE',  ( 6.983858524370772258, 9.241197259889668558, 1.443375672974063439 ) ) ;
#39181=CARTESIAN_POINT ( 'NONE',  ( 4.807927017778164114, 8.120258031035326951, 0.8434019511586322571 ) ) ;
#39187=CARTESIAN_POINT ( 'NONE',  ( 6.313256805818848960, 7.394496357324014113, 1.199719254218452047 ) ) ;
#39195=CARTESIAN_POINT ( 'NONE',  ( -4.197131071882288289, 7.054347462908075350, -1.199719254218455378 ) ) ;
#39197=CARTESIAN_POINT ( 'NONE',  ( 3.627688620108284745, 6.389997935838436227, 1.199719254218452047 ) ) ;
#39201=CARTESIAN_POINT ( 'NONE',  ( -6.611536185319534908, 7.742488966741438716, 1.199719254218452047 ) ) ;
#39205=CARTESIAN_POINT ( 'NONE',  ( 6.200875153403774043, 8.327716660428123419, -1.599625672291283607 ) ) ;
#39210=CARTESIAN_POINT ( 'NONE',  ( -4.986341270546564175, 8.046800470007955397, 1.126807992560383331 ) ) ;
#39219=CARTESIAN_POINT ( 'NONE',  ( -5.167065940139584868, 6.161236697318522637, 1.082531754730549078 ) ) ;
#39230=CARTESIAN_POINT ( 'NONE',  ( 5.085717018901939390, 5.105960408239938353, 0.000000000000000000 ) ) ;
#39234=CARTESIAN_POINT ( 'NONE',  ( -5.803772275101700906, 8.928762199997411386, -1.199719254218452047 ) ) ;
#39252=CARTESIAN_POINT ( 'NONE',  ( 6.008198349511364000, 7.038594824965278995, 1.199719254218453823 ) ) ;
#39274=CARTESIAN_POINT ( 'NONE',  ( -4.502716413514310290, 6.346531463890372926, -1.443375672974066548 ) ) ;
#39300=CARTESIAN_POINT ( 'NONE',  ( -4.380693030546956912, 6.204170850428461392, 1.443375672974065660 ) ) ;
#39306=CARTESIAN_POINT ( 'NONE',  ( -5.984998465789844069, 5.947196063035064206, 0.7998128361456281477 ) ) ;
#39309=CARTESIAN_POINT ( 'NONE',  ( 0.000000000000000000, 9.999999999999998224, 0.000000000000000000 ) ) ;
#39315=CARTESIAN_POINT ( 'NONE',  ( -3.383641855062333281, 6.105276709951447778, -1.199719254218452047 ) ) ;
#39317=CARTESIAN_POINT ( 'NONE',  ( 5.348589505275513467, 7.707351500233518671, -1.315919829448284784 ) ) ;
#39321=CARTESIAN_POINT ( 'NONE',  ( 3.691562964670865199, 7.528850235416478576, -0.7998128361456362523 ) ) ;
#39326=CARTESIAN_POINT ( 'NONE',  ( -6.882699257592852504, 8.058845884393651460, -1.199719254218452047 ) ) ;
#39330=CARTESIAN_POINT ( 'NONE',  ( -4.472210567661380587, 6.310941310395290493, 1.599625672291270506 ) ) ;
#39335=CARTESIAN_POINT ( 'NONE',  ( 3.228249973385329596, 6.780392379009261283, -1.734723475976807094E-15 ) ) ;
#39336=CARTESIAN_POINT ( 'NONE',  ( -4.950135482320926705, 6.868520377498098739, -1.443375672974066548 ) ) ;
#39341=CARTESIAN_POINT ( 'NONE',  ( -5.798046968499580345, 6.793418213784815585, 1.199719254218452935 ) ) ;
#39344=CARTESIAN_POINT ( 'NONE',  ( 5.011674058906918638, 5.875983152593414971, 1.199719254218452047 ) ) ;
#39350=CARTESIAN_POINT ( 'NONE',  ( 5.041653019435334393, 6.975290837464928728, -1.599625672291269396 ) ) ;
#39355=CARTESIAN_POINT ( 'NONE',  ( 5.141188686642438554, 7.897460914975725998, 1.230089993873971999 ) ) ;
#39360=DIRECTION ( 'NONE',  ( -0.9667253911244640951, 0.2558163758543454125, 0.000000000000000000 ) ) ;
#39365=CARTESIAN_POINT ( 'NONE',  ( 7.049313524462606395, 7.188896964819984525, 0.000000000000000000 ) ) ;
#39375=CARTESIAN_POINT ( 'NONE',  ( 6.233692552841108458, 6.917895963632635592, 0.8214459722771473293 ) ) ;
#39393=CARTESIAN_POINT ( 'NONE',  ( -5.986807348886189040, 9.142303119412650503, -1.199719254218452047 ) ) ;
#39397=CARTESIAN_POINT ( 'NONE',  ( -4.858757509019083543, 5.629766575900002401, -2.420000000000000373 ) ) ;
#39408=CARTESIAN_POINT ( 'NONE',  ( 4.362691568547328202, 8.311833606605697256, -0.7998128361456381397 ) ) ;
#39411=CARTESIAN_POINT ( 'NONE',  ( -4.036671995544492297, 7.285761072467114019, 0.7944190476826870073 ) ) ;
#39415=CARTESIAN_POINT ( 'NONE',  ( 3.902768115887398803, 5.646591783325653147, -1.599625672291269396 ) ) ;
#39418=CARTESIAN_POINT ( 'NONE',  ( 5.085717018457579286, 6.066329622022862189, -1.082531754730548412 ) ) ;
#39429=ORIENTED_EDGE ( 'NONE', *, *, #82785, .F. ) ;
#39432=CARTESIAN_POINT ( 'NONE',  ( -5.804299160426224624, 9.785783097223662352, -0.7216878364870338292 ) ) ;
#39433=CARTESIAN_POINT ( 'NONE',  ( 6.699137298928153683, 7.948653282571920720, 1.082531754730549967 ) ) ;
#39442=CARTESIAN_POINT ( 'NONE',  ( -5.611095471209320174, 7.639640364534566075, 1.599625672291263179 ) ) ;
#39443=CARTESIAN_POINT ( 'NONE',  ( -4.659162064951642535, 5.464719159645540003, 1.199719254218452935 ) ) ;
#39446=CARTESIAN_POINT ( 'NONE',  ( 5.790741006368192778, 8.809596036521288198, -1.082531754730548412 ) ) ;
#39453=CARTESIAN_POINT ( 'NONE',  ( -5.623011108385752799, 7.471940032223963968, 1.349922804658145292 ) ) ;
#39458=CARTESIAN_POINT ( 'NONE',  ( -4.969355510774519757, 7.965585441469681172, -1.036248007939699178 ) ) ;
#39462=CARTESIAN_POINT ( 'NONE',  ( 5.573810548993915148, 5.675402860013913475, 0.000000000000000000 ) ) ;
#39466=CARTESIAN_POINT ( 'NONE',  ( -6.981522756394290319, 7.109807735406931783, 0.7998128361456341429 ) ) ;
#39478=CARTESIAN_POINT ( 'NONE',  ( 4.258142763143749399, 7.125527769379820242, 1.199719254218451159 ) ) ;
#39494=CARTESIAN_POINT ( 'NONE',  ( -5.275531169048911728, 6.287779464379406491, -1.082531754730549967 ) ) ;
#39517=CARTESIAN_POINT ( 'NONE',  ( 5.885648082108177803, 9.880690172519326353, 0.7216878364870317197 ) ) ;
#39522=CARTESIAN_POINT ( 'NONE',  ( 5.831415467209187575, 9.817418788470464008, 0.000000000000000000 ) ) ;
#39537=CARTESIAN_POINT ( 'NONE',  ( -5.745623237141265882, 9.925253886631958622, 0.7998128361456291469 ) ) ;
#39549=CARTESIAN_POINT ( 'NONE',  ( 3.404505970362959655, 6.986024375483197879, 0.7216878364870257245 ) ) ;
#39555=CARTESIAN_POINT ( 'NONE',  ( -5.164730172163054966, 4.990216387137135889, -0.7998128361456362523 ) ) ;
#39559=CARTESIAN_POINT ( 'NONE',  ( 0.000000000000000000, 1.016439536705160407E-16, 2.080000000000000071 ) ) ;
#39560=CARTESIAN_POINT ( 'NONE',  ( -7.282137904315833410, 7.668451441222825515, 0.000000000000000000 ) ) ;
#39563=CARTESIAN_POINT ( 'NONE',  ( -8.100070429521727178, 8.414780020722290033, 0.7998128361456341429 ) ) ;
#39568=CARTESIAN_POINT ( 'NONE',  ( -3.610214042988883598, 7.433943160120816351, 0.7998128361456352531 ) ) ;
#39582=CARTESIAN_POINT ( 'NONE',  ( -5.668717624289589807, 5.786127781192186958, 0.7216878364870257245 ) ) ;
#39584=CARTESIAN_POINT ( 'NONE',  ( -5.451787166026575981, 5.533042246551999277, 0.000000000000000000 ) ) ;
#39585=CARTESIAN_POINT ( 'NONE',  ( 4.386945222473598527, 7.275797305264619652, -1.199719254218452047 ) ) ;
#39587=CARTESIAN_POINT ( 'NONE',  ( -6.493429226302317225, 6.540365283632955773, 0.7998128361456341429 ) ) ;
#39588=CARTESIAN_POINT ( 'NONE',  ( -5.824109505522200081, 8.952488968821326054, -1.199719254218452047 ) ) ;
#39606=CARTESIAN_POINT ( 'NONE',  ( 5.905458427204159477, 9.047396044116986502, 1.199719254218452047 ) ) ;
#39628=CARTESIAN_POINT ( 'NONE',  ( 5.182959862174088883, 9.268813282503625572, 0.7998128361456331437 ) ) ;
#39635=CARTESIAN_POINT ( 'NONE',  ( 4.492294583947371578, 8.028511867739082319, -2.500000000000000000 ) ) ;
#39644=CARTESIAN_POINT ( 'NONE',  ( 5.923986774528332333, 5.876015756563318426, -0.7998128361456481317 ) ) ;
#39647=DIRECTION ( 'NONE',  ( 0.000000000000000000, 0.000000000000000000, 1.000000000000000000 ) ) ;
#39663=CARTESIAN_POINT ( 'NONE',  ( 5.740951700743842423, 5.662474837148078421, -0.7998128361456481317 ) ) ;
#39668=CARTESIAN_POINT ( 'NONE',  ( -7.099629715411508890, 8.311931418515415615, 1.199719254218452047 ) ) ;
#39672=ORIENTED_EDGE ( 'NONE', *, *, #65893, .T. ) ;
#39673=CARTESIAN_POINT ( 'NONE',  ( 5.761288931164342486, 5.686201605971993978, -0.7998128361456481317 ) ) ;
#39678=DIRECTION ( 'NONE',  ( 1.000000000000000000, 0.000000000000000000, 0.000000000000000000 ) ) ;
#39681=FACE_OUTER_BOUND ( 'NONE', #194083, .T. ) ;
#39685=CARTESIAN_POINT ( 'NONE',  ( 7.078765600110826561, 8.391552967285011988, -1.082531754730548412 ) ) ;
#39686=CARTESIAN_POINT ( 'NONE',  ( -3.851925040058337579, 6.547644075826416277, -1.082531754730546636 ) ) ;
#39687=CARTESIAN_POINT ( 'NONE',  ( -4.911796789900812144, 8.952456364851418158, 0.7998128361456291469 ) ) ;
#39689=CARTESIAN_POINT ( 'NONE',  ( -5.436182321379713578, 6.108390213082993903, 1.083092214668917919 ) ) ;
#39700=CARTESIAN_POINT ( 'NONE',  ( 5.879395890181562834, 6.888325289080478697, -1.199719254218452047 ) ) ;
#39701=CARTESIAN_POINT ( 'NONE',  ( 6.235824307642648279, 6.239826211863360506, 0.000000000000000000 ) ) ;
#39704=CARTESIAN_POINT ( 'NONE',  ( 7.862802741282558294, 8.137967717776607657, 0.000000000000000000 ) ) ;
#39720=CARTESIAN_POINT ( 'NONE',  ( 5.178155719255617129, 7.862379301422712352, -1.251444257556088457 ) ) ;
#39724=CARTESIAN_POINT ( 'NONE',  ( 6.343551558972093218, 6.506286488053501849, -2.500000000000000444 ) ) ;
#39725=CARTESIAN_POINT ( 'NONE',  ( 3.250922972226694352, 7.014770244231638863, 0.7998128361456281477 ) ) ;
#39730=CARTESIAN_POINT ( 'NONE',  ( 3.250922972226694352, 7.014770244231638863, 0.7998128361456281477 ) ) ;
#39735=CARTESIAN_POINT ( 'NONE',  ( 7.991605200612358573, 8.288237253661408843, 0.7998128361456281477 ) ) ;
#39740=VECTOR ( 'NONE', #65806, 1000.000000000000227 ) ;
#39741=CARTESIAN_POINT ( 'NONE',  ( 5.966997003790217136, 8.054858819212300958, -1.443375672974078761 ) ) ;
#39743=CARTESIAN_POINT ( 'NONE',  ( -6.154475385960665790, 6.144919136567696505, 0.000000000000000000 ) ) ;
#39745=CARTESIAN_POINT ( 'NONE',  ( 5.225741863424510747, 5.061396693608882558, 0.7998128361456352531 ) ) ;
#39757=CARTESIAN_POINT ( 'NONE',  ( -3.526002468005825286, 6.271364091718859335, -1.199719254218450271 ) ) ;
#39767=CARTESIAN_POINT ( 'NONE',  ( 0.2949160023044670731, 2.710037616963835827, -2.050670093719204168 ) ) ;
#39788=CARTESIAN_POINT ( 'NONE',  ( 3.106226591306694651, 6.638031766584184368, 0.000000000000000000 ) ) ;
#39795=CARTESIAN_POINT ( 'NONE',  ( 4.136646265500957043, 5.919449624541475607, -1.443375672974068769 ) ) ;
#39803=EDGE_CURVE ( 'NONE', #49550, #130236, #200051, .T. ) ;
#39810=CARTESIAN_POINT ( 'NONE',  ( -6.231907884136888676, 7.299589282028351001, -1.199719254218453823 ) ) ;
#39812=CARTESIAN_POINT ( 'NONE',  ( 6.685579144870162693, 6.972466221869550118, -0.7216878364870458196 ) ) ;
#39822=CARTESIAN_POINT ( 'NONE',  ( -4.285259070371116863, 7.157163461145040095, 1.199719254218452935 ) ) ;
#39826=CARTESIAN_POINT ( 'NONE',  ( -4.828112100242294424, 5.765790550771681566, -1.082531754730549967 ) ) ;
#39830=CARTESIAN_POINT ( 'NONE',  ( -5.147255595043616516, 6.034161611419515125, 1.199719254218452935 ) ) ;
#39831=ORIENTED_EDGE ( 'NONE', *, *, #161571, .T. ) ;
#39840=CARTESIAN_POINT ( 'NONE',  ( -0.3866901564497978727, 3.102326550341739875, 2.027579305719746205 ) ) ;
#39856=CARTESIAN_POINT ( 'NONE',  ( -5.306037014901836990, 7.283738832175834510, 1.599625672291263179 ) ) ;
#39858=CARTESIAN_POINT ( 'NONE',  ( -2.830620210203090181, 6.524417021870718258, 0.000000000000000000 ) ) ;
#39859=VERTEX_POINT ( 'NONE', #66761 ) ;
#39863=ORIENTED_EDGE ( 'NONE', *, *, #107334, .T. ) ;
#39868=CARTESIAN_POINT ( 'NONE',  ( -6.423891471114925977, 6.884501071190606503, -0.7550301924055674574 ) ) ;
#39882=CARTESIAN_POINT ( 'NONE',  ( -6.656127069666307072, 6.730179434224282886, 0.7998128361456341429 ) ) ;
#39903=CARTESIAN_POINT ( 'NONE',  ( 4.037295881819344956, 7.932205305423046582, -0.7998128361456362523 ) ) ;
#39912=CARTESIAN_POINT ( 'NONE',  ( 7.212011367826596242, 7.378711115411311638, 0.000000000000000000 ) ) ;
#39914=CARTESIAN_POINT ( 'NONE',  ( 5.936491157937257235, 8.019268665717216749, 1.599625672291268286 ) ) ;
#39926=CARTESIAN_POINT ( 'NONE',  ( 6.348694402744908594, 6.841026321354189754, -0.6301123915167846645 ) ) ;
#39928=CARTESIAN_POINT ( 'NONE',  ( 5.560252395380215873, 6.619954228432645138, 1.082531754730549078 ) ) ;
#39936=CARTESIAN_POINT ( 'NONE',  ( -4.309512724297390740, 6.121127159803966933, 1.599625672291270506 ) ) ;
#39943=TOROIDAL_SURFACE ( 'NONE', #36363, 0.4800000000000000933, 0.08000000000000000167 ) ;
#39948=CARTESIAN_POINT ( 'NONE',  ( -5.194182247366913252, 7.153241603385088965, 1.443375672974058777 ) ) ;
#39952=CARTESIAN_POINT ( 'NONE',  ( 5.833751235630055376, 10.02806988486892514, 0.7998128361456331437 ) ) ;
#39968=CARTESIAN_POINT ( 'NONE',  ( 3.588273936444265289, 7.344317902764286643, -0.3372145678562175064 ) ) ;
#39970=CARTESIAN_POINT ( 'NONE',  ( 5.182959862174088883, 9.268813282503625572, 0.7998128361456331437 ) ) ;
#40000=LINE ( 'NONE', #124528, #116119 ) ;
#40008=CARTESIAN_POINT ( 'NONE',  ( 3.933273961740286317, 7.602920365423422311, 0.7216878364870257245 ) ) ;
#40018=CARTESIAN_POINT ( 'NONE',  ( -3.201133666602369310, 6.748756687762456963, -0.7216878364870458196 ) ) ;
#40021=ORIENTED_EDGE ( 'NONE', *, *, #77981, .T. ) ;
#40022=CARTESIAN_POINT ( 'NONE',  ( 4.663288057535367237, 8.288536188413402783, 0.5084364831346009916 ) ) ;
#40033=CARTESIAN_POINT ( 'NONE',  ( -3.928309112595642638, 7.388819966165147690, 0.6129890987886537079 ) ) ;
#40036=EDGE_CURVE ( 'NONE', #83383, #81693, #74135, .T. ) ;
#40040=B_SPLINE_CURVE_WITH_KNOTS ( 'NONE', 3,
 ( #157137, #77997, #94280, #192797 ),
 .UNSPECIFIED., .F., .F.,
 ( 4, 4 ),
 ( 0.000000000000000000, 0.0001577902508744045485 ),
 .UNSPECIFIED. ) ;
#40046=ORIENTED_EDGE ( 'NONE', *, *, #107183, .T. ) ;
#40050=CARTESIAN_POINT ( 'NONE',  ( 5.225741863424510747, 5.061396693608882558, 0.7998128361456352531 ) ) ;
#40062=CARTESIAN_POINT ( 'NONE',  ( -6.943184063974186415, 7.273005294157565359, -0.7216878364870338292 ) ) ;
#40065=CARTESIAN_POINT ( 'NONE',  ( 7.147083253059300922, 8.367293879104554577, 1.199719254218452935 ) ) ;
#40079=FACE_OUTER_BOUND ( 'NONE', #123994, .T. ) ;
#40081=CARTESIAN_POINT ( 'NONE',  ( -4.858757509019083543, 5.629766575900002401, -2.420000000000000373 ) ) ;
#40095=ORIENTED_EDGE ( 'NONE', *, *, #77256, .F. ) ;
#40112=CARTESIAN_POINT ( 'NONE',  ( -5.596483547390937119, 9.751257581923240991, 0.000000000000000000 ) ) ;
#40115=CARTESIAN_POINT ( 'NONE',  ( -7.259464905474441565, 7.434073576000447048, -0.7998128361456362523 ) ) ;
#40116=CARTESIAN_POINT ( 'NONE',  ( -4.145761110728687804, 8.058748072483927771, -0.7998128361456481317 ) ) ;
#40120=CARTESIAN_POINT ( 'NONE',  ( -5.600926855776877211, 9.548515408466085930, -0.7216878364870338292 ) ) ;
#40122=CARTESIAN_POINT ( 'NONE',  ( 6.156811153937166381, 10.19704708965311468, 0.000000000000000000 ) ) ;
#40128=CARTESIAN_POINT ( 'NONE',  ( -6.831329296439251131, 9.063246493969506545, -1.599625672291271394 ) ) ;
#40134=CARTESIAN_POINT ( 'NONE',  ( -5.257529707049291900, 9.355811434857983500, 0.7998128361456291469 ) ) ;
#40136=CARTESIAN_POINT ( 'NONE',  ( 5.228576739797318851, 7.698598165248225378, -1.206158463488806953 ) ) ;
#40141=CARTESIAN_POINT ( 'NONE',  ( 4.435452530326143616, 5.203724702582467998, -1.199719254218452047 ) ) ;
#40152=CARTESIAN_POINT ( 'NONE',  ( -5.427006627220116286, 9.553534508390610469, -0.7998128361456362523 ) ) ;
#40164=CARTESIAN_POINT ( 'NONE',  ( 6.318982112420993502, 9.529840343536603697, -1.199719254218452047 ) ) ;
#40173=FACE_OUTER_BOUND ( 'NONE', #37, .T. ) ;
#40179=CARTESIAN_POINT ( 'NONE',  ( 6.013528089337225602, 7.174620582783560963, 1.187335689305318853 ) ) ;
#40180=CARTESIAN_POINT ( 'NONE',  ( -3.811250578772977349, 7.460559751961507224, -0.7216878364870458196 ) ) ;
#40209=CARTESIAN_POINT ( 'NONE',  ( -6.198085906554800850, 7.039857339855744023, 1.052733950999720003 ) ) ;
#40218=DIRECTION ( 'NONE',  ( 0.000000000000000000, 0.000000000000000000, -1.000000000000000000 ) ) ;
#40228=CARTESIAN_POINT ( 'NONE',  ( -6.200875153403786477, 8.327716660428123419, -1.599625672291271394 ) ) ;
#40245=CARTESIAN_POINT ( 'NONE',  ( 4.492547798081839794, 6.334668079219206049, 1.599625672291262513 ) ) ;
#40247=CARTESIAN_POINT ( 'NONE',  ( 7.471952054462754234, 8.850270497362297206, 1.082531754730549078 ) ) ;
#40256=CARTESIAN_POINT ( 'NONE',  ( 4.920187338115698417, 7.999083482620499730, 0.9937779052983791717 ) ) ;
#40275=CARTESIAN_POINT ( 'NONE',  ( -3.817502770699643388, 6.611447778194983194, 1.199719254218452935 ) ) ;
#40277=CARTESIAN_POINT ( 'NONE',  ( 5.520104819419390907, 6.469152373191302985, 1.199719254218452935 ) ) ;
#40279=LINE ( 'NONE', #106389, #4812 ) ;
#40280=CARTESIAN_POINT ( 'NONE',  ( -5.448397627845328550, 7.449826213943242514, 1.599625672291263179 ) ) ;
#40284=CARTESIAN_POINT ( 'NONE',  ( 5.528692779322568640, 9.672168352510192690, 0.7998128361456341429 ) ) ;
#40285=CARTESIAN_POINT ( 'NONE',  ( 5.311496422476285062, 4.760750348442155833, -2.499999999999999556 ) ) ;
#40288=CARTESIAN_POINT ( 'NONE',  ( -5.227029541856937023, 7.814379162078399332, 1.287352361829100733 ) ) ;
#40298=EDGE_CURVE ( 'NONE', #45216, #56229, #200701, .T. ) ;
#40299=CARTESIAN_POINT ( 'NONE',  ( -4.624739795592936353, 7.449261290616792763, -1.082531754730549967 ) ) ;
#40312=CARTESIAN_POINT ( 'NONE',  ( 4.746763178560250651, 7.591621904078704297, 1.082531754730549078 ) ) ;
#40317=CARTESIAN_POINT ( 'NONE',  ( -5.264308783856126439, 9.363720357799287797, -0.7998128361456362523 ) ) ;
#40319=ORIENTED_EDGE ( 'NONE', *, *, #6983, .T. ) ;
#40348=VERTEX_POINT ( 'NONE', #151265 ) ;
#40360=CARTESIAN_POINT ( 'NONE',  ( -6.468648687495877958, 6.719380688266201496, 0.000000000000000000 ) ) ;
#40364=EDGE_CURVE ( 'NONE', #133393, #29771, #75620, .T. ) ;
#40373=ADVANCED_FACE ( 'NONE', ( #4961 ), #131532, .T. ) ;
#40384=CARTESIAN_POINT ( 'NONE',  ( -8.106849506328558164, 8.422688943663599659, 0.000000000000000000 ) ) ;
#40390=CARTESIAN_POINT ( 'NONE',  ( -5.483346782084204563, 5.361935765378481378, 0.000000000000000000 ) ) ;
#40393=CARTESIAN_POINT ( 'NONE',  ( 4.421367491832275398, 8.172362817197386775, 0.7216878364870369378 ) ) ;
#40400=CARTESIAN_POINT ( 'NONE',  ( -7.533490631048818109, 8.818102486758951031, -1.199719254218452047 ) ) ;
#40402=CARTESIAN_POINT ( 'NONE',  ( 6.463557619869761517, 6.860074278669063830, -0.6545079704341187909 ) ) ;
#40406=CARTESIAN_POINT ( 'NONE',  ( 4.420840606507738357, 7.315341919971147355, 1.199719254218451159 ) ) ;
#40411=CARTESIAN_POINT ( 'NONE',  ( -4.911796789900812144, 8.952456364851418158, 0.7998128361456291469 ) ) ;
#40414=CARTESIAN_POINT ( 'NONE',  ( -5.496904935697871863, 5.377753611261092637, 0.7998128361456281477 ) ) ;
#40419=CARTESIAN_POINT ( 'NONE',  ( 5.112833325684902341, 7.058334528089426740, -1.443375672974078761 ) ) ;
#40420=CARTESIAN_POINT ( 'NONE',  ( -3.811250578772977349, 7.460559751961507224, -0.7216878364870458196 ) ) ;
#40427=CARTESIAN_POINT ( 'NONE',  ( 3.705121118284530279, 7.544668081299086282, -1.734723475976807094E-15 ) ) ;
#40429=ORIENTED_EDGE ( 'NONE', *, *, #31198, .T. ) ;
#40436=CARTESIAN_POINT ( 'NONE',  ( 0.000000000000000000, 8.920000000000001705, 0.000000000000000000 ) ) ;
#40441=CARTESIAN_POINT ( 'NONE',  ( 5.502223863662048409, 7.574938096329499437, 1.338028725624084148 ) ) ;
#40449=CARTESIAN_POINT ( 'NONE',  ( 4.715203562502613188, 8.723097599553565118, 0.7998128361456341429 ) ) ;
#40459=CARTESIAN_POINT ( 'NONE',  ( 5.279289985772466665, 7.652873027719338417, 1.222721368963412214 ) ) ;
#40477=CARTESIAN_POINT ( 'NONE',  ( -6.149505192250180663, 9.332117270003974951, -1.199719254218452047 ) ) ;
#40490=CARTESIAN_POINT ( 'NONE',  ( 7.700104897918568447, 7.948153567185284096, 0.000000000000000000 ) ) ;
#40499=CARTESIAN_POINT ( 'NONE',  ( 3.715816618597135523, 6.492813934075403637, -1.199719254218453823 ) ) ;
#40502=CARTESIAN_POINT ( 'NONE',  ( 4.326460416092276162, 7.101268681199365496, -1.082531754730548412 ) ) ;
#40506=EDGE_CURVE ( 'NONE', #134461, #179867, #160588, .T. ) ;
#40518=CARTESIAN_POINT ( 'NONE',  ( -4.995253251992230581, 4.792493313604505367, 0.000000000000000000 ) ) ;
#40519=CARTESIAN_POINT ( 'NONE',  ( 2.891631901464575272, 6.595597328342462262, 0.000000000000000000 ) ) ;
#40529=CARTESIAN_POINT ( 'NONE',  ( -5.152980901645737077, 8.169505597632108262, -1.199719254218453823 ) ) ;
#40530=CARTESIAN_POINT ( 'NONE',  ( -5.957882158562513908, 5.915560371269843465, -0.7998128361456362523 ) ) ;
#40532=CARTESIAN_POINT ( 'NONE',  ( 6.251718229232841928, 8.387033582228703210, -1.443375672974078761 ) ) ;
#40535=EDGE_CURVE ( 'NONE', #212849, #116379, #211064, .T. ) ;
#40544=CARTESIAN_POINT ( 'NONE',  ( -4.651028767811522080, 8.324525799487361155, 0.4279074293446327171 ) ) ;
#40548=CARTESIAN_POINT ( 'NONE',  ( 3.879041347285658414, 6.579279767591636130, -1.082531754730548412 ) ) ;
#40553=CARTESIAN_POINT ( 'NONE',  ( -5.610041701004606196, 9.767075427805856691, -0.7998128361456362523 ) ) ;
#40565=CARTESIAN_POINT ( 'NONE',  ( 5.285699784481295183, 7.260012063351913625, 1.599625672291268286 ) ) ;
#40569=( BOUNDED_CURVE ( )  B_SPLINE_CURVE ( 2, ( #89813, #154790, #36753 ),
 .UNSPECIFIED., .F., .T. ) 
 B_SPLINE_CURVE_WITH_KNOTS ( ( 3, 3 ),
 ( 0.2499999999999997502, 0.2554818834627949897 ),
 .UNSPECIFIED. ) 
 CURVE ( )  GEOMETRIC_REPRESENTATION_ITEM ( )  RATIONAL_B_SPLINE_CURVE ( ( 1.000000000000003997, 0.9118680251885524779, 0.9396870620400654683 ) ) 
 REPRESENTATION_ITEM ( '' )  );
#40581=CARTESIAN_POINT ( 'NONE',  ( -5.049006180819098688, 6.469209200322729281, -1.249999994511374668 ) ) ;
#40603=CARTESIAN_POINT ( 'NONE',  ( 5.207740401424913124, 9.089797878388800711, -0.7216878364870458196 ) ) ;
#40609=CARTESIAN_POINT ( 'NONE',  ( 7.810905894804431426, 8.285347430126213553, 0.000000000000000000 ) ) ;
#40636=CARTESIAN_POINT ( 'NONE',  ( -3.467853430045390706, 7.267855778353407459, 0.7998128361456352531 ) ) ;
#40638=CARTESIAN_POINT ( 'NONE',  ( 4.055297343818923039, 7.745280977848496562, 0.7216878364870257245 ) ) ;
#40644=CARTESIAN_POINT ( 'NONE',  ( -3.980200614063634568, 6.801261928786307642, 1.199719254218452935 ) ) ;
#40648=CYLINDRICAL_SURFACE ( 'NONE', #22791, 0.7500000000000011102 ) ;
#40649=CARTESIAN_POINT ( 'NONE',  ( -7.105881907338178038, 7.462819444748888920, -0.7216878364870338292 ) ) ;
#40652=ORIENTED_EDGE ( 'NONE', *, *, #133456, .T. ) ;
#40654=CARTESIAN_POINT ( 'NONE',  ( -7.587723245503481095, 8.881373870289390737, 1.199719254218452047 ) ) ;
#40658=CARTESIAN_POINT ( 'NONE',  ( -3.298376509874564988, 7.070132704820777825, 0.000000000000000000 ) ) ;
#40669=CARTESIAN_POINT ( 'NONE',  ( -4.001064729808656573, 7.682009594836471500, 1.214306433183764966E-14 ) ) ;
#40672=CARTESIAN_POINT ( 'NONE',  ( -6.902509602688830626, 7.225551755991315162, -0.7216878364870338292 ) ) ;
#40673=CARTESIAN_POINT ( 'NONE',  ( 4.877901405866606588, 8.912911750144889567, 0.7998128361456341429 ) ) ;
#40674=CARTESIAN_POINT ( 'NONE',  ( -6.469175572376043348, 7.576401584974034265, 1.199719254218452047 ) ) ;
#40694=CARTESIAN_POINT ( 'NONE',  ( 7.526711554241970248, 8.810193563817646734, -1.199719254218452047 ) ) ;
#40720=CARTESIAN_POINT ( 'NONE',  ( 6.346625304528514810, 6.577020074804287297, 0.000000000000000000 ) ) ;
#40729=CARTESIAN_POINT ( 'NONE',  ( 3.901714345682657292, 7.774026846596938434, 0.7998128361456271485 ) ) ;
#40732=CARTESIAN_POINT ( 'NONE',  ( -3.006876207180748217, 6.730049018344652190, -0.7998128361456481317 ) ) ;
#40747=CARTESIAN_POINT ( 'NONE',  ( 5.204350862799327793, 7.165104988056252289, -1.599625672291281386 ) ) ;
#40754=VERTEX_POINT ( 'NONE', #201586 ) ;
#40756=CARTESIAN_POINT ( 'NONE',  ( -5.915100157312088491, 10.12297696016459092, -0.7998128361456362523 ) ) ;
#40761=CARTESIAN_POINT ( 'NONE',  ( 6.073126464278658432, 6.050012061272033392, 0.000000000000000000 ) ) ;
#40769=AXIS2_PLACEMENT_3D ( 'NONE', #143917, #209913, #193676 ) ;
#40774=CARTESIAN_POINT ( 'NONE',  ( 7.187230829020130329, 7.557726520044554697, 0.7216878364870267237 ) ) ;
#40775=CARTESIAN_POINT ( 'NONE',  ( -3.187575512988701565, 6.732938841879847480, 0.000000000000000000 ) ) ;
#40776=CARTESIAN_POINT ( 'NONE',  ( -5.798046968499580345, 6.793418213784815585, 1.199719254218452935 ) ) ;
#40787=CARTESIAN_POINT ( 'NONE',  ( 6.692885107001518286, 7.837396042037102717, -1.199719254218452047 ) ) ;
#40789=CARTESIAN_POINT ( 'NONE',  ( 6.554440917563797875, 6.611545590104705994, -0.7998128361456481317 ) ) ;
#40790=CARTESIAN_POINT ( 'NONE',  ( 4.213551878797002992, 8.137837301896977849, 0.000000000000000000 ) ) ;
#40793=CARTESIAN_POINT ( 'NONE',  ( 7.849244587668864348, 8.122149871893999062, 0.7998128361456291469 ) ) ;
#40807=VERTEX_POINT ( 'NONE', #65195 ) ;
#40811=CARTESIAN_POINT ( 'NONE',  ( 5.571474780572990504, 5.464751763615448787, 0.7998128361456352531 ) ) ;
#40815=CARTESIAN_POINT ( 'NONE',  ( 5.273195401072370281, 5.116759154198018855, -0.7998128361456481317 ) ) ;
#40820=CARTESIAN_POINT ( 'NONE',  ( 7.679767667498067496, 7.924426798361372093, 0.000000000000000000 ) ) ;
#40824=CARTESIAN_POINT ( 'NONE',  ( 5.478903473698239601, 7.485416367438324059, -1.443375672974078761 ) ) ;
#40827=CARTESIAN_POINT ( 'NONE',  ( -5.173318132066234476, 8.193232366456022930, -1.199719254218453823 ) ) ;
#40829=CARTESIAN_POINT ( 'NONE',  ( 5.578253857379852576, 5.472660686556754861, -0.7998128361456481317 ) ) ;
#40830=VERTEX_POINT ( 'NONE', #33778 ) ;
#40839=CARTESIAN_POINT ( 'NONE',  ( -5.307090785106547415, 5.156303768904543894, -0.7998128361456362523 ) ) ;
#40850=CARTESIAN_POINT ( 'NONE',  ( -0.1054627972275563597, 3.385846599571565640, -2.076146368081344118 ) ) ;
#40871=CARTESIAN_POINT ( 'NONE',  ( 4.936577329151614180, 4.931964103531220722, -0.7216878364870458196 ) ) ;
#40878=CARTESIAN_POINT ( 'NONE',  ( 8.025500584646550806, 8.327781868367935658, 0.000000000000000000 ) ) ;
#40890=CARTESIAN_POINT ( 'NONE',  ( -7.123883369337781879, 7.275895117174344229, 0.7998128361456341429 ) ) ;
#40893=CARTESIAN_POINT ( 'NONE',  ( 6.170369307550816806, 9.252495721234380355, 1.082531754730549967 ) ) ;
#40901=CARTESIAN_POINT ( 'NONE',  ( -3.962726036944197894, 7.845207153068690431, -0.7998128361456481317 ) ) ;
#40904=CARTESIAN_POINT ( 'NONE',  ( 7.065207446497155708, 9.336104335703744539, 0.000000000000000000 ) ) ;
#40910=CARTESIAN_POINT ( 'NONE',  ( -4.634908411025374875, 6.500755460986618495, 1.599625672291263179 ) ) ;
#40933=CARTESIAN_POINT ( 'NONE',  ( -7.130662446144611977, 7.283804040115648526, 0.000000000000000000 ) ) ;
#40934=CARTESIAN_POINT ( 'NONE',  ( -4.248501033035892327, 6.049946853332221153, -1.599625672291271394 ) ) ;
#40958=CARTESIAN_POINT ( 'NONE',  ( -4.444040490229335560, 8.406740681901359480, 0.7998128361456352531 ) ) ;
#40960=ORIENTED_EDGE ( 'NONE', *, *, #68201, .F. ) ;
#40968=CARTESIAN_POINT ( 'NONE',  ( 5.831415467209187575, 9.817418788470464008, 0.000000000000000000 ) ) ;
#40975=CARTESIAN_POINT ( 'NONE',  ( -4.828904602364790577, 7.233969404134618308, 1.215374634475984594 ) ) ;
#40979=CARTESIAN_POINT ( 'NONE',  ( 5.408776937209000657, 5.274937613024121674, 0.7998128361456352531 ) ) ;
#40986=CARTESIAN_POINT ( 'NONE',  ( 5.688527969385528849, 8.794310509995222347, -1.199719254218452047 ) ) ;
#40988=CARTESIAN_POINT ( 'NONE',  ( 6.313256805818848960, 7.394496357324014113, 1.199719254218452047 ) ) ;
#41001=AXIS2_PLACEMENT_3D ( 'NONE', #16960, #149115, #696 ) ;
#41002=CARTESIAN_POINT ( 'NONE',  ( 6.307155384238837037, 6.868572428096745064, 0.7081091520576547893 ) ) ;
#41004=CARTESIAN_POINT ( 'NONE',  ( 6.400857919427532572, 6.640291458853147866, -0.7216878364870458196 ) ) ;
#41013=CARTESIAN_POINT ( 'NONE',  ( -4.821859908315634158, 5.654533310236863564, 1.199719254218452935 ) ) ;
#41024=CARTESIAN_POINT ( 'NONE',  ( -5.953438849732214599, 6.118302544208584770, 0.7216878364870257245 ) ) ;
#41027=CARTESIAN_POINT ( 'NONE',  ( 7.666209513884374438, 7.908608952478760834, 0.7998128361456281477 ) ) ;
#41028=CARTESIAN_POINT ( 'NONE',  ( 5.069834057255440563, 4.910074306249716969, -0.2341815111036758823 ) ) ;
#41044=CARTESIAN_POINT ( 'NONE',  ( 6.703580607314123085, 6.785541894813420072, 0.000000000000000000 ) ) ;
#41058=AXIS2_PLACEMENT_3D ( 'NONE', #199024, #183865, #100485 ) ;
#41064=CARTESIAN_POINT ( 'NONE',  ( -5.250750630242457362, 9.347902511916677426, 0.000000000000000000 ) ) ;
#41069=CARTESIAN_POINT ( 'NONE',  ( -6.496151039430258400, 6.761311432142845135, -0.1280508955800782056 ) ) ;
#41077=CARTESIAN_POINT ( 'NONE',  ( 4.572363442555127833, 8.499999999999996447, 0.3169179603640607246 ) ) ;
#41087=CARTESIAN_POINT ( 'NONE',  ( 5.397554552016228691, 5.469770863539975991, 0.7216878364870328300 ) ) ;
#41091=CARTESIAN_POINT ( 'NONE',  ( -6.474900878978163021, 9.711745571186627402, -1.199719254218452047 ) ) ;
#41093=CARTESIAN_POINT ( 'NONE',  ( 6.393551957296131683, 9.616838495890963401, 1.199719254218452047 ) ) ;
#41096=CARTESIAN_POINT ( 'NONE',  ( -5.804299160426249493, 5.944306240018289778, -0.7216878364870338292 ) ) ;
#41108=CARTESIAN_POINT ( 'NONE',  ( -5.926322542504877333, 7.047036066744706950, -1.082531754730549967 ) ) ;
#41125=EDGE_LOOP ( 'NONE', ( #107040, #189646, #8415, #127939, #195716, #131393 ) ) ;
#41129=CARTESIAN_POINT ( 'NONE',  ( 5.174371902270911150, 6.065797303184739420, 1.199719254218452047 ) ) ;
#41134=LINE ( 'NONE', #90945, #168764 ) ;
#41142=CARTESIAN_POINT ( 'NONE',  ( -7.458393901293492334, 7.874083437696761223, 0.7216878364870317197 ) ) ;
#41145=CARTESIAN_POINT ( 'NONE',  ( 6.770317605177710085, 8.992066187497757213, 1.599625672291268286 ) ) ;
#41160=CARTESIAN_POINT ( 'NONE',  ( 5.063044020060520900, 4.871582543017558109, 0.7998128361456352531 ) ) ;
#41162=CARTESIAN_POINT ( 'NONE',  ( -4.340018570150318666, 6.156717313299049366, -1.443375672974066548 ) ) ;
#41164=DIRECTION ( 'NONE',  ( 1.000000000000000000, 0.000000000000000000, 0.000000000000000000 ) ) ;
#41179=EDGE_LOOP ( 'NONE', ( #96764, #54625, #15237, #158376, #197281 ) ) ;
#41194=CARTESIAN_POINT ( 'NONE',  ( -6.095272577795516789, 9.268845886473535245, 1.199719254218452047 ) ) ;
#41197=CARTESIAN_POINT ( 'NONE',  ( -4.749098946536820520, 8.762642214260091933, 0.7998128361456281477 ) ) ;
#41202=CARTESIAN_POINT ( 'NONE',  ( -6.034787771414192648, 9.094317262408276648, 1.082531754730549967 ) ) ;
#41205=CARTESIAN_POINT ( 'NONE',  ( -4.329849954717889915, 6.144853928627882489, 1.599625672291270506 ) ) ;
#41208=CARTESIAN_POINT ( 'NONE',  ( -7.075376061485238566, 9.347967719856493218, 1.599625672291269396 ) ) ;
#41217=CARTESIAN_POINT ( 'NONE',  ( -5.745623237141265882, 9.925253886631958622, 0.7998128361456291469 ) ) ;
#41219=CARTESIAN_POINT ( 'NONE',  ( 5.528015674651411970, 7.440572265265038787, -1.248273786418591103 ) ) ;
#41220=EDGE_CURVE ( 'NONE', #100853, #203895, #185806, .T. ) ;
#41223=CARTESIAN_POINT ( 'NONE',  ( 4.496171506534474283, 8.048216686630640382, 2.444650791391935307 ) ) ;
#41225=CARTESIAN_POINT ( 'NONE',  ( 2.898410978271408922, 6.603506251283770112, -0.7998128361456362523 ) ) ;
#41234=CARTESIAN_POINT ( 'NONE',  ( -6.237633190739009237, 9.434933268240943249, 1.199719254218452047 ) ) ;
#41246=CARTESIAN_POINT ( 'NONE',  ( 6.831329296439236032, 9.063246493969506545, -1.599625672291267398 ) ) ;
#41261=CARTESIAN_POINT ( 'NONE',  ( 6.599791786788117953, 6.770233575417231364, 0.1470628079319712123 ) ) ;
#41263=CARTESIAN_POINT ( 'NONE',  ( -4.082413651046300274, 6.816547455312373494, 1.082531754730549967 ) ) ;
#41266=EDGE_CURVE ( 'NONE', #56668, #118760, #61858, .T. ) ;
#41289=VERTEX_POINT ( 'NONE', #105678 ) ;
#41293=CARTESIAN_POINT ( 'NONE',  ( 8.014278199453778839, 8.522615118883788199, 0.000000000000000000 ) ) ;
#41297=ORIENTED_EDGE ( 'NONE', *, *, #193885, .F. ) ;
#41312=CARTESIAN_POINT ( 'NONE',  ( -4.471156797456668386, 8.438376373666578445, -0.7998128361456362523 ) ) ;
#41326=CARTESIAN_POINT ( 'NONE',  ( 3.898851692381625877, 6.706354853490643642, -1.199719254218452047 ) ) ;
#41328=CARTESIAN_POINT ( 'NONE',  ( 7.960045584554727327, 8.459343734834927631, 0.7216878364870267237 ) ) ;
#41339=CARTESIAN_POINT ( 'NONE',  ( 5.176795123377851304, 7.746134302493202561, 1.185296789734613387 ) ) ;
#41359=CARTESIAN_POINT ( 'NONE',  ( -3.983063267364693960, 7.868933921892603323, -0.7998128361456481317 ) ) ;
#41361=CARTESIAN_POINT ( 'NONE',  ( 5.923986774528332333, 5.876015756563318426, -0.7998128361456481317 ) ) ;
#41364=CARTESIAN_POINT ( 'NONE',  ( -6.286140498591554326, 7.362860665558790707, 1.199719254218452047 ) ) ;
#41367=CARTESIAN_POINT ( 'NONE',  ( 6.713222337422018349, 7.861122810861019161, -1.199719254218452047 ) ) ;
#41373=CARTESIAN_POINT ( 'NONE',  ( -5.072456052330698739, 7.961014115122230450, -1.198640345919316674 ) ) ;
#41382=CARTESIAN_POINT ( 'NONE',  ( -3.973948422136968084, 7.650373902552835226, -0.7216878364870458196 ) ) ;
#41389=CARTESIAN_POINT ( 'NONE',  ( 5.397554552016216256, 7.390509292142662723, 1.443375672974065660 ) ) ;
#41393=CARTESIAN_POINT ( 'NONE',  ( -7.259464905474441565, 7.434073576000447048, -0.7998128361456362523 ) ) ;
#41402=CARTESIAN_POINT ( 'NONE',  ( -3.634994582239682526, 6.294558541704648569, 1.082531754730549967 ) ) ;
#41407=EDGE_CURVE ( 'NONE', #158170, #36876, #182906, .T. ) ;
#41413=CARTESIAN_POINT ( 'NONE',  ( 4.929271367020211514, 7.908511140569038922, 1.199719254218452047 ) ) ;
#41435=CARTESIAN_POINT ( 'NONE',  ( -4.814553946628611136, 8.631080347793099961, 0.000000000000000000 ) ) ;
#41449=CARTESIAN_POINT ( 'NONE',  ( 3.147653791585717453, 8.999999999999998224, -2.420000000000002149 ) ) ;
#41460=CARTESIAN_POINT ( 'NONE',  ( -6.770317605177755382, 8.992066187497757213, 1.599625672291269396 ) ) ;
#41461=CARTESIAN_POINT ( 'NONE',  ( -5.029148636026397945, 4.832037928311032182, 0.7998128361456281477 ) ) ;
#41466=CARTESIAN_POINT ( 'NONE',  ( -3.688700311369816909, 6.461178242310183784, -1.199719254218450271 ) ) ;
#41470=VERTEX_POINT ( 'NONE', #155464 ) ;
#41474=CARTESIAN_POINT ( 'NONE',  ( -4.516801452008150086, 5.298631777878131111, 1.199719254218452935 ) ) ;
#41476=CARTESIAN_POINT ( 'NONE',  ( 5.595231165798738360, 7.497995327707586810, -1.335214257040851615 ) ) ;
#41480=CARTESIAN_POINT ( 'NONE',  ( 4.203910148689107729, 7.062256385849379647, -1.199719254218448494 ) ) ;
#41486=CARTESIAN_POINT ( 'NONE',  ( -7.598418745816086783, 7.829519723065708092, 0.000000000000000000 ) ) ;
#41489=CARTESIAN_POINT ( 'NONE',  ( -4.014095998097799267, 6.840806543492835345, -1.199719254218450271 ) ) ;
#41493=CARTESIAN_POINT ( 'NONE',  ( 6.197485614778188712, 6.403023770095574108, -0.7216878364870458196 ) ) ;
#41494=CARTESIAN_POINT ( 'NONE',  ( -6.265276382846530545, 6.482112999508623297, 0.000000000000000000 ) ) ;
#41500=CARTESIAN_POINT ( 'NONE',  ( 3.054329744828568227, 6.785411478933790264, 0.000000000000000000 ) ) ;
#41511=CARTESIAN_POINT ( 'NONE',  ( 4.978670620768666844, 8.057607364700732688, 1.103355461389814662 ) ) ;
#41521=CARTESIAN_POINT ( 'NONE',  ( 7.198453214212898743, 7.362893269528701268, 0.7998128361456291469 ) ) ;
#41531=CARTESIAN_POINT ( 'NONE',  ( 6.003728048595398548, 7.077753126805482076, 1.059392881431284961 ) ) ;
#41539=CARTESIAN_POINT ( 'NONE',  ( 6.047819040147648373, 9.213483425884394507, 1.199719254218452047 ) ) ;
#41543=CARTESIAN_POINT ( 'NONE',  ( -4.640257700270903563, 8.337993449908045918, -0.3781808898682629261 ) ) ;
#41552=CARTESIAN_POINT ( 'NONE',  ( -7.795011973214244883, 8.058878488363559356, 0.7998128361456341429 ) ) ;
#41556=CARTESIAN_POINT ( 'NONE',  ( -3.712022485150084705, 7.355926397811426654, 0.5818110939905510870 ) ) ;
#41565=CARTESIAN_POINT ( 'NONE',  ( 7.849244587668864348, 8.122149871893999062, 0.7998128361456291469 ) ) ;
#41571=CARTESIAN_POINT ( 'NONE',  ( -7.553300976144787349, 8.945177572657957654, -1.082531754730549967 ) ) ;
#41573=CARTESIAN_POINT ( 'NONE',  ( 4.146814880933355596, 5.931313009212638931, 1.599625672291261402 ) ) ;
#41576=CARTESIAN_POINT ( 'NONE',  ( 3.892599500454932304, 7.555466827257172113, 0.7216878364870257245 ) ) ;
#41594=CARTESIAN_POINT ( 'NONE',  ( -6.455090533882201775, 8.624301270986276080, -1.443375672974066548 ) ) ;
#41595=CARTESIAN_POINT ( 'NONE',  ( 7.865138509703455405, 8.348618814175074121, -0.7216878364870317197 ) ) ;
#41607=CARTESIAN_POINT ( 'NONE',  ( -5.960744811863571968, 6.983232364376142698, 1.199719254218452935 ) ) ;
#41608=CARTESIAN_POINT ( 'NONE',  ( -4.716257332707368910, 6.595662536282280719, -1.599625672291271394 ) ) ;
#41610=CARTESIAN_POINT ( 'NONE',  ( 6.604230223188150894, 9.758666789477915771, -1.082531754730548412 ) ) ;
#41620=CARTESIAN_POINT ( 'NONE',  ( -5.733196416021622888, 7.293175961584016598, -1.208997762321398550 ) ) ;
#41625=CARTESIAN_POINT ( 'NONE',  ( 3.919715808126649659, 7.587102519540811940, 0.000000000000000000 ) ) ;
#41631=CARTESIAN_POINT ( 'NONE',  ( -5.444481204339554736, 8.509589284108232121, 1.199719254218454489 ) ) ;
#41644=CARTESIAN_POINT ( 'NONE',  ( 6.066347387471824781, 6.042103138330730872, -0.7998128361456481317 ) ) ;
#41683=CARTESIAN_POINT ( 'NONE',  ( 5.560252395380198998, 9.501061871336672127, 0.7216878364870317197 ) ) ;
#41688=CARTESIAN_POINT ( 'NONE',  ( 7.661766205054107992, 8.111351125417501251, -0.7216878364870317197 ) ) ;
#41712=CARTESIAN_POINT ( 'NONE',  ( -5.503684012504701961, 5.385662534202396934, 0.000000000000000000 ) ) ;
#41714=CARTESIAN_POINT ( 'NONE',  ( 5.194182247366869731, 7.153241603385088965, 1.443375672974064550 ) ) ;
#41720=CARTESIAN_POINT ( 'NONE',  ( -5.113360211009450040, 5.994616996712990975, -1.199719254218453823 ) ) ;
#41725=CARTESIAN_POINT ( 'NONE',  ( -7.119440060951841787, 7.478637290631501067, 0.000000000000000000 ) ) ;
#41732=CARTESIAN_POINT ( 'NONE',  ( -5.093022980588950865, 5.970890227889075419, -1.199719254218453823 ) ) ;
#41745=CARTESIAN_POINT ( 'NONE',  ( -4.014622883422329203, 6.737458226417744278, -1.082531754730546636 ) ) ;
#41747=CARTESIAN_POINT ( 'NONE',  ( -6.102578539482539810, 6.292298848917299736, 0.000000000000000000 ) ) ;
#41748=CARTESIAN_POINT ( 'NONE',  ( 5.013482942003290255, 9.071090208970993274, -0.7998128361456481317 ) ) ;
#41749=CARTESIAN_POINT ( 'NONE',  ( -4.606738333593328072, 8.596554832492683929, 0.7998128361456281477 ) ) ;
#41769=CARTESIAN_POINT ( 'NONE',  ( 7.686546744304875389, 7.932335721302671949, 0.7998128361456291469 ) ) ;
#41776=CARTESIAN_POINT ( 'NONE',  ( -2.973437390567118310, 6.691037065628751002, -0.02693349654502708024 ) ) ;
#41800=CARTESIAN_POINT ( 'NONE',  ( -1.843739406749240750, 8.928444911142053186, -0.7749999999999996891 ) ) ;
#41806=ADVANCED_FACE ( 'NONE', ( #100061 ), #183436, .T. ) ;
#41808=CARTESIAN_POINT ( 'NONE',  ( 5.574337433874081427, 6.532423756721743580, -1.199719254218452047 ) ) ;
#41814=CARTESIAN_POINT ( 'NONE',  ( -6.916067756302494374, 7.241369601873926420, 0.000000000000000000 ) ) ;
#41825=CARTESIAN_POINT ( 'NONE',  ( 2.925527285498711549, 6.635141943048991742, 0.7998128361456281477 ) ) ;
#41826=CARTESIAN_POINT ( 'NONE',  ( 6.099189001301251523, 8.209082816308541197, 1.599625672291268286 ) ) ;
#41838=CARTESIAN_POINT ( 'NONE',  ( 4.064412189046650248, 7.963840997188264659, 0.7998128361456271485 ) ) ;
#41849=CARTESIAN_POINT ( 'NONE',  ( 6.699137298928153683, 7.948653282571920720, 1.082531754730549967 ) ) ;
#41851=CARTESIAN_POINT ( 'NONE',  ( -3.011319516011047082, 6.527306845405913549, 0.7216878364870328300 ) ) ;
#41852=CARTESIAN_POINT ( 'NONE',  ( -5.966470118465691641, 9.118576350588734059, -1.199719254218452047 ) ) ;
#41856=( BOUNDED_SURFACE ( )  B_SPLINE_SURFACE ( 1, 2, ( 
 ( #77530, #144715, #159854, #209646, #128514, #14649, #81798, #65520, #163068, #94876, #80743, #210727, #45063, #127448, #146831, #62353, #504, #148931, #53559, #66572, #153194, #152136, #37306, #17832, #199792, #67637, #84988, #86059, #2643, #50365, #181420, #132714, #115429, #82855, #150006, #34105, #1576, #166242, #165177, #116488, #51437, #136959, #100177, #99128, #83915, #184609, #3704, #49312, #169442, #87124, #16771, #198719, #133784, #35158, #183551, #118622, #119692, #68717, #33050, #69780, #182477, #167317, #117557, #101235, #18904, #151079, #134838, #200841, #135889, #4766, #52492, #36226, #102305, #201907, #185677, #168378, #21027, #19975, #103380, #70843, #6915, #5845, #54626, #123990, #23167, #107718, #205122, #120773, #108785, #170503, #206200, #202986, #204040, #189957, #157484, #56765, #7995, #139095, #106633, #174811, #22086, #173745, #88197, #26387, #74087, #154271, #105536, #104456, #71916, #25322, #172662, #24237, #156408, #140178, #138025, #186753, #41607, #57828, #72992, #55689, #121845, #171570, #38375, #187816, #122931, #91423, #191010, #75153, #90339, #39442, #9079, #89283, #155331, #188888, #40529, #141263, #207271, #58902, #125055, #42678, #92499, #158538, #10135, #76210, #78342, #160670, #177996, #179063, #95695, #143390, #59961, #27457, #208330, #175869, #28535, #127193, #94627, #44810, #43742, #209388, #144465, #15460, #193160, #192076, #110914, #63166, #96765, #142320, #48013, #180122, #109855, #93555, #12265, #128266, #62107, #211531, #146584, #161750, #126116, #162816, #61032, #45872, #210469, #159599, #194228, #111994, #176920, #11197, #14393, #31747, #29610, #13341, #79416, #80484, #212601, #145533, #114130, #129332, #77278, #195308, #46939, #113057, #30682, #64239, #130383, #196373, #97820, #163885, #2393, #201665, #69535, #53312, #164928, #200601, #147629, #115181, #103135, #19733, #169193, #51184, #18663, #150831, #16520, #99935, #33854, #68472, #182230, #1333, #32801, #84743, #149756, #181176, #134600, #52248, #67394, #199542, #117307, #132473, #257, #183303, #81546 ),
 ( #165997, #198475, #133535, #102066, #35985, #17582, #119444, #83665, #82603, #34910, #100982, #98875, #50120, #116241, #167071, #135642, #168131, #185432, #118375, #37052, #213647, #184363, #85812, #151891, #3466, #65273, #131419, #49061, #197419, #148688, #66328, #7745, #189706, #22919, #40275, #171323, #138849, #207020, #202737, #205955, #54388, #141012, #106385, #120526, #137782, #136712, #104208, #139928, #204866, #56521, #188644, #172408, #186505, #152948, #156164, #23996, #105287, #170255, #38136, #203800, #4523, #86881, #39195, #57588, #8827, #107469, #122681, #5589, #73832, #71668, #21840, #87948, #89034, #20786, #154022, #55446, #25071, #121598, #124805, #123745, #74904, #187570, #155089, #6675, #90099, #41359, #173495, #72752, #70598, #91173, #157232, #58651, #190764, #42428, #108533, #125870, #94374, #195046, #30428, #12020, #47762, #174563, #13080, #59710, #176668, #175617, #158298, #142069, #92252, #28280, #208083, #10943, #191829, #144219, #96514, #193970, #162563, #130135, #128016, #212341, #79160, #192896, #112802, #44552, #14135, #145276, #80228, #45618, #159346, #61849, #111735, #110668, #177741, #60780, #9889, #43492, #160415, #29356, #26139, #146326, #78092, #62905, #77017, #75966, #129075, #178815, #143146, #109612, #46684, #63982, #209141, #126939, #211282, #196124, #210213, #95450, #27204, #93311, #161500, #81300, #35727, #115986, #51996, #7, #113876, #31496, #67142, #147377, #101803, #100734, #99675, #82348, #167872, #19470, #97571, #50927, #1077, #163628, #213404, #85547, #151637, #197170, #18407, #179871, #65025, #135387, #118122, #201408, #83412, #117052, #183049, #48806, #132214, #66072, #34664, #198223, #33605, #131180, #166813, #181974, #114923, #84483, #150573, #165745, #17331, #149494, #164679, #32543, #133276, #15209, #16264, #180922, #98618, #199284, #2135, #148439, #3204, #68211, #69273, #134342, #49859, #200347, #184107, #90905, #172146, #71408, #205685, #137520, #189449, #106123, #41091, #138584, #37872, #154826, #72483, #203537, #204607, #153757, #102875, #86618, #38940 ) ),
 .UNSPECIFIED., .F., .F., .T. ) 
 B_SPLINE_SURFACE_WITH_KNOTS ( ( 2, 2 ),
 ( 3, 2, 2, 2, 2, 2, 2, 2, 2, 2, 2, 2, 2, 2, 2, 2, 2, 2, 2, 2, 2, 2, 2, 2, 2, 2, 2, 2, 2, 2, 2, 2, 2, 2, 2, 2, 2, 2, 2, 2, 2, 2, 2, 2, 2, 2, 2, 2, 2, 2, 2, 2, 2, 2, 2, 2, 2, 2, 2, 2, 2, 2, 2, 2, 2, 2, 2, 2, 2, 2, 2, 2, 2, 2, 2, 2, 2, 2, 2, 2, 2, 2, 2, 2, 2, 2, 2, 2, 2, 2, 2, 2, 2, 2, 2, 2, 2, 2, 2, 2, 2, 2, 2, 2, 2, 2, 2, 2, 2, 2, 2, 2, 2, 2, 2, 2, 2, 2, 2, 2, 3 ),
 ( 0.000000000000000000, 1.000000000000000000 ),
 ( 0.000000000000000000, 0.008333333333333333218, 0.01666666666666666644, 0.02500000000000000139, 0.03333333333333333287, 0.04166666666666666435, 0.05000000000000000278, 0.05833333333333333426, 0.06666666666666666574, 0.07499999999999999722, 0.08333333333333332871, 0.09166666666666666019, 0.1000000000000000056, 0.1083333333333333370, 0.1166666666666666685, 0.1250000000000000000, 0.1333333333333333315, 0.1416666666666666630, 0.1499999999999999944, 0.1583333333333333259, 0.1666666666666666574, 0.1749999999999999889, 0.1833333333333333204, 0.1916666666666666796, 0.2000000000000000111, 0.2083333333333333426, 0.2166666666666666741, 0.2250000000000000056, 0.2333333333333333370, 0.2416666666666666685, 0.2500000000000000000, 0.2583333333333333592, 0.2666666666666666630, 0.2750000000000000222, 0.2833333333333333259, 0.2916666666666666852, 0.2999999999999999889, 0.3083333333333333481, 0.3166666666666666519, 0.3250000000000000111, 0.3333333333333333148, 0.3416666666666666741, 0.3499999999999999778, 0.3583333333333333370, 0.3666666666666666408, 0.3750000000000000000, 0.3833333333333333592, 0.3916666666666666630, 0.4000000000000000222, 0.4083333333333333259, 0.4166666666666666852, 0.4249999999999999889, 0.4333333333333333481, 0.4416666666666666519, 0.4500000000000000111, 0.4583333333333333148, 0.4666666666666666741, 0.4749999999999999778, 0.4833333333333333370, 0.4916666666666666408, 0.5000000000000000000, 0.5083333333333333037, 0.5166666666666667185, 0.5250000000000000222, 0.5333333333333333259, 0.5416666666666666297, 0.5500000000000000444, 0.5583333333333333481, 0.5666666666666666519, 0.5749999999999999556, 0.5833333333333333703, 0.5916666666666666741, 0.5999999999999999778, 0.6083333333333332815, 0.6166666666666666963, 0.6250000000000000000, 0.6333333333333333037, 0.6416666666666667185, 0.6500000000000000222, 0.6583333333333333259, 0.6666666666666666297, 0.6750000000000000444, 0.6833333333333333481, 0.6916666666666666519, 0.6999999999999999556, 0.7083333333333333703, 0.7166666666666666741, 0.7249999999999999778, 0.7333333333333332815, 0.7416666666666666963, 0.7500000000000000000, 0.7583333333333333037, 0.7666666666666667185, 0.7750000000000000222, 0.7833333333333333259, 0.7916666666666666297, 0.8000000000000000444, 0.8083333333333333481, 0.8166666666666666519, 0.8249999999999999556, 0.8333333333333333703, 0.8416666666666666741, 0.8499999999999999778, 0.8583333333333332815, 0.8666666666666666963, 0.8750000000000000000, 0.8833333333333333037, 0.8916666666666667185, 0.9000000000000000222, 0.9083333333333333259, 0.9166666666666666297, 0.9250000000000000444, 0.9333333333333333481, 0.9416666666666666519, 0.9499999999999999556, 0.9583333333333333703, 0.9666666666666666741, 0.9749999999999999778, 0.9833333333333332815, 0.9916666666666666963, 1.000000000000000000 ),
 .UNSPECIFIED. ) 
 GEOMETRIC_REPRESENTATION_ITEM ( )  RATIONAL_B_SPLINE_SURFACE ( (
 ( 1.000000000000000000, 0.8660254037844387076, 1.000000000000000000, 0.8660254037844387076, 1.000000000000000000, 0.8660254037844387076, 1.000000000000000000, 0.8660254037844387076, 1.000000000000000000, 0.8660254037844387076, 1.000000000000000000, 0.8660254037844387076, 1.000000000000000000, 0.8660254037844387076, 1.000000000000000000, 0.8660254037844387076, 1.000000000000000000, 0.8660254037844387076, 1.000000000000000000, 0.8660254037844387076, 1.000000000000000000, 0.8660254037844387076, 1.000000000000000000, 0.8660254037844387076, 1.000000000000000000, 0.8660254037844387076, 1.000000000000000000, 0.8660254037844387076, 1.000000000000000000, 0.8660254037844387076, 1.000000000000000000, 0.8660254037844387076, 1.000000000000000000, 0.8660254037844387076, 1.000000000000000000, 0.8660254037844387076, 1.000000000000000000, 0.8660254037844387076, 1.000000000000000000, 0.8660254037844387076, 1.000000000000000000, 0.8660254037844387076, 1.000000000000000000, 0.8660254037844387076, 1.000000000000000000, 0.8660254037844387076, 1.000000000000000000, 0.8660254037844387076, 1.000000000000000000, 0.8660254037844387076, 1.000000000000000000, 0.8660254037844387076, 1.000000000000000000, 0.8660254037844387076, 1.000000000000000000, 0.8660254037844387076, 1.000000000000000000, 0.8660254037844387076, 1.000000000000000000, 0.8660254037844387076, 1.000000000000000000, 0.8660254037844387076, 1.000000000000000000, 0.8660254037844387076, 1.000000000000000000, 0.8660254037844387076, 1.000000000000000000, 0.8660254037844387076, 1.000000000000000000, 0.8660254037844387076, 1.000000000000000000, 0.8660254037844387076, 1.000000000000000000, 0.8660254037844387076, 1.000000000000000000, 0.8660254037844387076, 1.000000000000000000, 0.8660254037844387076, 1.000000000000000000, 0.8660254037844387076, 1.000000000000000000, 0.8660254037844387076, 1.000000000000000000, 0.8660254037844387076, 1.000000000000000000, 0.8660254037844387076, 1.000000000000000000, 0.8660254037844387076, 1.000000000000000000, 0.8660254037844387076, 1.000000000000000000, 0.8660254037844387076, 1.000000000000000000, 0.8660254037844387076, 1.000000000000000000, 0.8660254037844387076, 1.000000000000000000, 0.8660254037844387076, 1.000000000000000000, 0.8660254037844387076, 1.000000000000000000, 0.8660254037844387076, 1.000000000000000000, 0.8660254037844387076, 1.000000000000000000, 0.8660254037844387076, 1.000000000000000000, 0.8660254037844387076, 1.000000000000000000, 0.8660254037844387076, 1.000000000000000000, 0.8660254037844387076, 1.000000000000000000, 0.8660254037844387076, 1.000000000000000000, 0.8660254037844387076, 1.000000000000000000, 0.8660254037844387076, 1.000000000000000000, 0.8660254037844387076, 1.000000000000000000, 0.8660254037844387076, 1.000000000000000000, 0.8660254037844387076, 1.000000000000000000, 0.8660254037844387076, 1.000000000000000000, 0.8660254037844387076, 1.000000000000000000, 0.8660254037844387076, 1.000000000000000000, 0.8660254037844387076, 1.000000000000000000, 0.8660254037844387076, 1.000000000000000000, 0.8660254037844387076, 1.000000000000000000, 0.8660254037844387076, 1.000000000000000000, 0.8660254037844387076, 1.000000000000000000, 0.8660254037844387076, 1.000000000000000000, 0.8660254037844387076, 1.000000000000000000, 0.8660254037844387076, 1.000000000000000000, 0.8660254037844387076, 1.000000000000000000, 0.8660254037844387076, 1.000000000000000000, 0.8660254037844387076, 1.000000000000000000, 0.8660254037844387076, 1.000000000000000000, 0.8660254037844387076, 1.000000000000000000, 0.8660254037844387076, 1.000000000000000000, 0.8660254037844387076, 1.000000000000000000, 0.8660254037844387076, 1.000000000000000000, 0.8660254037844387076, 1.000000000000000000, 0.8660254037844387076, 1.000000000000000000, 0.8660254037844387076, 1.000000000000000000, 0.8660254037844387076, 1.000000000000000000, 0.8660254037844387076, 1.000000000000000000, 0.8660254037844387076, 1.000000000000000000, 0.8660254037844387076, 1.000000000000000000, 0.8660254037844387076, 1.000000000000000000, 0.8660254037844387076, 1.000000000000000000, 0.8660254037844387076, 1.000000000000000000, 0.8660254037844387076, 1.000000000000000000, 0.8660254037844387076, 1.000000000000000000, 0.8660254037844387076, 1.000000000000000000, 0.8660254037844387076, 1.000000000000000000, 0.8660254037844387076, 1.000000000000000000, 0.8660254037844387076, 1.000000000000000000, 0.8660254037844387076, 1.000000000000000000, 0.8660254037844387076, 1.000000000000000000, 0.8660254037844387076, 1.000000000000000000, 0.8660254037844387076, 1.000000000000000000, 0.8660254037844387076, 1.000000000000000000, 0.8660254037844387076, 1.000000000000000000, 0.8660254037844387076, 1.000000000000000000, 0.8660254037844387076, 1.000000000000000000, 0.8660254037844387076, 1.000000000000000000, 0.8660254037844387076, 1.000000000000000000, 0.8660254037844387076, 1.000000000000000000, 0.8660254037844387076, 1.000000000000000000, 0.8660254037844387076, 1.000000000000000000, 0.8660254037844387076, 1.000000000000000000, 0.8660254037844387076, 1.000000000000000000, 0.8660254037844387076, 1.000000000000000000, 0.8660254037844387076, 1.000000000000000000, 0.8660254037844387076, 1.000000000000000000, 0.8660254037844387076, 1.000000000000000000, 0.8660254037844387076, 1.000000000000000000, 0.8660254037844387076, 1.000000000000000000, 0.8660254037844387076, 1.000000000000000000, 0.8660254037844387076, 1.000000000000000000),
 ( 1.000000000000000000, 0.8660254037844387076, 1.000000000000000000, 0.8660254037844387076, 1.000000000000000000, 0.8660254037844387076, 1.000000000000000000, 0.8660254037844387076, 1.000000000000000000, 0.8660254037844387076, 1.000000000000000000, 0.8660254037844387076, 1.000000000000000000, 0.8660254037844387076, 1.000000000000000000, 0.8660254037844387076, 1.000000000000000000, 0.8660254037844387076, 1.000000000000000000, 0.8660254037844387076, 1.000000000000000000, 0.8660254037844387076, 1.000000000000000000, 0.8660254037844387076, 1.000000000000000000, 0.8660254037844387076, 1.000000000000000000, 0.8660254037844387076, 1.000000000000000000, 0.8660254037844387076, 1.000000000000000000, 0.8660254037844387076, 1.000000000000000000, 0.8660254037844387076, 1.000000000000000000, 0.8660254037844387076, 1.000000000000000000, 0.8660254037844387076, 1.000000000000000000, 0.8660254037844387076, 1.000000000000000000, 0.8660254037844387076, 1.000000000000000000, 0.8660254037844387076, 1.000000000000000000, 0.8660254037844387076, 1.000000000000000000, 0.8660254037844387076, 1.000000000000000000, 0.8660254037844387076, 1.000000000000000000, 0.8660254037844387076, 1.000000000000000000, 0.8660254037844387076, 1.000000000000000000, 0.8660254037844387076, 1.000000000000000000, 0.8660254037844387076, 1.000000000000000000, 0.8660254037844387076, 1.000000000000000000, 0.8660254037844387076, 1.000000000000000000, 0.8660254037844387076, 1.000000000000000000, 0.8660254037844387076, 1.000000000000000000, 0.8660254037844387076, 1.000000000000000000, 0.8660254037844387076, 1.000000000000000000, 0.8660254037844387076, 1.000000000000000000, 0.8660254037844387076, 1.000000000000000000, 0.8660254037844387076, 1.000000000000000000, 0.8660254037844387076, 1.000000000000000000, 0.8660254037844387076, 1.000000000000000000, 0.8660254037844387076, 1.000000000000000000, 0.8660254037844387076, 1.000000000000000000, 0.8660254037844387076, 1.000000000000000000, 0.8660254037844387076, 1.000000000000000000, 0.8660254037844387076, 1.000000000000000000, 0.8660254037844387076, 1.000000000000000000, 0.8660254037844387076, 1.000000000000000000, 0.8660254037844387076, 1.000000000000000000, 0.8660254037844387076, 1.000000000000000000, 0.8660254037844387076, 1.000000000000000000, 0.8660254037844387076, 1.000000000000000000, 0.8660254037844387076, 1.000000000000000000, 0.8660254037844387076, 1.000000000000000000, 0.8660254037844387076, 1.000000000000000000, 0.8660254037844387076, 1.000000000000000000, 0.8660254037844387076, 1.000000000000000000, 0.8660254037844387076, 1.000000000000000000, 0.8660254037844387076, 1.000000000000000000, 0.8660254037844387076, 1.000000000000000000, 0.8660254037844387076, 1.000000000000000000, 0.8660254037844387076, 1.000000000000000000, 0.8660254037844387076, 1.000000000000000000, 0.8660254037844387076, 1.000000000000000000, 0.8660254037844387076, 1.000000000000000000, 0.8660254037844387076, 1.000000000000000000, 0.8660254037844387076, 1.000000000000000000, 0.8660254037844387076, 1.000000000000000000, 0.8660254037844387076, 1.000000000000000000, 0.8660254037844387076, 1.000000000000000000, 0.8660254037844387076, 1.000000000000000000, 0.8660254037844387076, 1.000000000000000000, 0.8660254037844387076, 1.000000000000000000, 0.8660254037844387076, 1.000000000000000000, 0.8660254037844387076, 1.000000000000000000, 0.8660254037844387076, 1.000000000000000000, 0.8660254037844387076, 1.000000000000000000, 0.8660254037844387076, 1.000000000000000000, 0.8660254037844387076, 1.000000000000000000, 0.8660254037844387076, 1.000000000000000000, 0.8660254037844387076, 1.000000000000000000, 0.8660254037844387076, 1.000000000000000000, 0.8660254037844387076, 1.000000000000000000, 0.8660254037844387076, 1.000000000000000000, 0.8660254037844387076, 1.000000000000000000, 0.8660254037844387076, 1.000000000000000000, 0.8660254037844387076, 1.000000000000000000, 0.8660254037844387076, 1.000000000000000000, 0.8660254037844387076, 1.000000000000000000, 0.8660254037844387076, 1.000000000000000000, 0.8660254037844387076, 1.000000000000000000, 0.8660254037844387076, 1.000000000000000000, 0.8660254037844387076, 1.000000000000000000, 0.8660254037844387076, 1.000000000000000000, 0.8660254037844387076, 1.000000000000000000, 0.8660254037844387076, 1.000000000000000000, 0.8660254037844387076, 1.000000000000000000, 0.8660254037844387076, 1.000000000000000000, 0.8660254037844387076, 1.000000000000000000, 0.8660254037844387076, 1.000000000000000000, 0.8660254037844387076, 1.000000000000000000, 0.8660254037844387076, 1.000000000000000000, 0.8660254037844387076, 1.000000000000000000, 0.8660254037844387076, 1.000000000000000000, 0.8660254037844387076, 1.000000000000000000, 0.8660254037844387076, 1.000000000000000000, 0.8660254037844387076, 1.000000000000000000, 0.8660254037844387076, 1.000000000000000000, 0.8660254037844387076, 1.000000000000000000, 0.8660254037844387076, 1.000000000000000000, 0.8660254037844387076, 1.000000000000000000, 0.8660254037844387076, 1.000000000000000000, 0.8660254037844387076, 1.000000000000000000, 0.8660254037844387076, 1.000000000000000000, 0.8660254037844387076, 1.000000000000000000, 0.8660254037844387076, 1.000000000000000000, 0.8660254037844387076, 1.000000000000000000, 0.8660254037844387076, 1.000000000000000000, 0.8660254037844387076, 1.000000000000000000, 0.8660254037844387076, 1.000000000000000000, 0.8660254037844387076, 1.000000000000000000) ) ) 
 REPRESENTATION_ITEM ( '' )  SURFACE ( )  );
#41862=CARTESIAN_POINT ( 'NONE',  ( 5.169401708560450004, 9.252995436621013425, 0.000000000000000000 ) ) ;
#41864=CARTESIAN_POINT ( 'NONE',  ( 4.369470645354133431, 8.319742529546998000, 0.7998128361456271485 ) ) ;
#41865=CARTESIAN_POINT ( 'NONE',  ( 6.526270840131753737, 8.707344961610770540, -1.599625672291283607 ) ) ;
#41868=CARTESIAN_POINT ( 'NONE',  ( 7.361151057576892143, 7.552707420120024828, 0.7998128361456291469 ) ) ;
#41882=VERTEX_POINT ( 'NONE', #117441 ) ;
#41886=CARTESIAN_POINT ( 'NONE',  ( 4.899292406491845497, 6.809203455697518947, -1.599625672291273171 ) ) ;
#41890=CARTESIAN_POINT ( 'NONE',  ( 3.888156192069020634, 7.758209000714329839, 1.040834085586084257E-14 ) ) ;
#41895=CARTESIAN_POINT ( 'NONE',  ( 6.587282531393223728, 8.778525268082516320, 1.599625672291268286 ) ) ;
#41900=CARTESIAN_POINT ( 'NONE',  ( 6.265276383290871109, 7.442482214328385304, -1.082531754730548412 ) ) ;
#41902=CARTESIAN_POINT ( 'NONE',  ( -6.168033539574333979, 6.160736982450306876, 0.7998128361456281477 ) ) ;
#41903=CARTESIAN_POINT ( 'NONE',  ( 4.797606254389322089, 6.690569611577942943, 1.599625672291268286 ) ) ;
#41910=CARTESIAN_POINT ( 'NONE',  ( -5.876765390786736099, 6.215699210118543760, -0.5395277504373359179 ) ) ;
#41913=CARTESIAN_POINT ( 'NONE',  ( -3.637330350216213759, 7.465578851886037093, -0.7998128361456481317 ) ) ;
#41942=CARTESIAN_POINT ( 'NONE',  ( 3.716343503921665459, 6.389465617000312569, -1.082531754730549967 ) ) ;
#41948=CARTESIAN_POINT ( 'NONE',  ( 4.868786560638896255, 5.813244087901094481, 1.082531754730549078 ) ) ;
#41959=CARTESIAN_POINT ( 'NONE',  ( -6.798487682609798632, 6.896266815991691779, 0.7998128361456341429 ) ) ;
#41961=CARTESIAN_POINT ( 'NONE',  ( 5.682275777458829502, 9.643422483761748154, 0.7216878364870317197 ) ) ;
#41972=CARTESIAN_POINT ( 'NONE',  ( -5.123001941117347080, 7.070197912760590064, 1.599625672291263179 ) ) ;
#41979=CARTESIAN_POINT ( 'NONE',  ( -3.038435823238377687, 6.558942537171132514, -0.7216878364870458196 ) ) ;
#41984=CARTESIAN_POINT ( 'NONE',  ( -5.496904935697871863, 5.377753611261092637, 0.7998128361456281477 ) ) ;
#42008=CARTESIAN_POINT ( 'NONE',  ( -7.144220599758281054, 7.299621885998258897, 0.7998128361456341429 ) ) ;
#42010=CARTESIAN_POINT ( 'NONE',  ( -5.191846479390389568, 5.021852078902356631, 0.7998128361456281477 ) ) ;
#42011=ORIENTED_EDGE ( 'NONE', *, *, #81569, .F. ) ;
#42019=CARTESIAN_POINT ( 'NONE',  ( -5.994696786504495556, 7.186261032347766253, -1.212264510017725394 ) ) ;
#42026=DIRECTION ( 'NONE',  ( 0.7978120914393087570, -0.6029061840396366945, 2.113174082329822227E-15 ) ) ;
#42033=CARTESIAN_POINT ( 'NONE',  ( -6.791708605802965870, 6.888357893050385705, -0.7998128361456362523 ) ) ;
#42035=EDGE_LOOP ( 'NONE', ( #60899, #11888, #104877, #63561, #55660, #103365, #43012, #69389 ) ) ;
#42044=CARTESIAN_POINT ( 'NONE',  ( 2.972313222866368676, 6.545497292499366182, 0.5012468031770876964 ) ) ;
#42058=CARTESIAN_POINT ( 'NONE',  ( 6.444921918449731280, 8.612437886315108315, 1.599625672291268286 ) ) ;
#42060=CARTESIAN_POINT ( 'NONE',  ( 6.367489420273535039, 7.457767740854454708, -1.199719254218452047 ) ) ;
#42063=CARTESIAN_POINT ( 'NONE',  ( -1.813562444701080523, 2.470692551218654387, -2.500000000000000444 ) ) ;
#42073=CARTESIAN_POINT ( 'NONE',  ( 6.403672513108120690, 6.804938187689173468, -0.5019199613840990004 ) ) ;
#42076=CARTESIAN_POINT ( 'NONE',  ( 6.536439455564168277, 6.798469917679251573, 0.7216878364870328300 ) ) ;
#42093=CARTESIAN_POINT ( 'NONE',  ( -6.414416072596845986, 8.576847732820027659, -1.443375672974066548 ) ) ;
#42097=CARTESIAN_POINT ( 'NONE',  ( 7.530627977747744062, 7.750430493652658015, -0.7998128361456341429 ) ) ;
#42104=CARTESIAN_POINT ( 'NONE',  ( -3.284818356260900796, 7.054314858938165678, 0.7998128361456352531 ) ) ;
#42114=CARTESIAN_POINT ( 'NONE',  ( 7.828907357248368726, 8.098423103070084395, 0.7998128361456281477 ) ) ;
#42120=DIRECTION ( 'NONE',  ( 0.7592566023652996821, 0.6507913734559648278, 0.000000000000000000 ) ) ;
#42130=CARTESIAN_POINT ( 'NONE',  ( -3.469446951953614189E-15, 8.999999999999998224, -0.7749999999999996891 ) ) ;
#42133=CARTESIAN_POINT ( 'NONE',  ( -7.273023059088104425, 7.449891421883056530, 0.000000000000000000 ) ) ;
#42136=CARTESIAN_POINT ( 'NONE',  ( -6.470902446588409518, 6.777469385738574381, 0.2989120342885512871 ) ) ;
#42153=CARTESIAN_POINT ( 'NONE',  ( 5.722950238744200391, 7.770137593325314285, 1.443375672974065660 ) ) ;
#42164=CARTESIAN_POINT ( 'NONE',  ( -3.851925040058333582, 7.508013290127760087, -0.7216878364870458196 ) ) ;
#42169=CARTESIAN_POINT ( 'NONE',  ( 4.778146133183440725, 8.258034039491356282, 0.8222960688244035365 ) ) ;
#42176=CARTESIAN_POINT ( 'NONE',  ( 3.188928480291414846, 8.980740528189164351, -2.451733079074511767 ) ) ;
#42185=CARTESIAN_POINT ( 'NONE',  ( 4.207966135563057541, 7.175396087857926375, 1.156120096431498379 ) ) ;
#42196=CARTESIAN_POINT ( 'NONE',  ( 3.718679271898170491, 7.560485927181699317, 0.7998128361456271485 ) ) ;
#42206=CARTESIAN_POINT ( 'NONE',  ( -5.966997003790228682, 8.054858819212300958, -1.443375672974066548 ) ) ;
#42208=CARTESIAN_POINT ( 'NONE',  ( 3.567203813726958828, 6.215469311773181182, 1.082531754730549078 ) ) ;
#42216=DIRECTION ( 'NONE',  ( -0.6507913734559641616, -0.7592566023653004592, 0.000000000000000000 ) ) ;
#42226=DIRECTION ( 'NONE',  ( 0.3281536732072464768, 0.000000000000000000, 0.9446243521954066358 ) ) ;
#42229=CARTESIAN_POINT ( 'NONE',  ( 5.682275777458851707, 6.762314840857718501, 1.082531754730549078 ) ) ;
#42231=DIRECTION ( 'NONE',  ( 0.000000000000000000, 0.000000000000000000, 1.000000000000000000 ) ) ;
#42243=EDGE_LOOP ( 'NONE', ( #64766, #78974, #23402, #207936 ) ) ;
#42259=CARTESIAN_POINT ( 'NONE',  ( -6.149505192250180663, 9.332117270003974951, -1.199719254218452047 ) ) ;
#42262=CARTESIAN_POINT ( 'NONE',  ( -5.611095471209320174, 7.639640364534566075, 1.599625672291263179 ) ) ;
#42263=CARTESIAN_POINT ( 'NONE',  ( -5.224688093219837626, 7.188831756880171397, -1.599625672291271394 ) ) ;
#42264=CARTESIAN_POINT ( 'NONE',  ( -5.032163277954181169, 7.944720250727295152, 1.129701600186810095 ) ) ;
#42267=CARTESIAN_POINT ( 'NONE',  ( -6.739811759324828344, 8.956476034002674780, -1.443375672974066548 ) ) ;
#42270=CARTESIAN_POINT ( 'NONE',  ( -5.327428015527048366, 5.180030537728460338, -0.7998128361456362523 ) ) ;
#42273=CARTESIAN_POINT ( 'NONE',  ( -7.533490631048818109, 8.818102486758951031, -1.199719254218452047 ) ) ;
#42284=ORIENTED_EDGE ( 'NONE', *, *, #18887, .T. ) ;
#42285=CARTESIAN_POINT ( 'NONE',  ( 4.754190777897029818, 8.299541367957775861, -0.7767638722561143183 ) ) ;
#42290=CARTESIAN_POINT ( 'NONE',  ( 5.273195401072370281, 5.116759154198018855, -0.7998128361456481317 ) ) ;
#42312=CARTESIAN_POINT ( 'NONE',  ( 5.982890925380405456, 10.20206618957764100, 0.000000000000000000 ) ) ;
#42326=DIRECTION ( 'NONE',  ( 1.000000000000000000, 0.000000000000000000, 0.000000000000000000 ) ) ;
#42327=CARTESIAN_POINT ( 'NONE',  ( 5.820234798683411981, 7.319712794923219690, 1.284739950006764220 ) ) ;
#42329=CARTESIAN_POINT ( 'NONE',  ( -3.485854892044994102, 7.080931450778859215, -0.7216878364870458196 ) ) ;
#42351=CARTESIAN_POINT ( 'NONE',  ( -0.4000000000001999734, 2.876379076189460093, -2.023857702507711132 ) ) ;
#42359=CARTESIAN_POINT ( 'NONE',  ( 3.230585741806197841, 6.991043475407723307, 0.7998128361456271485 ) ) ;
#42380=CARTESIAN_POINT ( 'NONE',  ( -6.818824913030298696, 6.919993584815607335, 0.7998128361456341429 ) ) ;
#42395=CARTESIAN_POINT ( 'NONE',  ( 3.725458348705031231, 7.568394850123006279, -1.734723475976807094E-15 ) ) ;
#42400=EDGE_CURVE ( 'NONE', #49550, #61752, #145413, .T. ) ;
#42405=CARTESIAN_POINT ( 'NONE',  ( 4.827066317303362553, 8.099069806723665721, 0.8733865547906801696 ) ) ;
#42408=CARTESIAN_POINT ( 'NONE',  ( 6.162627863271451290, 6.966383021533493647, 0.9102919922300183320 ) ) ;
#42427=CARTESIAN_POINT ( 'NONE',  ( 5.346851039111009563, 6.199209027673978412, 2.419999999999999485 ) ) ;
#42428=CARTESIAN_POINT ( 'NONE',  ( -5.143339171537843590, 7.093924681584509173, 1.599625672291263179 ) ) ;
#42430=CARTESIAN_POINT ( 'NONE',  ( 5.422335090822693715, 5.290755458906732933, 0.000000000000000000 ) ) ;
#42432=CARTESIAN_POINT ( 'NONE',  ( -4.749098946536820520, 8.762642214260091933, 0.7998128361456281477 ) ) ;
#42435=CARTESIAN_POINT ( 'NONE',  ( 6.016786309414542622, 10.24161080428416426, 0.7998128361456341429 ) ) ;
#42441=CARTESIAN_POINT ( 'NONE',  ( -5.594533863947632746, 7.496198557292433229, -1.347124935377568722 ) ) ;
#42442=FACE_OUTER_BOUND ( 'NONE', #61707, .T. ) ;
#42457=CARTESIAN_POINT ( 'NONE',  ( 4.828112100242277549, 6.726159765073026264, -1.443375672974068769 ) ) ;
#42460=CARTESIAN_POINT ( 'NONE',  ( -6.882699257592852504, 8.058845884393651460, -1.199719254218452047 ) ) ;
#42469=CARTESIAN_POINT ( 'NONE',  ( -3.187575512988701565, 6.732938841879847480, 0.000000000000000000 ) ) ;
#42474=CARTESIAN_POINT ( 'NONE',  ( 4.115782150200256950, 6.959440387612411349, 1.199719254218452047 ) ) ;
#42479=DIRECTION ( 'NONE',  ( -0.2553555850663286608, -0.9650793847679529636, 0.05844062175698114953 ) ) ;
#42503=CARTESIAN_POINT ( 'NONE',  ( -6.631346530859867805, 6.909194838857525944, 0.000000000000000000 ) ) ;
#42531=CARTESIAN_POINT ( 'NONE',  ( -3.973948422136981407, 5.729635473950147606, -1.443375672974066548 ) ) ;
#42538=CARTESIAN_POINT ( 'NONE',  ( -4.228163802615396705, 6.026220084508304708, -1.599625672291271394 ) ) ;
#42543=ORIENTED_EDGE ( 'NONE', *, *, #126711, .F. ) ;
#42546=CARTESIAN_POINT ( 'NONE',  ( -3.654804927335652209, 6.421633627603656080, 1.199719254218452935 ) ) ;
#42549=CARTESIAN_POINT ( 'NONE',  ( 6.252685474373055996, 7.003816019006632310, -0.9791501464874209359 ) ) ;
#42553=CARTESIAN_POINT ( 'NONE',  ( 5.890091390494168522, 5.836471141856793388, 0.000000000000000000 ) ) ;
#42558=CARTESIAN_POINT ( 'NONE',  ( -3.006876207180748217, 6.730049018344652190, -0.7998128361456481317 ) ) ;
#42562=CARTESIAN_POINT ( 'NONE',  ( -5.984998465789844069, 5.947196063035064206, 0.7998128361456281477 ) ) ;
#42568=CARTESIAN_POINT ( 'NONE',  ( 5.519577934094852978, 7.532869904567736974, 1.443375672974064550 ) ) ;
#42569=CARTESIAN_POINT ( 'NONE',  ( -5.777182852754558340, 5.912670547734647286, 0.000000000000000000 ) ) ;
#42576=CARTESIAN_POINT ( 'NONE',  ( 4.848976215542928792, 5.686169002002086970, 1.199719254218452047 ) ) ;
#42583=CARTESIAN_POINT ( 'NONE',  ( 4.692003678781083487, 7.631698837623355658, -1.199719254218450271 ) ) ;
#42604=CARTESIAN_POINT ( 'NONE',  ( 4.954704567260191261, 7.963257648925383236, 1.029694947009308859 ) ) ;
#42611=CARTESIAN_POINT ( 'NONE',  ( 5.830888582329017744, 8.960397891762626799, -1.199719254218452047 ) ) ;
#42615=CARTESIAN_POINT ( 'NONE',  ( -4.864640111294652236, 8.076240785039992431, 0.9165970657895030627 ) ) ;
#42622=CARTESIAN_POINT ( 'NONE',  ( -7.781453819600577582, 8.043060642480948985, 0.000000000000000000 ) ) ;
#42636=CARTESIAN_POINT ( 'NONE',  ( 5.528692779322568640, 9.672168352510192690, 0.7998128361456341429 ) ) ;
#42644=CARTESIAN_POINT ( 'NONE',  ( 4.903208829997618423, 5.749440385532527564, -1.199719254218450271 ) ) ;
#42647=CARTESIAN_POINT ( 'NONE',  ( 6.333067150914820864, 6.561202228921677815, 0.7216878364870328300 ) ) ;
#42663=CARTESIAN_POINT ( 'NONE',  ( -5.157951095356222204, 4.982307464195829816, 0.000000000000000000 ) ) ;
#42664=CARTESIAN_POINT ( 'NONE',  ( 5.546694241766559230, 9.485244025454063532, 0.000000000000000000 ) ) ;
#42671=ORIENTED_EDGE ( 'NONE', *, *, #41266, .F. ) ;
#42678=CARTESIAN_POINT ( 'NONE',  ( -6.798487682609798632, 6.896266815991691779, 0.7998128361456341429 ) ) ;
#42679=CARTESIAN_POINT ( 'NONE',  ( -4.339491684825780737, 7.220434844675483355, -1.199719254218455378 ) ) ;
#42681=CARTESIAN_POINT ( 'NONE',  ( 7.797347741190739256, 8.269529584243604958, 0.7216878364870267237 ) ) ;
#42694=CARTESIAN_POINT ( 'NONE',  ( -5.686128154004278734, 7.329579007619248188, -1.223094714244008729 ) ) ;
#42699=CARTESIAN_POINT ( 'NONE',  ( 4.529832720741620022, 7.338536369956936589, -1.082531754730548412 ) ) ;
#42703=CARTESIAN_POINT ( 'NONE',  ( -5.986807348886189040, 9.142303119412650503, -1.199719254218452047 ) ) ;
#42716=CARTESIAN_POINT ( 'NONE',  ( 5.559725510055676168, 8.644040974110419384, 1.199719254218451159 ) ) ;
#42731=CARTESIAN_POINT ( 'NONE',  ( 2.971361445535975143, 6.558719713395274376, 0.4765173780192366593 ) ) ;
#42754=CARTESIAN_POINT ( 'NONE',  ( 7.024532985656136930, 8.328281583754568729, 1.082531754730549967 ) ) ;
#42759=CARTESIAN_POINT ( 'NONE',  ( 5.980555156959511898, 9.991415093179179863, -0.7216878364870458196 ) ) ;
#42782=CARTESIAN_POINT ( 'NONE',  ( -5.829079699232685208, 5.765290835385048496, 0.000000000000000000 ) ) ;
#42784=CARTESIAN_POINT ( 'NONE',  ( 5.112833325684902341, 7.058334528089426740, -1.443375672974078761 ) ) ;
#42789=CARTESIAN_POINT ( 'NONE',  ( -3.657667580636712934, 7.489305620709952649, -0.7998128361456481317 ) ) ;
#42794=CARTESIAN_POINT ( 'NONE',  ( -3.311934663488232733, 7.085950550703385531, -0.7998128361456481317 ) ) ;
#42802=CARTESIAN_POINT ( 'NONE',  ( -3.935609729716867289, 7.813571461303467913, 0.7998128361456352531 ) ) ;
#42812=CARTESIAN_POINT ( 'NONE',  ( -5.472651281771599763, 6.413789912602166687, 1.199719254218452935 ) ) ;
#42818=CARTESIAN_POINT ( 'NONE',  ( -5.817857314039913241, 5.960124085900898372, 0.000000000000000000 ) ) ;
#42819=CARTESIAN_POINT ( 'NONE',  ( -4.787437638956927977, 7.639075441208117212, -1.082531754730549967 ) ) ;
#42820=CARTESIAN_POINT ( 'NONE',  ( 5.027041095616958444, 9.086908054853605421, 0.000000000000000000 ) ) ;
#42821=CARTESIAN_POINT ( 'NONE',  ( -5.926849427829407269, 6.943687749669614995, -1.199719254218453823 ) ) ;
#42839=CARTESIAN_POINT ( 'NONE',  ( 7.095713291905693332, 9.371694488680407886, 1.599625672291268286 ) ) ;
#42858=CARTESIAN_POINT ( 'NONE',  ( 5.010605496441194795, 7.906410611435644498, -1.080668833775387139 ) ) ;
#42873=CARTESIAN_POINT ( 'NONE',  ( 7.361151057576892143, 7.552707420120024828, 0.7998128361456291469 ) ) ;
#42876=CARTESIAN_POINT ( 'NONE',  ( -4.329849954717889915, 6.144853928627882489, 1.599625672291270506 ) ) ;
#42879=CARTESIAN_POINT ( 'NONE',  ( -6.577113915960828727, 9.727031097712693253, -1.082531754730549967 ) ) ;
#42883=EDGE_CURVE ( 'NONE', #99015, #112384, #10047, .T. ) ;
#42890=CARTESIAN_POINT ( 'NONE',  ( 5.833751235630055376, 10.02806988486892514, 0.7998128361456331437 ) ) ;
#42891=CARTESIAN_POINT ( 'NONE',  ( 6.554440917563797875, 6.611545590104705994, -0.7998128361456481317 ) ) ;
#42898=CARTESIAN_POINT ( 'NONE',  ( 4.934241560730721510, 4.721313007132757811, 0.000000000000000000 ) ) ;
#42904=CARTESIAN_POINT ( 'NONE',  ( 5.061990249855835344, 6.999017606288844284, -1.599625672291273171 ) ) ;
#42905=ORIENTED_EDGE ( 'NONE', *, *, #209983, .F. ) ;
#42914=CARTESIAN_POINT ( 'NONE',  ( -5.777182852754558340, 5.912670547734647286, 0.000000000000000000 ) ) ;
#42915=CARTESIAN_POINT ( 'NONE',  ( 6.292392690518195941, 8.434487120394948079, -1.443375672974078761 ) ) ;
#42916=CARTESIAN_POINT ( 'NONE',  ( -5.397554552016258889, 7.390509292142662723, 1.443375672974058777 ) ) ;
#42917=CARTESIAN_POINT ( 'NONE',  ( -7.208094944320834863, 8.438474185576302133, -1.199719254218452047 ) ) ;
#42929=CARTESIAN_POINT ( 'NONE',  ( 5.234329823327693809, 8.264412672927770487, 1.199719254218451159 ) ) ;
#42930=CARTESIAN_POINT ( 'NONE',  ( 6.658989722967328717, 7.797851427330578566, 1.199719254218452935 ) ) ;
#42933=CARTESIAN_POINT ( 'NONE',  ( 3.228249973385329596, 6.780392379009261283, -1.734723475976807094E-15 ) ) ;
#42941=FACE_OUTER_BOUND ( 'NONE', #53527, .T. ) ;
#42949=ORIENTED_EDGE ( 'NONE', *, *, #15710, .F. ) ;
#42953=CARTESIAN_POINT ( 'NONE',  ( 3.147653791585713901, 8.920000000000001705, -2.500000000000002220 ) ) ;
#42954=CARTESIAN_POINT ( 'NONE',  ( 3.888156192069020634, 7.758209000714329839, 1.040834085586084257E-14 ) ) ;
#42956=CARTESIAN_POINT ( 'NONE',  ( -4.004454267989906668, 5.765225627445230927, 1.599625672291270506 ) ) ;
#42959=CARTESIAN_POINT ( 'NONE',  ( 6.547661840756936691, 6.603636667163397256, 0.7998128361456352531 ) ) ;
#42965=CARTESIAN_POINT ( 'NONE',  ( 6.912678218121202534, 9.158153569265168770, 1.599625672291268286 ) ) ;
#42970=CARTESIAN_POINT ( 'NONE',  ( 5.370438244788902971, 9.279612028980123384, -0.7216878364870458196 ) ) ;
#42972=CARTESIAN_POINT ( 'NONE',  ( -6.805266759416629618, 6.904175738932996964, 0.000000000000000000 ) ) ;
#42973=CARTESIAN_POINT ( 'NONE',  ( 5.499767588998890844, 6.445425604367387429, 1.199719254218451159 ) ) ;
#42974=ORIENTED_EDGE ( 'NONE', *, *, #147140, .T. ) ;
#42980=CARTESIAN_POINT ( 'NONE',  ( -4.003117076043361422, 7.684394865269255526, -0.1089946556460293509 ) ) ;
#42983=CARTESIAN_POINT ( 'NONE',  ( -4.111865726694519552, 8.019203457777400956, 0.000000000000000000 ) ) ;
#42998=CYLINDRICAL_SURFACE ( 'NONE', #170510, 0.7500000000000011102 ) ;
#43012=ORIENTED_EDGE ( 'NONE', *, *, #190135, .T. ) ;
#43017=CARTESIAN_POINT ( 'NONE',  ( 7.472478939787284169, 8.746922180287201698, 1.199719254218452935 ) ) ;
#43023=ADVANCED_FACE ( 'NONE', ( #49994 ), #148569, .T. ) ;
#43030=CARTESIAN_POINT ( 'NONE',  ( -6.154475385960665790, 6.144919136567696505, 0.000000000000000000 ) ) ;
#43032=CARTESIAN_POINT ( 'NONE',  ( -6.459533842268148973, 6.500820668926428958, 0.000000000000000000 ) ) ;
#43034=CARTESIAN_POINT ( 'NONE',  ( 7.065207446052794715, 9.336104335185329006, -1.443375672974064550 ) ) ;
#43043=CARTESIAN_POINT ( 'NONE',  ( -4.502189528189771472, 7.410248995266807803, -1.199719254218453823 ) ) ;
#43048=FACE_OUTER_BOUND ( 'NONE', #147921, .T. ) ;
#43050=CARTESIAN_POINT ( 'NONE',  ( -4.665414256878301025, 6.536345614481700927, -1.443375672974066548 ) ) ;
#43054=CARTESIAN_POINT ( 'NONE',  ( -4.773352600463090845, 7.726605912919016106, 1.199719254218452935 ) ) ;
#43077=CARTESIAN_POINT ( 'NONE',  ( -6.414942957921379474, 7.513130201443591005, -1.199719254218452047 ) ) ;
#43080=CARTESIAN_POINT ( 'NONE',  ( -5.330290668828105538, 6.247702530834755130, 1.199719254218452935 ) ) ;
#43105=CARTESIAN_POINT ( 'NONE',  ( -4.132202957115018727, 8.042930226601317401, 0.000000000000000000 ) ) ;
#43114=DIRECTION ( 'NONE',  ( 0.000000000000000000, 0.000000000000000000, 1.000000000000000000 ) ) ;
#43132=CARTESIAN_POINT ( 'NONE',  ( 5.996449078994045223, 10.21788403546024782, 0.7998128361456331437 ) ) ;
#43148=CARTESIAN_POINT ( 'NONE',  ( 6.124909263556299166, 6.992440323537196356, 0.9511531368890328020 ) ) ;
#43150=CARTESIAN_POINT ( 'NONE',  ( 7.702440666339465558, 8.158804663583751449, -0.7216878364870317197 ) ) ;
#43157=CARTESIAN_POINT ( 'NONE',  ( -3.474632506852224356, 7.275764701294714420, -0.7998128361456481317 ) ) ;
#43164=CARTESIAN_POINT ( 'NONE',  ( -6.089020385868867180, 7.236850217336030511, -1.082531754730549967 ) ) ;
#43168=CARTESIAN_POINT ( 'NONE',  ( 6.964048179274811012, 8.153752959689313684, 1.199719254218452047 ) ) ;
#43182=CARTESIAN_POINT ( 'NONE',  ( 5.969332771766739931, 10.18624834369502885, -0.7998128361456481317 ) ) ;
#43186=ORIENTED_EDGE ( 'NONE', *, *, #75725, .T. ) ;
#43200=CARTESIAN_POINT ( 'NONE',  ( -4.749098946536820520, 8.762642214260091933, 0.7998128361456281477 ) ) ;
#43204=CARTESIAN_POINT ( 'NONE',  ( 5.993586425693011144, 9.150212042353954800, -1.199719254218452047 ) ) ;
#43206=CARTESIAN_POINT ( 'NONE',  ( -6.497792602234238934, 6.760263899176822022, -0.1076752790035370722 ) ) ;
#43221=CARTESIAN_POINT ( 'NONE',  ( -1.843739406749240750, 8.920000000000001705, 0.7750000000000013545 ) ) ;
#43222=CARTESIAN_POINT ( 'NONE',  ( 5.234856708652227297, 7.200695141551334721, 1.443375672974065660 ) ) ;
#43223=EDGE_LOOP ( 'NONE', ( #192492, #13501, #19205 ) ) ;
#43230=CARTESIAN_POINT ( 'NONE',  ( -4.587666091342180508, 8.411066132956936059, -0.02982374410689043673 ) ) ;
#43233=CARTESIAN_POINT ( 'NONE',  ( -4.611181642423629157, 7.433443445252599702, 1.082531754730549967 ) ) ;
#43236=CARTESIAN_POINT ( 'NONE',  ( 2.974639739360878554, 6.521327805418967394, -0.5442850241774439546 ) ) ;
#43246=CARTESIAN_POINT ( 'NONE',  ( -2.969872605471120863, 6.605953636083950364, 2.420000000000000373 ) ) ;
#43259=ORIENTED_EDGE ( 'NONE', *, *, #30625, .T. ) ;
#43263=CARTESIAN_POINT ( 'NONE',  ( 3.691562964670865199, 7.528850235416478576, -0.7998128361456362523 ) ) ;
#43274=CARTESIAN_POINT ( 'NONE',  ( -6.970300371201519241, 7.304640985922785212, 0.7216878364870317197 ) ) ;
#43276=CARTESIAN_POINT ( 'NONE',  ( 5.356880090730874677, 5.422317325373725794, 0.7216878364870328300 ) ) ;
#43295=CARTESIAN_POINT ( 'NONE',  ( -3.038435823238377687, 6.558942537171132514, -0.7216878364870458196 ) ) ;
#43298=DIRECTION ( 'NONE',  ( 0.7592566023652995710, -0.6507913734559650498, 0.000000000000000000 ) ) ;
#43321=EDGE_CURVE ( 'NONE', #173093, #182271, #138186, .T. ) ;
#43326=CARTESIAN_POINT ( 'NONE',  ( -6.084577077482911101, 10.32070003369722144, 0.000000000000000000 ) ) ;
#43329=CARTESIAN_POINT ( 'NONE',  ( -6.448838341955544173, 7.552674816150118708, 1.199719254218452047 ) ) ;
#43330=CARTESIAN_POINT ( 'NONE',  ( -4.900510728191886933, 8.135641830034209931, 1.034109914766440541 ) ) ;
#43331=CARTESIAN_POINT ( 'NONE',  ( -5.981082042284069367, 7.006959133200059142, 1.199719254218452935 ) ) ;
#43335=CARTESIAN_POINT ( 'NONE',  ( -5.573810548549546162, 9.516879716700865188, 0.7216878364870267237 ) ) ;
#43337=CARTESIAN_POINT ( 'NONE',  ( -3.492107083971660586, 6.231819477012331632, 1.199719254218452935 ) ) ;
#43340=CARTESIAN_POINT ( 'NONE',  ( -3.481411583659053566, 7.283673624236017830, 0.000000000000000000 ) ) ;
#43353=CARTESIAN_POINT ( 'NONE',  ( 6.059568310664962709, 6.034194215389424798, 0.7998128361456352531 ) ) ;
#43375=CARTESIAN_POINT ( 'NONE',  ( 4.532168488718122390, 8.509556680138327778, 0.7998128361456271485 ) ) ;
#43376=CARTESIAN_POINT ( 'NONE',  ( 5.422335090822693715, 5.290755458906732933, 0.000000000000000000 ) ) ;
#43390=CARTESIAN_POINT ( 'NONE',  ( 6.218145995260431214, 7.027935176161393294, 1.016989286988238206 ) ) ;
#43391=CARTESIAN_POINT ( 'NONE',  ( -3.309598895067336510, 6.875299454304925284, 0.000000000000000000 ) ) ;
#43392=CARTESIAN_POINT ( 'NONE',  ( 4.421367491832282504, 5.291255174293369556, 1.082531754730549078 ) ) ;
#43413=CARTESIAN_POINT ( 'NONE',  ( -5.606868911964699720, 5.576453016528778228, -0.3534498849190413350 ) ) ;
#43421=CARTESIAN_POINT ( 'NONE',  ( 3.555981428534177091, 7.370671776590375757, 0.7998128361456271485 ) ) ;
#43440=CARTESIAN_POINT ( 'NONE',  ( -6.306477729012051725, 7.386587434382707151, 1.199719254218452047 ) ) ;
#43458=CARTESIAN_POINT ( 'NONE',  ( 4.980641328173811999, 6.904110530993182948, 1.599625672291269396 ) ) ;
#43471=CARTESIAN_POINT ( 'NONE',  ( 5.606371582794006159, 7.377293116531995487, 1.238817421570908905 ) ) ;
#43492=CARTESIAN_POINT ( 'NONE',  ( -5.712781623311813384, 7.758274208654143855, -1.599625672291271394 ) ) ;
#43494=CARTESIAN_POINT ( 'NONE',  ( 4.037295881819344956, 7.932205305423046582, -0.7998128361456362523 ) ) ;
#43498=CARTESIAN_POINT ( 'NONE',  ( -6.587282531393266360, 8.778525268082516320, 1.599625672291269396 ) ) ;
#43506=CARTESIAN_POINT ( 'NONE',  ( -4.941402330188276792, 8.092876352253616901, -1.081280284042404727 ) ) ;
#43522=CARTESIAN_POINT ( 'NONE',  ( 5.614485009834906393, 6.683225611963085733, -1.082531754730548412 ) ) ;
#43525=CARTESIAN_POINT ( 'NONE',  ( -5.749539660647037032, 8.865490816466966351, 1.199719254218454489 ) ) ;
#43540=CARTESIAN_POINT ( 'NONE',  ( 5.585032934186686226, 5.480569609498057382, 0.000000000000000000 ) ) ;
#43567=CIRCLE ( 'NONE', #71181, 0.08000000000000020983 ) ;
#43591=CARTESIAN_POINT ( 'NONE',  ( -4.787437638956939523, 5.718337012605431369, -1.082531754730549967 ) ) ;
#43596=CARTESIAN_POINT ( 'NONE',  ( -5.152980901645737077, 8.169505597632108262, -1.199719254218453823 ) ) ;
#43605=CARTESIAN_POINT ( 'NONE',  ( -4.132202957115018727, 8.042930226601317401, 0.000000000000000000 ) ) ;
#43607=CARTESIAN_POINT ( 'NONE',  ( 5.696489930276292135, 7.416392257432566026, -1.320530921439456273 ) ) ;
#43610=CARTESIAN_POINT ( 'NONE',  ( 2.980618654443941473, 6.479024054206157679, 0.4184689722446261473 ) ) ;
#43612=CARTESIAN_POINT ( 'NONE',  ( 4.667750024854814050, 8.667735138964429709, -0.7998128361456381397 ) ) ;
#43618=CARTESIAN_POINT ( 'NONE',  ( -7.910256278930404505, 8.193330178365746619, -0.7998128361456362523 ) ) ;
#43625=CARTESIAN_POINT ( 'NONE',  ( -6.134138155540168391, 6.121192367743780949, 0.000000000000000000 ) ) ;
#43630=CARTESIAN_POINT ( 'NONE',  ( 4.868786560638885597, 7.733982516503781213, 1.082531754730548412 ) ) ;
#43631=CARTESIAN_POINT ( 'NONE',  ( -5.411112705185557203, 9.327065566109540740, 0.7216878364870267237 ) ) ;
#43639=CARTESIAN_POINT ( 'NONE',  ( 3.528865121306874464, 7.339036084825155015, -0.7998128361456362523 ) ) ;
#43643=CYLINDRICAL_SURFACE ( 'NONE', #137595, 0.07999999999999972411 ) ;
#43647=CARTESIAN_POINT ( 'NONE',  ( 4.179656494762836516, 8.098292687190454586, -0.7998128361456361413 ) ) ;
#43667=CARTESIAN_POINT ( 'NONE',  ( 5.028717893731355026, 7.888467461587344687, 1.094519599958807765 ) ) ;
#43675=CARTESIAN_POINT ( 'NONE',  ( 6.638652492546827766, 7.774124658506663010, 1.199719254218452047 ) ) ;
#43676=ORIENTED_EDGE ( 'NONE', *, *, #205115, .T. ) ;
#43680=CARTESIAN_POINT ( 'NONE',  ( -4.907053429147543611, 8.030730943182621928, 0.9696864716568325271 ) ) ;
#43687=CARTESIAN_POINT ( 'NONE',  ( -6.903036488013351679, 8.082572653217566128, -1.199719254218452047 ) ) ;
#43693=CARTESIAN_POINT ( 'NONE',  ( -3.938278094839060994, 7.324765956376747766, 0.6593293099422595782 ) ) ;
#43699=CARTESIAN_POINT ( 'NONE',  ( 7.198453214212898743, 7.362893269528701268, 0.7998128361456291469 ) ) ;
#43708=CARTESIAN_POINT ( 'NONE',  ( 5.065906673361608270, 5.939254536123854677, -1.199719254218450271 ) ) ;
#43711=CARTESIAN_POINT ( 'NONE',  ( 5.573810548549551491, 6.635772073796838200, -1.082531754730548412 ) ) ;
#43721=CARTESIAN_POINT ( 'NONE',  ( -5.631831469557842418, 7.372220891417233801, 1.235678285582973546 ) ) ;
#43726=CARTESIAN_POINT ( 'NONE',  ( -3.284818356260900796, 7.054314858938165678, 0.7998128361456352531 ) ) ;
#43727=CARTESIAN_POINT ( 'NONE',  ( 7.241463443474815520, 8.581367117876336437, -1.082531754730548412 ) ) ;
#43737=DIRECTION ( 'NONE',  ( 0.6507913734559641616, -0.7592566023653004592, 0.000000000000000000 ) ) ;
#43739=ORIENTED_EDGE ( 'NONE', *, *, #143009, .T. ) ;
#43742=CARTESIAN_POINT ( 'NONE',  ( -5.478376588373717659, 8.549133898814758936, -1.199719254218452047 ) ) ;
#43743=CARTESIAN_POINT ( 'NONE',  ( -4.664887371553763096, 7.600063145858131364, -1.199719254218453823 ) ) ;
#43745=CARTESIAN_POINT ( 'NONE',  ( 6.821160681006781523, 9.051383109298340557, 1.443375672974063439 ) ) ;
#43757=CARTESIAN_POINT ( 'NONE',  ( -6.320392545075788959, 6.875563024200552320, -0.7000339101758262794 ) ) ;
#43761=CARTESIAN_POINT ( 'NONE',  ( 5.722950238744209273, 6.809768379023969587, 1.082531754730549967 ) ) ;
#43767=CARTESIAN_POINT ( 'NONE',  ( -5.582925393777276035, 9.735439736040634173, 0.7998128361456291469 ) ) ;
#43783=CARTESIAN_POINT ( 'NONE',  ( 5.017399365509065845, 8.011327138806002779, -1.199719254218450271 ) ) ;
#43808=VERTEX_POINT ( 'NONE', #36402 ) ;
#43816=CARTESIAN_POINT ( 'NONE',  ( 5.722950238744187956, 9.690876021928001904, 0.7216878364870317197 ) ) ;
#43847=CARTESIAN_POINT ( 'NONE',  ( -3.169574050544739841, 6.919863168935977527, -0.7998128361456481317 ) ) ;
#43849=CARTESIAN_POINT ( 'NONE',  ( 4.692530563661249765, 8.488719734331187539, 0.000000000000000000 ) ) ;
#43854=CARTESIAN_POINT ( 'NONE',  ( -4.145761110728687804, 8.058748072483927771, -0.7998128361456481317 ) ) ;
#43859=CARTESIAN_POINT ( 'NONE',  ( -3.461074353238556167, 7.259946855412102273, 0.000000000000000000 ) ) ;
#43861=CARTESIAN_POINT ( 'NONE',  ( -1.844764736977754005, 2.494476015512113509, 2.491383360649019885 ) ) ;
#43865=CARTESIAN_POINT ( 'NONE',  ( -6.961185525973791144, 7.086080966583015339, 0.7998128361456341429 ) ) ;
#43874=CARTESIAN_POINT ( 'NONE',  ( -3.461074353238556167, 7.259946855412102273, 0.000000000000000000 ) ) ;
#43875=EDGE_CURVE ( 'NONE', #40754, #206605, #91782, .T. ) ;
#43879=CARTESIAN_POINT ( 'NONE',  ( -4.990809943606273613, 7.876343129965691858, -1.082531754730549967 ) ) ;
#43880=CARTESIAN_POINT ( 'NONE',  ( -4.733205024502264102, 7.575804057677677505, 1.082531754730549967 ) ) ;
#43881=CARTESIAN_POINT ( 'NONE',  ( 4.864343252252968597, 8.897093904262280972, 0.000000000000000000 ) ) ;
#43882=CARTESIAN_POINT ( 'NONE',  ( -6.149505192250180663, 9.332117270003974951, -1.199719254218452047 ) ) ;
#43900=CARTESIAN_POINT ( 'NONE',  ( 8.174640274396848483, 8.501778173076651512, 0.7998128361456291469 ) ) ;
#43919=CARTESIAN_POINT ( 'NONE',  ( 4.634937608369048334, 8.440560775401745985, -0.4060563726728562139 ) ) ;
#43932=CARTESIAN_POINT ( 'NONE',  ( 7.388267364804250725, 7.584343111885245570, -0.7998128361456341429 ) ) ;
#43935=CARTESIAN_POINT ( 'NONE',  ( -5.327428015527048366, 5.180030537728460338, -0.7998128361456362523 ) ) ;
#43938=CARTESIAN_POINT ( 'NONE',  ( -6.333067150914850174, 8.481940657524365434, 1.443375672974064550 ) ) ;
#43949=CARTESIAN_POINT ( 'NONE',  ( 5.806634928402749196, 9.996434193103704402, -0.7998128361456481317 ) ) ;
#43950=CARTESIAN_POINT ( 'NONE',  ( 5.180097208873055692, 8.201141289397330780, -1.199719254218450271 ) ) ;
#43964=CARTESIAN_POINT ( 'NONE',  ( 5.176180785367283654, 9.260904359562321275, -0.7998128361456481317 ) ) ;
#43976=CARTESIAN_POINT ( 'NONE',  ( -4.665414256878293031, 7.496714828783040296, -1.082531754730549967 ) ) ;
#43977=CARTESIAN_POINT ( 'NONE',  ( -6.074935347375019390, 9.245119117649618801, 1.199719254218452047 ) ) ;
#43990=CARTESIAN_POINT ( 'NONE',  ( 6.313256805818848960, 7.394496357324014113, 1.199719254218452047 ) ) ;
#43991=CARTESIAN_POINT ( 'NONE',  ( 6.875920180786008196, 8.050936961452347163, -1.199719254218452047 ) ) ;
#43994=CARTESIAN_POINT ( 'NONE',  ( 5.989670002187236442, 10.20997511251894529, -0.7998128361456481317 ) ) ;
#43996=ORIENTED_EDGE ( 'NONE', *, *, #125545, .T. ) ;
#44000=CARTESIAN_POINT ( 'NONE',  ( 4.858757509019037357, 5.629766575900002401, 2.420000000000000373 ) ) ;
#44008=CARTESIAN_POINT ( 'NONE',  ( -6.147915675425737803, 6.345191967827721768, 0.2080023349117297582 ) ) ;
#44011=CARTESIAN_POINT ( 'NONE',  ( 5.194709132691408549, 6.089524072008651423, 1.199719254218452935 ) ) ;
#44013=CARTESIAN_POINT ( 'NONE',  ( -3.492107083971660586, 6.231819477012331632, 1.199719254218452935 ) ) ;
#44016=CARTESIAN_POINT ( 'NONE',  ( 6.384963997392946844, 6.413822516572072807, 0.7998128361456352531 ) ) ;
#44026=CARTESIAN_POINT ( 'NONE',  ( 7.200788982633824276, 7.573544365927161515, 0.000000000000000000 ) ) ;
#44028=CARTESIAN_POINT ( 'NONE',  ( -5.596483547390937119, 9.751257581923240991, 0.000000000000000000 ) ) ;
#44029=CARTESIAN_POINT ( 'NONE',  ( 5.011674058906918638, 5.875983152593414971, 1.199719254218452047 ) ) ;
#44039=CARTESIAN_POINT ( 'NONE',  ( -4.553559489343377287, 6.405848385690952718, -1.599625672291271394 ) ) ;
#44052=DIRECTION ( 'NONE',  ( 0.000000000000000000, 0.000000000000000000, 1.000000000000000000 ) ) ;
#44063=CIRCLE ( 'NONE', #175485, 1.250000000000000888 ) ;
#44074=CARTESIAN_POINT ( 'NONE',  ( 4.434925645001613681, 5.307073019657559065, -1.082531754730548412 ) ) ;
#44085=CARTESIAN_POINT ( 'NONE',  ( -4.630991987519598396, 7.560518531151607213, 1.199719254218452935 ) ) ;
#44087=CARTESIAN_POINT ( 'NONE',  ( -5.692444392891315097, 7.734547439830227411, -1.599625672291271394 ) ) ;
#44100=CARTESIAN_POINT ( 'NONE',  ( -4.827585214917754719, 7.789877296449459365, -1.199719254218453823 ) ) ;
#44106=CARTESIAN_POINT ( 'NONE',  ( -6.156811154381562012, 6.355570232966157640, 0.7216878364870257245 ) ) ;
#44110=CARTESIAN_POINT ( 'NONE',  ( -5.635349125135588721, 6.603604063193491136, 1.199719254218452935 ) ) ;
#44123=( BOUNDED_CURVE ( )  B_SPLINE_CURVE ( 2, ( #116286, #68515, #200647, #117356, #202784 ),
 .UNSPECIFIED., .F., .T. ) 
 B_SPLINE_CURVE_WITH_KNOTS ( ( 3, 2, 3 ),
 ( 0.5190269744418570808, 0.5250000000000000222, 0.5270515662701394932 ),
 .UNSPECIFIED. ) 
 CURVE ( )  GEOMETRIC_REPRESENTATION_ITEM ( )  RATIONAL_B_SPLINE_CURVE ( ( 0.9456026235272760871, 0.9039719575195083179, 1.000000000000000000, 0.9670170684818317763, 0.9502741377139820589 ) ) 
 REPRESENTATION_ITEM ( '' )  );
#44129=ORIENTED_EDGE ( 'NONE', *, *, #186987, .T. ) ;
#44130=CARTESIAN_POINT ( 'NONE',  ( -5.986807348886189040, 9.142303119412650503, -1.199719254218452047 ) ) ;
#44132=CARTESIAN_POINT ( 'NONE',  ( -3.980200614063634568, 6.801261928786307642, 1.199719254218452935 ) ) ;
#44133=ORIENTED_EDGE ( 'NONE', *, *, #64546, .F. ) ;
#44141=CARTESIAN_POINT ( 'NONE',  ( -7.065207446497166366, 9.336104335703744539, 0.000000000000000000 ) ) ;
#44157=CARTESIAN_POINT ( 'NONE',  ( -7.944151662964566540, 8.232874793072271657, 0.000000000000000000 ) ) ;
#44172=AXIS2_PLACEMENT_3D ( 'NONE', #774, #21305, #135109 ) ;
#44186=CARTESIAN_POINT ( 'NONE',  ( 7.126746022638799971, 8.343567110280638133, 1.199719254218452047 ) ) ;
#44199=CARTESIAN_POINT ( 'NONE',  ( 5.107728353013315292, 7.811434107096660640, 1.148430247377411728 ) ) ;
#44201=CARTESIAN_POINT ( 'NONE',  ( 6.373741612200171325, 7.569024981389272710, 1.082531754730549967 ) ) ;
#44209=CARTESIAN_POINT ( 'NONE',  ( -5.496904935697871863, 5.377753611261092637, 0.7998128361456281477 ) ) ;
#44217=CARTESIAN_POINT ( 'NONE',  ( -5.872089928050201024, 8.904503111816948646, 1.082531754730550855 ) ) ;
#44220=CARTESIAN_POINT ( 'NONE',  ( 5.969332771766739931, 10.18624834369502885, -0.7998128361456481317 ) ) ;
#44234=DIRECTION ( 'NONE',  ( 0.000000000000000000, 1.000000000000000000, 0.000000000000000000 ) ) ;
#44236=CARTESIAN_POINT ( 'NONE',  ( 3.061108821635398769, 6.793320401875094561, -0.7998128361456362523 ) ) ;
#44257=CARTESIAN_POINT ( 'NONE',  ( 7.679767667498067496, 7.924426798361372093, 0.000000000000000000 ) ) ;
#44258=CARTESIAN_POINT ( 'NONE',  ( -6.121671443416687453, 7.010146470470823843, 0.9629068762325782016 ) ) ;
#44262=EDGE_CURVE ( 'NONE', #120674, #39859, #117417, .T. ) ;
#44265=CARTESIAN_POINT ( 'NONE',  ( 4.854701522145073334, 7.821512988214679218, -1.199719254218450271 ) ) ;
#44274=CARTESIAN_POINT ( 'NONE',  ( 3.255366281057017197, 6.812028071292901998, -0.7216878364870338292 ) ) ;
#44277=CARTESIAN_POINT ( 'NONE',  ( 5.912764389335563919, 6.070849007079172743, -0.7216878364870458196 ) ) ;
#44285=CARTESIAN_POINT ( 'NONE',  ( -4.970620135051034616, 8.062850052469723749, -1.111334424012894617 ) ) ;
#44288=CARTESIAN_POINT ( 'NONE',  ( -5.695833931516914639, 6.778132687258748845, 1.082531754730549078 ) ) ;
#44299=DIRECTION ( 'NONE',  ( -1.000000000000000000, 0.000000000000000000, 0.000000000000000000 ) ) ;
#44309=SPHERICAL_SURFACE ( 'NONE', #142847, 0.08000000000000000167 ) ;
#44320=CARTESIAN_POINT ( 'NONE',  ( 3.770049233051776749, 6.556085317605844232, 1.199719254218451159 ) ) ;
#44332=CARTESIAN_POINT ( 'NONE',  ( -6.455090533882201775, 8.624301270986276080, -1.443375672974066548 ) ) ;
#44334=CARTESIAN_POINT ( 'NONE',  ( 5.031484404002889654, 6.003058238492422483, 1.082531754730549078 ) ) ;
#44352=CARTESIAN_POINT ( 'NONE',  ( -4.990809943606294929, 4.995235487061662205, -0.7216878364870338292 ) ) ;
#44357=CYLINDRICAL_SURFACE ( 'NONE', #130625, 0.4000000000000001332 ) ;
#44384=CARTESIAN_POINT ( 'NONE',  ( 4.787437623848783907, 6.678706240755900581, -1.249999999999999334 ) ) ;
#44389=CARTESIAN_POINT ( 'NONE',  ( -4.986341270546564175, 8.046800470007955397, 1.126807992560383331 ) ) ;
#44394=CARTESIAN_POINT ( 'NONE',  ( 6.966220764712121927, 6.002124920821316323, 2.420000000000000373 ) ) ;
#44397=CARTESIAN_POINT ( 'NONE',  ( -5.015590482412729756, 4.816220082428420923, 0.000000000000000000 ) ) ;
#44402=CARTESIAN_POINT ( 'NONE',  ( -5.815521545619021460, 5.749472989502435460, -0.7998128361456362523 ) ) ;
#44407=ORIENTED_EDGE ( 'NONE', *, *, #58668, .F. ) ;
#44416=CARTESIAN_POINT ( 'NONE',  ( 3.725458348705031231, 7.568394850123006279, -1.734723475976807094E-15 ) ) ;
#44440=CARTESIAN_POINT ( 'NONE',  ( 5.448397627845284141, 7.449826213943242514, 1.599625672291268286 ) ) ;
#44441=CARTESIAN_POINT ( 'NONE',  ( 5.598591087800349086, 5.496387455380669529, -0.7998128361456481317 ) ) ;
#44446=CYLINDRICAL_SURFACE ( 'NONE', #58221, 1.250000000000000000 ) ;
#44457=CARTESIAN_POINT ( 'NONE',  ( 4.749341595749815070, 8.305088035112140332, 0.7662636247844747395 ) ) ;
#44458=CARTESIAN_POINT ( 'NONE',  ( -4.380693030546956912, 6.204170850428461392, 1.443375672974065660 ) ) ;
#44459=CARTESIAN_POINT ( 'NONE',  ( 4.014622883422321209, 5.777089012116397804, -1.443375672974068769 ) ) ;
#44461=AXIS2_PLACEMENT_3D ( 'NONE', #23750, #74649, #89854 ) ;
#44481=AXIS2_PLACEMENT_3D ( 'NONE', #153401, #39647, #168575 ) ;
#44487=CARTESIAN_POINT ( 'NONE',  ( 3.878514461961128479, 6.682628084666728085, -1.199719254218448494 ) ) ;
#44506=CARTESIAN_POINT ( 'NONE',  ( -6.526270840131767059, 8.707344961610770540, -1.599625672291271394 ) ) ;
#44515=ORIENTED_EDGE ( 'NONE', *, *, #24434, .F. ) ;
#44521=CARTESIAN_POINT ( 'NONE',  ( 5.682802662783380754, 6.658966523782627434, 1.199719254218452935 ) ) ;
#44529=CARTESIAN_POINT ( 'NONE',  ( 4.848511436970775357, 8.075560130489554567, 0.9049096096846224180 ) ) ;
#44531=CARTESIAN_POINT ( 'NONE',  ( 5.825676364550436581, 7.207913871576331566, 1.168708750232345883 ) ) ;
#44547=CARTESIAN_POINT ( 'NONE',  ( -6.225321503573748139, 6.939195112795077947, 0.8439093341676749960 ) ) ;
#44552=CARTESIAN_POINT ( 'NONE',  ( -5.550083779947821760, 7.568460058062819407, -1.599625672291271394 ) ) ;
#44554=CARTESIAN_POINT ( 'NONE',  ( 5.408776937209000657, 5.274937613024121674, 0.7998128361456352531 ) ) ;
#44558=CARTESIAN_POINT ( 'NONE',  ( -7.910256278930404505, 8.193330178365746619, -0.7998128361456362523 ) ) ;
#44561=AXIS2_PLACEMENT_3D ( 'NONE', #205254, #89415, #73123 ) ;
#44562=CARTESIAN_POINT ( 'NONE',  ( 7.364013710877980401, 8.620379413226322285, -1.199719254218452047 ) ) ;
#44563=DIRECTION ( 'NONE',  ( 0.000000000000000000, 0.000000000000000000, -1.000000000000000000 ) ) ;
#44568=CARTESIAN_POINT ( 'NONE',  ( -5.978723031652583231, 7.198045494411626777, -1.221819409761595088 ) ) ;
#44586=CARTESIAN_POINT ( 'NONE',  ( 4.204437034013637664, 6.958908068774287692, -1.082531754730548412 ) ) ;
#44598=CARTESIAN_POINT ( 'NONE',  ( -3.526529353330355221, 6.168015774643768268, -1.082531754730546636 ) ) ;
#44602=CARTESIAN_POINT ( 'NONE',  ( 6.086684617892325733, 6.065829907154645539, -0.7998128361456481317 ) ) ;
#44609=DIRECTION ( 'NONE',  ( 0.000000000000000000, -1.000000000000000000, 0.000000000000000000 ) ) ;
#44652=ORIENTED_EDGE ( 'NONE', *, *, #31028, .F. ) ;
#44653=CARTESIAN_POINT ( 'NONE',  ( -4.950135482320926705, 6.868520377498098739, -1.443375672974066548 ) ) ;
#44660=CARTESIAN_POINT ( 'NONE',  ( -4.613517410400161722, 8.604463755433990002, -0.7998128361456362523 ) ) ;
#44670=CARTESIAN_POINT ( 'NONE',  ( -4.899292406491858820, 6.809203455697518947, -1.599625672291271394 ) ) ;
#44672=VERTEX_POINT ( 'NONE', #135547 ) ;
#44673=CARTESIAN_POINT ( 'NONE',  ( 5.568688238291347403, 7.519645578322940338, 1.337618216391135428 ) ) ;
#44678=CARTESIAN_POINT ( 'NONE',  ( 4.532168488718122390, 8.509556680138327778, 0.7998128361456271485 ) ) ;
#44687=CARTESIAN_POINT ( 'NONE',  ( -6.454563648557663846, 9.688018802362710957, -1.199719254218452047 ) ) ;
#44692=CARTESIAN_POINT ( 'NONE',  ( -5.808742468812186033, 5.741564066561132940, 0.000000000000000000 ) ) ;
#44696=CARTESIAN_POINT ( 'NONE',  ( 5.139949632912227173, 8.050339434155988627, -1.082531754730548412 ) ) ;
#44697=CARTESIAN_POINT ( 'NONE',  ( -5.099275172071237705, 8.963255110809500437, 0.000000000000000000 ) ) ;
#44705=CARTESIAN_POINT ( 'NONE',  ( 5.876533236880477240, 5.820653295974182129, 0.7998128361456352531 ) ) ;
#44730=CARTESIAN_POINT ( 'NONE',  ( 5.146153885717090759, 7.883215235610427918, -1.279915058160858710 ) ) ;
#44734=CARTESIAN_POINT ( 'NONE',  ( 4.629651883607522223, 8.329987488807731211, -0.3686744245932921937 ) ) ;
#44742=CARTESIAN_POINT ( 'NONE',  ( 5.169401708560450004, 9.252995436621013425, 0.000000000000000000 ) ) ;
#44747=CARTESIAN_POINT ( 'NONE',  ( -4.752344554418619360, 8.202642464201909789, 0.7248784622895955154 ) ) ;
#44751=EDGE_CURVE ( 'NONE', #213971, #29321, #112148, .T. ) ;
#44755=CARTESIAN_POINT ( 'NONE',  ( -5.275531169048922386, 5.327410250078064458, -0.7216878364870338292 ) ) ;
#44766=CARTESIAN_POINT ( 'NONE',  ( -4.462568837553487100, 5.235360394347691404, -1.199719254218453823 ) ) ;
#44768=CARTESIAN_POINT ( 'NONE',  ( 5.688527969385528849, 8.794310509995222347, -1.199719254218452047 ) ) ;
#44778=CARTESIAN_POINT ( 'NONE',  ( 3.770049233051776749, 6.556085317605844232, 1.199719254218451159 ) ) ;
#44781=CARTESIAN_POINT ( 'NONE',  ( 4.651856102820254968, 7.480896982382013505, -1.082531754730548412 ) ) ;
#44789=CARTESIAN_POINT ( 'NONE',  ( -6.478676351974181458, 6.772485410396933858, 0.2589597434300341394 ) ) ;
#44793=VERTEX_POINT ( 'NONE', #168036 ) ;
#44797=CARTESIAN_POINT ( 'NONE',  ( -3.959863383643135393, 6.777535159962392086, 1.199719254218452935 ) ) ;
#44798=CARTESIAN_POINT ( 'NONE',  ( 4.913904330310220558, 4.697586238308844919, 0.000000000000000000 ) ) ;
#44801=EDGE_CURVE ( 'NONE', #182295, #71404, #137655, .T. ) ;
#44810=CARTESIAN_POINT ( 'NONE',  ( -4.938913097128142304, 8.984092056616635347, -0.7998128361456362523 ) ) ;
#44811=CARTESIAN_POINT ( 'NONE',  ( -4.014095998097799267, 6.840806543492835345, -1.199719254218450271 ) ) ;
#44813=CARTESIAN_POINT ( 'NONE',  ( 7.499068361690118145, 7.921536974826172361, -0.7216878364870317197 ) ) ;
#44817=CARTESIAN_POINT ( 'NONE',  ( 4.927462483923885195, 4.713404084191450849, -0.7998128361456481317 ) ) ;
#44824=CARTESIAN_POINT ( 'NONE',  ( -6.114219544286552122, 7.015314154546907766, -0.9703045268592332961 ) ) ;
#44832=CARTESIAN_POINT ( 'NONE',  ( -4.055297343818976330, 5.824542549245813383, 1.443375672974065660 ) ) ;
#44849=CARTESIAN_POINT ( 'NONE',  ( 5.071631979963703962, 8.074598522336444262, 1.199719254218451159 ) ) ;
#44869=ADVANCED_FACE ( 'NONE', ( #40173 ), #6573, .F. ) ;
#44876=ORIENTED_EDGE ( 'NONE', *, *, #194169, .T. ) ;
#44882=CARTESIAN_POINT ( 'NONE',  ( -4.370663978927098015, 5.060324124126027279, 1.009771797811723326 ) ) ;
#44885=CARTESIAN_POINT ( 'NONE',  ( 7.024532985656128936, 9.288650798055913427, 1.443375672974065660 ) ) ;
#44889=DIRECTION ( 'NONE',  ( 0.7592566023653005702, -0.6507913734559639396, 0.000000000000000000 ) ) ;
#44913=CARTESIAN_POINT ( 'NONE',  ( -4.197131071882288289, 7.054347462908075350, -1.199719254218455378 ) ) ;
#44915=CARTESIAN_POINT ( 'NONE',  ( 5.736508391913541338, 6.825586224388162648, -1.082531754730548412 ) ) ;
#44920=CARTESIAN_POINT ( 'NONE',  ( -3.630551273409382329, 7.457669928944732796, 0.7998128361456352531 ) ) ;
#44925=CARTESIAN_POINT ( 'NONE',  ( -6.102578539926875933, 10.13377570664109051, 0.7216878364870267237 ) ) ;
#44932=CARTESIAN_POINT ( 'NONE',  ( -5.285699784481336927, 7.260012063351913625, 1.599625672291263179 ) ) ;
#44942=CARTESIAN_POINT ( 'NONE',  ( -5.334207092333882017, 5.187939460669764635, 0.7998128361456281477 ) ) ;
#44945=CARTESIAN_POINT ( 'NONE',  ( -4.475600106286965918, 8.235634200727838916, 0.7216878364870338292 ) ) ;
#44946=CARTESIAN_POINT ( 'NONE',  ( -4.950135482320914271, 8.789258806100786359, -0.7216878364870338292 ) ) ;
#44947=CARTESIAN_POINT ( 'NONE',  ( 5.203297092594585393, 9.292540051327542017, 0.7998128361456341429 ) ) ;
#44948=CARTESIAN_POINT ( 'NONE',  ( -6.119526231721793330, 8.232809585132461194, 1.599625672291263179 ) ) ;
#44986=CARTESIAN_POINT ( 'NONE',  ( 4.626831674679969808, 8.450518883791096059, -0.3637425496919588497 ) ) ;
#45000=CARTESIAN_POINT ( 'NONE',  ( 5.200434439293556643, 8.224868058221247225, -1.199719254218452047 ) ) ;
#45004=CARTESIAN_POINT ( 'NONE',  ( -2.428612866367529932E-14, 2.999999999999999112, 2.420000000000000373 ) ) ;
#45008=CARTESIAN_POINT ( 'NONE',  ( -7.580417283372126391, 8.016444050121833698, 0.7216878364870317197 ) ) ;
#45019=CARTESIAN_POINT ( 'NONE',  ( 4.598150373690133463, 5.393538853173795111, -1.199719254218452047 ) ) ;
#45020=CARTESIAN_POINT ( 'NONE',  ( 6.313256805818848960, 7.394496357324014113, 1.199719254218452047 ) ) ;
#45024=CARTESIAN_POINT ( 'NONE',  ( -4.829398645541163937, 4.822074999085563363, -0.2304323518458932241 ) ) ;
#45028=CARTESIAN_POINT ( 'NONE',  ( 3.410758162289653672, 6.136912401716668519, -1.199719254218453823 ) ) ;
#45034=CARTESIAN_POINT ( 'NONE',  ( 6.873057527484919937, 6.983264968346048818, 0.7998128361456352531 ) ) ;
#45049=CARTESIAN_POINT ( 'NONE',  ( -5.831415467653581430, 5.975941931783510519, 0.7216878364870257245 ) ) ;
#45050=CARTESIAN_POINT ( 'NONE',  ( -5.915100157312088491, 10.12297696016459092, -0.7998128361456362523 ) ) ;
#45058=CARTESIAN_POINT ( 'NONE',  ( 5.275531169048896629, 7.248148678680751189, -1.443375672974078316 ) ) ;
#45063=CARTESIAN_POINT ( 'NONE',  ( -2.972980823146582186, 6.690504403638126263, 0.000000000000000000 ) ) ;
#45064=CARTESIAN_POINT ( 'NONE',  ( 5.013482942003290255, 9.071090208970993274, -0.7998128361456481317 ) ) ;
#45067=CARTESIAN_POINT ( 'NONE',  ( 5.031484404002891431, 5.042689024191078673, 0.7216878364870328300 ) ) ;
#45086=CARTESIAN_POINT ( 'NONE',  ( 5.200434439293556643, 8.224868058221247225, -1.199719254218452047 ) ) ;
#45088=CARTESIAN_POINT ( 'NONE',  ( -3.006876207180748217, 6.730049018344652190, -0.7998128361456481317 ) ) ;
#45092=CARTESIAN_POINT ( 'NONE',  ( 6.561219994370630637, 6.619454513046008515, 0.000000000000000000 ) ) ;
#45102=CARTESIAN_POINT ( 'NONE',  ( 7.349928672384119288, 8.707909884937221179, 1.082531754730549967 ) ) ;
#45104=CARTESIAN_POINT ( 'NONE',  ( -5.582925393777276035, 9.735439736040634173, 0.7998128361456291469 ) ) ;
#45105=CARTESIAN_POINT ( 'NONE',  ( 4.960304097753311936, 6.880383762169266504, 1.599625672291268286 ) ) ;
#45115=CARTESIAN_POINT ( 'NONE',  ( -6.147696309153835692, 6.137010213626392208, 0.7998128361456281477 ) ) ;
#45141=CARTESIAN_POINT ( 'NONE',  ( 3.919715808126649659, 7.587102519540811940, 0.000000000000000000 ) ) ;
#45147=CARTESIAN_POINT ( 'NONE',  ( 4.706088717274895750, 6.583799151611112954, 1.443375672974065660 ) ) ;
#45158=CARTESIAN_POINT ( 'NONE',  ( -4.142898457427624415, 6.991076079377632091, 1.199719254218452935 ) ) ;
#45160=CARTESIAN_POINT ( 'NONE',  ( -7.910256278930404505, 8.193330178365746619, -0.7998128361456362523 ) ) ;
#45162=CARTESIAN_POINT ( 'NONE',  ( 6.577113915960825175, 8.766661883411348555, -1.443375672974078761 ) ) ;
#45166=CARTESIAN_POINT ( 'NONE',  ( -3.795153912786186634, 7.352191159395610853, -0.7064407198300488577 ) ) ;
#45172=CARTESIAN_POINT ( 'NONE',  ( -5.608757509019812737, 5.629195651549657065, 0.4603112365162060904 ) ) ;
#45173=CARTESIAN_POINT ( 'NONE',  ( -5.641074431737709283, 8.738948049406083385, -1.199719254218452047 ) ) ;
#45179=CARTESIAN_POINT ( 'NONE',  ( -3.851925040058333582, 7.508013290127760087, -0.7216878364870458196 ) ) ;
#45181=VERTEX_POINT ( 'NONE', #153393 ) ;
#45183=CARTESIAN_POINT ( 'NONE',  ( -6.120580001926503755, 6.105374521861167914, -0.7998128361456362523 ) ) ;
#45202=EDGE_LOOP ( 'NONE', ( #102903, #4276, #100395, #67535, #51300 ) ) ;
#45203=CARTESIAN_POINT ( 'NONE',  ( -6.967964602780620353, 7.093989889524320525, 0.000000000000000000 ) ) ;
#45205=CARTESIAN_POINT ( 'NONE',  ( -5.655686355556086120, 6.627330832017406692, 1.199719254218452935 ) ) ;
#45214=DIRECTION ( 'NONE',  ( -0.000000000000000000, -1.000000000000000000, -0.000000000000000000 ) ) ;
#45216=VERTEX_POINT ( 'NONE', #70642 ) ;
#45228=CARTESIAN_POINT ( 'NONE',  ( -5.064290697676250730, 7.960144884870772763, -1.236948567437242907 ) ) ;
#45229=CARTESIAN_POINT ( 'NONE',  ( -7.282664789195997912, 8.525472337930658284, 1.199719254218452047 ) ) ;
#45254=CARTESIAN_POINT ( 'NONE',  ( 7.180978637093494044, 8.406838493811077839, -1.199719254218452047 ) ) ;
#45266=CARTESIAN_POINT ( 'NONE',  ( 5.264264421420239870, 7.666326994050936428, 1.218248458220503094 ) ) ;
#45268=CARTESIAN_POINT ( 'NONE',  ( 7.078765600110826561, 8.391552967285011988, -1.082531754730548412 ) ) ;
#45273=CARTESIAN_POINT ( 'NONE',  ( -6.147696309153835692, 6.137010213626392208, 0.7998128361456281477 ) ) ;
#45280=CARTESIAN_POINT ( 'NONE',  ( -5.221298554594238084, 8.145246509451649075, 1.082531754730549967 ) ) ;
#45283=CARTESIAN_POINT ( 'NONE',  ( -4.000724900121314320, 7.680942274213022003, 0.03569885272684778649 ) ) ;
#45300=CARTESIAN_POINT ( 'NONE',  ( 5.657495238652423097, 9.822437888394988548, 0.000000000000000000 ) ) ;
#45306=DIRECTION ( 'NONE',  ( -0.6507913734559658270, 0.7592566023652989049, 0.000000000000000000 ) ) ;
#45320=CARTESIAN_POINT ( 'NONE',  ( -6.291865805193673111, 9.498204651771386509, -1.199719254218452047 ) ) ;
#45321=CARTESIAN_POINT ( 'NONE',  ( 4.260029445439534435, 7.236136616047147641, 2.499999999999999556 ) ) ;
#45322=CARTESIAN_POINT ( 'NONE',  ( 5.722423353419669567, 8.833855124701747386, 1.199719254218451159 ) ) ;
#45324=CARTESIAN_POINT ( 'NONE',  ( -5.349061533644712263, 7.606979636585072591, 1.237473162191610188 ) ) ;
#45331=CARTESIAN_POINT ( 'NONE',  ( 4.583538449871731757, 7.505156070562471804, 1.199719254218451159 ) ) ;
#45334=CARTESIAN_POINT ( 'NONE',  ( -5.567429050782688904, 5.875295893689919779, -0.7230728617713001460 ) ) ;
#45339=CARTESIAN_POINT ( 'NONE',  ( 3.092668437693027794, 6.622213920701574885, -0.7216878364870338292 ) ) ;
#45343=CARTESIAN_POINT ( 'NONE',  ( 4.082413651490639062, 7.776916670132135501, 0.000000000000000000 ) ) ;
#45344=VERTEX_POINT ( 'NONE', #20827 ) ;
#45351=CARTESIAN_POINT ( 'NONE',  ( -2.820451594992841482, 6.512553637458760036, 0.000000000000000000 ) ) ;
#45354=CARTESIAN_POINT ( 'NONE',  ( -5.804299160426237059, 7.865044668620976509, -1.443375672974066548 ) ) ;
#45366=AXIS2_PLACEMENT_3D ( 'NONE', #63584, #9501, #47360 ) ;
#45378=CARTESIAN_POINT ( 'NONE',  ( 3.696970665278032975, 7.535159219458173574, -0.4808056554564468787 ) ) ;
#45385=ORIENTED_EDGE ( 'NONE', *, *, #23022, .T. ) ;
#45389=CARTESIAN_POINT ( 'NONE',  ( 4.044074958626150185, 7.940114228364351767, 0.7998128361456271485 ) ) ;
#45401=CARTESIAN_POINT ( 'NONE',  ( -7.932929277771797238, 8.427708043588125975, 0.000000000000000000 ) ) ;
#45404=CARTESIAN_POINT ( 'NONE',  ( 3.838366886000300404, 6.531826229425389485, -1.082531754730548412 ) ) ;
#45421=CARTESIAN_POINT ( 'NONE',  ( -4.421367491832313590, 6.251624388594711590, 1.443375672974065660 ) ) ;
#45422=CARTESIAN_POINT ( 'NONE',  ( 5.558836782162523527, 7.518240855878357110, -1.384758111419038817 ) ) ;
#45428=CARTESIAN_POINT ( 'NONE',  ( -4.824649217201493201, 7.689440087634505261, -1.092232977752989331 ) ) ;
#45431=EDGE_CURVE ( 'NONE', #43808, #127442, #37262, .T. ) ;
#45457=CARTESIAN_POINT ( 'NONE',  ( -5.752402313948099533, 9.933162809573264695, -0.7998128361456362523 ) ) ;
#45458=CARTESIAN_POINT ( 'NONE',  ( -5.227029541856937023, 7.814379162078399332, 1.287352361829100733 ) ) ;
#45462=CARTESIAN_POINT ( 'NONE',  ( -6.075462232255183892, 10.10214001435745246, 0.000000000000000000 ) ) ;
#45465=CARTESIAN_POINT ( 'NONE',  ( -2.830620210203090181, 6.524417021870718258, 0.000000000000000000 ) ) ;
#45468=CARTESIAN_POINT ( 'NONE',  ( -3.657667580636712934, 7.489305620709952649, -0.7998128361456481317 ) ) ;
#45471=AXIS2_PLACEMENT_3D ( 'NONE', #110262, #45214, #145927 ) ;
#45484=CARTESIAN_POINT ( 'NONE',  ( 4.050854035433010480, 7.948023151305657841, 0.000000000000000000 ) ) ;
#45507=CARTESIAN_POINT ( 'NONE',  ( 4.583538449871731757, 7.505156070562471804, 1.199719254218451159 ) ) ;
#45508=CARTESIAN_POINT ( 'NONE',  ( 3.074666975249065626, 6.809138247757705820, 0.000000000000000000 ) ) ;
#45513=DIRECTION ( 'NONE',  ( 0.6507913734559641616, -0.7592566023653004592, 0.000000000000000000 ) ) ;
#45523=CARTESIAN_POINT ( 'NONE',  ( 4.812217717264355876, 8.234349973070900219, 0.8868998539744571419 ) ) ;
#45524=CARTESIAN_POINT ( 'NONE',  ( -4.773879485343255347, 8.583626809626847987, 0.000000000000000000 ) ) ;
#45539=ORIENTED_EDGE ( 'NONE', *, *, #25456, .T. ) ;
#45553=CARTESIAN_POINT ( 'NONE',  ( 5.041653019435334393, 6.975290837464928728, -1.599625672291269396 ) ) ;
#45571=CARTESIAN_POINT ( 'NONE',  ( -6.770317605177755382, 8.992066187497757213, 1.599625672291269396 ) ) ;
#45576=CARTESIAN_POINT ( 'NONE',  ( -5.608757509019735465, 5.634241678024821454, 0.4696088000558009679 ) ) ;
#45582=CARTESIAN_POINT ( 'NONE',  ( 5.020262018810099924, 9.078999131912302900, 0.7998128361456331437 ) ) ;
#45588=CARTESIAN_POINT ( 'NONE',  ( 6.547661840756936691, 6.603636667163397256, 0.7998128361456352531 ) ) ;
#45594=EDGE_CURVE ( 'NONE', #135468, #84217, #148224, .T. ) ;
#45599=CARTESIAN_POINT ( 'NONE',  ( 4.646267551848549004, 8.309382712783076386, 0.4446711254955729165 ) ) ;
#45618=CARTESIAN_POINT ( 'NONE',  ( -6.656127069666307072, 6.730179434224282886, 0.7998128361456341429 ) ) ;
#45620=CARTESIAN_POINT ( 'NONE',  ( 5.387385936583818591, 7.378645907471495846, -1.599625672291283607 ) ) ;
#45624=CARTESIAN_POINT ( 'NONE',  ( -6.291865805193673111, 9.498204651771386509, -1.199719254218452047 ) ) ;
#45632=CARTESIAN_POINT ( 'NONE',  ( -6.026230196168996578, 7.163122537909742071, -1.192248477780058380 ) ) ;
#45650=CARTESIAN_POINT ( 'NONE',  ( 5.506019780925567986, 8.477421273504887722, -1.082531754730548412 ) ) ;
#45670=CARTESIAN_POINT ( 'NONE',  ( 4.817943484809818600, 6.714296380401858499, 1.599625672291269396 ) ) ;
#45701=ORIENTED_EDGE ( 'NONE', *, *, #83796, .T. ) ;
#45712=ORIENTED_EDGE ( 'NONE', *, *, #81748, .T. ) ;
#45720=CARTESIAN_POINT ( 'NONE',  ( 5.695833931072550094, 5.817763472438987726, 0.000000000000000000 ) ) ;
#45723=ORIENTED_EDGE ( 'NONE', *, *, #38054, .T. ) ;
#45724=CARTESIAN_POINT ( 'NONE',  ( -4.136646265500958819, 7.840188053144158786, -0.7216878364870458196 ) ) ;
#45725=CARTESIAN_POINT ( 'NONE',  ( 0.000000000000000000, 8.999999999999998224, 0.000000000000000000 ) ) ;
#45730=CARTESIAN_POINT ( 'NONE',  ( -5.448397627845328550, 7.449826213943242514, 1.599625672291263179 ) ) ;
#45739=CARTESIAN_POINT ( 'NONE',  ( -3.657667580636712934, 7.489305620709952649, -0.7998128361456481317 ) ) ;
#45742=CARTESIAN_POINT ( 'NONE',  ( 6.536750166778501736, 6.811520125210166476, 0.4662371894542677864 ) ) ;
#45747=CARTESIAN_POINT ( 'NONE',  ( 5.071631979963703962, 8.074598522336444262, 1.199719254218451159 ) ) ;
#45753=CARTESIAN_POINT ( 'NONE',  ( -5.164730172163054966, 4.990216387137135889, -0.7998128361456362523 ) ) ;
#45758=CARTESIAN_POINT ( 'NONE',  ( -4.437261413422502798, 8.398831758960053406, 0.000000000000000000 ) ) ;
#45763=CARTESIAN_POINT ( 'NONE',  ( 5.017926250389229459, 8.868348035513836436, 0.000000000000000000 ) ) ;
#45765=CARTESIAN_POINT ( 'NONE',  ( -5.709392084686210289, 8.714688961225625974, 1.082531754730550855 ) ) ;
#45773=CARTESIAN_POINT ( 'NONE',  ( 4.179656494762836516, 8.098292687190454586, -0.7998128361456362523 ) ) ;
#45779=CARTESIAN_POINT ( 'NONE',  ( 6.378184920586140727, 6.405913593630768510, 0.000000000000000000 ) ) ;
#45799=ORIENTED_EDGE ( 'NONE', *, *, #77256, .T. ) ;
#45801=CARTESIAN_POINT ( 'NONE',  ( 4.607663176575717223, 8.357619647684677133, 0.2284409323990380658 ) ) ;
#45809=CARTESIAN_POINT ( 'NONE',  ( 4.993145711582793744, 9.047363440147082159, -0.7998128361456481317 ) ) ;
#45814=CARTESIAN_POINT ( 'NONE',  ( -4.638545736399841246, 8.340143690112583386, 0.3695662286686048903 ) ) ;
#45820=CARTESIAN_POINT ( 'NONE',  ( -5.302647476276252547, 5.359045941843285199, 0.7216878364870257245 ) ) ;
#45830=CARTESIAN_POINT ( 'NONE',  ( -3.006876207180748217, 6.730049018344652190, -0.7998128361456481317 ) ) ;
#45843=CARTESIAN_POINT ( 'NONE',  ( 4.366607992053101128, 7.252070536440704096, -1.199719254218448494 ) ) ;
#45846=CARTESIAN_POINT ( 'NONE',  ( 6.672020991256494504, 6.956648375986938859, 0.000000000000000000 ) ) ;
#45854=CARTESIAN_POINT ( 'NONE',  ( -6.502161524297833672, 6.757477167027320597, -0.005777863564433716181 ) ) ;
#45858=ORIENTED_EDGE ( 'NONE', *, *, #15314, .F. ) ;
#45861=CARTESIAN_POINT ( 'NONE',  ( -3.135678666510573365, 6.880318554229450712, 0.000000000000000000 ) ) ;
#45862=CARTESIAN_POINT ( 'NONE',  ( 4.903208829997618423, 5.749440385532527564, -1.199719254218450271 ) ) ;
#45872=CARTESIAN_POINT ( 'NONE',  ( -5.264308783856126439, 9.363720357799287797, -0.7998128361456362523 ) ) ;
#45873=CARTESIAN_POINT ( 'NONE',  ( 6.367489420273535039, 7.457767740854454708, -1.199719254218452047 ) ) ;
#45875=CARTESIAN_POINT ( 'NONE',  ( 6.156811153937166381, 10.19704708965311468, 0.000000000000000000 ) ) ;
#45887=CARTESIAN_POINT ( 'NONE',  ( -5.857301623663916601, 7.199535845156014524, -1.157093103336486628 ) ) ;
#45895=CARTESIAN_POINT ( 'NONE',  ( -6.851666526859749418, 9.086973262793417661, -1.599625672291271394 ) ) ;
#45905=CARTESIAN_POINT ( 'NONE',  ( -5.346851039111045978, 6.199209027673978412, -1.060622344683157747 ) ) ;
#45914=CARTESIAN_POINT ( 'NONE',  ( 5.169401708560450004, 9.252995436621013425, 0.000000000000000000 ) ) ;
#45947=CARTESIAN_POINT ( 'NONE',  ( 4.577813143269636065, 5.369812084349879555, -1.199719254218450271 ) ) ;
#45977=CARTESIAN_POINT ( 'NONE',  ( -4.793689830883590020, 7.750332681742931662, 1.199719254218452935 ) ) ;
#45979=CARTESIAN_POINT ( 'NONE',  ( 7.010974831598141499, 7.352094523052197239, -0.7216878364870317197 ) ) ;
#45984=CARTESIAN_POINT ( 'NONE',  ( -4.736594563127865420, 6.619389305106191834, -1.599625672291271394 ) ) ;
#45990=CARTESIAN_POINT ( 'NONE',  ( -4.821859908315634158, 5.654533310236863564, 1.199719254218452935 ) ) ;
#45997=CARTESIAN_POINT ( 'NONE',  ( -5.743814354044916470, 6.730146830254374990, -1.199719254218453823 ) ) ;
#46006=CARTESIAN_POINT ( 'NONE',  ( -5.795184315198522285, 5.725746220678519904, -0.7998128361456362523 ) ) ;
#46009=CARTESIAN_POINT ( 'NONE',  ( -6.468648687495877958, 6.719380688266201496, 0.000000000000000000 ) ) ;
#46011=CARTESIAN_POINT ( 'NONE',  ( -7.092323753280154186, 7.447001598347859463, 0.7216878364870317197 ) ) ;
#46012=CARTESIAN_POINT ( 'NONE',  ( 6.176621499477501054, 9.363752961769195693, -1.199719254218452047 ) ) ;
#46013=CARTESIAN_POINT ( 'NONE',  ( -5.284646014276622950, 9.387447126623207794, -0.7998128361456362523 ) ) ;
#46050=CARTESIAN_POINT ( 'NONE',  ( 4.890561790263044273, 8.149264200713410844, -1.004099907704804950 ) ) ;
#46064=CARTESIAN_POINT ( 'NONE',  ( 6.333594036239346359, 7.418223126147930557, 1.199719254218453823 ) ) ;
#46067=CARTESIAN_POINT ( 'NONE',  ( -4.468294144155606773, 7.370704380560280100, 1.199719254218452935 ) ) ;
#46071=CARTESIAN_POINT ( 'NONE',  ( -6.794044373779495771, 8.059378203231773341, 1.082531754730549078 ) ) ;
#46083=CARTESIAN_POINT ( 'NONE',  ( 4.435452530326143616, 5.203724702582467998, -1.199719254218452047 ) ) ;
#46084=CARTESIAN_POINT ( 'NONE',  ( 7.042534447655770080, 7.180988041878682004, -0.7998128361456341429 ) ) ;
#46099=ORIENTED_EDGE ( 'NONE', *, *, #189724, .T. ) ;
#46100=CARTESIAN_POINT ( 'NONE',  ( 5.254667053748194760, 8.288139441751686931, 1.199719254218452047 ) ) ;
#46112=CARTESIAN_POINT ( 'NONE',  ( -4.312902262922974295, 8.045820050136510915, 0.7216878364870338292 ) ) ;
#46113=CARTESIAN_POINT ( 'NONE',  ( -6.749980374757255319, 8.968339418673846097, 1.599625672291269396 ) ) ;
#46125=DIRECTION ( 'NONE',  ( 0.7592566023653005702, 0.6507913734559639396, 0.000000000000000000 ) ) ;
#46126=CARTESIAN_POINT ( 'NONE',  ( 7.147083253059300922, 8.367293879104554577, 1.199719254218452935 ) ) ;
#46129=CARTESIAN_POINT ( 'NONE',  ( 3.892599500454941630, 6.595097612955829192, 1.082531754730549078 ) ) ;
#46149=CARTESIAN_POINT ( 'NONE',  ( 4.929271367020211514, 7.908511140569038922, 1.199719254218452047 ) ) ;
#46151=CARTESIAN_POINT ( 'NONE',  ( -3.169574050544739841, 6.919863168935977527, -0.7998128361456481317 ) ) ;
#46163=CARTESIAN_POINT ( 'NONE',  ( 6.048345925472178308, 9.110135108809304327, 1.082531754730549967 ) ) ;
#46165=CARTESIAN_POINT ( 'NONE',  ( -5.498713818794216834, 8.572860667638675380, -1.199719254218452047 ) ) ;
#46166=CARTESIAN_POINT ( 'NONE',  ( 5.987861119090863049, 7.014868056141362551, 1.199719254218452047 ) ) ;
#46175=CARTESIAN_POINT ( 'NONE',  ( -5.581116510680924847, 6.540332679663050541, -1.199719254218453823 ) ) ;
#46202=CARTESIAN_POINT ( 'NONE',  ( 5.411112705629925301, 5.485588709422586362, 0.000000000000000000 ) ) ;
#46208=CARTESIAN_POINT ( 'NONE',  ( 4.326460416092276162, 7.101268681199365496, -1.082531754730548412 ) ) ;
#46215=ADVANCED_FACE ( 'NONE', ( #39681 ), #20102, .T. ) ;
#46222=CARTESIAN_POINT ( 'NONE',  ( -6.306477729012051725, 7.386587434382707151, 1.199719254218452047 ) ) ;
#46224=CARTESIAN_POINT ( 'NONE',  ( -7.435720902452096936, 7.639705572474380091, 0.000000000000000000 ) ) ;
#46230=CARTESIAN_POINT ( 'NONE',  ( 7.849244587668864348, 8.122149871893999062, 0.7998128361456291469 ) ) ;
#46235=CARTESIAN_POINT ( 'NONE',  ( -5.960744811863571968, 6.983232364376142698, 1.199719254218452935 ) ) ;
#46241=CARTESIAN_POINT ( 'NONE',  ( -5.831415467653581430, 5.975941931783510519, 0.7216878364870257245 ) ) ;
#46244=CARTESIAN_POINT ( 'NONE',  ( -6.459533842268148973, 6.500820668926428958, 0.000000000000000000 ) ) ;
#46264=CARTESIAN_POINT ( 'NONE',  ( -4.516274566683622815, 5.401980094953223066, 1.082531754730549078 ) ) ;
#46266=CARTESIAN_POINT ( 'NONE',  ( -4.305596300791617814, 7.180890229968955651, 1.199719254218452935 ) ) ;
#46280=EDGE_CURVE ( 'NONE', #154266, #70814, #179234, .T. ) ;
#46293=CARTESIAN_POINT ( 'NONE',  ( -6.444921918449773024, 8.612437886315108315, 1.599625672291269396 ) ) ;
#46295=CIRCLE ( 'NONE', #87704, 0.07999999999999997391 ) ;
#46317=CARTESIAN_POINT ( 'NONE',  ( 6.556249800660121529, 9.806652646482286073, 1.199719254218452047 ) ) ;
#46318=CARTESIAN_POINT ( 'NONE',  ( 6.535912570239620578, 9.782925877658371405, 1.199719254218452047 ) ) ;
#46332=CARTESIAN_POINT ( 'NONE',  ( 4.826264338009964128, 8.099924789650724932, 0.8724150771263041726 ) ) ;
#46334=CARTESIAN_POINT ( 'NONE',  ( 6.292392690518195941, 8.434487120394948079, -1.443375672974078761 ) ) ;
#46340=CARTESIAN_POINT ( 'NONE',  ( -5.204350862799341115, 7.165104988056252289, -1.599625672291271394 ) ) ;
#46345=AXIS2_PLACEMENT_3D ( 'NONE', #49926, #151705, #201474 ) ;
#46346=CARTESIAN_POINT ( 'NONE',  ( -6.007671464186866928, 8.102312356341712984, 1.443375672974058777 ) ) ;
#46362=CARTESIAN_POINT ( 'NONE',  ( 7.679767667498067496, 7.924426798361372093, 0.000000000000000000 ) ) ;
#46384=CARTESIAN_POINT ( 'NONE',  ( 6.261886844665240481, 8.398896966899865646, 1.599625672291268286 ) ) ;
#46386=CARTESIAN_POINT ( 'NONE',  ( -5.710744021720588925, 7.310394840978843511, 1.216594670743395445 ) ) ;
#46393=CARTESIAN_POINT ( 'NONE',  ( 4.692003678781083487, 7.631698837623355658, -1.199719254218450271 ) ) ;
#46400=CARTESIAN_POINT ( 'NONE',  ( 4.909461021924256485, 4.900328411765999981, 0.7216878364870338292 ) ) ;
#46404=CARTESIAN_POINT ( 'NONE',  ( 4.746763178560241769, 8.551991118380046331, 0.7216878364870328300 ) ) ;
#46415=CARTESIAN_POINT ( 'NONE',  ( -5.316205630334263965, 7.295602216847000498, -1.443375672974066548 ) ) ;
#46448=CARTESIAN_POINT ( 'NONE',  ( 6.554440917563797875, 6.611545590104705994, -0.7998128361456481317 ) ) ;
#46450=CARTESIAN_POINT ( 'NONE',  ( 6.547661840756936691, 6.603636667163397256, 0.7998128361456352531 ) ) ;
#46460=CARTESIAN_POINT ( 'NONE',  ( -4.442231607132987925, 5.211633625523774960, -1.199719254218453823 ) ) ;
#46463=CARTESIAN_POINT ( 'NONE',  ( 6.007671464186837618, 6.181573927739029806, 0.7216878364870328300 ) ) ;
#46478=CARTESIAN_POINT ( 'NONE',  ( -6.943184063974186415, 7.273005294157565359, -0.7216878364870338292 ) ) ;
#46480=CARTESIAN_POINT ( 'NONE',  ( -4.502716413514301408, 7.306900678191715848, -1.082531754730549967 ) ) ;
#46484=CARTESIAN_POINT ( 'NONE',  ( -5.614485009390564940, 5.722856397143323726, 0.000000000000000000 ) ) ;
#46488=CARTESIAN_POINT ( 'NONE',  ( 3.540436255445079894, 7.352535741319725204, -0.1172168222480891864 ) ) ;
#46520=CARTESIAN_POINT ( 'NONE',  ( -6.563028877466991595, 9.814561569423593923, 1.199719254218452935 ) ) ;
#46521=CARTESIAN_POINT ( 'NONE',  ( -4.601933621211449221, 8.477299672830683974, 0.2703350597391823706 ) ) ;
#46530=CARTESIAN_POINT ( 'NONE',  ( -3.481411583659053566, 7.283673624236017830, 0.000000000000000000 ) ) ;
#46533=CARTESIAN_POINT ( 'NONE',  ( -5.276058054373441664, 6.184431147304315424, -1.199719254218453823 ) ) ;
#46545=CARTESIAN_POINT ( 'NONE',  ( 6.398522151006641678, 6.429640362454684954, 0.000000000000000000 ) ) ;
#46549=CARTESIAN_POINT ( 'NONE',  ( 0.1377316631404259251, 3.380484790530137840, -2.074674412079231089 ) ) ;
#46569=CARTESIAN_POINT ( 'NONE',  ( 6.540882763950133238, 6.595727744222092959, 0.000000000000000000 ) ) ;
#46570=CARTESIAN_POINT ( 'NONE',  ( 4.736594563127852098, 6.619389305106191834, -1.599625672291273171 ) ) ;
#46575=DIRECTION ( 'NONE',  ( 0.7592566023653005702, 0.6507913734559639396, 0.000000000000000000 ) ) ;
#46585=CARTESIAN_POINT ( 'NONE',  ( 5.502223863662048409, 7.574938096329499437, 1.338028725624084148 ) ) ;
#46586=CARTESIAN_POINT ( 'NONE',  ( -4.611181641979265500, 8.393812659035525314, 0.000000000000000000 ) ) ;
#46587=CARTESIAN_POINT ( 'NONE',  ( 3.851925040058331806, 5.587274861525073355, -1.443375672974066548 ) ) ;
#46613=CARTESIAN_POINT ( 'NONE',  ( 6.066347387471824781, 6.042103138330730872, -0.7998128361456481317 ) ) ;
#46615=CARTESIAN_POINT ( 'NONE',  ( 3.562760505341037831, 7.378580699531681830, -1.734723475976807094E-15 ) ) ;
#46631=CARTESIAN_POINT ( 'NONE',  ( -8.093291352714894415, 8.406871097780989288, -0.7998128361456362523 ) ) ;
#46643=CARTESIAN_POINT ( 'NONE',  ( 6.866278450678116485, 6.975356045404744521, 0.000000000000000000 ) ) ;
#46649=CARTESIAN_POINT ( 'NONE',  ( 5.091969210384201361, 8.098325291160362482, 1.199719254218452047 ) ) ;
#46661=CARTESIAN_POINT ( 'NONE',  ( -4.624739795592936353, 7.449261290616792763, -1.082531754730549967 ) ) ;
#46662=CARTESIAN_POINT ( 'NONE',  ( 4.600487305768355739, 8.366733224642864286, -0.1591645125929436189 ) ) ;
#46674=CARTESIAN_POINT ( 'NONE',  ( -6.305084897752638362, 6.885715524493735806, 0.7263500631976427258 ) ) ;
#46677=( BOUNDED_SURFACE ( )  B_SPLINE_SURFACE ( 3, 2, ( 
 ( #122285, #24673, #204474 ),
 ( #155765, #52917, #86488 ),
 ( #88638, #22529, #36659 ),
 ( #57194, #137390, #55059 ),
 ( #70208, #102744, #121210 ),
 ( #168800, #173092, #156841 ),
 ( #152552, #136320, #202338 ),
 ( #153630, #53991, #187179 ) ),
 .UNSPECIFIED., .F., .F., .F. ) 
 B_SPLINE_SURFACE_WITH_KNOTS ( ( 4, 2, 2, 4 ),
 ( 3, 3 ),
 ( 0.000000000000000000, 0.003135730046001661882, 0.004703595069002492607, 0.006271460092003323765 ),
 ( 0.000000000000000000, 1.000000000000000000 ),
 .UNSPECIFIED. ) 
 GEOMETRIC_REPRESENTATION_ITEM ( )  RATIONAL_B_SPLINE_SURFACE ( (
 ( 1.000000000000000000, 0.7762074382822415908, 1.000000000000000000),
 ( 1.000000000000000000, 0.7833603871956243969, 1.000000000000000000),
 ( 1.000000000000000000, 0.7921476697835092562, 1.000000000000000000),
 ( 1.000000000000000000, 0.8128220030700816778, 1.000000000000000000),
 ( 1.000000000000000000, 0.8210052159720273579, 1.000000000000000000),
 ( 1.000000000000000000, 0.8412342355963777774, 1.000000000000000000),
 ( 1.000000000000000000, 0.8534349975675549205, 1.000000000000000000),
 ( 1.000000000000000000, 0.8671614222306939235, 1.000000000000000000) ) ) 
 REPRESENTATION_ITEM ( '' )  SURFACE ( )  );
#46684=CARTESIAN_POINT ( 'NONE',  ( -6.414942957921379474, 7.513130201443591005, -1.199719254218452047 ) ) ;
#46686=CARTESIAN_POINT ( 'NONE',  ( 6.561219994370630637, 6.619454513046008515, 0.000000000000000000 ) ) ;
#46691=CARTESIAN_POINT ( 'NONE',  ( -7.923814432544069142, 8.209148024248356990, 0.000000000000000000 ) ) ;
#46694=CARTESIAN_POINT ( 'NONE',  ( 6.339319342841494453, 9.553567112360518365, -1.199719254218452047 ) ) ;
#46699=CARTESIAN_POINT ( 'NONE',  ( -6.581660514134937578, 6.779899958900003298, -0.3344319070191399401 ) ) ;
#46709=AXIS2_PLACEMENT_3D ( 'NONE', #39397, #154218, #55643 ) ;
#46713=CARTESIAN_POINT ( 'NONE',  ( 3.599450258230072475, 3.565770338845029919, 2.499999999999999112 ) ) ;
#46718=ORIENTED_EDGE ( 'NONE', *, *, #33948, .F. ) ;
#46719=CARTESIAN_POINT ( 'NONE',  ( 7.051649292883499953, 7.399548061218447437, -0.7216878364870317197 ) ) ;
#46728=CARTESIAN_POINT ( 'NONE',  ( 7.065207446497155708, 9.336104335703744539, 0.000000000000000000 ) ) ;
#46735=CARTESIAN_POINT ( 'NONE',  ( -4.421367491832313590, 6.251624388594711590, 1.443375672974065660 ) ) ;
#46738=CARTESIAN_POINT ( 'NONE',  ( 4.227110032410640095, 8.153655147779589996, 0.7998128361456271485 ) ) ;
#46752=B_SPLINE_CURVE_WITH_KNOTS ( 'NONE', 3,
 ( #194132, #144375, #65180, #163787, #111899, #47925, #29515, #97729 ),
 .UNSPECIFIED., .F., .F.,
 ( 4, 2, 2, 4 ),
 ( 0.000000000000000000, 0.001555696184809488535, 0.003111392369618977069, 0.006222784739237952403 ),
 .UNSPECIFIED. ) ;
#46758=CARTESIAN_POINT ( 'NONE',  ( 7.960045584554727327, 8.459343734834927631, 0.7216878364870267237 ) ) ;
#46782=CARTESIAN_POINT ( 'NONE',  ( 3.106226591306694651, 6.638031766584184368, 0.000000000000000000 ) ) ;
#46792=CARTESIAN_POINT ( 'NONE',  ( -4.245111494410291897, 7.006361605903701495, 1.082531754730549967 ) ) ;
#46799=CARTESIAN_POINT ( 'NONE',  ( -4.773352600463090845, 7.726605912919016106, 1.199719254218452935 ) ) ;
#46807=CARTESIAN_POINT ( 'NONE',  ( -5.679940009482361774, 5.591294530676332641, 0.7998128361456281477 ) ) ;
#46809=CARTESIAN_POINT ( 'NONE',  ( 6.472394699177205446, 6.854181287346997387, 0.6349317888264572884 ) ) ;
#46814=CARTESIAN_POINT ( 'NONE',  ( 6.391743074199808916, 6.421731439513382433, -0.7998128361456481317 ) ) ;
#46822=CARTESIAN_POINT ( 'NONE',  ( -4.787964524281469458, 5.614988695530339413, -1.199719254218453823 ) ) ;
#46828=CARTESIAN_POINT ( 'NONE',  ( -5.635349125135588721, 6.603604063193491136, 1.199719254218452935 ) ) ;
#46832=CARTESIAN_POINT ( 'NONE',  ( 5.167065940139554669, 9.042344340222555843, -0.7216878364870458196 ) ) ;
#46834=CARTESIAN_POINT ( 'NONE',  ( -6.143253000323532831, 7.300121600866474658, 1.082531754730548412 ) ) ;
#46840=CARTESIAN_POINT ( 'NONE',  ( 4.908934136599710563, 7.884784371745123366, 1.199719254218451159 ) ) ;
#46847=CARTESIAN_POINT ( 'NONE',  ( 6.229045230835819069, 6.231917288922055320, -0.7998128361456481317 ) ) ;
#46883=CARTESIAN_POINT ( 'NONE',  ( -6.237206930280429162, 6.931128591455327559, -0.8289643595828979361 ) ) ;
#46890=CARTESIAN_POINT ( 'NONE',  ( -3.594320120954326292, 6.247105003538398371, 1.082531754730549967 ) ) ;
#46901=CARTESIAN_POINT ( 'NONE',  ( -2.979759899953417612, 6.698413326579433225, 0.7998128361456352531 ) ) ;
#46906=ORIENTED_EDGE ( 'NONE', *, *, #78821, .F. ) ;
#46910=CARTESIAN_POINT ( 'NONE',  ( 5.903649544107831382, 5.852288987739402870, -0.7998128361456481317 ) ) ;
#46913=CARTESIAN_POINT ( 'NONE',  ( 5.519577934094861860, 6.572500690266394940, 1.082531754730549078 ) ) ;
#46927=CARTESIAN_POINT ( 'NONE',  ( -4.797606254389363833, 6.690569611577942943, 1.599625672291263179 ) ) ;
#46928=CARTESIAN_POINT ( 'NONE',  ( 5.228604516725597229, 6.129068686715179126, -1.199719254218450271 ) ) ;
#46939=CARTESIAN_POINT ( 'NONE',  ( -7.099629715411508890, 8.311931418515415615, 1.199719254218452047 ) ) ;
#46940=CARTESIAN_POINT ( 'NONE',  ( 6.866278450678116485, 6.975356045404744521, 0.000000000000000000 ) ) ;
#46954=CARTESIAN_POINT ( 'NONE',  ( -6.502837976706968171, 6.831778935668112673, 0.5908271424688981144 ) ) ;
#46958=EDGE_CURVE ( 'NONE', #175863, #136449, #79977, .T. ) ;
#46962=CARTESIAN_POINT ( 'NONE',  ( -5.126391479298592735, 5.153413945369351268, 0.000000000000000000 ) ) ;
#46978=EDGE_CURVE ( 'NONE', #123356, #110637, #140493, .T. ) ;
#46979=CARTESIAN_POINT ( 'NONE',  ( 6.855582950365507244, 8.027210192628430718, -1.199719254218452047 ) ) ;
#47012=CARTESIAN_POINT ( 'NONE',  ( 3.366167277942881064, 7.149221934233827014, -0.7998128361456362523 ) ) ;
#47044=CARTESIAN_POINT ( 'NONE',  ( -6.330731382938325602, 6.350551133041632212, 0.7998128361456281477 ) ) ;
#47045=EDGE_CURVE ( 'NONE', #35911, #158170, #31617, .T. ) ;
#47047=CARTESIAN_POINT ( 'NONE',  ( 7.160114521348466710, 7.526090827760914870, 0.000000000000000000 ) ) ;
#47052=CARTESIAN_POINT ( 'NONE',  ( -4.294900800479008574, 8.232744377192641849, 0.000000000000000000 ) ) ;
#47056=DIRECTION ( 'NONE',  ( -1.000000000000000000, 0.000000000000000000, 0.000000000000000000 ) ) ;
#47057=CARTESIAN_POINT ( 'NONE',  ( -3.149236820124241110, 6.896136400112061970, -0.7998128361456481317 ) ) ;
#47062=CARTESIAN_POINT ( 'NONE',  ( -5.936491157937300756, 8.019268665717216749, 1.599625672291263179 ) ) ;
#47073=CARTESIAN_POINT ( 'NONE',  ( -3.800028193580205382, 7.655393002477360653, -0.7998128361456481317 ) ) ;
#47076=CARTESIAN_POINT ( 'NONE',  ( -5.139949633356594383, 9.010708648975750634, 0.000000000000000000 ) ) ;
#47077=CARTESIAN_POINT ( 'NONE',  ( -5.763624699140874164, 8.777960344756069233, -1.082531754730549967 ) ) ;
#47078=CARTESIAN_POINT ( 'NONE',  ( 6.933015448541703485, 9.181880338089085214, 1.599625672291268286 ) ) ;
#47079=CARTESIAN_POINT ( 'NONE',  ( -6.851666526859749418, 9.086973262793417661, -1.599625672291271394 ) ) ;
#47120=CARTESIAN_POINT ( 'NONE',  ( 4.616554244727909762, 8.463227371007752353, -0.2998622348379786362 ) ) ;
#47135=CARTESIAN_POINT ( 'NONE',  ( 6.200875153403774043, 8.327716660428123419, -1.599625672291283607 ) ) ;
#47138=CARTESIAN_POINT ( 'NONE',  ( -4.736594563127865420, 6.619389305106191834, -1.599625672291271394 ) ) ;
#47142=CARTESIAN_POINT ( 'NONE',  ( -5.872089928050201024, 8.904503111816948646, 1.082531754730550855 ) ) ;
#47152=EDGE_CURVE ( 'NONE', #188684, #50747, #18885, .T. ) ;
#47154=CARTESIAN_POINT ( 'NONE',  ( 4.899292406491845497, 6.809203455697518947, -1.599625672291273171 ) ) ;
#47156=CARTESIAN_POINT ( 'NONE',  ( 8.005163354226054295, 8.304055099544019214, 0.000000000000000000 ) ) ;
#47164=ORIENTED_EDGE ( 'NONE', *, *, #28177, .F. ) ;
#47166=CARTESIAN_POINT ( 'NONE',  ( 5.246079093845007257, 5.085123462432798114, 0.7998128361456352531 ) ) ;
#47172=CARTESIAN_POINT ( 'NONE',  ( 6.333594036239346359, 7.418223126147930557, 1.199719254218453823 ) ) ;
#47185=CARTESIAN_POINT ( 'NONE',  ( -4.990809943606281607, 6.915973915664348937, -1.443375672974066548 ) ) ;
#47187=CARTESIAN_POINT ( 'NONE',  ( 5.478903473698239601, 7.485416367438324059, -1.443375672974078761 ) ) ;
#47193=ORIENTED_EDGE ( 'NONE', *, *, #36937, .T. ) ;
#47198=CARTESIAN_POINT ( 'NONE',  ( -5.790741006812557323, 9.769965251341050205, 0.000000000000000000 ) ) ;
#47199=CARTESIAN_POINT ( 'NONE',  ( 5.840530312436913007, 10.03597880781023299, 0.000000000000000000 ) ) ;
#47202=CARTESIAN_POINT ( 'NONE',  ( 5.844973620822844218, 5.991759777147701804, 0.7216878364870328300 ) ) ;
#47211=DIRECTION ( 'NONE',  ( 0.000000000000000000, -1.000000000000000000, 0.000000000000000000 ) ) ;
#47216=CARTESIAN_POINT ( 'NONE',  ( -5.845336483073759304, 6.639953436172111978, 0.9360796054654503262 ) ) ;
#47218=CARTESIAN_POINT ( 'NONE',  ( 6.086684617892325733, 6.065829907154645539, -0.7998128361456481317 ) ) ;
#47220=CARTESIAN_POINT ( 'NONE',  ( -3.657667580636712934, 7.489305620709952649, -0.7998128361456481317 ) ) ;
#47234=CARTESIAN_POINT ( 'NONE',  ( 6.319508997745523438, 9.426492026461511742, -1.082531754730548412 ) ) ;
#47236=CARTESIAN_POINT ( 'NONE',  ( -7.469616286486262524, 7.679250187180907794, 0.7998128361456341429 ) ) ;
#47237=CARTESIAN_POINT ( 'NONE',  ( 6.204791576909545192, 7.267953590263130259, -1.199719254218452047 ) ) ;
#47244=AXIS2_PLACEMENT_3D ( 'NONE', #197633, #185644, #166207 ) ;
#47247=CARTESIAN_POINT ( 'NONE',  ( -5.960744811863571968, 6.983232364376142698, 1.199719254218452935 ) ) ;
#47264=VERTEX_POINT ( 'NONE', #4749 ) ;
#47274=CARTESIAN_POINT ( 'NONE',  ( 3.770576118376306241, 6.452737000530752276, 1.082531754730549078 ) ) ;
#47281=CARTESIAN_POINT ( 'NONE',  ( 6.170369307550831017, 6.371388078330353366, 0.7216878364870328300 ) ) ;
#47293=CARTESIAN_POINT ( 'NONE',  ( -5.336015975430226099, 8.383046517047350932, -1.199719254218453823 ) ) ;
#47295=CARTESIAN_POINT ( 'NONE',  ( -5.562588163356775972, 9.711712967216715953, 0.7998128361456291469 ) ) ;
#47301=CARTESIAN_POINT ( 'NONE',  ( 3.553238514845298734, 7.337208092372121904, -0.2327671511505452484 ) ) ;
#47302=CARTESIAN_POINT ( 'NONE',  ( 8.039058738260216330, 8.343599714250547805, -0.7998128361456341429 ) ) ;
#47308=CARTESIAN_POINT ( 'NONE',  ( -6.635789839245807897, 6.706452665400368218, 0.7998128361456341429 ) ) ;
#47314=CARTESIAN_POINT ( 'NONE',  ( -4.990809943606281607, 6.915973915664348937, -1.443375672974066548 ) ) ;
#47318=CARTESIAN_POINT ( 'NONE',  ( -5.971440312176176768, 5.931378217152456500, 0.000000000000000000 ) ) ;
#47338=CARTESIAN_POINT ( 'NONE',  ( -5.772739544368596043, 9.956889578397179363, -0.7998128361456362523 ) ) ;
#47340=CARTESIAN_POINT ( 'NONE',  ( -4.793689830883590020, 7.750332681742931662, 1.199719254218452935 ) ) ;
#47358=EDGE_CURVE ( 'NONE', #120674, #128658, #1559, .T. ) ;
#47360=DIRECTION ( 'NONE',  ( -1.000000000000000000, 0.000000000000000000, 0.000000000000000000 ) ) ;
#47366=CARTESIAN_POINT ( 'NONE',  ( -7.767895665986912057, 8.027242796598338614, -0.7998128361456362523 ) ) ;
#47391=CARTESIAN_POINT ( 'NONE',  ( 6.851666526859736983, 9.086973262793417661, -1.599625672291269396 ) ) ;
#47392=CARTESIAN_POINT ( 'NONE',  ( 7.354371980770088690, 7.544798497178720531, 0.000000000000000000 ) ) ;
#47393=DIRECTION ( 'NONE',  ( 0.6507913734559640506, -0.7592566023653003482, 0.000000000000000000 ) ) ;
#47406=CARTESIAN_POINT ( 'NONE',  ( 5.054560120293923653, 7.862967615930308796, 1.113740650586869219 ) ) ;
#47408=CARTESIAN_POINT ( 'NONE',  ( 7.051649292883499953, 7.399548061218447437, -0.7216878364870317197 ) ) ;
#47413=CARTESIAN_POINT ( 'NONE',  ( -4.111865726694519552, 8.019203457777400956, 0.000000000000000000 ) ) ;
#47418=CARTESIAN_POINT ( 'NONE',  ( -6.685579144870156476, 9.853573864773576219, 1.082531754730549967 ) ) ;
#47422=CARTESIAN_POINT ( 'NONE',  ( -4.175548912258498113, 7.500701962048164972, 0.7682608395963886894 ) ) ;
#47428=CARTESIAN_POINT ( 'NONE',  ( -4.014095998097799267, 6.840806543492835345, -1.199719254218450271 ) ) ;
#47438=CARTESIAN_POINT ( 'NONE',  ( 3.576318658954677598, 7.394398545414291313, 0.7998128361456281477 ) ) ;
#47455=CARTESIAN_POINT ( 'NONE',  ( -6.328953403633620134, 6.883256856249502675, 0.7255120703185078401 ) ) ;
#47459=CARTESIAN_POINT ( 'NONE',  ( -7.747558435566414659, 8.003516027774422170, -0.7998128361456362523 ) ) ;
#47462=CARTESIAN_POINT ( 'NONE',  ( 7.693325821111733021, 7.940244644243982464, -0.7998128361456341429 ) ) ;
#47464=CARTESIAN_POINT ( 'NONE',  ( -5.200254360346833415, 7.740598053885397789, 1.191768289972208628 ) ) ;
#47470=CARTESIAN_POINT ( 'NONE',  ( 4.529305835417093640, 7.441884687032027657, -1.199719254218450271 ) ) ;
#47472=EDGE_CURVE ( 'NONE', #206426, #63064, #107738, .T. ) ;
#47475=CARTESIAN_POINT ( 'NONE',  ( 2.993041990875914493, 6.420974562437304911, 0.3677586026352899218 ) ) ;
#47483=CARTESIAN_POINT ( 'NONE',  ( -4.596923820214036560, 8.483565078729160547, 0.2266403168418751335 ) ) ;
#47484=CARTESIAN_POINT ( 'NONE',  ( 5.722950238744198614, 8.730506807626655430, 1.082531754730549967 ) ) ;
#47495=CARTESIAN_POINT ( 'NONE',  ( -6.631346530859867805, 6.909194838857525944, 0.000000000000000000 ) ) ;
#47517=CARTESIAN_POINT ( 'NONE',  ( 5.602074566136501232, 5.729665287594564838, 0.6253354971682704155 ) ) ;
#47527=CARTESIAN_POINT ( 'NONE',  ( 4.016958651398847557, 7.908478536599129249, -0.7998128361456362523 ) ) ;
#47529=CARTESIAN_POINT ( 'NONE',  ( 4.227110032410640095, 8.153655147779589996, 0.7998128361456271485 ) ) ;
#47542=CARTESIAN_POINT ( 'NONE',  ( -6.116136693540540570, 10.14959355252370266, 0.000000000000000000 ) ) ;
#47546=CARTESIAN_POINT ( 'NONE',  ( 4.028181036591620412, 7.713645286083276709, -0.7216878364870338292 ) ) ;
#47561=CARTESIAN_POINT ( 'NONE',  ( -4.651856103264620401, 8.441266197201775512, 0.000000000000000000 ) ) ;
#47563=CARTESIAN_POINT ( 'NONE',  ( -5.045042558060949034, 6.018876084893449274, 1.082531754730549078 ) ) ;
#47570=CARTESIAN_POINT ( 'NONE',  ( -4.357933079043927016, 8.048364350591832306, -0.3271847907353189200 ) ) ;
#47589=CARTESIAN_POINT ( 'NONE',  ( -5.652823702255029836, 5.559658838911111900, -0.7998128361456362523 ) ) ;
#47590=CARTESIAN_POINT ( 'NONE',  ( -5.606283457547605487, 5.690634927916947916, -0.2483668091577979076 ) ) ;
#47599=CARTESIAN_POINT ( 'NONE',  ( -7.611976899429754084, 7.845337568948314022, 0.7998128361456341429 ) ) ;
#47600=CARTESIAN_POINT ( 'NONE',  ( -5.823544721894389653, 7.314923355733134791, 1.295626528688619272 ) ) ;
#47605=CARTESIAN_POINT ( 'NONE',  ( -6.577113915960828727, 9.727031097712693253, -1.082531754730549967 ) ) ;
#47608=CARTESIAN_POINT ( 'NONE',  ( -5.991777542596674166, 5.955104985976372944, 0.000000000000000000 ) ) ;
#47621=CARTESIAN_POINT ( 'NONE',  ( 3.562760505341037831, 7.378580699531681830, -1.734723475976807094E-15 ) ) ;
#47648=CARTESIAN_POINT ( 'NONE',  ( 4.206772801990143584, 8.129928378955675328, 0.7998128361456271485 ) ) ;
#47649=CARTESIAN_POINT ( 'NONE',  ( 5.923986774528332333, 5.876015756563318426, -0.7998128361456481317 ) ) ;
#47651=CARTESIAN_POINT ( 'NONE',  ( 4.848976215542928792, 5.686169002002086970, 1.199719254218452047 ) ) ;
#47662=CARTESIAN_POINT ( 'NONE',  ( 4.609415035364720303, 8.472105597856021575, 0.2450749143364742144 ) ) ;
#47663=CARTESIAN_POINT ( 'NONE',  ( -5.194182247366913252, 7.153241603385088965, 1.443375672974058777 ) ) ;
#47664=CARTESIAN_POINT ( 'NONE',  ( 4.760321332173959696, 4.726332107057286791, 0.000000000000000000 ) ) ;
#47689=CARTESIAN_POINT ( 'NONE',  ( 5.554000203453580475, 6.508696987897830688, -1.199719254218452047 ) ) ;
#47691=CARTESIAN_POINT ( 'NONE',  ( 5.096939404094710468, 4.911127157724081371, 0.000000000000000000 ) ) ;
#47697=ADVANCED_FACE ( 'NONE', ( #105518 ), #135360, .T. ) ;
#47709=DIRECTION ( 'NONE',  ( -1.000000000000000000, 0.000000000000000000, 0.000000000000000000 ) ) ;
#47713=CARTESIAN_POINT ( 'NONE',  ( -5.608757509019071996, 5.629766575911039794, 0.4613631940431175416 ) ) ;
#47714=DIRECTION ( 'NONE',  ( 1.000000000000000000, 0.000000000000000000, 0.000000000000000000 ) ) ;
#47721=CARTESIAN_POINT ( 'NONE',  ( 6.852720297064418986, 6.959538199522133262, 0.7998128361456331437 ) ) ;
#47726=CARTESIAN_POINT ( 'NONE',  ( 5.363132282657546490, 8.414682208812571673, -1.199719254218452047 ) ) ;
#47736=CIRCLE ( 'NONE', #199977, 0.08000000000000012657 ) ;
#47738=CARTESIAN_POINT ( 'NONE',  ( 4.629651883607522223, 8.329987488807731211, -0.3686744245932921937 ) ) ;
#47753=CARTESIAN_POINT ( 'NONE',  ( -6.024748404907106725, 7.078120102419984683, 1.049236913528932780 ) ) ;
#47757=CARTESIAN_POINT ( 'NONE',  ( 3.092668437693027794, 6.622213920701574885, -0.7216878364870338292 ) ) ;
#47762=CARTESIAN_POINT ( 'NONE',  ( -5.764151584465413869, 6.753873599078290546, -1.199719254218453823 ) ) ;
#47764=CARTESIAN_POINT ( 'NONE',  ( 4.715203562502613188, 8.723097599553565118, 0.7998128361456341429 ) ) ;
#47769=CARTESIAN_POINT ( 'NONE',  ( -6.936931872047518155, 8.122117267924091166, 1.199719254218452047 ) ) ;
#47773=DIRECTION ( 'NONE',  ( -0.6507913734559640506, 0.7592566023653005702, 0.000000000000000000 ) ) ;
#47777=CARTESIAN_POINT ( 'NONE',  ( -0.2880152382563990754, 3.298359159248693828, -1.980637607101966235 ) ) ;
#47786=ADVANCED_FACE ( 'NONE', ( #12246 ), #110894, .F. ) ;
#47793=CARTESIAN_POINT ( 'NONE',  ( 6.536439455564168277, 6.798469917679251573, 0.7216878364870328300 ) ) ;
#47809=CARTESIAN_POINT ( 'NONE',  ( -5.492461627311929995, 5.580495784718250363, 0.000000000000000000 ) ) ;
#47811=CARTESIAN_POINT ( 'NONE',  ( 5.580062740476173566, 8.667767742934335828, 1.199719254218451159 ) ) ;
#47855=CARTESIAN_POINT ( 'NONE',  ( 3.851925040058331806, 5.587274861525073355, -1.443375672974066548 ) ) ;
#47866=CARTESIAN_POINT ( 'NONE',  ( -4.624739795592936353, 7.449261290616792763, -1.082531754730549967 ) ) ;
#47872=CARTESIAN_POINT ( 'NONE',  ( -4.664887371553763096, 7.600063145858131364, -1.199719254218453823 ) ) ;
#47880=CARTESIAN_POINT ( 'NONE',  ( -6.317173229324657413, 6.334733287159020954, 0.000000000000000000 ) ) ;
#47881=CARTESIAN_POINT ( 'NONE',  ( -6.343551558972095883, 6.506286488053499184, 2.499999999999999556 ) ) ;
#47883=CARTESIAN_POINT ( 'NONE',  ( 5.420206975164616026, 7.644856803259713729, 1.330009527941821368 ) ) ;
#47888=B_SPLINE_CURVE_WITH_KNOTS ( 'NONE', 3,
 ( #18382, #65002, #166788, #84460, #113852, #67118, #132192, #50903, #130109, #213379, #196102, #181950, #16240, #49835, #33579, #81275 ),
 .UNSPECIFIED., .F., .F.,
 ( 4, 3, 3, 3, 3, 4 ),
 ( 0.000000000000000000, 3.083448363908645134E-05, 6.173412828017592617E-05, 9.147751612222092168E-05, 0.0001189036761826360979, 0.0001300740652511593359 ),
 .UNSPECIFIED. ) ;
#47889=CARTESIAN_POINT ( 'NONE',  ( 6.364626766972446781, 6.390095747748157251, 0.7998128361456352531 ) ) ;
#47898=CARTESIAN_POINT ( 'NONE',  ( -5.113360211009450040, 5.994616996712990975, -1.199719254218453823 ) ) ;
#47904=CARTESIAN_POINT ( 'NONE',  ( -6.123442655227560927, 7.173046514967467147, 1.199719254218452047 ) ) ;
#47908=CARTESIAN_POINT ( 'NONE',  ( 7.010974831598141499, 7.352094523052197239, -0.7216878364870317197 ) ) ;
#47910=CARTESIAN_POINT ( 'NONE',  ( -6.197485614778184271, 9.284131412999601096, 1.082531754730549967 ) ) ;
#47916=CARTESIAN_POINT ( 'NONE',  ( 5.367048706163317640, 7.354919138647580290, -1.599625672291281386 ) ) ;
#47919=CARTESIAN_POINT ( 'NONE',  ( -4.926979960302503514, 4.882856496153904935, 0.5425924526549028570 ) ) ;
#47924=DIRECTION ( 'NONE',  ( -0.7592566023652990159, 0.6507913734559659380, 0.000000000000000000 ) ) ;
#47925=CARTESIAN_POINT ( 'NONE',  ( -5.311662079954674986, 4.760874550186750653, -2.500000000000000444 ) ) ;
#47939=CARTESIAN_POINT ( 'NONE',  ( 3.188928480291412626, 8.980740528189164351, -2.451733079074510435 ) ) ;
#47952=CARTESIAN_POINT ( 'NONE',  ( 6.535912570239620578, 9.782925877658371405, 1.199719254218452047 ) ) ;
#47957=CARTESIAN_POINT ( 'NONE',  ( -5.163927922758308142, 7.774463771048841565, -1.174891720174384480 ) ) ;
#47959=VERTEX_POINT ( 'NONE', #163863 ) ;
#47964=CARTESIAN_POINT ( 'NONE',  ( -4.624739795592943459, 6.488892076315448065, -1.443375672974066548 ) ) ;
#47975=CARTESIAN_POINT ( 'NONE',  ( -5.679940009482361774, 5.591294530676332641, 0.7998128361456281477 ) ) ;
#47986=CARTESIAN_POINT ( 'NONE',  ( 4.420840606507738357, 7.315341919971147355, 1.199719254218451159 ) ) ;
#47989=CARTESIAN_POINT ( 'NONE',  ( 5.953438849732186178, 8.999410187112612647, -1.082531754730548412 ) ) ;
#48001=CARTESIAN_POINT ( 'NONE',  ( -4.936050443827081580, 7.916420063510339666, 1.199719254218452935 ) ) ;
#48002=CARTESIAN_POINT ( 'NONE',  ( 5.578253857379852576, 5.472660686556754861, -0.7998128361456481317 ) ) ;
#48013=CARTESIAN_POINT ( 'NONE',  ( -5.088052786878465739, 9.158088361325352977, 0.000000000000000000 ) ) ;
#48014=CARTESIAN_POINT ( 'NONE',  ( 6.424584688029230328, 8.588711117491191871, 1.599625672291268286 ) ) ;
#48022=CARTESIAN_POINT ( 'NONE',  ( 4.390861645979372341, 6.216034235099629157, -1.599625672291269396 ) ) ;
#48028=( BOUNDED_CURVE ( )  B_SPLINE_CURVE ( 2, ( #61660, #46488, #12887, #10757, #28091 ),
 .UNSPECIFIED., .F., .T. ) 
 B_SPLINE_CURVE_WITH_KNOTS ( ( 3, 2, 3 ),
 ( 0.2236210349743807946, 0.2250000000000000056, 0.2267133053327668735 ),
 .UNSPECIFIED. ) 
 CURVE ( )  GEOMETRIC_REPRESENTATION_ITEM ( )  RATIONAL_B_SPLINE_CURVE ( ( 0.9629979416702594275, 0.9778304460996741776, 1.000000000000000000, 0.9724552731818310036, 0.9562367529269841793 ) ) 
 REPRESENTATION_ITEM ( '' )  );
#48030=CARTESIAN_POINT ( 'NONE',  ( -5.987767821832088444, 7.191367801968548079, 1.216456708157914512 ) ) ;
#48034=CARTESIAN_POINT ( 'NONE',  ( 2.896029359114099755, 6.600727695600251188, 0.2594116555042840777 ) ) ;
#48039=CARTESIAN_POINT ( 'NONE',  ( -7.930593509350902792, 8.217056947189661287, -0.7998128361456362523 ) ) ;
#48089=CARTESIAN_POINT ( 'NONE',  ( 5.063044020060520900, 4.871582543017558109, 0.7998128361456352531 ) ) ;
#48090=CARTESIAN_POINT ( 'NONE',  ( -4.258669648468323743, 6.061810238003387141, 1.443375672974065660 ) ) ;
#48117=ORIENTED_EDGE ( 'NONE', *, *, #125035, .T. ) ;
#48118=CARTESIAN_POINT ( 'NONE',  ( -4.847922445338252118, 7.813604065273374921, -1.199719254218453823 ) ) ;
#48120=CARTESIAN_POINT ( 'NONE',  ( 6.821160681006788629, 8.091013894996997635, 1.082531754730549967 ) ) ;
#48125=CARTESIAN_POINT ( 'NONE',  ( -5.607179047703544583, 8.699403434699558346, 1.199719254218454489 ) ) ;
#48133=CARTESIAN_POINT ( 'NONE',  ( -4.586401103172829785, 8.572828063668767484, 0.7998128361456281477 ) ) ;
#48146=CARTESIAN_POINT ( 'NONE',  ( -5.367048706163331850, 7.354919138647580290, -1.599625672291271394 ) ) ;
#48149=CARTESIAN_POINT ( 'NONE',  ( -7.756673280794142755, 8.222076047114187602, -0.7216878364870338292 ) ) ;
#48151=CARTESIAN_POINT ( 'NONE',  ( -5.085717018457573957, 8.947437264926888290, 0.7216878364870267237 ) ) ;
#48152=CARTESIAN_POINT ( 'NONE',  ( 7.700104897918568447, 7.948153567185284096, 0.000000000000000000 ) ) ;
#48154=CARTESIAN_POINT ( 'NONE',  ( -6.933015448541747006, 9.181880338089085214, 1.599625672291269396 ) ) ;
#48173=CARTESIAN_POINT ( 'NONE',  ( -1.840093022230759878, 2.503055443996555329, -2.494806138668435036 ) ) ;
#48192=CARTESIAN_POINT ( 'NONE',  ( 6.348694402744908594, 6.841026321354189754, -0.6301123915167846645 ) ) ;
#48208=CARTESIAN_POINT ( 'NONE',  ( -3.806807270387036368, 7.663301925418665839, 0.000000000000000000 ) ) ;
#48212=CARTESIAN_POINT ( 'NONE',  ( -7.065207446052809814, 9.336104335185325453, -1.443375672974066548 ) ) ;
#48222=CARTESIAN_POINT ( 'NONE',  ( 4.115782150200256950, 6.959440387612411349, 1.199719254218452047 ) ) ;
#48224=CARTESIAN_POINT ( 'NONE',  ( 7.126746022638799971, 8.343567110280638133, 1.199719254218452047 ) ) ;
#48236=CARTESIAN_POINT ( 'NONE',  ( 6.363572996767764778, 8.517530811019446091, -1.599625672291283607 ) ) ;
#48242=DIRECTION ( 'NONE',  ( -1.000000000000000000, 0.000000000000000000, 0.000000000000000000 ) ) ;
#48249=CARTESIAN_POINT ( 'NONE',  ( -5.885648082108231982, 7.959951743916638733, 1.443375672974058777 ) ) ;
#48250=CARTESIAN_POINT ( 'NONE',  ( 6.238160076063542725, 6.450477308261824305, -0.7216878364870458196 ) ) ;
#48260=CYLINDRICAL_SURFACE ( 'NONE', #99114, 1.250000000000000000 ) ;
#48261=CARTESIAN_POINT ( 'NONE',  ( -5.587368702607575344, 8.572328348800551723, 1.082531754730550855 ) ) ;
#48262=CARTESIAN_POINT ( 'NONE',  ( 6.230854113932139171, 9.427024345299638952, 1.199719254218452047 ) ) ;
#48266=CARTESIAN_POINT ( 'NONE',  ( 5.438229012412886476, 7.437962829272074750, -1.443375672974078761 ) ) ;
#48284=EDGE_CURVE ( 'NONE', #134461, #13120, #99850, .T. ) ;
#48285=CARTESIAN_POINT ( 'NONE',  ( -5.517242166118370150, 5.401480380085008193, 0.7998128361456281477 ) ) ;
#48297=CARTESIAN_POINT ( 'NONE',  ( 4.472210567661338843, 6.310941310395290493, 1.599625672291261402 ) ) ;
#48299=CARTESIAN_POINT ( 'NONE',  ( -7.632314129850253259, 7.869064337772231355, 0.7998128361456341429 ) ) ;
#48300=CARTESIAN_POINT ( 'NONE',  ( 5.855142236255289845, 7.924361590421551860, -1.599625672291281386 ) ) ;
#48308=CARTESIAN_POINT ( 'NONE',  ( -4.613517410400161722, 8.604463755433990002, -0.7998128361456362523 ) ) ;
#48337=CARTESIAN_POINT ( 'NONE',  ( 4.340018570150304456, 6.156717313299049366, -1.443375672974068769 ) ) ;
#48343=CARTESIAN_POINT ( 'NONE',  ( 4.814553946184248368, 7.670711132973337065, -1.082531754730548412 ) ) ;
#48355=CARTESIAN_POINT ( 'NONE',  ( -7.130662446144611977, 7.283804040115648526, 0.000000000000000000 ) ) ;
#48357=CARTESIAN_POINT ( 'NONE',  ( -6.749980374757255319, 8.968339418673846097, 1.599625672291269396 ) ) ;
#48364=CARTESIAN_POINT ( 'NONE',  ( 6.068156270568149324, 9.237210194708310951, 1.199719254218452047 ) ) ;
#48369=CARTESIAN_POINT ( 'NONE',  ( 4.936581118797800372, 8.100871430792054184, -1.059671831818540966 ) ) ;
#48370=CARTESIAN_POINT ( 'NONE',  ( -5.237192476628793614, 9.332084666034067055, 0.7998128361456291469 ) ) ;
#48377=CARTESIAN_POINT ( 'NONE',  ( -5.722950238744243023, 7.770137593325314285, 1.443375672974058777 ) ) ;
#48380=CARTESIAN_POINT ( 'NONE',  ( -6.947627372360122955, 7.070263120700404968, 0.000000000000000000 ) ) ;
#48403=CARTESIAN_POINT ( 'NONE',  ( -8.120407659942227241, 8.438506789546210030, 0.7998128361456341429 ) ) ;
#48404=CARTESIAN_POINT ( 'NONE',  ( 2.898410978271408922, 6.603506251283770112, -0.7998128361456362523 ) ) ;
#48405=EDGE_CURVE ( 'NONE', #24930, #51151, #88673, .T. ) ;
#48406=CARTESIAN_POINT ( 'NONE',  ( -4.796552484184649856, 8.818004674849227342, -0.7998128361456362523 ) ) ;
#48420=CARTESIAN_POINT ( 'NONE',  ( -5.524540912749783317, 5.975067110676214988, -0.9400251737342411040 ) ) ;
#48428=CARTESIAN_POINT ( 'NONE',  ( -7.228432174741334038, 8.462200954400218578, -1.199719254218452047 ) ) ;
#48455=CARTESIAN_POINT ( 'NONE',  ( 5.598591087800349086, 5.496387455380669529, -0.7998128361456481317 ) ) ;
#48469=CARTESIAN_POINT ( 'NONE',  ( 7.241463443474815520, 8.581367117876336437, -1.082531754730548412 ) ) ;
#48474=CARTESIAN_POINT ( 'NONE',  ( -6.459533842268148973, 6.500820668926428958, 0.000000000000000000 ) ) ;
#48479=CARTESIAN_POINT ( 'NONE',  ( -7.553300976144794454, 7.984808358356614733, -0.7216878364870338292 ) ) ;
#48482=CARTESIAN_POINT ( 'NONE',  ( -4.995253251992230581, 4.792493313604505367, 0.000000000000000000 ) ) ;
#48487=CARTESIAN_POINT ( 'NONE',  ( -3.610214042988883598, 7.433943160120816351, 0.7998128361456352531 ) ) ;
#48496=CARTESIAN_POINT ( 'NONE',  ( 4.224247379109608680, 7.085983154673295203, -1.199719254218452047 ) ) ;
#48516=CARTESIAN_POINT ( 'NONE',  ( -7.937372586157736443, 8.224965870130965584, 0.7998128361456341429 ) ) ;
#48519=CARTESIAN_POINT ( 'NONE',  ( 7.289443866002793371, 8.533381260871966134, 1.199719254218452047 ) ) ;
#48521=( BOUNDED_CURVE ( )  B_SPLINE_CURVE ( 2, ( #111441, #31200, #13850, #193678, #61553 ),
 .UNSPECIFIED., .F., .T. ) 
 B_SPLINE_CURVE_WITH_KNOTS ( ( 3, 2, 3 ),
 ( 0.2461390157910678111, 0.2500000000000000000, 0.2545216234105981967 ),
 .UNSPECIFIED. ) 
 CURVE ( )  GEOMETRIC_REPRESENTATION_ITEM ( )  RATIONAL_B_SPLINE_CURVE ( ( 0.9333732439868740460, 0.9379271439536381871, 1.000000000000000000, 0.9273060795191534478, 0.9334988468753528945 ) ) 
 REPRESENTATION_ITEM ( '' )  );
#48527=CARTESIAN_POINT ( 'NONE',  ( 4.505052181490820651, 8.477920988373101707, -0.7998128361456381397 ) ) ;
#48535=CARTESIAN_POINT ( 'NONE',  ( 4.340018570150304456, 6.156717313299049366, -1.443375672974068769 ) ) ;
#48538=CARTESIAN_POINT ( 'NONE',  ( 7.526184669361807522, 7.953172667109813077, 0.000000000000000000 ) ) ;
#48539=ORIENTED_EDGE ( 'NONE', *, *, #111774, .F. ) ;
#48542=ORIENTED_EDGE ( 'NONE', *, *, #116473, .T. ) ;
#48550=CARTESIAN_POINT ( 'NONE',  ( -5.302647476720585118, 9.200522799567075083, 0.000000000000000000 ) ) ;
#48585=CARTESIAN_POINT ( 'NONE',  ( 5.692444392891300886, 7.734547439830227411, -1.599625672291281386 ) ) ;
#48587=CARTESIAN_POINT ( 'NONE',  ( 6.900173834712277632, 7.014900660111269559, -0.7998128361456341429 ) ) ;
#48598=CARTESIAN_POINT ( 'NONE',  ( -3.797165540279144214, 6.587721009371067638, 1.199719254218452935 ) ) ;
#48601=CARTESIAN_POINT ( 'NONE',  ( 4.950135482320912494, 6.868520377498098739, -1.443375672974068769 ) ) ;
#48615=CARTESIAN_POINT ( 'NONE',  ( -5.912764389335557702, 8.951956649983198844, 1.082531754730550855 ) ) ;
#48617=CARTESIAN_POINT ( 'NONE',  ( -4.001064729808656573, 7.682009594836471500, 1.214306433183764966E-14 ) ) ;
#48618=CARTESIAN_POINT ( 'NONE',  ( 4.318982125183886467, 7.080239525325785266, 1.240331472013181058 ) ) ;
#48642=CARTESIAN_POINT ( 'NONE',  ( -5.666381855868691808, 5.575476684793721383, 0.000000000000000000 ) ) ;
#48644=EDGE_CURVE ( 'NONE', #80951, #80427, #148123, .T. ) ;
#48652=CARTESIAN_POINT ( 'NONE',  ( -5.576146316970437944, 9.727530813099326323, 0.000000000000000000 ) ) ;
#48653=CARTESIAN_POINT ( 'NONE',  ( -5.492869780704572769, 7.580512000422499952, -1.348893862496753249 ) ) ;
#48657=DIRECTION ( 'NONE',  ( 1.000000000000000000, 0.000000000000000000, 0.000000000000000000 ) ) ;
#48671=CARTESIAN_POINT ( 'NONE',  ( 4.715203562502613188, 8.723097599553565118, 0.7998128361456341429 ) ) ;
#48674=B_SPLINE_CURVE_WITH_KNOTS ( 'NONE', 3,
 ( #76508, #42980, #138329, #8307, #60261, #157783, #171884, #57070, #172968, #74391, #88514, #142619, #204345, #25620, #22405, #89588, #9381, #191312, #140492, #41910, #206503, #158839, #75452 ),
 .UNSPECIFIED., .F., .F.,
 ( 4, 2, 2, 2, 2, 2, 2, 2, 2, 1, 2, 4 ),
 ( 0.2533959729413839401, 0.2675222111384283896, 0.2816484493354728391, 0.2957746875325172331, 0.3099009257295616826, 0.3240271639266061321, 0.3381534021236505816, 0.3452165212221727786, 0.3469823009968033278, 0.3487480807714339326, 0.3522796403206950311, 0.3664058785177394806 ),
 .UNSPECIFIED. ) ;
#48677=CARTESIAN_POINT ( 'NONE',  ( 0.3399812269560758549, 3.243416237969932503, -2.042960595231173571 ) ) ;
#48686=EDGE_CURVE ( 'NONE', #79641, #111999, #7610, .T. ) ;
#48697=CARTESIAN_POINT ( 'NONE',  ( 7.018280793729500644, 8.217024343219755167, -1.199719254218452047 ) ) ;
#48698=CARTESIAN_POINT ( 'NONE',  ( 6.873057527484919937, 6.983264968346048818, 0.7998128361456352531 ) ) ;
#48700=CARTESIAN_POINT ( 'NONE',  ( 3.379725431556547477, 7.165039780116438273, -1.734723475976807094E-15 ) ) ;
#48711=CARTESIAN_POINT ( 'NONE',  ( 5.420206975164616026, 7.644856803259713729, 1.330009527941821368 ) ) ;
#48713=CARTESIAN_POINT ( 'NONE',  ( -4.624739795592931912, 8.409630504918133909, -0.7216878364870338292 ) ) ;
#48714=CARTESIAN_POINT ( 'NONE',  ( 4.068855497876973537, 7.761098824249525130, -0.7216878364870338292 ) ) ;
#48739=CARTESIAN_POINT ( 'NONE',  ( 5.876533236880477240, 5.820653295974182129, 0.7998128361456352531 ) ) ;
#48741=CARTESIAN_POINT ( 'NONE',  ( 4.411198876399872404, 6.239761003923544713, -1.599625672291273171 ) ) ;
#48749=DIRECTION ( 'NONE',  ( 0.000000000000000000, 1.000000000000000000, 0.000000000000000000 ) ) ;
#48760=CARTESIAN_POINT ( 'NONE',  ( -7.767895665986912057, 8.027242796598338614, -0.7998128361456362523 ) ) ;
#48769=CARTESIAN_POINT ( 'NONE',  ( 5.448397627845284141, 7.449826213943242514, 1.599625672291268286 ) ) ;
#48772=AXIS2_PLACEMENT_3D ( 'NONE', #155761, #107063, #90775 ) ;
#48774=CARTESIAN_POINT ( 'NONE',  ( 4.362691568547328202, 8.311833606605697256, -0.7998128361456381397 ) ) ;
#48785=CARTESIAN_POINT ( 'NONE',  ( 4.771497086726927073, 8.161215468402982509, 0.7801120568680236511 ) ) ;
#48792=CARTESIAN_POINT ( 'NONE',  ( 5.560252395380215873, 6.619954228432645138, 1.082531754730549078 ) ) ;
#48794=LINE ( 'NONE', #114911, #174693 ) ;
#48806=CARTESIAN_POINT ( 'NONE',  ( -5.420227550413282636, 9.545625585449309725, 0.7998128361456291469 ) ) ;
#48808=CARTESIAN_POINT ( 'NONE',  ( 5.956828388357757298, 8.042995434541133193, 1.599625672291269396 ) ) ;
#48817=DIRECTION ( 'NONE',  ( 1.000000000000000000, 0.000000000000000000, 0.000000000000000000 ) ) ;
#48820=CARTESIAN_POINT ( 'NONE',  ( -0.1054627972275563597, 3.385846599571565640, -2.076146368081344118 ) ) ;
#48838=CARTESIAN_POINT ( 'NONE',  ( 6.753369913382843315, 8.011924666102361314, -1.082531754730548412 ) ) ;
#48853=CARTESIAN_POINT ( 'NONE',  ( -3.987506576194992824, 7.666191748953863794, 0.7216878364870338292 ) ) ;
#48855=CARTESIAN_POINT ( 'NONE',  ( 5.845500506147374153, 6.848780674373954547, 1.199719254218453823 ) ) ;
#48860=CARTESIAN_POINT ( 'NONE',  ( -7.075376061485238566, 9.347967719856493218, 1.599625672291269396 ) ) ;
#48870=CARTESIAN_POINT ( 'NONE',  ( -2.353140975214501829, 2.704741401632028808, 2.456000212125921678 ) ) ;
#48903=CARTESIAN_POINT ( 'NONE',  ( 5.090160327287878594, 4.903218234782778850, -0.7998128361456481317 ) ) ;
#48909=CARTESIAN_POINT ( 'NONE',  ( -3.621436428181653788, 7.239109909604962922, 0.7216878364870338292 ) ) ;
#48915=CARTESIAN_POINT ( 'NONE',  ( -5.088052786878465739, 9.158088361325352977, 0.000000000000000000 ) ) ;
#48925=CARTESIAN_POINT ( 'NONE',  ( -6.493429226302317225, 6.540365283632955773, 0.7998128361456341429 ) ) ;
#48928=CARTESIAN_POINT ( 'NONE',  ( 5.950060389077887812, 7.221515259811701171, 1.225279837341096689 ) ) ;
#48934=CARTESIAN_POINT ( 'NONE',  ( 5.481239241674765950, 9.616805891921051952, -0.7998128361456481317 ) ) ;
#48942=CARTESIAN_POINT ( 'NONE',  ( -4.329849954717889915, 6.144853928627882489, 1.599625672291270506 ) ) ;
#48946=CARTESIAN_POINT ( 'NONE',  ( -6.231907884136888676, 7.299589282028351001, -1.199719254218453823 ) ) ;
#48947=B_SPLINE_CURVE_WITH_KNOTS ( 'NONE', 3,
 ( #17397, #149563, #68281, #19544, #151709, #69345, #20603, #105096, #157043, #74712 ),
 .UNSPECIFIED., .F., .F.,
 ( 4, 3, 3, 4 ),
 ( 7.433113292862203613E-18, 0.0001748236543164608252, 0.0003403917518363700173, 0.0005070588120444130585 ),
 .UNSPECIFIED. ) ;
#48952=CARTESIAN_POINT ( 'NONE',  ( 6.983858524370782028, 8.280828045588322084, 1.082531754730549967 ) ) ;
#48954=CARTESIAN_POINT ( 'NONE',  ( -7.566859129758459979, 8.000626204239226880, 0.000000000000000000 ) ) ;
#48960=CARTESIAN_POINT ( 'NONE',  ( 6.150558962454855561, 7.204682206732687000, 1.199719254218452047 ) ) ;
#48963=CARTESIAN_POINT ( 'NONE',  ( -4.944262139963866431, 4.884656545040805042, 0.5135224484073761531 ) ) ;
#48998=CARTESIAN_POINT ( 'NONE',  ( 6.994027139803230320, 9.253060644560830994, -1.599625672291267398 ) ) ;
#49003=CARTESIAN_POINT ( 'NONE',  ( -5.670379370357061077, 7.341873695786736320, -1.227147999111227294 ) ) ;
#49020=CARTESIAN_POINT ( 'NONE',  ( -2.993318053567081360, 6.714231172462041819, 0.000000000000000000 ) ) ;
#49030=ORIENTED_EDGE ( 'NONE', *, *, #84368, .F. ) ;
#49033=CARTESIAN_POINT ( 'NONE',  ( 6.554440917563797875, 6.611545590104705994, -0.7998128361456481317 ) ) ;
#49036=CARTESIAN_POINT ( 'NONE',  ( 6.997416677984476863, 7.336276677169590421, 0.000000000000000000 ) ) ;
#49050=CARTESIAN_POINT ( 'NONE',  ( -6.147696309153835692, 6.137010213626392208, 0.7998128361456281477 ) ) ;
#49051=CARTESIAN_POINT ( 'NONE',  ( 5.174371902270911150, 6.065797303184739420, 1.199719254218452047 ) ) ;
#49061=CARTESIAN_POINT ( 'NONE',  ( -4.248501033035892327, 6.049946853332221153, -1.599625672291271394 ) ) ;
#49062=CARTESIAN_POINT ( 'NONE',  ( 7.042534447655770080, 7.180988041878682004, -0.7998128361456341429 ) ) ;
#49069=CARTESIAN_POINT ( 'NONE',  ( 4.095444919779759552, 6.935713618788495793, 1.199719254218451159 ) ) ;
#49076=CARTESIAN_POINT ( 'NONE',  ( -6.486107617800834113, 6.842887492708185526, 0.6303255377333163434 ) ) ;
#49080=CIRCLE ( 'NONE', #76721, 0.7500000000000006661 ) ;
#49086=CARTESIAN_POINT ( 'NONE',  ( -6.583366107887490770, 9.838288338247510367, 1.199719254218452935 ) ) ;
#49098=CARTESIAN_POINT ( 'NONE',  ( -6.343417644169881520, 6.506394916555812813, 2.500000000000000444 ) ) ;
#49099=CARTESIAN_POINT ( 'NONE',  ( -4.517335436343488553, 8.499999999999996447, -0.7750000000000013545 ) ) ;
#49116=B_SPLINE_CURVE_WITH_KNOTS ( 'NONE', 3,
 ( #25438, #43861, #61150, #171691, #109976, #187932, #12383, #65122, #131279, #199386 ),
 .UNSPECIFIED., .F., .F.,
 ( 4, 3, 3, 4 ),
 ( 0.000000000000000000, 4.084796759526023937E-05, 5.706657677113307714E-05, 5.895014842486881381E-05 ),
 .UNSPECIFIED. ) ;
#49119=CARTESIAN_POINT ( 'NONE',  ( 4.199993725183333915, 8.122019456014369254, -0.7998128361456361413 ) ) ;
#49138=CARTESIAN_POINT ( 'NONE',  ( 4.146814880933355596, 5.931313009212638931, 1.599625672291261402 ) ) ;
#49166=CARTESIAN_POINT ( 'NONE',  ( -5.764151584465413869, 6.753873599078290546, -1.199719254218453823 ) ) ;
#49168=CARTESIAN_POINT ( 'NONE',  ( 7.499068361690118145, 7.921536974826172361, -0.7216878364870317197 ) ) ;
#49174=CARTESIAN_POINT ( 'NONE',  ( -6.363572996767778100, 8.517530811019446091, -1.599625672291271394 ) ) ;
#49182=CARTESIAN_POINT ( 'NONE',  ( -5.101610940492132151, 9.173906207207963348, -0.7998128361456362523 ) ) ;
#49193=CARTESIAN_POINT ( 'NONE',  ( -4.274563570058511175, 8.209017608368725405, 0.000000000000000000 ) ) ;
#49197=CARTESIAN_POINT ( 'NONE',  ( -6.563555762791521531, 9.711213252348503744, 1.082531754730549967 ) ) ;
#49199=CARTESIAN_POINT ( 'NONE',  ( -5.275531169048895741, 9.168887107283438809, -0.7216878364870338292 ) ) ;
#49200=CARTESIAN_POINT ( 'NONE',  ( 8.039058738260216330, 8.343599714250547805, -0.7998128361456341429 ) ) ;
#49201=CARTESIAN_POINT ( 'NONE',  ( -2.997761361953021009, 6.511488999004883205, -0.7216878364870458196 ) ) ;
#49222=CARTESIAN_POINT ( 'NONE',  ( 6.562153376633583335, 6.794832157118596783, -0.3727171428496069971 ) ) ;
#49227=( BOUNDED_CURVE ( )  B_SPLINE_CURVE ( 2, ( #16575, #169252, #50174, #68523, #184421, #99987, #98930, #53365, #168187, #32855, #66382, #102118, #19786, #182285, #116294, #82658, #51240, #199597, #183363, #85868, #119499, #34967, #200655, #131472, #101039, #166053, #37111, #33911, #164984, #52304, #197474, #167129, #118434, #310, #17638, #185485, #103189, #49119, #150886, #151945, #20838, #83724, #18714, #148742, #84798, #86937, #57641, #105345, #4580, #136764, #172465, #206006, #41413, #26192, #39252, #204927, #122737, #188700, #187625, #157287, #207073 ),
 .UNSPECIFIED., .F., .T. ) 
 B_SPLINE_CURVE_WITH_KNOTS ( ( 3, 2, 2, 2, 2, 2, 2, 2, 2, 2, 2, 2, 2, 2, 2, 2, 2, 2, 2, 2, 2, 2, 2, 2, 2, 2, 2, 2, 2, 2, 3 ),
 ( 0.2691230753395070785, 0.2750000000000000222, 0.2833333333333333259, 0.2916666666666666852, 0.2999999999999999889, 0.3083333333333333481, 0.3166666666666666519, 0.3250000000000000111, 0.3333333333333333148, 0.3416666666666666741, 0.3499999999999999778, 0.3583333333333333370, 0.3666666666666666408, 0.3750000000000000000, 0.3833333333333333592, 0.3916666666666666630, 0.4000000000000000222, 0.4083333333333333259, 0.4166666666666666852, 0.4249999999999999889, 0.4333333333333333481, 0.4416666666666666519, 0.4500000000000000111, 0.4583333333333333148, 0.4666666666666666741, 0.4749999999999999778, 0.4833333333333333370, 0.4916666666666666408, 0.5000000000000000000, 0.5083333333333333037, 0.5097603473456372436 ),
 .UNSPECIFIED. ) 
 CURVE ( )  GEOMETRIC_REPRESENTATION_ITEM ( )  RATIONAL_B_SPLINE_CURVE ( ( 0.9442986539893905018, 0.9055169669945422051, 1.000000000000000000, 0.8660254037844387076, 1.000000000000000000, 0.8660254037844387076, 1.000000000000000000, 0.8660254037844387076, 1.000000000000000000, 0.8660254037844387076, 1.000000000000000000, 0.8660254037844387076, 1.000000000000000000, 0.8660254037844387076, 1.000000000000000000, 0.8660254037844387076, 1.000000000000000000, 0.8660254037844387076, 1.000000000000000000, 0.8660254037844387076, 1.000000000000000000, 0.8660254037844387076, 1.000000000000000000, 0.8660254037844387076, 1.000000000000000000, 0.8660254037844387076, 1.000000000000000000, 0.8660254037844387076, 1.000000000000000000, 0.8660254037844387076, 1.000000000000000000, 0.8660254037844387076, 1.000000000000000000, 0.8660254037844387076, 1.000000000000000000, 0.8660254037844387076, 1.000000000000000000, 0.8660254037844387076, 1.000000000000000000, 0.8660254037844387076, 1.000000000000000000, 0.8660254037844387076, 1.000000000000000000, 0.8660254037844387076, 1.000000000000000000, 0.8660254037844387076, 1.000000000000000000, 0.8660254037844387076, 1.000000000000000000, 0.8660254037844387076, 1.000000000000000000, 0.8660254037844387076, 1.000000000000000000, 0.8660254037844387076, 1.000000000000000000, 0.8660254037844387076, 1.000000000000000000, 0.8660254037844387076, 1.000000000000000000, 0.9770579648689160512, 0.9619731950825103350 ) ) 
 REPRESENTATION_ITEM ( '' )  );
#49241=CARTESIAN_POINT ( 'NONE',  ( 6.381672224870991172, 6.819330018336470012, -0.5576268912585117254 ) ) ;
#49254=CARTESIAN_POINT ( 'NONE',  ( 7.849244587668864348, 8.122149871893999062, 0.7998128361456291469 ) ) ;
#49257=CARTESIAN_POINT ( 'NONE',  ( -3.820365424000704557, 7.679119771301277098, -0.7998128361456481317 ) ) ;
#49271=CARTESIAN_POINT ( 'NONE',  ( 3.736153849017632922, 6.516540702899320081, -1.199719254218453823 ) ) ;
#49274=CARTESIAN_POINT ( 'NONE',  ( 6.692885107001518286, 7.837396042037102717, -1.199719254218452047 ) ) ;
#49282=CARTESIAN_POINT ( 'NONE',  ( -5.573810548549546162, 9.516879716700865188, 0.7216878364870267237 ) ) ;
#49290=CARTESIAN_POINT ( 'NONE',  ( 6.851666526859736983, 9.086973262793417661, -1.599625672291269396 ) ) ;
#49296=CIRCLE ( 'NONE', #201385, 2.000000000000000000 ) ;
#49297=CARTESIAN_POINT ( 'NONE',  ( 1.845237968648437032, 8.937006183319889274, 0.7750000000000004663 ) ) ;
#49303=CARTESIAN_POINT ( 'NONE',  ( -6.129694847154220305, 8.244672969803623630, -1.443375672974066548 ) ) ;
#49304=CARTESIAN_POINT ( 'NONE',  ( 4.407809338218622308, 8.156544971314787063, 0.000000000000000000 ) ) ;
#49308=VERTEX_POINT ( 'NONE', #149769 ) ;
#49312=CARTESIAN_POINT ( 'NONE',  ( -3.447516199624892419, 7.244129009529488350, 0.7998128361456352531 ) ) ;
#49313=CARTESIAN_POINT ( 'NONE',  ( -5.641601317062239218, 8.635599732330991429, -1.082531754730549967 ) ) ;
#49314=CARTESIAN_POINT ( 'NONE',  ( 1.865311119267500040, 2.483290406177208975, -2.476007760152826531 ) ) ;
#49318=CARTESIAN_POINT ( 'NONE',  ( 4.868786560638889149, 6.773613302202437403, 1.443375672974065660 ) ) ;
#49329=DIRECTION ( 'NONE',  ( 0.000000000000000000, 0.000000000000000000, -1.000000000000000000 ) ) ;
#49337=CARTESIAN_POINT ( 'NONE',  ( -5.327428015527048366, 5.180030537728460338, -0.7998128361456362523 ) ) ;
#49347=CARTESIAN_POINT ( 'NONE',  ( 3.444653546323793947, 6.176457016423196222, 1.199719254218451159 ) ) ;
#49350=CARTESIAN_POINT ( 'NONE',  ( 4.355912491740495440, 8.303924683664389406, 0.000000000000000000 ) ) ;
#49357=CARTESIAN_POINT ( 'NONE',  ( -4.827585214917754719, 7.789877296449459365, -1.199719254218453823 ) ) ;
#49382=CARTESIAN_POINT ( 'NONE',  ( 3.580761967785000888, 7.191656372475549119, -0.7216878364870338292 ) ) ;
#49389=CARTESIAN_POINT ( 'NONE',  ( 4.868786560638885597, 7.733982516503781213, 1.082531754730548412 ) ) ;
#49400=CARTESIAN_POINT ( 'NONE',  ( -5.121948170912633991, 9.197632976031879792, -0.7998128361456362523 ) ) ;
#49402=CARTESIAN_POINT ( 'NONE',  ( -5.576146316970437944, 9.727530813099326323, 0.000000000000000000 ) ) ;
#49408=CARTESIAN_POINT ( 'NONE',  ( 7.526711554241970248, 8.810193563817646734, -1.199719254218452047 ) ) ;
#49414=CARTESIAN_POINT ( 'NONE',  ( -5.608744109800250399, 5.623033084029449569, 0.4489015171048596486 ) ) ;
#49415=CARTESIAN_POINT ( 'NONE',  ( -5.901542003698421190, 10.10715911428198055, 0.000000000000000000 ) ) ;
#49421=CARTESIAN_POINT ( 'NONE',  ( -4.814553946628611136, 8.631080347793099961, 0.000000000000000000 ) ) ;
#49424=CARTESIAN_POINT ( 'NONE',  ( -5.088052786878465739, 9.158088361325352977, 0.000000000000000000 ) ) ;
#49431=CARTESIAN_POINT ( 'NONE',  ( 4.570507181582611267, 8.346359121906111511, 0.000000000000000000 ) ) ;
#49444=CARTESIAN_POINT ( 'NONE',  ( -4.882344714696960075, 5.829061934302122161, 1.082531754730549078 ) ) ;
#49446=CARTESIAN_POINT ( 'NONE',  ( -4.977251789548269301, 4.979417640660637190, 0.7216878364870257245 ) ) ;
#49447=CARTESIAN_POINT ( 'NONE',  ( 4.329849954717849947, 6.144853928627882489, 1.599625672291262513 ) ) ;
#49448=CARTESIAN_POINT ( 'NONE',  ( -4.444040490229335560, 8.406740681901359480, 0.7998128361456352531 ) ) ;
#49464=CARTESIAN_POINT ( 'NONE',  ( -5.542386507442576438, 5.938373294205037567, -0.8979104349328557166 ) ) ;
#49496=CARTESIAN_POINT ( 'NONE',  ( 2.925527285498711549, 6.635141943048991742, 0.7998128361456281477 ) ) ;
#49509=CARTESIAN_POINT ( 'NONE',  ( 4.675188888464441028, 8.274035074156913083, -0.5495550137140058355 ) ) ;
#49511=CARTESIAN_POINT ( 'NONE',  ( 4.228163802615382494, 6.026220084508304708, -1.599625672291269396 ) ) ;
#49516=CARTESIAN_POINT ( 'NONE',  ( -6.934069218746458318, 7.054445274817795486, -0.7998128361456362523 ) ) ;
#49521=CARTESIAN_POINT ( 'NONE',  ( -5.926322542504860458, 9.928143709648733051, -0.7216878364870338292 ) ) ;
#49525=CARTESIAN_POINT ( 'NONE',  ( -5.821562047661695161, 5.964446275831489785, 0.1636455158913159846 ) ) ;
#49528=CARTESIAN_POINT ( 'NONE',  ( 5.343321937561575474, 8.287607122913563273, -1.082531754730548412 ) ) ;
#49531=CARTESIAN_POINT ( 'NONE',  ( -4.664887371553763096, 7.600063145858131364, -1.199719254218453823 ) ) ;
#49540=CARTESIAN_POINT ( 'NONE',  ( 4.278479993564246797, 7.149254538203735798, 1.199719254218452047 ) ) ;
#49550=VERTEX_POINT ( 'NONE', #19743 ) ;
#49558=ADVANCED_FACE ( 'NONE', ( #85824 ), #56026, .T. ) ;
#49565=DIRECTION ( 'NONE',  ( 0.000000000000000000, 0.000000000000000000, 1.000000000000000000 ) ) ;
#49566=AXIS2_PLACEMENT_3D ( 'NONE', #199096, #116868, #26224 ) ;
#49573=CARTESIAN_POINT ( 'NONE',  ( 7.517069824134078537, 7.734612647770044092, 0.000000000000000000 ) ) ;
#49581=CARTESIAN_POINT ( 'NONE',  ( 4.584065335196260804, 6.441438539186039591, 1.443375672974065660 ) ) ;
#49585=CARTESIAN_POINT ( 'NONE',  ( 6.129694847154206983, 8.244672969803623630, -1.443375672974078761 ) ) ;
#49597=CARTESIAN_POINT ( 'NONE',  ( -5.139949633356594383, 9.010708648975750634, 0.000000000000000000 ) ) ;
#49620=DIRECTION ( 'NONE',  ( 0.6507913734559641616, -0.7592566023653004592, 0.000000000000000000 ) ) ;
#49630=CARTESIAN_POINT ( 'NONE',  ( 5.773793314573267388, 7.829454515125894964, 1.599625672291268286 ) ) ;
#49633=CARTESIAN_POINT ( 'NONE',  ( 5.363132282657546490, 8.414682208812571673, -1.199719254218452047 ) ) ;
#49647=CARTESIAN_POINT ( 'NONE',  ( -3.471769853551161411, 6.208092708188416076, 1.199719254218452935 ) ) ;
#49650=CARTESIAN_POINT ( 'NONE',  ( 4.055297343818923039, 7.745280977848496562, 0.7216878364870257245 ) ) ;
#49659=CARTESIAN_POINT ( 'NONE',  ( -2.972980823146582186, 6.690504403638126263, 0.000000000000000000 ) ) ;
#49666=CARTESIAN_POINT ( 'NONE',  ( -7.593975437430151132, 8.032261896522864930, -0.7216878364870338292 ) ) ;
#49668=CARTESIAN_POINT ( 'NONE',  ( -4.909461021924285795, 6.821066840368686712, 1.443375672974058777 ) ) ;
#49682=CARTESIAN_POINT ( 'NONE',  ( -4.767627293860968507, 5.591261926706423857, -1.199719254218453823 ) ) ;
#49693=CARTESIAN_POINT ( 'NONE',  ( -3.820365424000704557, 7.679119771301277098, -0.7998128361456481317 ) ) ;
#49704=CARTESIAN_POINT ( 'NONE',  ( -4.586029276033976920, 8.497253585842676316, 0.07182003436798957419 ) ) ;
#49721=CARTESIAN_POINT ( 'NONE',  ( 6.658989722967328717, 7.797851427330578566, 1.199719254218452935 ) ) ;
#49726=CARTESIAN_POINT ( 'NONE',  ( 1.806654366501771136, 0.000000000000000000, 2.419999999999998597 ) ) ;
#49747=CARTESIAN_POINT ( 'NONE',  ( 6.587282531393223728, 8.778525268082516320, 1.599625672291268286 ) ) ;
#49748=CARTESIAN_POINT ( 'NONE',  ( 5.682802662783380754, 6.658966523782627434, 1.199719254218452935 ) ) ;
#49750=CARTESIAN_POINT ( 'NONE',  ( 5.727393547130178675, 5.646656991265468939, 0.000000000000000000 ) ) ;
#49754=CARTESIAN_POINT ( 'NONE',  ( -5.817857313595549584, 6.920493299683823096, 1.082531754730549078 ) ) ;
#49757=B_SPLINE_CURVE_WITH_KNOTS ( 'NONE', 3,
 ( #106060, #92981, #125541, #160087, #189386, #23675, #77762, #41028, #75645, #11690 ),
 .UNSPECIFIED., .F., .F.,
 ( 4, 3, 3, 4 ),
 ( 0.000000000000000000, 6.254645189632222226E-05, 9.576573040555354656E-05, 0.0001290265995014244630 ),
 .UNSPECIFIED. ) ;
#49763=CARTESIAN_POINT ( 'NONE',  ( 5.318333368960210805, 7.618274611128187601, -1.232678415538956518 ) ) ;
#49764=CARTESIAN_POINT ( 'NONE',  ( -5.926322542504872892, 8.007405281046052536, -1.443375672974066548 ) ) ;
#49765=CARTESIAN_POINT ( 'NONE',  ( 5.234856708652235291, 5.279956712948652431, 0.7216878364870338292 ) ) ;
#49784=( BOUNDED_CURVE ( )  B_SPLINE_CURVE ( 2, ( #93191, #137665, #74786, #88916, #141951 ),
 .UNSPECIFIED., .F., .T. ) 
 B_SPLINE_CURVE_WITH_KNOTS ( ( 3, 2, 3 ),
 ( 0.02182863351722338224, 0.02500000000000000139, 0.02741006098507890384 ),
 .UNSPECIFIED. ) 
 CURVE ( )  GEOMETRIC_REPRESENTATION_ITEM ( )  RATIONAL_B_SPLINE_CURVE ( ( 0.9368349873065047184, 0.9490140947222125423, 1.000000000000000000, 0.9612535663203012337, 0.9449186369899758020 ) ) 
 REPRESENTATION_ITEM ( '' )  );
#49789=CARTESIAN_POINT ( 'NONE',  ( 4.193214648376505593, 8.114110533073061404, 0.000000000000000000 ) ) ;
#49791=CARTESIAN_POINT ( 'NONE',  ( 3.386504508363381571, 7.172948703057747011, -0.7998128361456362523 ) ) ;
#49821=CARTESIAN_POINT ( 'NONE',  ( 4.667750024854814050, 8.667735138964429709, -0.7998128361456381397 ) ) ;
#49825=CARTESIAN_POINT ( 'NONE',  ( -6.492041734278776843, 6.763935894940780180, 0.1675349064616058481 ) ) ;
#49826=CARTESIAN_POINT ( 'NONE',  ( 6.038177310039780643, 8.137902509836795417, -1.599625672291283607 ) ) ;
#49831=ORIENTED_EDGE ( 'NONE', *, *, #115920, .T. ) ;
#49835=CARTESIAN_POINT ( 'NONE',  ( -1.844031106778978302, 8.927559574663328945, 0.7750000000000013545 ) ) ;
#49836=CARTESIAN_POINT ( 'NONE',  ( 4.851297196472967421, 8.072458764906237150, -0.9094135686919021522 ) ) ;
#49844=CARTESIAN_POINT ( 'NONE',  ( -7.065207446497166366, 9.336104335703744539, 0.000000000000000000 ) ) ;
#49859=CARTESIAN_POINT ( 'NONE',  ( -7.391130018105325661, 8.652015104991543026, -1.199719254218452047 ) ) ;
#49861=CARTESIAN_POINT ( 'NONE',  ( 6.550524494058025837, 7.671308660269694712, -1.199719254218452047 ) ) ;
#49865=CARTESIAN_POINT ( 'NONE',  ( -5.017926250833627755, 5.026871178826882947, 0.7216878364870257245 ) ) ;
#49870=CYLINDRICAL_SURFACE ( 'NONE', #165490, 1.250000000000000000 ) ;
#49876=CARTESIAN_POINT ( 'NONE',  ( -0.1074958596846934122, 2.600571376352757813, -2.078930272764640375 ) ) ;
#49894=CARTESIAN_POINT ( 'NONE',  ( 5.383996398402570271, 9.295429874862735531, 0.000000000000000000 ) ) ;
#49896=EDGE_CURVE ( 'NONE', #184855, #38781, #80134, .T. ) ;
#49898=CARTESIAN_POINT ( 'NONE',  ( 1.833030277982334422, 0.000000000000000000, -2.500000000000000444 ) ) ;
#49909=CARTESIAN_POINT ( 'NONE',  ( -3.512971199716682591, 7.112567143062499930, 0.000000000000000000 ) ) ;
#49911=CARTESIAN_POINT ( 'NONE',  ( 5.387385936583818591, 7.378645907471495846, -1.599625672291283607 ) ) ;
#49916=CARTESIAN_POINT ( 'NONE',  ( -3.142457743317409680, 6.888227477170756785, 0.7998128361456352531 ) ) ;
#49926=CARTESIAN_POINT ( 'NONE',  ( 0.000000000000000000, 8.499999999999996447, 0.000000000000000000 ) ) ;
#49929=DIRECTION ( 'NONE',  ( 0.6507913734559640506, -0.7592566023653003482, 0.000000000000000000 ) ) ;
#49954=CARTESIAN_POINT ( 'NONE',  ( 3.390947817193682656, 6.009837315817661008, -1.082531754730549967 ) ) ;
#49959=CARTESIAN_POINT ( 'NONE',  ( 5.713835393516482952, 5.630839145382857680, 0.7998128361456352531 ) ) ;
#49961=CARTESIAN_POINT ( 'NONE',  ( -4.163462365945426846, 7.871304665867801198, 0.01791990254118821721 ) ) ;
#49965=CARTESIAN_POINT ( 'NONE',  ( -5.763624699140883934, 6.857221916153382502, -1.082531754730549967 ) ) ;
#49971=CARTESIAN_POINT ( 'NONE',  ( -5.803772275101700906, 8.928762199997411386, -1.199719254218452047 ) ) ;
#49975=ORIENTED_EDGE ( 'NONE', *, *, #88237, .T. ) ;
#49977=CARTESIAN_POINT ( 'NONE',  ( 3.615147460157889903, 7.348606074266929689, 0.4009180521483968196 ) ) ;
#49980=CARTESIAN_POINT ( 'NONE',  ( -5.010620288702242853, 8.003418215864698482, -1.199719254218453823 ) ) ;
#49983=CARTESIAN_POINT ( 'NONE',  ( 4.842126824027952026, 8.201492973507317430, 0.9351865777775794086 ) ) ;
#49988=CARTESIAN_POINT ( 'NONE',  ( 6.638652492546827766, 7.774124658506663010, 1.199719254218452047 ) ) ;
#49994=FACE_OUTER_BOUND ( 'NONE', #72789, .T. ) ;
#49995=CARTESIAN_POINT ( 'NONE',  ( -3.806807270387036368, 7.663301925418665839, 0.000000000000000000 ) ) ;
#49999=CARTESIAN_POINT ( 'NONE',  ( -6.635789839245807897, 6.706452665400368218, 0.7998128361456341429 ) ) ;
#50003=CARTESIAN_POINT ( 'NONE',  ( 6.007671464186825183, 8.102312356341712984, 1.443375672974064550 ) ) ;
#50005=CARTESIAN_POINT ( 'NONE',  ( -7.227905289416804102, 8.565549271475310533, -1.082531754730549967 ) ) ;
#50011=CARTESIAN_POINT ( 'NONE',  ( 5.180097208873055692, 8.201141289397330780, -1.199719254218450271 ) ) ;
#50027=CARTESIAN_POINT ( 'NONE',  ( 6.454497976780569246, 6.866128686250288382, -0.6735470152485992790 ) ) ;
#50044=CARTESIAN_POINT ( 'NONE',  ( 4.893454165248502186, 8.027304163657891678, -0.9628252682179049282 ) ) ;
#50053=CARTESIAN_POINT ( 'NONE',  ( 7.506374323821472849, 8.786466794993730289, -1.199719254218452047 ) ) ;
#50059=CARTESIAN_POINT ( 'NONE',  ( -5.622963654236769138, 7.379252650573795869, -1.237363127855268141 ) ) ;
#50079=CARTESIAN_POINT ( 'NONE',  ( -4.145761110728687804, 8.058748072483927771, -0.7998128361456481317 ) ) ;
#50081=CARTESIAN_POINT ( 'NONE',  ( 5.989670002187236442, 10.20997511251894529, -0.7998128361456481317 ) ) ;
#50093=CARTESIAN_POINT ( 'NONE',  ( 6.017840079619279692, 8.114175741012878973, -1.599625672291281386 ) ) ;
#50096=CARTESIAN_POINT ( 'NONE',  ( 7.336370518326124746, 7.731722824234849689, -0.7216878364870317197 ) ) ;
#50109=CARTESIAN_POINT ( 'NONE',  ( -6.798487682609798632, 6.896266815991691779, 0.7998128361456341429 ) ) ;
#50111=CARTESIAN_POINT ( 'NONE',  ( 3.718679271898170491, 7.560485927181699317, 0.7998128361456271485 ) ) ;
#50115=EDGE_CURVE ( 'NONE', #136751, #80820, #49080, .T. ) ;
#50120=CARTESIAN_POINT ( 'NONE',  ( -2.993318053567081360, 6.714231172462041819, 0.000000000000000000 ) ) ;
#50121=CARTESIAN_POINT ( 'NONE',  ( 7.205232291019763480, 7.370802192470005565, -0.7998128361456341429 ) ) ;
#50123=CARTESIAN_POINT ( 'NONE',  ( -5.763039058787290614, 7.049721345481786194, -2.500000000000000000 ) ) ;
#50128=CARTESIAN_POINT ( 'NONE',  ( 4.366607992053101128, 7.252070536440704096, -1.199719254218448494 ) ) ;
#50134=CARTESIAN_POINT ( 'NONE',  ( -6.606716786301501720, 6.763562328987043237, 0.1806677948501221598 ) ) ;
#50142=CARTESIAN_POINT ( 'NONE',  ( -6.420668264523499147, 9.648474187656182366, 1.199719254218452935 ) ) ;
#50147=CARTESIAN_POINT ( 'NONE',  ( -7.013428937081410020, 5.939655416065873439, 2.436399677959149024 ) ) ;
#50154=CARTESIAN_POINT ( 'NONE',  ( -5.765600714192440357, 7.067438534623913249, 2.440103264412582185 ) ) ;
#50156=EDGE_CURVE ( 'NONE', #8487, #96867, #182183, .T. ) ;
#50174=CARTESIAN_POINT ( 'NONE',  ( 3.725458348705031231, 7.568394850123006279, -1.734723475976807094E-15 ) ) ;
#50193=AXIS2_PLACEMENT_3D ( 'NONE', #172162, #91995, #59462 ) ;
#50195=CARTESIAN_POINT ( 'NONE',  ( 5.713835393516482952, 5.630839145382857680, 0.7998128361456352531 ) ) ;
#50196=CARTESIAN_POINT ( 'NONE',  ( -3.689227196694346400, 6.357829925235092716, -1.082531754730546636 ) ) ;
#50221=CARTESIAN_POINT ( 'NONE',  ( -6.444921918449773024, 8.612437886315108315, 1.599625672291269396 ) ) ;
#50223=CARTESIAN_POINT ( 'NONE',  ( 5.668717623845194176, 9.627604637879139560, 0.000000000000000000 ) ) ;
#50236=CARTESIAN_POINT ( 'NONE',  ( -6.505933609711270549, 8.683618192786854095, -1.599625672291271394 ) ) ;
#50243=CARTESIAN_POINT ( 'NONE',  ( 3.444653546323793947, 6.176457016423196222, 1.199719254218451159 ) ) ;
#50248=CARTESIAN_POINT ( 'NONE',  ( -4.960304097753355457, 6.880383762169266504, 1.599625672291263179 ) ) ;
#50253=CARTESIAN_POINT ( 'NONE',  ( -6.455090533882201775, 8.624301270986276080, -1.443375672974066548 ) ) ;
#50255=CARTESIAN_POINT ( 'NONE',  ( -6.577113915960836721, 8.766661883411348555, -1.443375672974066548 ) ) ;
#50256=CARTESIAN_POINT ( 'NONE',  ( 8.188198428010544205, 8.517596018959260107, 0.000000000000000000 ) ) ;
#50258=CARTESIAN_POINT ( 'NONE',  ( -3.323157048681004699, 6.891117300187535655, -0.7216878364870458196 ) ) ;
#50272=CARTESIAN_POINT ( 'NONE',  ( -0.2855459137565004024, 2.699313886258678963, 1.981008070493679218 ) ) ;
#50276=CARTESIAN_POINT ( 'NONE',  ( 1.860129666708600693, 2.485233703330023580, 2.479905445520987239 ) ) ;
#50277=CARTESIAN_POINT ( 'NONE',  ( 6.606590233575550641, 6.765807905838774339, 0.03828827652692379235 ) ) ;
#50298=CARTESIAN_POINT ( 'NONE',  ( 6.093313910611117379, 7.014445836765536235, -0.9825430356366869900 ) ) ;
#50309=B_SPLINE_SURFACE_WITH_KNOTS ( 'NONE', 1, 3, ( 
 ( #171853, #136165, #54903, #104735, #170781, #21302, #38655, #39720, #89558, #118896, #187023, #53840, #73266, #184881, #105827, #23448, #202183, #139371, #71122, #137238, #203260, #87409, #155609, #205401, #22371, #88483, #6123, #138300, #57041, #70051, #152404, #119971, #185948, #3983, #204315, #169712, #123207, #153473, #37580, #55972, #52761, #103664, #36506, #102586, #168645, #20248, #100089, #17736, #181333, #133695, #51344, #182384, #53467, #34014, #118534, #199699, #197578, #36138, #15618, #85971, #150987, #35068, #147789, #166150, #117469, #83825, #149918, #49222, #183462, #102221, #101139, #32960, #97984, #3616, #1486, #167227, #81708, #50277, #99035, #213805, #184517, #119604, #132624, #116396, #69694, #66484, #67551, #65427, #200758, #18813, #84900, #164043, #2551, #68626, #19887, #134749, #52407, #148840, #168290, #135798, #152046, #201822, #16681, #31907, #131577, #115341, #165091, #82766, #412, #198630, #70755, #37218, #153106, #139010, #140085, #137935, #104365, #169353, #156320, #171487, #21999, #122843, #170410, #88109, #71825, #154180, #87034, #186661, #187726, #58806, #5748, #207181, #90253, #24150, #55604, #40441, #107624, #206110, #121759, #73992, #203957, #57742, #123900, #189868, #38288, #20938, #141171, #39355, #185588, #105451, #75059, #4681, #103291, #136867, #202893, #41511, #54538, #155245, #188805, #106542, #205033, #23078, #120685, #89194, #6827, #72906, #56678, #172567, #157390, #7903, #173655, #25229, #91332, #8984, #192256, #143575, #209567, #159778, #13520, #30865, #28716, #61213, #94803, #127370, #63346, #10316, #26569, #142499, #208505, #92674, #193341, #176046, #195486, #11378, #158718, #178175, #162993, #60140, #79593, #126297, #47120, #76390, #44986, #111095, #43919, #177101, #160851, #77457, #96943, #12443, #161930, #78522, #110034, #145712, #59073, #129505, #194408, #144639, #191191, #210654, #62282, #128442, #46050, #27639 ),
 ( #112171, #125233, #93739, #29790, #42858, #211710, #75330, #95875, #113237, #179241, #141447, #207454, #108965, #174985, #148859, #100109, #80669, #32978, #133715, #2576, #149936, #165109, #131596, #151006, #200777, #182407, #66504, #213828, #433, #64413, #183481, #132643, #166170, #146760, #99054, #199721, #68646, #1505, #16701, #197598, #134769, #52429, #34036, #198649, #65445, #82787, #50298, #118555, #212778, #116416, #180302, #184536, #114304, #130559, #196549, #17758, #35090, #181352, #147809, #48192, #51367, #83847, #49241, #67571, #115360, #117490, #101160, #167246, #31924, #15639, #18834, #102238, #84918, #36159, #14574, #98003, #164060, #81726, #156341, #19907, #203976, #87055, #74012, #85992, #106563, #90272, #206131, #24169, #70774, #22019, #88129, #38308, #172590, #123922, #121780, #154200, #187747, #5767, #7926, #103311, #56697, #140104, #39375, #104385, #55623, #119624, #71848, #188825, #57761, #53486, #105472, #189890, #41531, #136887, #168309, #152066, #170432, #3636, #137956, #171505, #201842, #155266, #69715, #135818, #185608, #37240, #169373, #20957, #23098, #89213, #122864, #153127, #4698, #186680, #202914, #6847, #54559, #72925, #120705, #139031, #205055, #40459, #91350, #211458, #63093, #77200, #9003, #13272, #94554, #209313, #62038, #43667, #159524, #157412, #79345, #42604, #60960, #128192, #109784, #11123, #75078, #145463, #108711, #210396, #141191, #126039, #129262, #107643, #76141, #144395, #195232, #192002, #175793, #160592, #143319, #194153, #207201, #173675, #59890, #25250, #12199, #78269, #27384, #176847, #29536, #45801, #93485, #111922, #142244, #177922, #95628, #161678, #174739, #58826, #124979, #26312, #190940, #92425, #158465, #10065, #208256, #127117, #193084, #44734, #110841, #28460, #198402, #116167, #184, #114058, #64167, #130310, #96697, #15385, #16448, #14318, #18591, #180051, #132400, #65200, #196297, #17509, #31673, #50044 ) ),
 .UNSPECIFIED., .F., .T., .F.,
 ( 2, 2 ),
 ( 4, 2, 2, 2, 2, 2, 2, 2, 2, 2, 2, 2, 2, 2, 2, 2, 2, 2, 2, 2, 2, 2, 2, 2, 2, 2, 2, 2, 2, 2, 2, 2, 2, 2, 2, 2, 2, 2, 2, 2, 2, 2, 2, 2, 2, 2, 2, 2, 2, 2, 2, 2, 2, 2, 2, 2, 2, 2, 2, 2, 2, 2, 2, 2, 2, 2, 2, 2, 2, 2, 2, 2, 2, 2, 2, 2, 2, 2, 2, 2, 2, 2, 2, 2, 2, 2, 2, 2, 2, 2, 2, 2, 2, 2, 2, 2, 2, 2, 2, 2, 2, 2, 2, 2, 2, 2, 2, 2, 2, 2, 2, 4 ),
 ( 0.000000000000000000, 1.000000000000000000 ),
 ( 0.0003185708494972700616, 0.0004481554763622086794, 0.0005777401032271472971, 0.0007073247300920859149, 0.0008369093569570245326, 0.0009017016703894938957, 0.0009664939838219631504, 0.001031286297254432405, 0.001096078610686901768, 0.001225663237551840277, 0.001290455550984309641, 0.001322851707700544322, 0.001355247864416779004, 0.001420040177849248367, 0.001484832491281717730, 0.001614417118146656239, 0.001679209431579125385, 0.001744001745011594749, 0.001808794058444064112, 0.001873586371876533475, 0.001938378685309002621, 0.002003170998741471767, 0.002067963312173941130, 0.002132755625606410493, 0.002197547939038879856, 0.002229944095755114538, 0.002262340252471349220, 0.002391924879336287946, 0.002521509506201226672, 0.002586301819633696035, 0.002651094133066165398, 0.002715886446498634761, 0.002780678759931104124, 0.002910263386796042417, 0.002975055700228511346, 0.003039848013660980709, 0.003104640327093450072, 0.003169432640525919435, 0.003299017267390858162, 0.003428601894255796888, 0.003493394207688266251, 0.003558186521120735614, 0.003622978834553204977, 0.003687771147985673906, 0.003817355774850612199, 0.003946940401715550925, 0.003979336558431785173, 0.004011732715148020288, 0.004076525028580489651, 0.004141317342012959014, 0.004206109655445428377, 0.004270901968877897741, 0.004335694282310367104, 0.004400486595742836467, 0.004465278909175305830, 0.004594863536040244556, 0.004659655849472713919, 0.004724448162905183282, 0.004789240476337652645, 0.004854032789770122008, 0.004918825103202591371, 0.004983617416635060735, 0.005048409730067530098, 0.005113202043499999461, 0.005177994356932468824, 0.005210390513648703939, 0.005242786670364938187, 0.005372371297229876913, 0.005501955924094814772, 0.005566748237527284135, 0.005631540550959752631, 0.005696332864392221994, 0.005761125177824691357, 0.005890709804689630083, 0.005955502118122099446, 0.006020294431554568809, 0.006085086744987038172, 0.006149879058419507535, 0.006214671371851976898, 0.006279463685284446262, 0.006409048312149384988, 0.006473840625581854351, 0.006506236782298089466, 0.006538632939014323714, 0.006603425252446793077, 0.006668217565879262440, 0.006797802192744201166, 0.006862594506176670529, 0.006927386819609139892, 0.006992179133041609256, 0.007056971446474078619, 0.007121763759906547982, 0.007186556073339017345, 0.007251348386771486708, 0.007316140700203956071, 0.007380933013636425434, 0.007445725327068894797, 0.007510517640501363293, 0.007575309953933832656, 0.007704894580798770515, 0.007769686894231239878, 0.007834479207663709241, 0.007866875364379945224, 0.007899271521096179471, 0.007964063834528647967, 0.008093648461393586693, 0.008158440774826056924, 0.008223233088258525419, 0.008288025401690993915, 0.008352817715123464146, 0.008482402341988402872, 0.008611986968853341598 ),
 .UNSPECIFIED. ) ;
#50311=CARTESIAN_POINT ( 'NONE',  ( 7.635176783151273128, 8.936736330878529699, 1.199719254218452935 ) ) ;
#50314=CARTESIAN_POINT ( 'NONE',  ( -4.630991987519598396, 7.560518531151607213, 1.199719254218452935 ) ) ;
#50327=CARTESIAN_POINT ( 'NONE',  ( 3.711900195091365262, 7.552577004240394132, -0.7998128361456362523 ) ) ;
#50329=CARTESIAN_POINT ( 'NONE',  ( 6.912678218121202534, 9.158153569265168770, 1.599625672291268286 ) ) ;
#50334=CARTESIAN_POINT ( 'NONE',  ( -7.729556973122450714, 8.190440354830551328, 0.000000000000000000 ) ) ;
#50340=CARTESIAN_POINT ( 'NONE',  ( 5.840530312436913007, 10.03597880781023299, 0.000000000000000000 ) ) ;
#50354=CARTESIAN_POINT ( 'NONE',  ( -5.153507786970267013, 8.066157280557016307, -1.082531754730549967 ) ) ;
#50355=CARTESIAN_POINT ( 'NONE',  ( 5.736508392357904107, 5.865217010605237924, 0.000000000000000000 ) ) ;
#50358=EDGE_CURVE ( 'NONE', #96370, #141262, #93659, .T. ) ;
#50365=CARTESIAN_POINT ( 'NONE',  ( -5.307090785106547415, 5.156303768904543894, -0.7998128361456362523 ) ) ;
#50366=CARTESIAN_POINT ( 'NONE',  ( -7.322812365156824654, 8.676274193172000437, 1.082531754730549078 ) ) ;
#50367=CARTESIAN_POINT ( 'NONE',  ( 1.854520591217061476, 2.487866942973022244, -2.484107071883403961 ) ) ;
#50370=CARTESIAN_POINT ( 'NONE',  ( 4.706088717274895750, 6.583799151611112954, 1.443375672974065660 ) ) ;
#50389=CARTESIAN_POINT ( 'NONE',  ( -3.980200614063634568, 6.801261928786307642, 1.199719254218452935 ) ) ;
#50403=CARTESIAN_POINT ( 'NONE',  ( 4.228163802615382494, 6.026220084508304708, -1.599625672291269396 ) ) ;
#50437=DIRECTION ( 'NONE',  ( -0.000000000000000000, 1.000000000000000000, -0.000000000000000000 ) ) ;
#50441=CARTESIAN_POINT ( 'NONE',  ( 4.909461021924240498, 7.781436054670031410, 1.082531754730549078 ) ) ;
#50442=ORIENTED_EDGE ( 'NONE', *, *, #69350, .T. ) ;
#50447=CARTESIAN_POINT ( 'NONE',  ( 6.509323147892504657, 6.766834225395614411, 0.000000000000000000 ) ) ;
#50460=CARTESIAN_POINT ( 'NONE',  ( -6.794571259104023930, 7.956029886156682274, 1.199719254218452047 ) ) ;
#50470=CARTESIAN_POINT ( 'NONE',  ( 3.512971199272317602, 6.152197928242737923, -1.082531754730549967 ) ) ;
#50476=CARTESIAN_POINT ( 'NONE',  ( -5.562588163356775972, 9.711712967216715953, 0.7998128361456291469 ) ) ;
#50483=CARTESIAN_POINT ( 'NONE',  ( -5.099275172515603138, 8.002885897026576600, 1.082531754730549967 ) ) ;
#50486=CARTESIAN_POINT ( 'NONE',  ( -5.478376588373717659, 8.549133898814758936, -1.199719254218452047 ) ) ;
#50508=CARTESIAN_POINT ( 'NONE',  ( -8.093291352714894415, 8.406871097780989288, -0.7998128361456362523 ) ) ;
#50509=CARTESIAN_POINT ( 'NONE',  ( 3.549202351727371862, 7.362762853649070571, -0.7998128361456362523 ) ) ;
#50510=CARTESIAN_POINT ( 'NONE',  ( -5.281783360975562225, 8.319775133516907673, 1.199719254218452935 ) ) ;
#50541=EDGE_CURVE ( 'NONE', #69383, #202042, #53265, .T. ) ;
#50561=CARTESIAN_POINT ( 'NONE',  ( 4.061549535745618833, 6.896169004081968090, -1.199719254218452047 ) ) ;
#50573=CARTESIAN_POINT ( 'NONE',  ( 4.871809496981259535, 8.050285353323946680, -0.9368363805376724862 ) ) ;
#50575=CARTESIAN_POINT ( 'NONE',  ( 3.984117037569365305, 5.741498858621315371, 1.599625672291261402 ) ) ;
#50581=CARTESIAN_POINT ( 'NONE',  ( -4.613517410400161722, 8.604463755433990002, -0.7998128361456362523 ) ) ;
#50586=CARTESIAN_POINT ( 'NONE',  ( -6.197485614778184271, 9.284131412999601096, 1.082531754730549967 ) ) ;
#50588=CARTESIAN_POINT ( 'NONE',  ( -4.489157070319179432, 8.251450656689856444, 5.811111664500048210E-05 ) ) ;
#50592=CARTESIAN_POINT ( 'NONE',  ( 6.265276383290871109, 7.442482214328385304, -1.082531754730548412 ) ) ;
#50595=CARTESIAN_POINT ( 'NONE',  ( -5.808742468812186033, 5.741564066561132940, 0.000000000000000000 ) ) ;
#50607=CARTESIAN_POINT ( 'NONE',  ( 5.415556014015861841, 5.282846535965431300, -0.7998128361456481317 ) ) ;
#50608=CARTESIAN_POINT ( 'NONE',  ( 5.086243903782109221, 5.962981304947771122, -1.199719254218452047 ) ) ;
#50629=ORIENTED_EDGE ( 'NONE', *, *, #52880, .F. ) ;
#50641=CARTESIAN_POINT ( 'NONE',  ( 7.367930134383754215, 7.560616343061329125, -0.7998128361456341429 ) ) ;
#50647=CARTESIAN_POINT ( 'NONE',  ( 5.750066545971570520, 5.881034856487848295, -0.7216878364870458196 ) ) ;
#50651=CARTESIAN_POINT ( 'NONE',  ( 7.038091139269835317, 7.383730215335837954, 0.000000000000000000 ) ) ;
#50664=CARTESIAN_POINT ( 'NONE',  ( -7.105881907338178038, 7.462819444748888920, -0.7216878364870338292 ) ) ;
#50699=CARTESIAN_POINT ( 'NONE',  ( 6.587282531393223728, 8.778525268082516320, 1.599625672291268286 ) ) ;
#50701=CARTESIAN_POINT ( 'NONE',  ( 6.873057527484919937, 6.983264968346048818, 0.7998128361456352531 ) ) ;
#50714=CARTESIAN_POINT ( 'NONE',  ( -5.984998465789844069, 5.947196063035064206, 0.7998128361456281477 ) ) ;
#50716=CARTESIAN_POINT ( 'NONE',  ( 4.787437638956922648, 6.678706226906775179, -1.443375672974068769 ) ) ;
#50730=CARTESIAN_POINT ( 'NONE',  ( -7.431277594066160397, 7.842447745931541370, -0.7216878364870338292 ) ) ;
#50732=CARTESIAN_POINT ( 'NONE',  ( -5.641601317062247212, 7.675230518029648508, -1.443375672974066548 ) ) ;
#50747=VERTEX_POINT ( 'NONE', #155037 ) ;
#50757=CARTESIAN_POINT ( 'NONE',  ( -5.164730172163054966, 4.990216387137135889, -0.7998128361456362523 ) ) ;
#50764=B_SPLINE_CURVE_WITH_KNOTS ( 'NONE', 3,
 ( #91620, #41800, #23365, #18299, #155529, #6040, #120972, #157671, #72111, #105742, #206392, #170696, #54823, #107913, #138220, #55885 ),
 .UNSPECIFIED., .F., .F.,
 ( 4, 3, 3, 3, 3, 4 ),
 ( 0.000000000000000000, 2.533473342638976539E-05, 5.061406379858726976E-05, 7.673069672129158672E-05, 0.0001048028779199228796, 0.0001300696341146173867 ),
 .UNSPECIFIED. ) ;
#50768=CARTESIAN_POINT ( 'NONE',  ( 4.057816120971201812, 3.809087209364407478, -2.500000000000000888 ) ) ;
#50769=CARTESIAN_POINT ( 'NONE',  ( -5.031572470839103417, 8.001347149079229837, -1.166850223539055875 ) ) ;
#50773=ORIENTED_EDGE ( 'NONE', *, *, #133776, .T. ) ;
#50787=CARTESIAN_POINT ( 'NONE',  ( 4.688087255275310561, 8.691461907788344377, -0.7998128361456381397 ) ) ;
#50795=CARTESIAN_POINT ( 'NONE',  ( 2.969872605471563176, 6.610416373784151034, 0.02023234969686484030 ) ) ;
#50812=CARTESIAN_POINT ( 'NONE',  ( 5.936491157937257235, 8.019268665717216749, 1.599625672291268286 ) ) ;
#50813=CARTESIAN_POINT ( 'NONE',  ( 6.561219994370630637, 6.619454513046008515, 0.000000000000000000 ) ) ;
#50815=CARTESIAN_POINT ( 'NONE',  ( 4.203910148689107729, 7.062256385849379647, -1.199719254218448494 ) ) ;
#50829=CARTESIAN_POINT ( 'NONE',  ( 5.348725299209624140, 7.591689785053232775, -1.238827213252717163 ) ) ;
#50830=CARTESIAN_POINT ( 'NONE',  ( -5.709392084686210289, 8.714688961225625974, 1.082531754730550855 ) ) ;
#50831=CARTESIAN_POINT ( 'NONE',  ( 4.204437034013637664, 6.958908068774287692, -1.082531754730548412 ) ) ;
#50833=AXIS2_PLACEMENT_3D ( 'NONE', #188080, #205393, #123198 ) ;
#50858=CARTESIAN_POINT ( 'NONE',  ( 7.178115983792402233, 7.339166500704784823, 0.7998128361456281477 ) ) ;
#50859=EDGE_CURVE ( 'NONE', #192662, #6739, #210530, .T. ) ;
#50861=VECTOR ( 'NONE', #52059, 1000.000000000000114 ) ;
#50889=CARTESIAN_POINT ( 'NONE',  ( 5.481239241674765950, 9.616805891921051952, -0.7998128361456481317 ) ) ;
#50893=CARTESIAN_POINT ( 'NONE',  ( -6.488192154978348114, 6.766396236290696642, 0.1981293719705672085 ) ) ;
#50894=CARTESIAN_POINT ( 'NONE',  ( 5.742760583840166966, 8.857581893525663830, 1.199719254218452047 ) ) ;
#50903=CARTESIAN_POINT ( 'NONE',  ( -1.865214468731750452, 8.973543201141316317, 0.7750000000000013545 ) ) ;
#50921=CARTESIAN_POINT ( 'NONE',  ( 2.929970594329034395, 6.432399770110250437, -0.7216878364870338292 ) ) ;
#50927=CARTESIAN_POINT ( 'NONE',  ( -7.306918443122272677, 7.489436036589583345, 0.7998128361456341429 ) ) ;
#50929=CARTESIAN_POINT ( 'NONE',  ( 5.027041095616958444, 9.086908054853605421, 0.000000000000000000 ) ) ;
#50938=DIRECTION ( 'NONE',  ( 0.000000000000000000, -1.000000000000000000, 0.000000000000000000 ) ) ;
#50951=CARTESIAN_POINT ( 'NONE',  ( 7.018280793729500644, 8.217024343219755167, -1.199719254218452047 ) ) ;
#50960=CARTESIAN_POINT ( 'NONE',  ( 7.865138509703455405, 8.348618814175074121, -0.7216878364870317197 ) ) ;
#50974=CARTESIAN_POINT ( 'NONE',  ( -4.340018570150318666, 6.156717313299049366, -1.443375672974066548 ) ) ;
#50976=CARTESIAN_POINT ( 'NONE',  ( 6.873057527484919937, 6.983264968346048818, 0.7998128361456352531 ) ) ;
#50982=CARTESIAN_POINT ( 'NONE',  ( -5.666381855868691808, 5.575476684793721383, 0.000000000000000000 ) ) ;
#50995=CARTESIAN_POINT ( 'NONE',  ( -4.272227801637582090, 7.998366511970294468, 0.7216878364870059626 ) ) ;
#50997=CARTESIAN_POINT ( 'NONE',  ( 7.634649897826744080, 9.040084647953621655, 1.082531754730549078 ) ) ;
#51010=ORIENTED_EDGE ( 'NONE', *, *, #50541, .F. ) ;
#51023=CARTESIAN_POINT ( 'NONE',  ( 4.421367491832282504, 5.291255174293369556, 1.082531754730549078 ) ) ;
#51028=CARTESIAN_POINT ( 'NONE',  ( 5.578253857379852576, 5.472660686556754861, -0.7998128361456481317 ) ) ;
#51030=CARTESIAN_POINT ( 'NONE',  ( -5.984998465789844069, 5.947196063035064206, 0.7998128361456281477 ) ) ;
#51034=CARTESIAN_POINT ( 'NONE',  ( -4.936577328707246082, 8.773440960218172435, 0.000000000000000000 ) ) ;
#51039=VERTEX_POINT ( 'NONE', #187740 ) ;
#51040=CARTESIAN_POINT ( 'NONE',  ( -5.413448473606448985, 9.537716662508005427, 0.000000000000000000 ) ) ;
#51048=CARTESIAN_POINT ( 'NONE',  ( -6.119526231721793330, 8.232809585132461194, 1.599625672291263179 ) ) ;
#51049=CARTESIAN_POINT ( 'NONE',  ( -5.717785742877115496, 7.006476535625803415, 2.500000000000000000 ) ) ;
#51051=CARTESIAN_POINT ( 'NONE',  ( 4.690754089986846509, 8.373302309308519042, 0.6171781843518510113 ) ) ;
#51056=CARTESIAN_POINT ( 'NONE',  ( 6.505933609711257226, 8.683618192786854095, -1.599625672291281386 ) ) ;
#51063=CARTESIAN_POINT ( 'NONE',  ( -5.601453741101424022, 6.564059448486966986, -1.199719254218453823 ) ) ;
#51065=( BOUNDED_CURVE ( )  B_SPLINE_CURVE ( 2, ( #70732, #170388, #21977, #154159, #5726, #121739, #89173 ),
 .UNSPECIFIED., .F., .T. ) 
 B_SPLINE_CURVE_WITH_KNOTS ( ( 3, 2, 2, 3 ),
 ( 0.4000000000000002998, 0.4083333333333336590, 0.4166666666666671293, 0.4250000000000004885 ),
 .UNSPECIFIED. ) 
 CURVE ( )  GEOMETRIC_REPRESENTATION_ITEM ( )  RATIONAL_B_SPLINE_CURVE ( ( 0.9999999999999955591, 0.8660254037844431485, 1.000000000000000000, 0.8660254037844387076, 1.000000000000000000, 0.8660254037844307140, 1.000000000000007994 ) ) 
 REPRESENTATION_ITEM ( '' )  );
#51068=CARTESIAN_POINT ( 'NONE',  ( -5.803772275101700906, 8.928762199997411386, -1.199719254218452047 ) ) ;
#51071=CARTESIAN_POINT ( 'NONE',  ( 6.604230223188150894, 9.758666789477915771, -1.082531754730548412 ) ) ;
#51073=CARTESIAN_POINT ( 'NONE',  ( -7.444835747235459600, 8.818634805597074688, 1.082531754730549078 ) ) ;
#51080=CARTESIAN_POINT ( 'NONE',  ( 7.205232291019763480, 7.370802192470005565, -0.7998128361456341429 ) ) ;
#51093=CARTESIAN_POINT ( 'NONE',  ( 6.098455030413784783, 7.112933956528650015, -1.126327413477963502 ) ) ;
#51098=CARTESIAN_POINT ( 'NONE',  ( -5.606383287671886428, 5.556235044223195807, 0.1555002321169836055 ) ) ;
#51115=CARTESIAN_POINT ( 'NONE',  ( 5.969332771766739931, 10.18624834369502885, -0.7998128361456481317 ) ) ;
#51122=CARTESIAN_POINT ( 'NONE',  ( -5.527359202251545867, 7.456348097644321271, -1.248928334283349040 ) ) ;
#51141=CARTESIAN_POINT ( 'NONE',  ( -5.829079699232685208, 5.765290835385048496, 0.000000000000000000 ) ) ;
#51151=VERTEX_POINT ( 'NONE', #153120 ) ;
#51154=ORIENTED_EDGE ( 'NONE', *, *, #207587, .T. ) ;
#51157=CARTESIAN_POINT ( 'NONE',  ( 7.503511670520385479, 7.718794801887437274, 0.7998128361456281477 ) ) ;
#51158=CARTESIAN_POINT ( 'NONE',  ( -5.403060590669224617, 6.145745408126818354, 1.120749285529927697 ) ) ;
#51160=CARTESIAN_POINT ( 'NONE',  ( 5.682275777458841048, 8.683053269460405232, 1.082531754730547524 ) ) ;
#51174=CARTESIAN_POINT ( 'NONE',  ( -5.472651281771599763, 6.413789912602166687, 1.199719254218452935 ) ) ;
#51175=CARTESIAN_POINT ( 'NONE',  ( 4.532168488718122390, 8.509556680138327778, 0.7998128361456271485 ) ) ;
#51184=CARTESIAN_POINT ( 'NONE',  ( -6.831329296439251131, 9.063246493969506545, -1.599625672291271394 ) ) ;
#51185=CARTESIAN_POINT ( 'NONE',  ( 6.373214726875630731, 9.593111727067046957, 1.199719254218452047 ) ) ;
#51187=CARTESIAN_POINT ( 'NONE',  ( -3.853900823548705112, 8.531065964594302997, -2.447540105570083391 ) ) ;
#51194=CARTESIAN_POINT ( 'NONE',  ( 4.716257332707354699, 6.595662536282280719, -1.599625672291269396 ) ) ;
#51196=CARTESIAN_POINT ( 'NONE',  ( 4.875038752565570732, 7.845239757038595663, -1.199719254218452047 ) ) ;
#51201=CARTESIAN_POINT ( 'NONE',  ( -6.602617837901656017, 6.766230214585198688, 0.2136612715164920018 ) ) ;
#51211=CARTESIAN_POINT ( 'NONE',  ( -4.136646265500970365, 5.919449624541475607, -1.443375672974066548 ) ) ;
#51223=CARTESIAN_POINT ( 'NONE',  ( -3.855102659574803248, 8.506872032339188650, 2.500000000000000888 ) ) ;
#51240=CARTESIAN_POINT ( 'NONE',  ( 4.441177836928239309, 7.339068688795062911, 1.199719254218452047 ) ) ;
#51261=CARTESIAN_POINT ( 'NONE',  ( 0.3857320732078016179, 2.894052512584738501, 1.963429802559124138 ) ) ;
#51263=CARTESIAN_POINT ( 'NONE',  ( 5.551137550152489553, 5.441024994791534120, 0.7998128361456352531 ) ) ;
#51289=CARTESIAN_POINT ( 'NONE',  ( -5.444481204339554736, 8.509589284108232121, 1.199719254218454489 ) ) ;
#51291=CARTESIAN_POINT ( 'NONE',  ( 7.200788982189461507, 8.533913579710086239, -1.082531754730548412 ) ) ;
#51300=ORIENTED_EDGE ( 'NONE', *, *, #161121, .F. ) ;
#51303=CARTESIAN_POINT ( 'NONE',  ( -6.291865805193673111, 9.498204651771386509, -1.199719254218452047 ) ) ;
#51310=CARTESIAN_POINT ( 'NONE',  ( 6.337523607829048444, 6.943994947614124058, 0.8959833429097040502 ) ) ;
#51312=AXIS2_PLACEMENT_3D ( 'NONE', #33061, #114385, #130639 ) ;
#51314=DIRECTION ( 'NONE',  ( -0.7592566023653005702, -0.6507913734559640506, 0.000000000000000000 ) ) ;
#51315=CARTESIAN_POINT ( 'NONE',  ( -6.473091995881817162, 6.516638514809040217, 0.7998128361456281477 ) ) ;
#51318=CARTESIAN_POINT ( 'NONE',  ( -5.451787166470911217, 9.374519104275787384, 0.7216878364870267237 ) ) ;
#51321=CARTESIAN_POINT ( 'NONE',  ( -6.224601922005509991, 10.27613631906616476, 0.7216878364870267237 ) ) ;
#51322=CARTESIAN_POINT ( 'NONE',  ( 5.695833931072550094, 5.817763472438987726, 0.000000000000000000 ) ) ;
#51323=CARTESIAN_POINT ( 'NONE',  ( -4.299344108864961989, 6.109263775132799168, -1.443375672974066548 ) ) ;
#51325=EDGE_LOOP ( 'NONE', ( #77345, #180769, #62173, #182 ) ) ;
#51328=EDGE_CURVE ( 'NONE', #84217, #81797, #173238, .T. ) ;
#51332=ORIENTED_EDGE ( 'NONE', *, *, #70875, .T. ) ;
#51344=CARTESIAN_POINT ( 'NONE',  ( 6.252685474373055996, 7.003816019006632310, -0.9791501464874209359 ) ) ;
#51361=CIRCLE ( 'NONE', #9909, 2.000000000000000000 ) ;
#51367=CARTESIAN_POINT ( 'NONE',  ( 6.357275476766607980, 6.835366726881293431, -0.6123070361637416026 ) ) ;
#51383=CARTESIAN_POINT ( 'NONE',  ( 7.014364370223726830, 9.276787413384745662, -1.599625672291269396 ) ) ;
#51386=CARTESIAN_POINT ( 'NONE',  ( -5.387385936583832802, 7.378645907471495846, -1.599625672291271394 ) ) ;
#51399=CARTESIAN_POINT ( 'NONE',  ( 5.408776937209000657, 5.274937613024121674, 0.7998128361456352531 ) ) ;
#51401=CARTESIAN_POINT ( 'NONE',  ( 6.424584688029230328, 8.588711117491191871, 1.599625672291268286 ) ) ;
#51407=CARTESIAN_POINT ( 'NONE',  ( -7.417719440008134768, 7.826629899530511025, 0.7216878364870317197 ) ) ;
#51412=CARTESIAN_POINT ( 'NONE',  ( 6.068156270568149324, 9.237210194708310951, 1.199719254218452047 ) ) ;
#51421=CARTESIAN_POINT ( 'NONE',  ( 5.536872897005128635, 5.953237723320745189, 0.6961998893310636927 ) ) ;
#51426=CARTESIAN_POINT ( 'NONE',  ( -7.282137904315833410, 7.668451441222825515, 0.000000000000000000 ) ) ;
#51427=CARTESIAN_POINT ( 'NONE',  ( 5.072158865288233898, 7.971250205261355859, 1.082531754730549078 ) ) ;
#51437=CARTESIAN_POINT ( 'NONE',  ( -4.930325137224961907, 5.781076077297750970, -1.199719254218453823 ) ) ;
#51438=CARTESIAN_POINT ( 'NONE',  ( -6.997416678428844072, 8.296645891989347987, 1.082531754730549078 ) ) ;
#51439=CARTESIAN_POINT ( 'NONE',  ( 1.879624969287899683, 2.480000000000013305, -2.465175922436416922 ) ) ;
#51442=CARTESIAN_POINT ( 'NONE',  ( 6.183927461164522299, 6.387205924212962849, 0.000000000000000000 ) ) ;
#51453=CARTESIAN_POINT ( 'NONE',  ( -6.147489916148834332, 6.992309281770507923, 0.9361876800342925353 ) ) ;
#51457=CARTESIAN_POINT ( 'NONE',  ( -0.04117949675282415317, 3.478559061295773525, -1.999678960129391836 ) ) ;
#51458=CARTESIAN_POINT ( 'NONE',  ( 3.282482588284323821, 6.843663763058119187, 0.7216878364870257245 ) ) ;
#51461=CARTESIAN_POINT ( 'NONE',  ( -5.655686355556086120, 6.627330832017406692, 1.199719254218452935 ) ) ;
#51472=CARTESIAN_POINT ( 'NONE',  ( 3.932747076415766596, 6.745899468197171345, 1.199719254218451159 ) ) ;
#51485=CARTESIAN_POINT ( 'NONE',  ( 3.231779075379113131, 6.036511184309971689, 0.9899555337401855226 ) ) ;
#51511=CARTESIAN_POINT ( 'NONE',  ( 5.072158865288233898, 7.971250205261355859, 1.082531754730549078 ) ) ;
#51517=CARTESIAN_POINT ( 'NONE',  ( 4.692530563661249765, 8.488719734331187539, 0.000000000000000000 ) ) ;
#51542=CARTESIAN_POINT ( 'NONE',  ( -4.085803189671902480, 5.860132702740892263, -1.599625672291271394 ) ) ;
#51544=CARTESIAN_POINT ( 'NONE',  ( 5.519577934094864524, 5.612131475965050242, 0.7216878364870328300 ) ) ;
#51550=CARTESIAN_POINT ( 'NONE',  ( -7.910256278930404505, 8.193330178365746619, -0.7998128361456362523 ) ) ;
#51556=CARTESIAN_POINT ( 'NONE',  ( -4.963693636378939011, 8.805076652501815815, 0.7216878364870267237 ) ) ;
#51560=CARTESIAN_POINT ( 'NONE',  ( -6.611536185319534908, 7.742488966741438716, 1.199719254218452047 ) ) ;
#51574=CIRCLE ( 'NONE', #172641, 0.4800000000000000933 ) ;
#51580=CARTESIAN_POINT ( 'NONE',  ( -5.004368097219957789, 5.011053332944274352, 0.000000000000000000 ) ) ;
#51582=CARTESIAN_POINT ( 'NONE',  ( -5.167065940139584868, 6.161236697318522637, 1.082531754730549078 ) ) ;
#51583=CARTESIAN_POINT ( 'NONE',  ( 3.223806664999388172, 6.983134552466421674, -0.7998128361456362523 ) ) ;
#51584=CARTESIAN_POINT ( 'NONE',  ( -4.573896719763875574, 6.429575154514868274, -1.599625672291271394 ) ) ;
#51585=CARTESIAN_POINT ( 'NONE',  ( -6.577640801285370209, 7.702944352034914566, -1.199719254218452047 ) ) ;
#51586=ORIENTED_EDGE ( 'NONE', *, *, #96537, .T. ) ;
#51641=CARTESIAN_POINT ( 'NONE',  ( 3.573456005653643519, 6.326726552307992080, -1.199719254218453823 ) ) ;
#51656=CARTESIAN_POINT ( 'NONE',  ( 4.661274270878652537, 8.290979908523663511, 0.5017903844357074483 ) ) ;
#51659=CARTESIAN_POINT ( 'NONE',  ( 3.217027588192558074, 6.975225629525113824, -1.734723475976807094E-15 ) ) ;
#51665=CARTESIAN_POINT ( 'NONE',  ( -4.911796789900812144, 8.952456364851418158, 0.7998128361456291469 ) ) ;
#51671=SPHERICAL_SURFACE ( 'NONE', #117188, 0.08000000000000000167 ) ;
#51673=CARTESIAN_POINT ( 'NONE',  ( -4.662342535738044802, 8.068669011459252971, 0.7682199413396522125 ) ) ;
#51678=CARTESIAN_POINT ( 'NONE',  ( 6.712695452541852070, 7.004101914153185504, 0.000000000000000000 ) ) ;
#51681=CARTESIAN_POINT ( 'NONE',  ( -5.635349125135588721, 6.603604063193491136, 1.199719254218452935 ) ) ;
#51693=CARTESIAN_POINT ( 'NONE',  ( 4.146814880933355596, 5.931313009212638931, 1.599625672291261402 ) ) ;
#51694=CARTESIAN_POINT ( 'NONE',  ( 3.088225128862704949, 6.824956093640315302, 0.7998128361456281477 ) ) ;
#51717=CARTESIAN_POINT ( 'NONE',  ( 5.346851039111033543, 6.199209027673978412, -2.420000000000000373 ) ) ;
#51719=CARTESIAN_POINT ( 'NONE',  ( 8.154303043976348420, 8.478051404252736845, 0.7998128361456281477 ) ) ;
#51725=CARTESIAN_POINT ( 'NONE',  ( 7.015418140428412386, 7.149352350113456822, 0.7998128361456331437 ) ) ;
#51729=CARTESIAN_POINT ( 'NONE',  ( 4.041739190649647817, 6.769093918182960579, -1.082531754730548412 ) ) ;
#51732=CARTESIAN_POINT ( 'NONE',  ( 7.349928672384119288, 8.707909884937221179, 1.082531754730549967 ) ) ;
#51741=CARTESIAN_POINT ( 'NONE',  ( 0.000000000000000000, 3.480000000000000426, -2.000000000000000000 ) ) ;
#51744=CARTESIAN_POINT ( 'NONE',  ( 6.276967689384127524, 6.888745287521969907, 0.7578909454171089966 ) ) ;
#51745=CARTESIAN_POINT ( 'NONE',  ( -6.455090533882201775, 8.624301270986276080, -1.443375672974066548 ) ) ;
#51784=CARTESIAN_POINT ( 'NONE',  ( 6.099189001301251523, 8.209082816308541197, 1.599625672291268286 ) ) ;
#51785=CARTESIAN_POINT ( 'NONE',  ( -6.265276382846530545, 6.482112999508623297, 0.000000000000000000 ) ) ;
#51786=CARTESIAN_POINT ( 'NONE',  ( 6.688968683495743583, 8.897159112202094988, -1.599625672291283607 ) ) ;
#51788=CARTESIAN_POINT ( 'NONE',  ( -7.065207446497166366, 9.336104335703744539, 0.000000000000000000 ) ) ;
#51799=CARTESIAN_POINT ( 'NONE',  ( -4.773352600463090845, 7.726605912919016106, 1.199719254218452935 ) ) ;
#51801=CARTESIAN_POINT ( 'NONE',  ( 6.170369307550815030, 8.292126506933040986, 1.443375672974064550 ) ) ;
#51816=CARTESIAN_POINT ( 'NONE',  ( -6.834718835064852449, 8.106831741398025315, 1.082531754730549078 ) ) ;
#51818=CARTESIAN_POINT ( 'NONE',  ( -4.828112100242279325, 8.646898193675708555, -0.7216878364870338292 ) ) ;
#51840=CARTESIAN_POINT ( 'NONE',  ( -3.817502770699643388, 6.611447778194983194, 1.199719254218452935 ) ) ;
#51851=CARTESIAN_POINT ( 'NONE',  ( -5.114454317065560751, 7.920171510810852133, -1.228010840421199568 ) ) ;
#51854=ORIENTED_EDGE ( 'NONE', *, *, #26150, .F. ) ;
#51868=CARTESIAN_POINT ( 'NONE',  ( 4.552505719138623341, 8.533283448962240669, 0.7998128361456341429 ) ) ;
#51889=CARTESIAN_POINT ( 'NONE',  ( 6.866278450678116485, 6.975356045404744521, 0.000000000000000000 ) ) ;
#51890=CARTESIAN_POINT ( 'NONE',  ( 4.525389411911321602, 8.501647757197021704, -0.7998128361456381397 ) ) ;
#51892=CARTESIAN_POINT ( 'NONE',  ( 4.692003678781083487, 7.631698837623355658, -1.199719254218450271 ) ) ;
#51896=CARTESIAN_POINT ( 'NONE',  ( -5.351242870924207473, 4.712735630379591534, -2.500000000000000444 ) ) ;
#51906=CARTESIAN_POINT ( 'NONE',  ( 5.880365472892705725, 7.167286867907723291, -1.140585135024022811 ) ) ;
#51907=CARTESIAN_POINT ( 'NONE',  ( -6.590672069574513792, 6.861741300691274859, 0.000000000000000000 ) ) ;
#51908=CARTESIAN_POINT ( 'NONE',  ( 4.041739190649647817, 6.769093918182960579, -1.082531754730548412 ) ) ;
#51929=CARTESIAN_POINT ( 'NONE',  ( -4.217995187182965289, 6.014356699837137832, 1.443375672974065660 ) ) ;
#51934=CARTESIAN_POINT ( 'NONE',  ( 5.332099551924443404, 9.442809587212341427, 0.000000000000000000 ) ) ;
#51943=( BOUNDED_CURVE ( )  B_SPLINE_CURVE ( 2, ( #177549, #12883, #208947 ),
 .UNSPECIFIED., .F., .T. ) 
 B_SPLINE_CURVE_WITH_KNOTS ( ( 3, 3 ),
 ( 0.000000000000000000, 0.005706871658383422079 ),
 .UNSPECIFIED. ) 
 CURVE ( )  GEOMETRIC_REPRESENTATION_ITEM ( )  RATIONAL_B_SPLINE_CURVE ( ( 1.000000000000000000, 0.9082509008696860731, 0.9421658817815319331 ) ) 
 REPRESENTATION_ITEM ( '' )  );
#51959=CARTESIAN_POINT ( 'NONE',  ( 0.000000000000000000, 1000.000000000000000, 0.000000000000000000 ) ) ;
#51963=CARTESIAN_POINT ( 'NONE',  ( 5.885121196783658526, 9.023669275293071834, 1.199719254218452047 ) ) ;
#51967=CARTESIAN_POINT ( 'NONE',  ( -5.214720930002679999, 7.727253977155453590, 1.197825571464938399 ) ) ;
#51968=CARTESIAN_POINT ( 'NONE',  ( 5.826972158823246595, 10.02016096192762085, -0.7998128361456481317 ) ) ;
#51996=CARTESIAN_POINT ( 'NONE',  ( -7.130662446144611977, 7.283804040115648526, 0.000000000000000000 ) ) ;
#51998=CARTESIAN_POINT ( 'NONE',  ( 5.525830126021535449, 8.604496359403894346, -1.199719254218452047 ) ) ;
#52019=EDGE_CURVE ( 'NONE', #155820, #97415, #101278, .T. ) ;
#52021=CARTESIAN_POINT ( 'NONE',  ( 6.831329296439236032, 9.063246493969506545, -1.599625672291267398 ) ) ;
#52030=CARTESIAN_POINT ( 'NONE',  ( 2.891631901464575272, 6.595597328342462262, 0.000000000000000000 ) ) ;
#52032=VERTEX_POINT ( 'NONE', #183221 ) ;
#52042=CARTESIAN_POINT ( 'NONE',  ( -6.644904684473536882, 6.925012684740138980, 0.7216878364870317197 ) ) ;
#52045=CARTESIAN_POINT ( 'NONE',  ( 5.468734858265785093, 7.473552982767158070, 1.599625672291269396 ) ) ;
#52048=CARTESIAN_POINT ( 'NONE',  ( -5.759181390754928742, 9.941071732514568993, 0.000000000000000000 ) ) ;
#52049=CARTESIAN_POINT ( 'NONE',  ( -4.787964524281469458, 5.614988695530339413, -1.199719254218453823 ) ) ;
#52059=DIRECTION ( 'NONE',  ( -0.6507913734559640506, -0.7592566023653003482, 0.000000000000000000 ) ) ;
#52088=CARTESIAN_POINT ( 'NONE',  ( 5.560252395380222090, 5.659585014131299552, 0.7216878364870328300 ) ) ;
#52093=CARTESIAN_POINT ( 'NONE',  ( 3.770049233051776749, 6.556085317605844232, 1.199719254218451159 ) ) ;
#52096=CARTESIAN_POINT ( 'NONE',  ( -5.635349125135588721, 6.603604063193491136, 1.199719254218452935 ) ) ;
#52099=VERTEX_POINT ( 'NONE', #53725 ) ;
#52100=CARTESIAN_POINT ( 'NONE',  ( -6.739811759324840779, 7.035737605399991601, -0.7216878364870338292 ) ) ;
#52106=CARTESIAN_POINT ( 'NONE',  ( -6.947627372360122955, 7.070263120700404968, 0.000000000000000000 ) ) ;
#52112=EDGE_LOOP ( 'NONE', ( #92291, #84604, #21276, #87130, #78659 ) ) ;
#52116=CARTESIAN_POINT ( 'NONE',  ( -5.794130544993808307, 7.853181283949808744, 1.599625672291263179 ) ) ;
#52118=CARTESIAN_POINT ( 'NONE',  ( 4.595652554671352696, 8.489339133230261680, -0.03962354257190832396 ) ) ;
#52123=CARTESIAN_POINT ( 'NONE',  ( 7.367930134383754215, 7.560616343061329125, -0.7998128361456341429 ) ) ;
#52130=CARTESIAN_POINT ( 'NONE',  ( -6.168033539574333979, 6.160736982450306876, 0.7998128361456281477 ) ) ;
#52133=CARTESIAN_POINT ( 'NONE',  ( -5.692444392891315097, 7.734547439830227411, -1.599625672291271394 ) ) ;
#52138=CARTESIAN_POINT ( 'NONE',  ( -7.553300976144787349, 8.945177572657957654, -1.082531754730549967 ) ) ;
#52144=CARTESIAN_POINT ( 'NONE',  ( 4.844006021832467646, 8.873367135438366304, 0.000000000000000000 ) ) ;
#52154=CARTESIAN_POINT ( 'NONE',  ( -4.758575512226618009, 6.703445193574907535, 1.360375859659995523 ) ) ;
#52155=CARTESIAN_POINT ( 'NONE',  ( -4.370663978927099791, 5.060324124126027279, 7.500000000000000000 ) ) ;
#52159=CARTESIAN_POINT ( 'NONE',  ( 5.991454128980707949, 7.190850779781567503, -1.201235417510186254 ) ) ;
#52188=CARTESIAN_POINT ( 'NONE',  ( -6.317530715954224441, 6.956803165068716766, 0.9171252194158643345 ) ) ;
#52207=CARTESIAN_POINT ( 'NONE',  ( -6.493429226302317225, 6.540365283632955773, 0.7998128361456341429 ) ) ;
#52217=ORIENTED_EDGE ( 'NONE', *, *, #961, .T. ) ;
#52220=CARTESIAN_POINT ( 'NONE',  ( 6.505933609711257226, 8.683618192786854095, -1.599625672291281386 ) ) ;
#52224=CARTESIAN_POINT ( 'NONE',  ( 5.465345319640213972, 8.429967735338637524, -1.082531754730548412 ) ) ;
#52238=CARTESIAN_POINT ( 'NONE',  ( -3.962726036944197894, 7.845207153068690431, -0.7998128361456481317 ) ) ;
#52239=CARTESIAN_POINT ( 'NONE',  ( 4.016958651398847557, 7.908478536599129249, -0.7998128361456362523 ) ) ;
#52248=CARTESIAN_POINT ( 'NONE',  ( -8.072954122294394352, 8.383144328957069291, -0.7998128361456362523 ) ) ;
#52249=CARTESIAN_POINT ( 'NONE',  ( 7.343676480457483002, 8.596652644402405841, -1.199719254218452047 ) ) ;
#52258=CARTESIAN_POINT ( 'NONE',  ( 5.254667053748194760, 8.288139441751686931, 1.199719254218452047 ) ) ;
#52263=CARTESIAN_POINT ( 'NONE',  ( -4.611335679197930304, 8.465601755996580380, 0.3353434889079315862 ) ) ;
#52275=CARTESIAN_POINT ( 'NONE',  ( -6.312203035614172286, 9.521931420595302953, -1.199719254218452047 ) ) ;
#52279=CARTESIAN_POINT ( 'NONE',  ( -7.005397802120316264, 5.950282834973755541, 2.500000000000000000 ) ) ;
#52284=CARTESIAN_POINT ( 'NONE',  ( 4.258669648468281110, 6.061810238003387141, 1.443375672974058777 ) ) ;
#52304=CARTESIAN_POINT ( 'NONE',  ( 5.143339171537801846, 7.093924681584510061, 1.599625672291269396 ) ) ;
#52324=CARTESIAN_POINT ( 'NONE',  ( -0.1286694677790374830, 3.477644553696438656, 1.998596537245283411 ) ) ;
#52326=CARTESIAN_POINT ( 'NONE',  ( 3.705121118284530279, 7.544668081299086282, -1.734723475976807094E-15 ) ) ;
#52327=CARTESIAN_POINT ( 'NONE',  ( -5.478903473698268023, 5.564677938835638216, -0.7216878364870338292 ) ) ;
#52330=( BOUNDED_CURVE ( )  B_SPLINE_CURVE ( 2, ( #99862, #148615, #165924, #34837, #67318, #83597, #149679 ),
 .UNSPECIFIED., .F., .T. ) 
 B_SPLINE_CURVE_WITH_KNOTS ( ( 3, 2, 2, 3 ),
 ( 0.3250000000000000666, 0.3333333333333333703, 0.3416666666666667851, 0.3500000000000000888 ),
 .UNSPECIFIED. ) 
 CURVE ( )  GEOMETRIC_REPRESENTATION_ITEM ( )  RATIONAL_B_SPLINE_CURVE ( ( 0.9999999999999991118, 0.8660254037844395958, 1.000000000000000000, 0.8660254037844387076, 1.000000000000000000, 0.8660254037844369313, 1.000000000000001776 ) ) 
 REPRESENTATION_ITEM ( '' )  );
#52354=CARTESIAN_POINT ( 'NONE',  ( -7.306918443122272677, 7.489436036589583345, 0.7998128361456341429 ) ) ;
#52360=CARTESIAN_POINT ( 'NONE',  ( -5.171509248969888617, 4.998125310078441075, 0.7998128361456281477 ) ) ;
#52368=CARTESIAN_POINT ( 'NONE',  ( -6.424584688029276514, 8.588711117491191871, 1.599625672291269396 ) ) ;
#52375=CARTESIAN_POINT ( 'NONE',  ( 5.239300017038202917, 5.077214539491492928, 0.000000000000000000 ) ) ;
#52379=CARTESIAN_POINT ( 'NONE',  ( -6.286140498591554326, 7.362860665558790707, 1.199719254218452047 ) ) ;
#52380=AXIS2_PLACEMENT_3D ( 'NONE', #84091, #115586, #150178 ) ;
#52383=CARTESIAN_POINT ( 'NONE',  ( -5.939880696562884310, 9.943961556049767836, 0.7216878364870267237 ) ) ;
#52387=CARTESIAN_POINT ( 'NONE',  ( 5.533136087708556694, 5.627949321847663278, 0.000000000000000000 ) ) ;
#52388=CARTESIAN_POINT ( 'NONE',  ( -4.380693030546956912, 6.204170850428461392, 1.443375672974065660 ) ) ;
#52402=CARTESIAN_POINT ( 'NONE',  ( 0.3562973855445230598, 2.786757976255979319, 1.969129866515958005 ) ) ;
#52407=CARTESIAN_POINT ( 'NONE',  ( 6.430738266435902517, 6.882057634903050669, 0.7203813067775278745 ) ) ;
#52415=VERTEX_POINT ( 'NONE', #80681 ) ;
#52429=CARTESIAN_POINT ( 'NONE',  ( 5.997574213172828905, 7.082153300894140635, -1.064076030282636420 ) ) ;
#52443=CARTESIAN_POINT ( 'NONE',  ( 6.230854113932139171, 9.427024345299638952, 1.199719254218452047 ) ) ;
#52446=CARTESIAN_POINT ( 'NONE',  ( -5.444481204339554736, 8.509589284108232121, 1.199719254218454489 ) ) ;
#52457=CARTESIAN_POINT ( 'NONE',  ( 4.877901405866606588, 8.912911750144889567, 0.7998128361456341429 ) ) ;
#52459=CARTESIAN_POINT ( 'NONE',  ( 6.061904079085887354, 6.244845311787889486, 0.000000000000000000 ) ) ;
#52464=CARTESIAN_POINT ( 'NONE',  ( -6.007671464186866928, 8.102312356341712984, 1.443375672974058777 ) ) ;
#52469=CARTESIAN_POINT ( 'NONE',  ( 4.434925645001613681, 5.307073019657559065, -1.082531754730548412 ) ) ;
#52481=CARTESIAN_POINT ( 'NONE',  ( -4.800995793014949165, 8.615262501910491366, 0.7216878364870267237 ) ) ;
#52482=CARTESIAN_POINT ( 'NONE',  ( 5.668717624289557833, 8.667235424096215723, -1.082531754730548412 ) ) ;
#52492=CARTESIAN_POINT ( 'NONE',  ( -4.285259070371116863, 7.157163461145040095, 1.199719254218452935 ) ) ;
#52493=CARTESIAN_POINT ( 'NONE',  ( -3.984117037569407938, 5.741498858621315371, 1.599625672291270506 ) ) ;
#52496=CARTESIAN_POINT ( 'NONE',  ( 6.061904078641523697, 7.205214525570814210, -1.082531754730548412 ) ) ;
#52500=CARTESIAN_POINT ( 'NONE',  ( -5.652456368805534481, 5.782309656923097840, 0.2304340072341204693 ) ) ;
#52507=CARTESIAN_POINT ( 'NONE',  ( -4.699286343732877569, 8.265425651823845143, 0.5948934201362279239 ) ) ;
#52511=CARTESIAN_POINT ( 'NONE',  ( -5.764847698752922689, 6.714788497190617989, 1.023463827431342343 ) ) ;
#52514=CARTESIAN_POINT ( 'NONE',  ( -5.143339171537843590, 7.093924681584509173, 1.599625672291263179 ) ) ;
#52527=CARTESIAN_POINT ( 'NONE',  ( 3.878514461961128479, 6.682628084666728085, -1.199719254218448494 ) ) ;
#52538=CARTESIAN_POINT ( 'NONE',  ( 3.098963836025306229, 6.178100804120803424, 0.8152952010215334111 ) ) ;
#52565=CARTESIAN_POINT ( 'NONE',  ( 4.746763178560250651, 7.591621904078704297, 1.082531754730549078 ) ) ;
#52571=CARTESIAN_POINT ( 'NONE',  ( 5.017926250389229459, 8.868348035513836436, 0.000000000000000000 ) ) ;
#52585=CARTESIAN_POINT ( 'NONE',  ( -5.986807348886189040, 9.142303119412650503, -1.199719254218452047 ) ) ;
#52597=CARTESIAN_POINT ( 'NONE',  ( 5.709392084686216506, 5.833581318321598985, -0.7216878364870458196 ) ) ;
#52603=CARTESIAN_POINT ( 'NONE',  ( -5.915100157312088491, 10.12297696016459092, -0.7998128361456362523 ) ) ;
#52608=CARTESIAN_POINT ( 'NONE',  ( -6.807602527837528505, 7.114826835331461652, 0.7216878364870317197 ) ) ;
#52611=CARTESIAN_POINT ( 'NONE',  ( -6.882699257592852504, 8.058845884393651460, -1.199719254218452047 ) ) ;
#52631=CARTESIAN_POINT ( 'NONE',  ( 4.726684935852882852, 4.891486930089099516, -0.8194250277325197951 ) ) ;
#52633=CARTESIAN_POINT ( 'NONE',  ( -4.136646265500958819, 7.840188053144158786, -0.7216878364870458196 ) ) ;
#52635=CARTESIAN_POINT ( 'NONE',  ( 5.306037014901791693, 7.283738832175834510, 1.599625672291269396 ) ) ;
#52636=CARTESIAN_POINT ( 'NONE',  ( -3.983063267364693960, 7.868933921892603323, -0.7998128361456481317 ) ) ;
#52637=CARTESIAN_POINT ( 'NONE',  ( -7.144220599758281054, 7.299621885998258897, 0.7998128361456341429 ) ) ;
#52644=ORIENTED_EDGE ( 'NONE', *, *, #92114, .T. ) ;
#52663=CARTESIAN_POINT ( 'NONE',  ( -7.014364370223741929, 9.276787413384745662, -1.599625672291271394 ) ) ;
#52674=AXIS2_PLACEMENT_3D ( 'NONE', #212604, #98879, #1336 ) ;
#52690=CARTESIAN_POINT ( 'NONE',  ( 4.736594563127852098, 6.619389305106191834, -1.599625672291273171 ) ) ;
#52702=CARTESIAN_POINT ( 'NONE',  ( 4.624009687016504166, 8.337032093926254106, -0.3390773965592456252 ) ) ;
#52703=ADVANCED_FACE ( 'NONE', ( #167263 ), #17771, .F. ) ;
#52706=CARTESIAN_POINT ( 'NONE',  ( 4.041212305325117882, 6.872442235258051646, -1.199719254218448494 ) ) ;
#52713=CARTESIAN_POINT ( 'NONE',  ( -6.343235766347277149, 8.493804042195527870, -1.599625672291271394 ) ) ;
#52725=CARTESIAN_POINT ( 'NONE',  ( 6.549997609177859559, 6.814287763561861944, 0.000000000000000000 ) ) ;
#52728=CARTESIAN_POINT ( 'NONE',  ( -6.099189001301292379, 8.209082816308541197, 1.599625672291263179 ) ) ;
#52739=CARTESIAN_POINT ( 'NONE',  ( 5.564695703766185275, 5.456842840674144490, 0.000000000000000000 ) ) ;
#52740=CARTESIAN_POINT ( 'NONE',  ( 6.170896192875352959, 7.228408975556602556, 1.199719254218453823 ) ) ;
#52741=ORIENTED_EDGE ( 'NONE', *, *, #142525, .T. ) ;
#52746=ORIENTED_EDGE ( 'NONE', *, *, #164497, .F. ) ;
#52761=CARTESIAN_POINT ( 'NONE',  ( 6.053423048675670159, 7.145495228771222784, -1.160209803801291795 ) ) ;
#52768=CARTESIAN_POINT ( 'NONE',  ( 5.259637247458703868, 5.100941308315409373, 0.000000000000000000 ) ) ;
#52773=CARTESIAN_POINT ( 'NONE',  ( 6.855582950365507244, 8.027210192628430718, -1.199719254218452047 ) ) ;
#52778=CARTESIAN_POINT ( 'NONE',  ( 5.614485009834906393, 6.683225611963085733, -1.082531754730548412 ) ) ;
#52782=CARTESIAN_POINT ( 'NONE',  ( 4.577813143269636065, 5.369812084349879555, -1.199719254218450271 ) ) ;
#52794=CARTESIAN_POINT ( 'NONE',  ( 6.151318917739748038, 6.974181327834800825, -0.9227930848511676221 ) ) ;
#52795=CARTESIAN_POINT ( 'NONE',  ( -7.458393901293492334, 7.874083437696761223, 0.7216878364870317197 ) ) ;
#52830=CARTESIAN_POINT ( 'NONE',  ( 5.397027666691686321, 8.454226823519094935, 1.199719254218451159 ) ) ;
#52832=CARTESIAN_POINT ( 'NONE',  ( 6.038177310039780643, 8.137902509836795417, -1.599625672291283607 ) ) ;
#52847=CARTESIAN_POINT ( 'NONE',  ( -5.123001941117347080, 7.070197912760590064, 1.599625672291263179 ) ) ;
#52850=CARTESIAN_POINT ( 'NONE',  ( 7.336370518326124746, 7.731722824234849689, -0.7216878364870317197 ) ) ;
#52861=CARTESIAN_POINT ( 'NONE',  ( -2.823841133396259639, 6.516508098929413961, -0.7998128361456481317 ) ) ;
#52867=CARTESIAN_POINT ( 'NONE',  ( -5.790741006812557323, 9.769965251341050205, 0.000000000000000000 ) ) ;
#52869=CARTESIAN_POINT ( 'NONE',  ( -4.340018570150306232, 8.077455741901736985, -0.7216878364870338292 ) ) ;
#52880=EDGE_CURVE ( 'NONE', #162079, #162324, #124398, .T. ) ;
#52891=CARTESIAN_POINT ( 'NONE',  ( -5.010620288702242853, 8.003418215864698482, -1.199719254218453823 ) ) ;
#52901=CARTESIAN_POINT ( 'NONE',  ( -4.584844773125573703, 8.498748274393685520, 0.004977730536110530624 ) ) ;
#52905=B_SPLINE_CURVE_WITH_KNOTS ( 'NONE', 3,
 ( #147415, #17370, #144262, #131219 ),
 .UNSPECIFIED., .F., .F.,
 ( 4, 4 ),
 ( 0.002022417813501748915, 0.002304360150591485551 ),
 .UNSPECIFIED. ) ;
#52917=CARTESIAN_POINT ( 'NONE',  ( 6.177789192050737732, 5.326704385421541232, 2.500000000000899281 ) ) ;
#52940=CARTESIAN_POINT ( 'NONE',  ( 4.213551878797002992, 8.137837301896977849, 0.000000000000000000 ) ) ;
#52942=CARTESIAN_POINT ( 'NONE',  ( 6.039231080244466199, 6.010467446565510130, 0.7998128361456352531 ) ) ;
#52954=CARTESIAN_POINT ( 'NONE',  ( 5.647444738788365726, 7.344714329438926548, -1.230740020431456028 ) ) ;
#52955=CIRCLE ( 'NONE', #135998, 0.08000000000000020983 ) ;
#52957=CARTESIAN_POINT ( 'NONE',  ( -5.058600711230246461, 7.955432358860325515, 1.082531754730549967 ) ) ;
#52958=CARTESIAN_POINT ( 'NONE',  ( 5.736508392357904107, 5.865217010605237924, 0.000000000000000000 ) ) ;
#52978=CARTESIAN_POINT ( 'NONE',  ( -4.136646265500958819, 7.840188053144158786, -0.7216878364870458196 ) ) ;
#52983=CARTESIAN_POINT ( 'NONE',  ( 4.830447868218803897, 8.857549289555754157, -0.7998128361456481317 ) ) ;
#53008=CARTESIAN_POINT ( 'NONE',  ( 0.4799999999999758349, 2.999999999999999112, 2.500000000000000444 ) ) ;
#53013=CARTESIAN_POINT ( 'NONE',  ( 6.343235766347262938, 8.493804042195527870, -1.599625672291281386 ) ) ;
#53023=CARTESIAN_POINT ( 'NONE',  ( -2.995508107964761191, 6.411541510041463887, -0.7147908198718248007 ) ) ;
#53040=VERTEX_POINT ( 'NONE', #155279 ) ;
#53041=CARTESIAN_POINT ( 'NONE',  ( 5.085717018901939390, 5.105960408239938353, 0.000000000000000000 ) ) ;
#53042=ORIENTED_EDGE ( 'NONE', *, *, #207178, .T. ) ;
#53049=CARTESIAN_POINT ( 'NONE',  ( 6.688968683495743583, 8.897159112202094988, -1.599625672291283607 ) ) ;
#53051=CARTESIAN_POINT ( 'NONE',  ( 4.207966135563078858, 7.175396087857926375, 7.500000000000000000 ) ) ;
#53072=CARTESIAN_POINT ( 'NONE',  ( 7.856023664475727308, 8.130058794835305136, -0.7998128361456341429 ) ) ;
#53079=ORIENTED_EDGE ( 'NONE', *, *, #18341, .F. ) ;
#53082=CARTESIAN_POINT ( 'NONE',  ( 6.373741612200160667, 9.489763409991955001, 1.082531754730549078 ) ) ;
#53096=CARTESIAN_POINT ( 'NONE',  ( -5.858531774880906262, 6.967946837850073294, 1.082531754730549078 ) ) ;
#53100=CARTESIAN_POINT ( 'NONE',  ( 6.230854113932139171, 9.427024345299638952, 1.199719254218452047 ) ) ;
#53103=CARTESIAN_POINT ( 'NONE',  ( -1.843739406749240750, 8.499999999999996447, -0.7749999999999996891 ) ) ;
#53105=CARTESIAN_POINT ( 'NONE',  ( -5.004894982100124068, 5.868074229652107121, 1.199719254218452935 ) ) ;
#53107=CARTESIAN_POINT ( 'NONE',  ( 3.953965674029162436, 7.318484642604417445, -0.9046105126420730391 ) ) ;
#53118=CYLINDRICAL_SURFACE ( 'NONE', #102730, 1.250000000000000000 ) ;
#53149=CARTESIAN_POINT ( 'NONE',  ( 4.041739190649647817, 6.769093918182960579, -1.082531754730548412 ) ) ;
#53154=CARTESIAN_POINT ( 'NONE',  ( -6.642568916052639771, 6.714361588341672515, 0.000000000000000000 ) ) ;
#53158=CARTESIAN_POINT ( 'NONE',  ( -4.797606254389363833, 6.690569611577942943, 1.599625672291263179 ) ) ;
#53159=CARTESIAN_POINT ( 'NONE',  ( -5.438755897737433287, 6.374245297895642537, -1.199719254218453823 ) ) ;
#53161=VERTEX_POINT ( 'NONE', #98819 ) ;
#53162=CARTESIAN_POINT ( 'NONE',  ( -6.007671464186866928, 8.102312356341712984, 1.443375672974058777 ) ) ;
#53169=CARTESIAN_POINT ( 'NONE',  ( -6.180537922983287302, 8.303989891604203422, -1.599625672291271394 ) ) ;
#53176=CARTESIAN_POINT ( 'NONE',  ( -1.861683537984881509, 2.483860266822599083, 2.478752606221127142 ) ) ;
#53177=CARTESIAN_POINT ( 'NONE',  ( -5.468734858265826837, 7.473552982767158070, 1.599625672291263179 ) ) ;
#53179=CARTESIAN_POINT ( 'NONE',  ( 5.184698244283005408, 7.856242361780820360, 1.254847465626233616 ) ) ;
#53184=CARTESIAN_POINT ( 'NONE',  ( 7.679767667498067496, 7.924426798361372093, 0.000000000000000000 ) ) ;
#53195=CARTESIAN_POINT ( 'NONE',  ( -7.425025402139490360, 8.691559719698066289, 1.199719254218452047 ) ) ;
#53197=ORIENTED_EDGE ( 'NONE', *, *, #212020, .T. ) ;
#53207=CARTESIAN_POINT ( 'NONE',  ( 5.397027666691686321, 8.454226823519094935, 1.199719254218451159 ) ) ;
#53221=CARTESIAN_POINT ( 'NONE',  ( -0.4000000000000114575, 2.902482508373164904, 2.023857702507793288 ) ) ;
#53222=CARTESIAN_POINT ( 'NONE',  ( 5.364607279338250656, 7.693244595681929532, -1.319704323257679057 ) ) ;
#53246=CARTESIAN_POINT ( 'NONE',  ( -5.277545713794630444, 7.647399700472480077, -1.235574677996098325 ) ) ;
#53251=CARTESIAN_POINT ( 'NONE',  ( -6.592485395868785680, 6.772832640907240354, 0.2792626473412176957 ) ) ;
#53265=LINE ( 'NONE', #205903, #73478 ) ;
#53269=CARTESIAN_POINT ( 'NONE',  ( -4.817943484809863008, 6.714296380401858499, 1.599625672291263179 ) ) ;
#53287=CARTESIAN_POINT ( 'NONE',  ( 6.441532379824158383, 9.568852638886589546, -1.082531754730548412 ) ) ;
#53302=CARTESIAN_POINT ( 'NONE',  ( -4.776215253764153346, 8.794277906025310898, -0.7998128361456362523 ) ) ;
#53304=CARTESIAN_POINT ( 'NONE',  ( 4.583538449871731757, 7.505156070562471804, 1.199719254218451159 ) ) ;
#53312=CARTESIAN_POINT ( 'NONE',  ( -7.774674742793745708, 8.035151719539642912, 0.7998128361456341429 ) ) ;
#53313=CARTESIAN_POINT ( 'NONE',  ( 6.481679955784983349, 9.719654494127929922, -1.199719254218452047 ) ) ;
#53320=CARTESIAN_POINT ( 'NONE',  ( 7.700104897918568447, 7.948153567185284096, 0.000000000000000000 ) ) ;
#53323=DIRECTION ( 'NONE',  ( 0.000000000000000000, 0.000000000000000000, 1.000000000000000000 ) ) ;
#53325=CARTESIAN_POINT ( 'NONE',  ( -4.681723370323557454, 8.380211346474826684, 0.6239904028470877329 ) ) ;
#53335=CARTESIAN_POINT ( 'NONE',  ( -3.757017964318317471, 6.436919154129725484, 1.082531754730549967 ) ) ;
#53339=CARTESIAN_POINT ( 'NONE',  ( -2.246985366954051155, 2.726529103553844813, 2.500000000000000444 ) ) ;
#53345=CARTESIAN_POINT ( 'NONE',  ( 5.397554552016228691, 5.469770863539975991, 0.7216878364870328300 ) ) ;
#53349=CARTESIAN_POINT ( 'NONE',  ( -4.936050443827081580, 7.916420063510339666, 1.199719254218452935 ) ) ;
#53359=CARTESIAN_POINT ( 'NONE',  ( 4.145001782281397595, 7.224479003952448686, 1.099888014807400616 ) ) ;
#53361=CARTESIAN_POINT ( 'NONE',  ( 4.869313445963426190, 5.709895770826003414, 1.199719254218452935 ) ) ;
#53365=CARTESIAN_POINT ( 'NONE',  ( 5.896870467300973750, 5.844380064798101237, 0.7998128361456350310 ) ) ;
#53385=CARTESIAN_POINT ( 'NONE',  ( 5.499767588998890844, 6.445425604367387429, 1.199719254218451159 ) ) ;
#53386=CARTESIAN_POINT ( 'NONE',  ( -3.675669043080673770, 7.302381293653823491, 0.000000000000000000 ) ) ;
#53406=CARTESIAN_POINT ( 'NONE',  ( -3.894033820048823813, 8.999999999999998224, -0.7749999999999979128 ) ) ;
#53409=CARTESIAN_POINT ( 'NONE',  ( -5.661411662158206681, 8.762674818229999829, -1.199719254218452047 ) ) ;
#53424=CARTESIAN_POINT ( 'NONE',  ( -7.096767062110449942, 7.244259425409119046, -0.7998128361456362523 ) ) ;
#53436=CARTESIAN_POINT ( 'NONE',  ( -6.557303570864871034, 7.679217583210999010, -1.199719254218452047 ) ) ;
#53437=TOROIDAL_SURFACE ( 'NONE', #95060, 0.8299999999999999600, 0.08000000000000000167 ) ;
#53441=CARTESIAN_POINT ( 'NONE',  ( -4.146814880933400005, 5.931313009212638931, 1.599625672291270506 ) ) ;
#53444=CARTESIAN_POINT ( 'NONE',  ( -7.892254816486440561, 8.380254505421877553, 0.000000000000000000 ) ) ;
#53445=CARTESIAN_POINT ( 'NONE',  ( 4.868786560638889149, 6.773613302202437403, 1.443375672974065660 ) ) ;
#53446=CARTESIAN_POINT ( 'NONE',  ( -4.963693635934603776, 4.963599794778024155, 0.000000000000000000 ) ) ;
#53462=CARTESIAN_POINT ( 'NONE',  ( -0.4141348083894534349, 3.002424519313423801, 1.957929617241564335 ) ) ;
#53467=CARTESIAN_POINT ( 'NONE',  ( 6.272253174914359519, 6.990222103910356921, -0.9563742486745248073 ) ) ;
#53476=VECTOR ( 'NONE', #108209, 1000.000000000000000 ) ;
#53486=CARTESIAN_POINT ( 'NONE',  ( 6.086061792568233209, 7.019478939793144967, 0.9900148145245997178 ) ) ;
#53507=CARTESIAN_POINT ( 'NONE',  ( -6.629010762438975135, 6.698543742459062145, -0.7998128361456362523 ) ) ;
#53519=CARTESIAN_POINT ( 'NONE',  ( 6.496291879603339758, 7.608037276739255006, 1.199719254218452935 ) ) ;
#53526=CARTESIAN_POINT ( 'NONE',  ( -6.685579144870156476, 9.853573864773576219, 1.082531754730549967 ) ) ;
#53527=EDGE_LOOP ( 'NONE', ( #92713, #68394, #30388, #70297 ) ) ;
#53532=CARTESIAN_POINT ( 'NONE',  ( 5.356880090730874677, 5.422317325373725794, 0.7216878364870328300 ) ) ;
#53538=CARTESIAN_POINT ( 'NONE',  ( 1.887367962963598211, 8.990012987145949097, 0.7750000000000004663 ) ) ;
#53548=CARTESIAN_POINT ( 'NONE',  ( -5.790741006812557323, 9.769965251341050205, 0.000000000000000000 ) ) ;
#53549=CARTESIAN_POINT ( 'NONE',  ( 6.048345925472183637, 8.149765894507963182, 1.443375672974065660 ) ) ;
#53555=CARTESIAN_POINT ( 'NONE',  ( -6.116136693540540570, 10.14959355252369910, 0.000000000000000000 ) ) ;
#53559=CARTESIAN_POINT ( 'NONE',  ( -5.157951095356222204, 4.982307464195829816, 0.000000000000000000 ) ) ;
#53560=CARTESIAN_POINT ( 'NONE',  ( -5.008811405605897882, 4.808311159487113073, 0.7998128361456281477 ) ) ;
#53563=CARTESIAN_POINT ( 'NONE',  ( 5.519577934094852978, 7.532869904567736974, 1.443375672974064550 ) ) ;
#53569=B_SPLINE_CURVE_WITH_KNOTS ( 'NONE', 3,
 ( #153714, #150525, #87644, #22614, #137476, #203490, #120215, #121289 ),
 .UNSPECIFIED., .F., .F.,
 ( 4, 2, 2, 4 ),
 ( 3.127317220692750373E-18, 0.003096353334791364376, 0.004644530002187043961, 0.006192706669582723547 ),
 .UNSPECIFIED. ) ;
#53575=CARTESIAN_POINT ( 'NONE',  ( -4.620365152176808543, 8.363145938788004941, -0.2588828456067792660 ) ) ;
#53583=CARTESIAN_POINT ( 'NONE',  ( -6.642568916052639771, 6.714361588341672515, 0.000000000000000000 ) ) ;
#53596=CARTESIAN_POINT ( 'NONE',  ( 5.662465432362883355, 6.635239754958710989, 1.199719254218451159 ) ) ;
#53633=CARTESIAN_POINT ( 'NONE',  ( 6.549997609177859559, 6.814287763561861944, 0.000000000000000000 ) ) ;
#53638=CARTESIAN_POINT ( 'NONE',  ( 5.194182247366861738, 9.073980031987776584, 0.7216878364870317197 ) ) ;
#53653=CARTESIAN_POINT ( 'NONE',  ( -5.447343857640614573, 9.577261277214532242, -0.7998128361456362523 ) ) ;
#53667=CARTESIAN_POINT ( 'NONE',  ( 4.380693030546913391, 7.164540064729805202, 1.082531754730549078 ) ) ;
#53672=CARTESIAN_POINT ( 'NONE',  ( -5.490125858891038213, 5.369844688319787451, -0.7998128361456362523 ) ) ;
#53677=CARTESIAN_POINT ( 'NONE',  ( -5.790741006812557323, 9.769965251341050205, 0.000000000000000000 ) ) ;
#53681=CARTESIAN_POINT ( 'NONE',  ( -6.237633190739009237, 9.434933268240943249, 1.199719254218452047 ) ) ;
#53686=CARTESIAN_POINT ( 'NONE',  ( -5.171509248969888617, 4.998125310078441075, 0.7998128361456281477 ) ) ;
#53697=CARTESIAN_POINT ( 'NONE',  ( -3.363304624641834106, 6.081549941127532222, -1.199719254218452047 ) ) ;
#53702=CARTESIAN_POINT ( 'NONE',  ( -4.719646871332968452, 5.639247783710797712, 1.082531754730549078 ) ) ;
#53704=CARTESIAN_POINT ( 'NONE',  ( -4.109529958273628658, 7.808552361378938045, 0.7216878364870338292 ) ) ;
#53705=CARTESIAN_POINT ( 'NONE',  ( 6.222266154028957885, 6.224008365980749247, 0.7998128361456352531 ) ) ;
#53706=CARTESIAN_POINT ( 'NONE',  ( -5.143339171537843590, 7.093924681584509173, 1.599625672291263179 ) ) ;
#53707=CARTESIAN_POINT ( 'NONE',  ( -6.631873415740034083, 7.766215735565355160, 1.199719254218452047 ) ) ;
#53708=VERTEX_POINT ( 'NONE', #167014 ) ;
#53715=ORIENTED_EDGE ( 'NONE', *, *, #56647, .F. ) ;
#53725=CARTESIAN_POINT ( 'NONE',  ( 4.370663978927065152, 5.060324124126029943, 1.009771797811723326 ) ) ;
#53734=CARTESIAN_POINT ( 'NONE',  ( -6.474900878978163021, 9.711745571186627402, -1.199719254218452047 ) ) ;
#53766=CARTESIAN_POINT ( 'NONE',  ( 4.817943484809818600, 6.714296380401858499, 1.599625672291269396 ) ) ;
#53782=CARTESIAN_POINT ( 'NONE',  ( 5.662465432362883355, 6.635239754958710989, 1.199719254218451159 ) ) ;
#53790=CARTESIAN_POINT ( 'NONE',  ( -5.576146316970437944, 9.727530813099326323, 0.000000000000000000 ) ) ;
#53806=CARTESIAN_POINT ( 'NONE',  ( 6.373741612200171325, 7.569024981389272710, 1.082531754730549967 ) ) ;
#53810=CARTESIAN_POINT ( 'NONE',  ( -5.773793314573309132, 7.829454515125894964, 1.599625672291263179 ) ) ;
#53816=EDGE_LOOP ( 'NONE', ( #210474, #191284, #204265, #207156 ) ) ;
#53820=CARTESIAN_POINT ( 'NONE',  ( 5.011674058906918638, 5.875983152593414971, 1.199719254218452047 ) ) ;
#53821=CARTESIAN_POINT ( 'NONE',  ( 4.037295881819344956, 7.932205305423046582, -0.7998128361456362523 ) ) ;
#53840=CARTESIAN_POINT ( 'NONE',  ( 5.300918301777743480, 7.749796750553542779, -1.302405036909856761 ) ) ;
#53848=CARTESIAN_POINT ( 'NONE',  ( 5.598591087800349086, 5.496387455380669529, -0.7998128361456481317 ) ) ;
#53853=CARTESIAN_POINT ( 'NONE',  ( 5.234329823327693809, 8.264412672927770487, 1.199719254218451159 ) ) ;
#53858=CARTESIAN_POINT ( 'NONE',  ( 4.909461021924244051, 6.821066840368686712, 1.443375672974065660 ) ) ;
#53861=CARTESIAN_POINT ( 'NONE',  ( 4.415115299905642665, 5.179997933758551554, -1.199719254218450271 ) ) ;
#53870=CARTESIAN_POINT ( 'NONE',  ( 4.207966135563082410, 7.175396087857922822, -1.043745235818753780 ) ) ;
#53873=CARTESIAN_POINT ( 'NONE',  ( 6.272547281004660746, 6.891683285556123195, -0.7655605874731727933 ) ) ;
#53874=CARTESIAN_POINT ( 'NONE',  ( -4.995253251992230581, 4.792493313604505367, 0.000000000000000000 ) ) ;
#53897=AXIS2_PLACEMENT_3D ( 'NONE', #202847, #122796, #72857 ) ;
#53898=CARTESIAN_POINT ( 'NONE',  ( -5.688757509019083614, 5.629766575900002401, -2.500000000000000444 ) ) ;
#53907=CARTESIAN_POINT ( 'NONE',  ( 7.205232291019763480, 7.370802192470005565, -0.7998128361456341429 ) ) ;
#53909=CARTESIAN_POINT ( 'NONE',  ( 6.770317605177710085, 8.992066187497757213, 1.599625672291268286 ) ) ;
#53922=CARTESIAN_POINT ( 'NONE',  ( -5.418418667316934112, 6.350518529071726981, -1.199719254218453823 ) ) ;
#53924=CARTESIAN_POINT ( 'NONE',  ( 6.658462837642799670, 7.901199744405670522, 1.082531754730549967 ) ) ;
#53935=CARTESIAN_POINT ( 'NONE',  ( -4.981695098378565945, 4.776675467721892332, -0.7998128361456362523 ) ) ;
#53938=CARTESIAN_POINT ( 'NONE',  ( -3.933273961740340496, 5.682181936820735579, 1.443375672974065660 ) ) ;
#53941=CARTESIAN_POINT ( 'NONE',  ( -4.390861645979385663, 6.216034235099629157, -1.599625672291271394 ) ) ;
#53942=ORIENTED_EDGE ( 'NONE', *, *, #64855, .F. ) ;
#53943=CARTESIAN_POINT ( 'NONE',  ( -4.489158259900630554, 8.251452046610447510, 0.000000000000000000 ) ) ;
#53966=CARTESIAN_POINT ( 'NONE',  ( -3.983063267364693960, 7.868933921892603323, -0.7998128361456481317 ) ) ;
#53977=CARTESIAN_POINT ( 'NONE',  ( -6.481153920547079395, 6.846182452143763086, -0.6414432093310319383 ) ) ;
#53979=CARTESIAN_POINT ( 'NONE',  ( 4.871153761480780275, 8.051123856976298399, 0.9350251597124116243 ) ) ;
#53990=B_SPLINE_CURVE_WITH_KNOTS ( 'NONE', 1,
 ( #168294, #166153 ),
 .UNSPECIFIED., .F., .F.,
 ( 2, 2 ),
 ( 0.000000000000000000, 0.6655069273901945692 ),
 .UNSPECIFIED. ) ;
#53991=CARTESIAN_POINT ( 'NONE',  ( 1.792484642137021078, 2.460830816602564752, 2.500000000000000444 ) ) ;
#54008=CARTESIAN_POINT ( 'NONE',  ( 5.585032934186686226, 5.480569609498057382, 0.000000000000000000 ) ) ;
#54017=CARTESIAN_POINT ( 'NONE',  ( 5.013482942003290255, 9.071090208970993274, -0.7998128361456481317 ) ) ;
#54019=CARTESIAN_POINT ( 'NONE',  ( 4.366607992053101128, 7.252070536440704096, -1.199719254218448494 ) ) ;
#54033=CARTESIAN_POINT ( 'NONE',  ( 6.229241538080760421, 6.920885192246182704, -0.8282608007674150397 ) ) ;
#54035=CARTESIAN_POINT ( 'NONE',  ( -4.760321331729590710, 8.567808963744235839, 0.7216878364870267237 ) ) ;
#54036=CARTESIAN_POINT ( 'NONE',  ( 4.909461021924231616, 8.741805268971372556, 0.7216878364870317197 ) ) ;
#54050=CARTESIAN_POINT ( 'NONE',  ( 0.1145072494591141549, 3.480000000000001315, -2.000000000000000000 ) ) ;
#54051=AXIS2_PLACEMENT_3D ( 'NONE', #122606, #109536, #172335 ) ;
#54056=CARTESIAN_POINT ( 'NONE',  ( -6.251718229232867685, 6.466295153626015590, -0.7216878364870338292 ) ) ;
#54057=DIRECTION ( 'NONE',  ( -0.7592566023653016805, 0.6507913734559627184, 0.000000000000000000 ) ) ;
#54062=CARTESIAN_POINT ( 'NONE',  ( 6.150558962454855561, 7.204682206732687000, 1.199719254218452047 ) ) ;
#54090=CARTESIAN_POINT ( 'NONE',  ( 7.666209513884374438, 7.908608952478760834, 0.7998128361456281477 ) ) ;
#54112=CIRCLE ( 'NONE', #81785, 0.07999999999999983513 ) ;
#54120=CARTESIAN_POINT ( 'NONE',  ( 4.665414256878284149, 6.536345614481700927, -1.443375672974068769 ) ) ;
#54126=CARTESIAN_POINT ( 'NONE',  ( -4.137366601288475110, 8.820714325924946309, -0.7750000000000000222 ) ) ;
#54128=CARTESIAN_POINT ( 'NONE',  ( 5.040599249230596435, 9.102725900736217568, 0.7998128361456341429 ) ) ;
#54133=CARTESIAN_POINT ( 'NONE',  ( -5.668717624289589807, 5.786127781192186958, 0.7216878364870257245 ) ) ;
#54136=CARTESIAN_POINT ( 'NONE',  ( 0.3866926556111174862, 2.897682894409570054, 2.027578619373079594 ) ) ;
#54151=CARTESIAN_POINT ( 'NONE',  ( 8.167861197590044142, 8.493869250135347215, 0.000000000000000000 ) ) ;
#54160=CARTESIAN_POINT ( 'NONE',  ( 5.858531774880875176, 9.849054480754103835, -0.7216878364870458196 ) ) ;
#54171=CARTESIAN_POINT ( 'NONE',  ( -5.072158865288277418, 7.010880990960010273, 1.443375672974058777 ) ) ;
#54173=CARTESIAN_POINT ( 'NONE',  ( 6.444921918449731280, 8.612437886315108315, 1.599625672291268286 ) ) ;
#54178=CARTESIAN_POINT ( 'NONE',  ( -6.466312919074983512, 6.508729591867735031, -0.7998128361456362523 ) ) ;
#54191=CARTESIAN_POINT ( 'NONE',  ( -3.765305043611756552, 7.354576300424668922, -0.6638232778202641793 ) ) ;
#54221=CARTESIAN_POINT ( 'NONE',  ( 3.770576118376306241, 6.452737000530752276, 1.082531754730549078 ) ) ;
#54226=CARTESIAN_POINT ( 'NONE',  ( -5.875479466675803231, 7.948088359245467416, -1.599625672291271394 ) ) ;
#54230=CARTESIAN_POINT ( 'NONE',  ( -5.123001941117347080, 7.070197912760590064, 1.599625672291263179 ) ) ;
#54231=CARTESIAN_POINT ( 'NONE',  ( -5.991777542596674166, 5.955104985976372944, 0.000000000000000000 ) ) ;
#54233=EDGE_LOOP ( 'NONE', ( #109194, #88953, #86656, #28151, #152869 ) ) ;
#54235=CARTESIAN_POINT ( 'NONE',  ( -5.112833325684904118, 8.979072956692109031, -0.7216878364870338292 ) ) ;
#54240=ORIENTED_EDGE ( 'NONE', *, *, #56647, .T. ) ;
#54241=CARTESIAN_POINT ( 'NONE',  ( -4.516801452008150086, 5.298631777878131111, 1.199719254218452935 ) ) ;
#54250=CARTESIAN_POINT ( 'NONE',  ( -6.095272577795516789, 9.268845886473535245, 1.199719254218452047 ) ) ;
#54252=CARTESIAN_POINT ( 'NONE',  ( 4.636584873806110174, 8.438537862545894441, 0.4145994950837776916 ) ) ;
#54255=CARTESIAN_POINT ( 'NONE',  ( 4.542476715900265916, 4.951051008190067826, -0.8264431066547142102 ) ) ;
#54257=CARTESIAN_POINT ( 'NONE',  ( 3.464990776744291345, 6.200183785247111778, 1.199719254218452047 ) ) ;
#54268=CARTESIAN_POINT ( 'NONE',  ( -6.994027139803241866, 9.253060644560830994, -1.599625672291271394 ) ) ;
#54281=CARTESIAN_POINT ( 'NONE',  ( 6.017840079619279692, 8.114175741012878973, -1.599625672291281386 ) ) ;
#54295=CARTESIAN_POINT ( 'NONE',  ( 6.083581728852979431, 7.123651168416324175, -1.137916992902558100 ) ) ;
#54322=CARTESIAN_POINT ( 'NONE',  ( -6.329738897986983304, 6.948428204275519882, 0.9008771187248975076 ) ) ;
#54344=CARTESIAN_POINT ( 'NONE',  ( -6.466312919074983512, 6.508729591867735031, -0.7998128361456362523 ) ) ;
#54378=CARTESIAN_POINT ( 'NONE',  ( 4.681308178468477799, 8.683552984847038303, 0.000000000000000000 ) ) ;
#54388=CARTESIAN_POINT ( 'NONE',  ( -4.950662367645459305, 5.804802846121667415, -1.199719254218453823 ) ) ;
#54389=CARTESIAN_POINT ( 'NONE',  ( 8.167861197590044142, 8.493869250135347215, 0.000000000000000000 ) ) ;
#54396=CARTESIAN_POINT ( 'NONE',  ( 6.176621499477501054, 9.363752961769195693, -1.199719254218452047 ) ) ;
#54402=CARTESIAN_POINT ( 'NONE',  ( -5.289925464687482481, 7.757115612407050165, 1.311310741419260628 ) ) ;
#54411=CARTESIAN_POINT ( 'NONE',  ( -4.299344108864953995, 7.069632989434141201, -1.082531754730551743 ) ) ;
#54420=CARTESIAN_POINT ( 'NONE',  ( 3.445180431648313224, 7.033477913649446300, 0.7216878364870257245 ) ) ;
#54425=CARTESIAN_POINT ( 'NONE',  ( -5.692444392891315097, 7.734547439830227411, -1.599625672291271394 ) ) ;
#54438=CARTESIAN_POINT ( 'NONE',  ( 5.435893244436359240, 5.306573304789342416, -0.7998128361456481317 ) ) ;
#54442=CARTESIAN_POINT ( 'NONE',  ( -4.908225742414364490, 4.881379242517357220, -0.5727826874471857455 ) ) ;
#54463=CARTESIAN_POINT ( 'NONE',  ( -3.838366886444665393, 7.492195444245147939, 0.000000000000000000 ) ) ;
#54486=CARTESIAN_POINT ( 'NONE',  ( -5.824109505522200081, 8.952488968821326054, -1.199719254218452047 ) ) ;
#54488=CARTESIAN_POINT ( 'NONE',  ( 5.831415467209187575, 9.817418788470464008, 0.000000000000000000 ) ) ;
#54500=CARTESIAN_POINT ( 'NONE',  ( -6.563028877466991595, 9.814561569423593923, 1.199719254218452935 ) ) ;
#54511=CARTESIAN_POINT ( 'NONE',  ( -5.936491157937300756, 8.019268665717216749, 1.599625672291263179 ) ) ;
#54515=CARTESIAN_POINT ( 'NONE',  ( -4.659162064951642535, 5.464719159645540003, 1.199719254218452935 ) ) ;
#54519=CARTESIAN_POINT ( 'NONE',  ( 5.383996397958233260, 5.453953017138946535, -0.7216878364870458196 ) ) ;
#54520=CARTESIAN_POINT ( 'NONE',  ( -6.441532379824190357, 6.687744995982559892, 0.7216878364870257245 ) ) ;
#54522=ORIENTED_EDGE ( 'NONE', *, *, #152126, .T. ) ;
#54525=CARTESIAN_POINT ( 'NONE',  ( -6.283277845290492714, 6.295188672452495915, -0.7998128361456361413 ) ) ;
#54528=CARTESIAN_POINT ( 'NONE',  ( 4.913904330310220558, 4.697586238308844919, 0.000000000000000000 ) ) ;
#54538=CARTESIAN_POINT ( 'NONE',  ( 4.966250736084032447, 8.070317005903060448, 1.090833899539983554 ) ) ;
#54548=CARTESIAN_POINT ( 'NONE',  ( 6.170896192875352959, 7.228408975556602556, 1.199719254218453823 ) ) ;
#54559=CARTESIAN_POINT ( 'NONE',  ( 5.417061852544872380, 7.532864896096530316, 1.248242807326222392 ) ) ;
#54573=CARTESIAN_POINT ( 'NONE',  ( 3.982994815507484354, 7.308283119008860851, -0.9368446653362592080 ) ) ;
#54576=CARTESIAN_POINT ( 'NONE',  ( -5.794130544993808307, 7.853181283949808744, 1.599625672291263179 ) ) ;
#54584=ADVANCED_FACE ( 'NONE', ( #123682 ), #187121, .T. ) ;
#54590=CARTESIAN_POINT ( 'NONE',  ( 6.561219994370630637, 6.619454513046008515, 0.000000000000000000 ) ) ;
#54592=CARTESIAN_POINT ( 'NONE',  ( 6.535912570239620578, 9.782925877658371405, 1.199719254218452047 ) ) ;
#54597=CARTESIAN_POINT ( 'NONE',  ( -7.905812970100109638, 8.396072351304486148, 0.7216878364870317197 ) ) ;
#54601=CARTESIAN_POINT ( 'NONE',  ( 3.241808126998965811, 6.796210224891872542, 0.7216878364870257245 ) ) ;
#54607=CARTESIAN_POINT ( 'NONE',  ( 1.860351378971565550, 8.967085675740335660, 0.7750000000000004663 ) ) ;
#54612=ORIENTED_EDGE ( 'NONE', *, *, #17110, .T. ) ;
#54615=CARTESIAN_POINT ( 'NONE',  ( -6.563555762791521531, 9.711213252348503744, 1.082531754730549967 ) ) ;
#54616=CARTESIAN_POINT ( 'NONE',  ( 5.370438244788902971, 9.279612028980123384, -0.7216878364870458196 ) ) ;
#54625=ORIENTED_EDGE ( 'NONE', *, *, #135323, .F. ) ;
#54626=CARTESIAN_POINT ( 'NONE',  ( -4.447956913735107598, 7.346977611736363656, 1.199719254218452935 ) ) ;
#54627=CARTESIAN_POINT ( 'NONE',  ( -7.431277594066152403, 8.802816960232885179, -1.082531754730549967 ) ) ;
#54629=CARTESIAN_POINT ( 'NONE',  ( 4.855228407025239612, 8.678533884922511987, 0.000000000000000000 ) ) ;
#54641=CARTESIAN_POINT ( 'NONE',  ( -4.606260857482554982, 8.381206713624141713, 0.1075878075270080697 ) ) ;
#54649=CARTESIAN_POINT ( 'NONE',  ( -4.606738333593328072, 8.596554832492683929, 0.7998128361456281477 ) ) ;
#54662=CARTESIAN_POINT ( 'NONE',  ( 4.420840606507738357, 7.315341919971147355, 1.199719254218451159 ) ) ;
#54680=AXIS2_PLACEMENT_3D ( 'NONE', #92884, #207664, #158929 ) ;
#54699=CARTESIAN_POINT ( 'NONE',  ( 4.556949027968946631, 8.330541276023501140, -0.7216878364870357165 ) ) ;
#54704=DIRECTION ( 'NONE',  ( 0.000000000000000000, 0.000000000000000000, -1.000000000000000000 ) ) ;
#54705=CARTESIAN_POINT ( 'NONE',  ( 4.868786560638878491, 8.694351730805124134, 0.7216878364870317197 ) ) ;
#54720=CARTESIAN_POINT ( 'NONE',  ( -7.445362632559989535, 8.715286488521982733, 1.199719254218452047 ) ) ;
#54722=CARTESIAN_POINT ( 'NONE',  ( -6.563028877466991595, 9.814561569423593923, 1.199719254218452935 ) ) ;
#54731=CARTESIAN_POINT ( 'NONE',  ( 4.217995187182922656, 6.014356699837137832, 1.443375672974058777 ) ) ;
#54738=CARTESIAN_POINT ( 'NONE',  ( -2.993318053567081360, 6.714231172462041819, 0.000000000000000000 ) ) ;
#54743=CARTESIAN_POINT ( 'NONE',  ( -5.804299160426224624, 9.785783097223662352, -0.7216878364870338292 ) ) ;
#54746=CARTESIAN_POINT ( 'NONE',  ( -7.611976899429754084, 7.845337568948314022, 0.7998128361456341429 ) ) ;
#54751=CARTESIAN_POINT ( 'NONE',  ( -4.146814880933400005, 5.931313009212638931, 1.599625672291270506 ) ) ;
#54761=CARTESIAN_POINT ( 'NONE',  ( -2.959422669532919326, 6.674686557755516780, 0.7998128361456352531 ) ) ;
#54767=CARTESIAN_POINT ( 'NONE',  ( -4.285785955695645910, 7.053815144069948140, 1.082531754730549967 ) ) ;
#54769=CARTESIAN_POINT ( 'NONE',  ( -3.472296738431328134, 7.065113604896248845, 0.000000000000000000 ) ) ;
#54772=CARTESIAN_POINT ( 'NONE',  ( 3.874598038455354665, 7.742391154831717692, -0.7998128361456362523 ) ) ;
#54773=CARTESIAN_POINT ( 'NONE',  ( -5.173318132066234476, 8.193232366456022930, -1.199719254218453823 ) ) ;
#54774=CARTESIAN_POINT ( 'NONE',  ( -5.769876891067536206, 8.889217585290882795, 1.199719254218454489 ) ) ;
#54775=CARTESIAN_POINT ( 'NONE',  ( -6.645678883216806554, 6.734777780655774038, 0.1184763017797350326 ) ) ;
#54817=AXIS2_PLACEMENT_3D ( 'NONE', #68333, #146445, #81412 ) ;
#54823=CARTESIAN_POINT ( 'NONE',  ( -1.905110947044342140, 8.996536036952683446, -0.7749999999999996891 ) ) ;
#54825=CARTESIAN_POINT ( 'NONE',  ( 6.343417644170677328, 6.506394916557118435, -2.500000000000000444 ) ) ;
#54833=CARTESIAN_POINT ( 'NONE',  ( 3.888156192069020634, 7.758209000714329839, 1.040834085586084257E-14 ) ) ;
#54834=CARTESIAN_POINT ( 'NONE',  ( 5.346851039111029991, 6.199209027673978412, 7.500000000000000000 ) ) ;
#54835=CARTESIAN_POINT ( 'NONE',  ( 7.013428937081407355, 5.939655416065874327, -2.436399677959149468 ) ) ;
#54850=CARTESIAN_POINT ( 'NONE',  ( 3.691562964670865199, 7.528850235416478576, -0.7998128361456362523 ) ) ;
#54855=CARTESIAN_POINT ( 'NONE',  ( -5.562588163356775972, 9.711712967216715953, 0.7998128361456291469 ) ) ;
#54860=CARTESIAN_POINT ( 'NONE',  ( 4.875038752565570732, 7.845239757038595663, -1.199719254218452047 ) ) ;
#54870=CARTESIAN_POINT ( 'NONE',  ( 6.536439455564150514, 9.679577560583279450, 1.082531754730549078 ) ) ;
#54873=CARTESIAN_POINT ( 'NONE',  ( -3.201133666602369310, 6.748756687762456963, -0.7216878364870458196 ) ) ;
#54874=CARTESIAN_POINT ( 'NONE',  ( -5.855142236255304944, 7.924361590421551860, -1.599625672291271394 ) ) ;
#54884=CARTESIAN_POINT ( 'NONE',  ( 3.553118775233146120, 6.302999783484076524, -1.199719254218453823 ) ) ;
#54885=CARTESIAN_POINT ( 'NONE',  ( 4.227110032410640095, 8.153655147779589996, 0.7998128361456271485 ) ) ;
#54891=ORIENTED_EDGE ( 'NONE', *, *, #34539, .T. ) ;
#54903=CARTESIAN_POINT ( 'NONE',  ( 4.960800185296459830, 8.075801985472857325, -1.085925974634168290 ) ) ;
#54905=ORIENTED_EDGE ( 'NONE', *, *, #77903, .F. ) ;
#54907=VECTOR ( 'NONE', #173947, 1000.000000000000000 ) ;
#54912=CARTESIAN_POINT ( 'NONE',  ( 5.234856708652227297, 7.200695141551334721, 1.443375672974065660 ) ) ;
#54914=CARTESIAN_POINT ( 'NONE',  ( 4.923546060418115822, 5.773167154356443120, -1.199719254218452047 ) ) ;
#54918=CARTESIAN_POINT ( 'NONE',  ( 7.289443866002793371, 8.533381260871966134, 1.199719254218452047 ) ) ;
#54923=CARTESIAN_POINT ( 'NONE',  ( 5.397554552016212703, 8.350878506444006533, 1.082531754730547524 ) ) ;
#54925=CARTESIAN_POINT ( 'NONE',  ( -4.132202957115018727, 8.042930226601317401, 0.000000000000000000 ) ) ;
#54927=CARTESIAN_POINT ( 'NONE',  ( 3.607351389687783794, 6.366271167014519783, 1.199719254218451159 ) ) ;
#54938=CARTESIAN_POINT ( 'NONE',  ( 6.011645680221167076, 7.072102904328817274, -1.053258377668888857 ) ) ;
#54939=CARTESIAN_POINT ( 'NONE',  ( -3.851398154733808088, 6.650992392901508232, -1.199719254218450271 ) ) ;
#54975=CARTESIAN_POINT ( 'NONE',  ( 5.830888582329017744, 8.960397891762626799, -1.199719254218452047 ) ) ;
#54977=CARTESIAN_POINT ( 'NONE',  ( 5.742760583840166966, 8.857581893525663830, 1.199719254218452047 ) ) ;
#54991=CARTESIAN_POINT ( 'NONE',  ( -3.962726036944197894, 7.845207153068690431, -0.7998128361456481317 ) ) ;
#54993=CARTESIAN_POINT ( 'NONE',  ( 5.343321937117211817, 9.247976336696488886, 0.000000000000000000 ) ) ;
#55003=CARTESIAN_POINT ( 'NONE',  ( -5.659602779061863487, 5.567567761852417085, 0.7998128361456281477 ) ) ;
#55007=CARTESIAN_POINT ( 'NONE',  ( -4.340018570150322219, 5.196348098997705556, -1.082531754730551743 ) ) ;
#55011=CARTESIAN_POINT ( 'NONE',  ( -3.902768115887413014, 5.646591783325653147, -1.599625672291283607 ) ) ;
#55020=CARTESIAN_POINT ( 'NONE',  ( -0.04359940615404794828, 3.409091168011650463, 2.082493747991086330 ) ) ;
#55035=CARTESIAN_POINT ( 'NONE',  ( -6.089547271193396227, 7.133501900260939443, -1.199719254218453823 ) ) ;
#55045=CARTESIAN_POINT ( 'NONE',  ( -6.597731880524014159, 6.769412454161013670, -0.2479414380717175903 ) ) ;
#55059=CARTESIAN_POINT ( 'NONE',  ( 4.053528829375365738, 3.783736749027409196, 2.445701138906706706 ) ) ;
#55062=CIRCLE ( 'NONE', #144930, 0.7499999999999997780 ) ;
#55066=CARTESIAN_POINT ( 'NONE',  ( 7.363486825553451354, 8.723727730301414240, -1.082531754730548412 ) ) ;
#55071=CARTESIAN_POINT ( 'NONE',  ( 1.919948509414024951, 8.999999999999998224, -0.7749999999999996891 ) ) ;
#55075=DIRECTION ( 'NONE',  ( -1.000000000000000000, 0.000000000000000000, 0.000000000000000000 ) ) ;
#55079=CARTESIAN_POINT ( 'NONE',  ( 4.061549535745618833, 6.896169004081968090, -1.199719254218452047 ) ) ;
#55087=CARTESIAN_POINT ( 'NONE',  ( 7.049313524462606395, 7.188896964819984525, 0.000000000000000000 ) ) ;
#55089=CARTESIAN_POINT ( 'NONE',  ( 6.475954649182838807, 7.584310507915338562, 1.199719254218452047 ) ) ;
#55102=CARTESIAN_POINT ( 'NONE',  ( 6.465908158583062892, 6.764574590967027845, 0.2795716154820517829 ) ) ;
#55104=CARTESIAN_POINT ( 'NONE',  ( 4.407809338218622308, 8.156544971314787063, 0.000000000000000000 ) ) ;
#55123=CARTESIAN_POINT ( 'NONE',  ( -5.356880090730904875, 7.343055753976412525, 1.443375672974058777 ) ) ;
#55128=CARTESIAN_POINT ( 'NONE',  ( 5.006703865196457492, 9.063181286029688977, 0.000000000000000000 ) ) ;
#55175=FACE_OUTER_BOUND ( 'NONE', #104521, .T. ) ;
#55185=CARTESIAN_POINT ( 'NONE',  ( 5.587368702607580673, 5.691220705896524734, -0.7216878364870458196 ) ) ;
#55193=CARTESIAN_POINT ( 'NONE',  ( 5.203297092594585393, 9.292540051327542017, 0.7998128361456341429 ) ) ;
#55196=CARTESIAN_POINT ( 'NONE',  ( -4.828112100242294424, 5.765790550771681566, -1.082531754730549967 ) ) ;
#55206=CARTESIAN_POINT ( 'NONE',  ( -0.1216878429548682999, 3.463015919485879834, -1.996294584693599994 ) ) ;
#55218=CARTESIAN_POINT ( 'NONE',  ( 7.126746022638799971, 8.343567110280638133, 1.199719254218452047 ) ) ;
#55227=CARTESIAN_POINT ( 'NONE',  ( 3.390420931869152721, 6.113185632892752075, -1.199719254218452047 ) ) ;
#55240=CARTESIAN_POINT ( 'NONE',  ( -4.665414256878287702, 8.457084043084382330, -0.7216878364870338292 ) ) ;
#55243=CARTESIAN_POINT ( 'NONE',  ( 7.550965208168244125, 7.774157262476569130, -0.7998128361456341429 ) ) ;
#55248=CARTESIAN_POINT ( 'NONE',  ( -5.842637852846353397, 5.781108681267656202, 0.7998128361456281477 ) ) ;
#55251=EDGE_CURVE ( 'NONE', #201520, #108645, #124635, .T. ) ;
#55264=CARTESIAN_POINT ( 'NONE',  ( 1.886825320689233809, 2.480000000000016858, 2.459652456995882641 ) ) ;
#55265=FACE_OUTER_BOUND ( 'NONE', #128906, .T. ) ;
#55287=CARTESIAN_POINT ( 'NONE',  ( 4.095971805104285934, 6.832365301713403838, 1.082531754730549078 ) ) ;
#55291=CARTESIAN_POINT ( 'NONE',  ( -7.293360289508603600, 7.473618190706972086, 0.000000000000000000 ) ) ;
#55295=CARTESIAN_POINT ( 'NONE',  ( -3.637330350216213759, 7.465578851886037093, -0.7998128361456481317 ) ) ;
#55300=CARTESIAN_POINT ( 'NONE',  ( -7.905812970100109638, 8.396072351304486148, 0.7216878364870317197 ) ) ;
#55307=CARTESIAN_POINT ( 'NONE',  ( -5.327428015527048366, 5.180030537728460338, -0.7998128361456362523 ) ) ;
#55315=CARTESIAN_POINT ( 'NONE',  ( -8.120407659942227241, 8.438506789546210030, 0.7998128361456341429 ) ) ;
#55316=CARTESIAN_POINT ( 'NONE',  ( 4.708029738644283313, 8.352945002179891887, -0.6661931671527853149 ) ) ;
#55321=CARTESIAN_POINT ( 'NONE',  ( 3.061108821635398769, 6.793320401875094561, -0.7998128361456362523 ) ) ;
#55331=CARTESIAN_POINT ( 'NONE',  ( -7.045397100956844127, 8.248660034984974132, -1.199719254218452047 ) ) ;
#55342=CARTESIAN_POINT ( 'NONE',  ( 5.083381250481017410, 4.895309311841474553, 0.7998128361456352531 ) ) ;
#55355=CARTESIAN_POINT ( 'NONE',  ( 0.1443076407905200254, 2.614873645970688276, 2.074999080605917090 ) ) ;
#55356=CARTESIAN_POINT ( 'NONE',  ( 5.720439131930858956, 7.397432110343761025, 1.315134405782365956 ) ) ;
#55383=CARTESIAN_POINT ( 'NONE',  ( -6.212075186202199006, 7.030024481103895440, 1.038766164041710738 ) ) ;
#55401=CARTESIAN_POINT ( 'NONE',  ( -5.498713818794216834, 8.572860667638675380, -1.199719254218452047 ) ) ;
#55416=ORIENTED_EDGE ( 'NONE', *, *, #68201, .T. ) ;
#55418=CARTESIAN_POINT ( 'NONE',  ( 2.911969131885072670, 6.619324097166378706, 0.000000000000000000 ) ) ;
#55428=CARTESIAN_POINT ( 'NONE',  ( 4.668873160992260019, 8.281730553837055808, 0.5279080060728712498 ) ) ;
#55436=CARTESIAN_POINT ( 'NONE',  ( 6.150558962454855561, 7.204682206732687000, 1.199719254218452047 ) ) ;
#55446=CARTESIAN_POINT ( 'NONE',  ( -4.899292406491858820, 6.809203455697518947, -1.599625672291271394 ) ) ;
#55448=CARTESIAN_POINT ( 'NONE',  ( 3.088225128862704949, 6.824956093640315302, 0.7998128361456281477 ) ) ;
#55452=CARTESIAN_POINT ( 'NONE',  ( -6.017840079619296567, 8.114175741012878973, -1.599625672291271394 ) ) ;
#55455=CARTESIAN_POINT ( 'NONE',  ( 7.361151057576892143, 7.552707420120024828, 0.7998128361456291469 ) ) ;
#55460=CARTESIAN_POINT ( 'NONE',  ( -5.151759543144467379, 7.884679950488731492, 1.249873765817657079 ) ) ;
#55469=CARTESIAN_POINT ( 'NONE',  ( -4.136646265500958819, 7.840188053144158786, -0.7216878364870458196 ) ) ;
#55481=CARTESIAN_POINT ( 'NONE',  ( 5.587368702607580673, 5.691220705896524734, -0.7216878364870458196 ) ) ;
#55485=CARTESIAN_POINT ( 'NONE',  ( -6.237633190739009237, 9.434933268240943249, 1.199719254218452047 ) ) ;
#55499=CARTESIAN_POINT ( 'NONE',  ( 5.259637247458703868, 5.100941308315409373, 0.000000000000000000 ) ) ;
#55504=DIRECTION ( 'NONE',  ( 0.9667316390278627436, -0.2557927639760400607, 0.000000000000000000 ) ) ;
#55526=CARTESIAN_POINT ( 'NONE',  ( -4.773879485787619892, 7.623257595843924150, 1.082531754730549967 ) ) ;
#55553=CARTESIAN_POINT ( 'NONE',  ( -3.811250578772981346, 6.500190537660166079, -1.082531754730546636 ) ) ;
#55559=CARTESIAN_POINT ( 'NONE',  ( -4.447956913735107598, 7.346977611736363656, 1.199719254218452935 ) ) ;
#55567=CARTESIAN_POINT ( 'NONE',  ( -4.411198876399886615, 6.239761003923544713, -1.599625672291271394 ) ) ;
#55569=CARTESIAN_POINT ( 'NONE',  ( 5.316739912341137853, 7.735632174496787528, -1.307268462668280673 ) ) ;
#55573=CARTESIAN_POINT ( 'NONE',  ( 3.867818961648523235, 7.734482231890414283, 1.040834085586084257E-14 ) ) ;
#55577=CARTESIAN_POINT ( 'NONE',  ( -5.641074431737709283, 8.738948049406083385, -1.199719254218452047 ) ) ;
#55581=CARTESIAN_POINT ( 'NONE',  ( -5.334207092333882017, 5.187939460669764635, 0.7998128361456281477 ) ) ;
#55584=CARTESIAN_POINT ( 'NONE',  ( -7.444835747235459600, 8.818634805597074688, 1.082531754730549078 ) ) ;
#55585=CARTESIAN_POINT ( 'NONE',  ( 4.543390873910906791, 6.393985001019784953, 1.443375672974065660 ) ) ;
#55586=CARTESIAN_POINT ( 'NONE',  ( -4.109529958273628658, 7.808552361378938045, 0.7216878364870338292 ) ) ;
#55592=CARTESIAN_POINT ( 'NONE',  ( 4.146814880933355596, 5.931313009212638931, 1.599625672291261402 ) ) ;
#55597=CARTESIAN_POINT ( 'NONE',  ( 5.912764389335556814, 6.070849007079178072, -0.7216878364870512597 ) ) ;
#55599=CARTESIAN_POINT ( 'NONE',  ( 5.391302360089590628, 6.318882837306503575, -1.199719254218452047 ) ) ;
#55604=CARTESIAN_POINT ( 'NONE',  ( 5.568688238291347403, 7.519645578322940338, 1.337618216391135428 ) ) ;
#55613=CARTESIAN_POINT ( 'NONE',  ( 5.365994935958575240, 9.482354201918870018, 0.7998128361456341429 ) ) ;
#55623=CARTESIAN_POINT ( 'NONE',  ( 6.198956711081595294, 6.941498593865138567, 0.8670033951987624610 ) ) ;
#55639=CARTESIAN_POINT ( 'NONE',  ( -4.945692173934974178, 8.992000979557944973, 0.000000000000000000 ) ) ;
#55643=DIRECTION ( 'NONE',  ( -1.000000000000000000, 0.000000000000000000, 0.000000000000000000 ) ) ;
#55644=CYLINDRICAL_SURFACE ( 'NONE', #66941, 1.250000000000000000 ) ;
#55653=CARTESIAN_POINT ( 'NONE',  ( 4.875038752565570732, 7.845239757038595663, -1.199719254218452047 ) ) ;
#55659=CARTESIAN_POINT ( 'NONE',  ( -6.360183458142173230, 9.473945563590925545, 1.082531754730549967 ) ) ;
#55660=ORIENTED_EDGE ( 'NONE', *, *, #31289, .T. ) ;
#55663=CARTESIAN_POINT ( 'NONE',  ( 5.194182247366881278, 5.232503174782402233, 0.7216878364870328300 ) ) ;
#55665=EDGE_CURVE ( 'NONE', #114168, #127442, #150243, .T. ) ;
#55677=CARTESIAN_POINT ( 'NONE',  ( -2.959422669532919326, 6.674686557755516780, 0.7998128361456352531 ) ) ;
#55678=CARTESIAN_POINT ( 'NONE',  ( 5.343321937561575474, 8.287607122913563273, -1.082531754730548412 ) ) ;
#55689=CARTESIAN_POINT ( 'NONE',  ( -4.423703259808839938, 8.383013913077441259, 0.7998128361456352531 ) ) ;
#55690=CARTESIAN_POINT ( 'NONE',  ( -5.966997003790217136, 9.975597247814986801, -0.7216878364870338292 ) ) ;
#55693=CARTESIAN_POINT ( 'NONE',  ( 6.658462837642799670, 7.901199744405670522, 1.082531754730549967 ) ) ;
#55700=FACE_OUTER_BOUND ( 'NONE', #13591, .T. ) ;
#55706=CARTESIAN_POINT ( 'NONE',  ( -4.662190612263335865, 8.310640895677696705, -0.4745246276153299858 ) ) ;
#55711=CARTESIAN_POINT ( 'NONE',  ( 3.770576118376296471, 7.413106214832098750, 0.7216878364870257245 ) ) ;
#55715=CARTESIAN_POINT ( 'NONE',  ( -4.769436176957319695, 8.786368983084006601, 0.7998128361456281477 ) ) ;
#55727=CARTESIAN_POINT ( 'NONE',  ( 5.903649544107831382, 5.852288987739402870, -0.7998128361456481317 ) ) ;
#55744=CARTESIAN_POINT ( 'NONE',  ( 3.006787879153326681, 6.373552747333731006, -0.4818892653130519843 ) ) ;
#55748=CARTESIAN_POINT ( 'NONE',  ( 0.3999999999999758193, 3.000000000000047518, 2.023857702507768419 ) ) ;
#55764=CARTESIAN_POINT ( 'NONE',  ( 5.221298555038576872, 9.105615724271411082, 0.000000000000000000 ) ) ;
#55769=CARTESIAN_POINT ( 'NONE',  ( 7.363486825553451354, 8.723727730301414240, -1.082531754730548412 ) ) ;
#55784=CARTESIAN_POINT ( 'NONE',  ( -7.944151662964566540, 8.232874793072271657, 0.000000000000000000 ) ) ;
#55797=CARTESIAN_POINT ( 'NONE',  ( 5.045042557616584489, 5.058506870073687267, 0.000000000000000000 ) ) ;
#55804=CARTESIAN_POINT ( 'NONE',  ( -4.516801452008150086, 5.298631777878131111, 1.199719254218452935 ) ) ;
#55809=CARTESIAN_POINT ( 'NONE',  ( -5.628043163448566588, 9.580151100749725757, 0.000000000000000000 ) ) ;
#55812=CARTESIAN_POINT ( 'NONE',  ( -5.399890319992785237, 9.521898816625391504, 0.7998128361456291469 ) ) ;
#55817=CARTESIAN_POINT ( 'NONE',  ( -5.659602779061863487, 5.567567761852417085, 0.7998128361456281477 ) ) ;
#55832=CARTESIAN_POINT ( 'NONE',  ( -3.851925040058333582, 7.508013290127760087, -0.7216878364870458196 ) ) ;
#55833=ORIENTED_EDGE ( 'NONE', *, *, #18887, .F. ) ;
#55834=CARTESIAN_POINT ( 'NONE',  ( -4.787437638956935082, 6.678706226906775179, -1.443375672974066548 ) ) ;
#55836=CARTESIAN_POINT ( 'NONE',  ( 5.143339171537801846, 7.093924681584509173, 1.599625672291269396 ) ) ;
#55837=CARTESIAN_POINT ( 'NONE',  ( -6.143779885648060102, 7.196773283791382703, 1.199719254218452047 ) ) ;
#55838=CARTESIAN_POINT ( 'NONE',  ( -7.065734331377342414, 8.272386803808890576, -1.199719254218452047 ) ) ;
#55839=CARTESIAN_POINT ( 'NONE',  ( -6.337068562759858636, 6.936200024879327408, -0.9492287992594623525 ) ) ;
#55850=ORIENTED_EDGE ( 'NONE', *, *, #131846, .F. ) ;
#55857=CARTESIAN_POINT ( 'NONE',  ( 5.027041095616958444, 9.086908054853605421, 0.000000000000000000 ) ) ;
#55862=CARTESIAN_POINT ( 'NONE',  ( -2.974142338115852269, 6.685868392857900133, 0.1038623869373533903 ) ) ;
#55879=CARTESIAN_POINT ( 'NONE',  ( 6.343235766347262938, 8.493804042195527870, -1.599625672291281386 ) ) ;
#55884=CARTESIAN_POINT ( 'NONE',  ( 5.066970889784239596, 4.909229436870949925, 0.2438227144904350496 ) ) ;
#55885=CARTESIAN_POINT ( 'NONE',  ( -1.930226670627066099, 8.999999999999998224, -0.7749999999999996891 ) ) ;
#55887=CARTESIAN_POINT ( 'NONE',  ( 2.987253516826691158, 6.445425535883942736, -0.5244392418292821434 ) ) ;
#55895=CARTESIAN_POINT ( 'NONE',  ( 4.386945222473598527, 7.275797305264619652, -1.199719254218452047 ) ) ;
#55898=CARTESIAN_POINT ( 'NONE',  ( 4.370663978927065152, 5.060324124126027279, 2.420000000000000373 ) ) ;
#55912=CARTESIAN_POINT ( 'NONE',  ( 5.903649544107831382, 5.852288987739402870, -0.7998128361456481317 ) ) ;
#55917=EDGE_LOOP ( 'NONE', ( #26101, #203870, #112865 ) ) ;
#55919=CARTESIAN_POINT ( 'NONE',  ( -7.910256278930404505, 8.193330178365746619, -0.7998128361456362523 ) ) ;
#55925=CARTESIAN_POINT ( 'NONE',  ( 4.603875680292229156, 7.528882839386387360, 1.199719254218452047 ) ) ;
#55939=CARTESIAN_POINT ( 'NONE',  ( 6.048345925472178308, 9.110135108809304327, 1.082531754730549967 ) ) ;
#55940=CARTESIAN_POINT ( 'NONE',  ( -2.875737979874388284, 6.369128386579808954, -0.7216878364870458196 ) ) ;
#55941=CARTESIAN_POINT ( 'NONE',  ( -6.961185525973791144, 7.086080966583015339, 0.7998128361456341429 ) ) ;
#55943=CARTESIAN_POINT ( 'NONE',  ( -5.808742468812186033, 5.741564066561132940, 0.000000000000000000 ) ) ;
#55953=CARTESIAN_POINT ( 'NONE',  ( 4.529305835417093640, 7.441884687032027657, -1.199719254218450271 ) ) ;
#55954=CARTESIAN_POINT ( 'NONE',  ( 5.061990249855835344, 6.999017606288844284, -1.599625672291273171 ) ) ;
#55957=CARTESIAN_POINT ( 'NONE',  ( 7.212011367826596242, 7.378711115411311638, 0.000000000000000000 ) ) ;
#55972=CARTESIAN_POINT ( 'NONE',  ( 6.038137670975392446, 7.156622065392123311, -1.170913047369964710 ) ) ;
#55977=CARTESIAN_POINT ( 'NONE',  ( 4.923546060418115822, 5.773167154356443120, -1.199719254218452047 ) ) ;
#55981=CARTESIAN_POINT ( 'NONE',  ( 4.085803189671889157, 5.860132702740892263, -1.599625672291273171 ) ) ;
#55986=CARTESIAN_POINT ( 'NONE',  ( 6.535912570239620578, 9.782925877658371405, 1.199719254218452047 ) ) ;
#55991=CARTESIAN_POINT ( 'NONE',  ( 4.407809338218622308, 8.156544971314787063, 0.000000000000000000 ) ) ;
#55993=CARTESIAN_POINT ( 'NONE',  ( -4.630991987519598396, 7.560518531151607213, 1.199719254218452935 ) ) ;
#55995=CARTESIAN_POINT ( 'NONE',  ( 3.217027588192558074, 6.975225629525113824, -1.734723475976807094E-15 ) ) ;
#56007=CARTESIAN_POINT ( 'NONE',  ( -7.783789588021474692, 8.253711738879413673, 0.7216878364870317197 ) ) ;
#56016=CARTESIAN_POINT ( 'NONE',  ( 0.1250758119425495474, 3.478658522888401716, -1.998845934954712966 ) ) ;
#56026=TOROIDAL_SURFACE ( 'NONE', #627, 0.4800000000000000933, 0.08000000000000000167 ) ;
#56042=CARTESIAN_POINT ( 'NONE',  ( 8.167861197590044142, 8.493869250135347215, 0.000000000000000000 ) ) ;
#56044=CARTESIAN_POINT ( 'NONE',  ( 6.119526231721748033, 8.232809585132461194, 1.599625672291269396 ) ) ;
#56057=CARTESIAN_POINT ( 'NONE',  ( -5.641074431737709283, 8.738948049406083385, -1.199719254218452047 ) ) ;
#56059=CARTESIAN_POINT ( 'NONE',  ( 7.173672674962134899, 7.541908673643526129, -0.7216878364870317197 ) ) ;
#56071=CARTESIAN_POINT ( 'NONE',  ( -4.125423880308188629, 8.035021303660014880, -0.7998128361456481317 ) ) ;
#56075=CARTESIAN_POINT ( 'NONE',  ( -4.340018570150318666, 6.156717313299049366, -1.443375672974066548 ) ) ;
#56078=CARTESIAN_POINT ( 'NONE',  ( -2.959422669532919326, 6.674686557755516780, 0.7998128361456352531 ) ) ;
#56101=CARTESIAN_POINT ( 'NONE',  ( -6.303615075710993665, 6.318915441276411471, -0.7998128361456362523 ) ) ;
#56123=CARTESIAN_POINT ( 'NONE',  ( -4.036671995544492297, 7.285761072467114019, 0.7944190476826870073 ) ) ;
#56126=CARTESIAN_POINT ( 'NONE',  ( -4.685224601974262271, 7.623789914682047808, -1.199719254218453823 ) ) ;
#56133=CARTESIAN_POINT ( 'NONE',  ( 7.661766205054107992, 8.111351125417501251, -0.7216878364870317197 ) ) ;
#56144=CARTESIAN_POINT ( 'NONE',  ( 5.061990249855835344, 6.999017606288844284, -1.599625672291273171 ) ) ;
#56152=CARTESIAN_POINT ( 'NONE',  ( 5.352436782344940802, 9.466536356036257871, 0.000000000000000000 ) ) ;
#56154=CARTESIAN_POINT ( 'NONE',  ( 4.857564175446106525, 8.889184981320973122, 0.7998128361456331437 ) ) ;
#56165=CARTESIAN_POINT ( 'NONE',  ( 6.477827756726281194, 6.756902019748111776, -0.2091553196570776485 ) ) ;
#56167=CARTESIAN_POINT ( 'NONE',  ( 5.017926250833595780, 7.907978821730911712, -1.082531754730548412 ) ) ;
#56178=DIRECTION ( 'NONE',  ( 0.000000000000000000, 0.000000000000000000, -1.000000000000000000 ) ) ;
#56189=CARTESIAN_POINT ( 'NONE',  ( -6.102578539482539810, 6.292298848917299736, 0.000000000000000000 ) ) ;
#56192=CARTESIAN_POINT ( 'NONE',  ( 7.614839552730775729, 8.913009562054615031, 1.199719254218452047 ) ) ;
#56209=CARTESIAN_POINT ( 'NONE',  ( 5.180097208873055692, 8.201141289397330780, -1.199719254218450271 ) ) ;
#56229=VERTEX_POINT ( 'NONE', #67556 ) ;
#56231=PLANE ( 'NONE',  #35128 ) ;
#56234=CARTESIAN_POINT ( 'NONE',  ( -6.486760921661624657, 6.767311426390788753, 0.2083394120615672529 ) ) ;
#56246=ADVANCED_FACE ( 'NONE', ( #169358 ), #2557, .F. ) ;
#56253=CARTESIAN_POINT ( 'NONE',  ( 4.367134877377630175, 7.148722219365612141, -1.082531754730548412 ) ) ;
#56264=CARTESIAN_POINT ( 'NONE',  ( -3.512971199716682591, 7.112567143062499930, 0.000000000000000000 ) ) ;
#56294=CARTESIAN_POINT ( 'NONE',  ( 5.551137550152489553, 5.441024994791534120, 0.7998128361456352531 ) ) ;
#56306=CARTESIAN_POINT ( 'NONE',  ( -5.153507786970267013, 8.066157280557016307, -1.082531754730549967 ) ) ;
#56309=CARTESIAN_POINT ( 'NONE',  ( 8.025500584646550806, 8.327781868367935658, 0.000000000000000000 ) ) ;
#56324=CARTESIAN_POINT ( 'NONE',  ( 2.905190055078214595, 6.611415174225076186, 0.7998128361456271485 ) ) ;
#56327=CARTESIAN_POINT ( 'NONE',  ( 4.757850744675321764, 8.278777181968248300, -0.9081679900534248562 ) ) ;
#56331=CARTESIAN_POINT ( 'NONE',  ( -1.930226670627066099, 8.999999999999998224, 0.7750000000000013545 ) ) ;
#56342=ORIENTED_EDGE ( 'NONE', *, *, #67389, .T. ) ;
#56356=CARTESIAN_POINT ( 'NONE',  ( -5.420227550413282636, 9.545625585449309725, 0.7998128361456291469 ) ) ;
#56359=CARTESIAN_POINT ( 'NONE',  ( -6.720001414228860881, 7.869031733802326123, -1.199719254218452047 ) ) ;
#56360=CARTESIAN_POINT ( 'NONE',  ( -6.168033539574335755, 6.160736982450306876, 0.7998128361456282587 ) ) ;
#56364=CARTESIAN_POINT ( 'NONE',  ( -5.872089928050201024, 8.904503111816948646, 1.082531754730550855 ) ) ;
#56367=B_SPLINE_CURVE_WITH_KNOTS ( 'NONE', 3,
 ( #193402, #33034, #13578, #30924 ),
 .UNSPECIFIED., .F., .F.,
 ( 4, 4 ),
 ( 0.000000000000000000, 1.000000000000000000 ),
 .UNSPECIFIED. ) ;
#56371=CARTESIAN_POINT ( 'NONE',  ( -5.164730172163054966, 4.990216387137135889, -0.7998128361456362523 ) ) ;
#56372=VECTOR ( 'NONE', #126403, 1000.000000000000000 ) ;
#56379=CARTESIAN_POINT ( 'NONE',  ( -7.767895665986912057, 8.027242796598338614, -0.7998128361456362523 ) ) ;
#56381=CARTESIAN_POINT ( 'NONE',  ( 4.985841187518467166, 7.931359929992748192, -1.059499378661461710 ) ) ;
#56384=DIRECTION ( 'NONE',  ( 0.000000000000000000, -1.000000000000000000, 0.000000000000000000 ) ) ;
#56386=CARTESIAN_POINT ( 'NONE',  ( 4.085803189671889157, 5.860132702740892263, -1.599625672291273171 ) ) ;
#56398=CARTESIAN_POINT ( 'NONE',  ( -5.413448473606448985, 9.537716662508005427, 0.000000000000000000 ) ) ;
#56411=CARTESIAN_POINT ( 'NONE',  ( 7.075376061485196821, 9.347967719856493218, 1.599625672291268286 ) ) ;
#56421=CARTESIAN_POINT ( 'NONE',  ( 4.560489089606875268, 8.500000000000003553, -0.2119548090071901036 ) ) ;
#56428=CARTESIAN_POINT ( 'NONE',  ( 5.678247172832384670, 7.430942480705488684, 1.324022058552588366 ) ) ;
#56434=CARTESIAN_POINT ( 'NONE',  ( -5.586581854188635177, 5.810800913040471194, -0.4357733342581562863 ) ) ;
#56454=CARTESIAN_POINT ( 'NONE',  ( -6.449404147558570166, 6.867377544759197150, 0.7074503392771516186 ) ) ;
#56472=CARTESIAN_POINT ( 'NONE',  ( -6.631873415740034083, 7.766215735565355160, 1.199719254218452047 ) ) ;
#56474=VERTEX_POINT ( 'NONE', #136873 ) ;
#56492=CARTESIAN_POINT ( 'NONE',  ( 4.037295881819344956, 7.932205305423046582, -0.7998128361456362523 ) ) ;
#56494=CARTESIAN_POINT ( 'NONE',  ( 7.797347741190739256, 8.269529584243604958, 0.7216878364870267237 ) ) ;
#56501=CARTESIAN_POINT ( 'NONE',  ( 6.174897528274166270, 6.957956273452501783, 0.8961316764096085574 ) ) ;
#56512=EDGE_CURVE ( 'NONE', #40754, #88097, #46295, .T. ) ;
#56521=CARTESIAN_POINT ( 'NONE',  ( -3.494969737272722643, 7.299491470118629088, -0.7998128361456481317 ) ) ;
#56523=CARTESIAN_POINT ( 'NONE',  ( 3.874598038455354665, 7.742391154831717692, -0.7998128361456362523 ) ) ;
#56526=CARTESIAN_POINT ( 'NONE',  ( -5.611095471209320174, 7.639640364534566075, 1.599625672291263179 ) ) ;
#56529=CARTESIAN_POINT ( 'NONE',  ( 7.550965208168244125, 7.774157262476569130, -0.7998128361456341429 ) ) ;
#56534=CARTESIAN_POINT ( 'NONE',  ( -4.601933621211449221, 8.477299672830683974, 0.2703350597391823706 ) ) ;
#56543=CARTESIAN_POINT ( 'NONE',  ( -5.953438849732214599, 6.118302544208584770, 0.7216878364870257245 ) ) ;
#56553=ORIENTED_EDGE ( 'NONE', *, *, #18226, .T. ) ;
#56556=CARTESIAN_POINT ( 'NONE',  ( 5.072158865288245444, 5.090142562357324429, 0.7216878364870338292 ) ) ;
#56560=CARTESIAN_POINT ( 'NONE',  ( -5.725286006720766707, 9.901527117808042178, 0.7998128361456291469 ) ) ;
#56564=CIRCLE ( 'NONE', #156768, 7.426656976154414558 ) ;
#56565=ORIENTED_EDGE ( 'NONE', *, *, #84212, .F. ) ;
#56578=CARTESIAN_POINT ( 'NONE',  ( 0.4640311867334303564, 2.877219473291478646, 2.027578619373314073 ) ) ;
#56599=CARTESIAN_POINT ( 'NONE',  ( -4.828112100242291760, 6.726159765073026264, -1.443375672974066548 ) ) ;
#56621=CARTESIAN_POINT ( 'NONE',  ( -6.933015448541747006, 9.181880338089085214, 1.599625672291269396 ) ) ;
#56622=CARTESIAN_POINT ( 'NONE',  ( -2.830620210203090181, 6.524417021870718258, 0.000000000000000000 ) ) ;
#56628=CARTESIAN_POINT ( 'NONE',  ( -3.284818356260900796, 7.054314858938165678, 0.7998128361456352531 ) ) ;
#56631=CYLINDRICAL_SURFACE ( 'NONE', #53897, 0.7499999999999997780 ) ;
#56637=CARTESIAN_POINT ( 'NONE',  ( -5.004894982100124068, 5.868074229652107121, 1.199719254218452935 ) ) ;
#56639=CARTESIAN_POINT ( 'NONE',  ( 6.170730229783032428, 7.061345527190763249, -1.063955632616358615 ) ) ;
#56643=CARTESIAN_POINT ( 'NONE',  ( 3.878514461961128479, 6.682628084666728085, -1.199719254218448494 ) ) ;
#56647=EDGE_CURVE ( 'NONE', #172448, #169017, #31320, .T. ) ;
#56650=CARTESIAN_POINT ( 'NONE',  ( -6.587282531393266360, 8.778525268082516320, 1.599625672291269396 ) ) ;
#56654=CARTESIAN_POINT ( 'NONE',  ( -3.959863383643135393, 6.777535159962392086, 1.199719254218452935 ) ) ;
#56659=CARTESIAN_POINT ( 'NONE',  ( 5.573810548549551491, 6.635772073796838200, -1.082531754730548412 ) ) ;
#56660=CARTESIAN_POINT ( 'NONE',  ( -4.299344108864949554, 8.030002203735486788, -0.7216878364870338292 ) ) ;
#56667=CARTESIAN_POINT ( 'NONE',  ( 4.095444919779759552, 6.935713618788495793, 1.199719254218451159 ) ) ;
#56668=VERTEX_POINT ( 'NONE', #184522 ) ;
#56674=CARTESIAN_POINT ( 'NONE',  ( 5.662465432362883355, 6.635239754958710989, 1.199719254218451159 ) ) ;
#56678=CARTESIAN_POINT ( 'NONE',  ( 4.797842130449009090, 8.250315290282747682, 0.8618622828703215166 ) ) ;
#56687=CARTESIAN_POINT ( 'NONE',  ( 6.723917837734620484, 6.809268663637336516, 0.000000000000000000 ) ) ;
#56697=CARTESIAN_POINT ( 'NONE',  ( 6.266472554743693912, 6.895788939045927712, 0.7740814723603481884 ) ) ;
#56714=CARTESIAN_POINT ( 'NONE',  ( -6.363572996767778100, 8.517530811019446091, -1.599625672291271394 ) ) ;
#56720=CARTESIAN_POINT ( 'NONE',  ( -4.370663978927101567, 5.060324124126029943, -1.009771797811724214 ) ) ;
#56727=CARTESIAN_POINT ( 'NONE',  ( 6.068156270568149324, 9.237210194708310951, 1.199719254218452047 ) ) ;
#56734=ORIENTED_EDGE ( 'NONE', *, *, #27310, .T. ) ;
#56735=CARTESIAN_POINT ( 'NONE',  ( 5.239300017038202917, 5.077214539491492928, 0.000000000000000000 ) ) ;
#56738=CARTESIAN_POINT ( 'NONE',  ( 4.787437638956922648, 6.678706226906775179, -1.443375672974068769 ) ) ;
#56744=DIRECTION ( 'NONE',  ( -0.000000000000000000, -0.000000000000000000, 1.000000000000000000 ) ) ;
#56754=CARTESIAN_POINT ( 'NONE',  ( -5.777182853198894463, 9.754147405458438058, 0.7216878364870267237 ) ) ;
#56755=CARTESIAN_POINT ( 'NONE',  ( 7.024532985656128936, 9.288650798055913427, 1.443375672974065660 ) ) ;
#56765=CARTESIAN_POINT ( 'NONE',  ( -4.098307573080856692, 8.003385611894792362, 0.7998128361456352531 ) ) ;
#56766=CARTESIAN_POINT ( 'NONE',  ( -4.502189528189771472, 7.410248995266807803, -1.199719254218453823 ) ) ;
#56768=CARTESIAN_POINT ( 'NONE',  ( 5.600926855776875435, 7.627776979863398310, -1.443375672974078761 ) ) ;
#56779=CARTESIAN_POINT ( 'NONE',  ( -4.611386515133914621, 8.374621496872018511, -0.1785149356163841239 ) ) ;
#56782=CARTESIAN_POINT ( 'NONE',  ( 5.899206235721897507, 6.055031161196562373, 0.000000000000000000 ) ) ;
#56786=CARTESIAN_POINT ( 'NONE',  ( -5.932574734431526942, 9.079031735882207244, 1.199719254218454489 ) ) ;
#56799=CARTESIAN_POINT ( 'NONE',  ( 4.342354338126830804, 8.288106837781779035, -0.7998128361456381397 ) ) ;
#56837=CARTESIAN_POINT ( 'NONE',  ( 5.045042558060919724, 8.899983727797476263, -0.7216878364870458196 ) ) ;
#56841=DIRECTION ( 'NONE',  ( 0.000000000000000000, 1.000000000000000000, 0.000000000000000000 ) ) ;
#56842=CARTESIAN_POINT ( 'NONE',  ( 6.875393295461478260, 8.154285278527437342, -1.082531754730548412 ) ) ;
#56866=CARTESIAN_POINT ( 'NONE',  ( -5.666381855868691808, 5.575476684793721383, 0.000000000000000000 ) ) ;
#56868=CARTESIAN_POINT ( 'NONE',  ( 5.763624699140868834, 7.817591130454727200, -1.443375672974078761 ) ) ;
#56874=CARTESIAN_POINT ( 'NONE',  ( -4.950662367645459305, 5.804802846121667415, -1.199719254218453823 ) ) ;
#56879=CARTESIAN_POINT ( 'NONE',  ( -5.153507786970262572, 9.026526494858359229, -0.7216878364870338292 ) ) ;
#56882=CARTESIAN_POINT ( 'NONE',  ( -7.747558435566414659, 8.003516027774422170, -0.7998128361456362523 ) ) ;
#56887=CARTESIAN_POINT ( 'NONE',  ( -4.472210567661380587, 6.310941310395290493, 1.599625672291270506 ) ) ;
#56901=CARTESIAN_POINT ( 'NONE',  ( -4.665414256878293031, 7.496714828783040296, -1.082531754730549967 ) ) ;
#56903=CARTESIAN_POINT ( 'NONE',  ( -5.519577934094894722, 7.532869904567736974, 1.443375672974058777 ) ) ;
#56905=CARTESIAN_POINT ( 'NONE',  ( 6.008198349511364000, 7.038594824965278995, 1.199719254218453823 ) ) ;
#56906=CARTESIAN_POINT ( 'NONE',  ( -6.252245114557387851, 7.323316050852266557, -1.199719254218453823 ) ) ;
#56922=CARTESIAN_POINT ( 'NONE',  ( 6.189669738297051360, 5.317594965474103041, 2.438128856460785698 ) ) ;
#56927=CARTESIAN_POINT ( 'NONE',  ( 6.851666526859736983, 9.086973262793417661, -1.599625672291269396 ) ) ;
#56933=CARTESIAN_POINT ( 'NONE',  ( -5.436182321379713578, 6.108390213082993903, 1.083092214668917919 ) ) ;
#56956=CARTESIAN_POINT ( 'NONE',  ( 5.081368137764759041, 4.913552992540472175, 0.1930038310255646206 ) ) ;
#56965=CARTESIAN_POINT ( 'NONE',  ( 5.550083779947807550, 7.568460058062819407, -1.599625672291283607 ) ) ;
#56968=CARTESIAN_POINT ( 'NONE',  ( -5.490125858891038213, 5.369844688319787451, -0.7998128361456362523 ) ) ;
#56982=CARTESIAN_POINT ( 'NONE',  ( 5.716698046817569434, 6.698511138489155137, -1.199719254218452047 ) ) ;
#56988=CARTESIAN_POINT ( 'NONE',  ( -6.400331034103001748, 9.624747418832267698, 1.199719254218452935 ) ) ;
#56992=CARTESIAN_POINT ( 'NONE',  ( 4.362691568547328202, 8.311833606605697256, -0.7998128361456381397 ) ) ;
#57004=CARTESIAN_POINT ( 'NONE',  ( 7.241463443474815520, 8.581367117876336437, -1.082531754730548412 ) ) ;
#57005=CARTESIAN_POINT ( 'NONE',  ( -3.526529353330355221, 6.168015774643768268, -1.082531754730546636 ) ) ;
#57006=CARTESIAN_POINT ( 'NONE',  ( -7.096767062110449942, 7.244259425409119046, -0.7998128361456362523 ) ) ;
#57022=CARTESIAN_POINT ( 'NONE',  ( 4.044074958626150185, 7.940114228364351767, 0.7998128361456271485 ) ) ;
#57023=CARTESIAN_POINT ( 'NONE',  ( 5.631432701629774051, 7.663367133358481631, 1.599625672291269396 ) ) ;
#57026=CARTESIAN_POINT ( 'NONE',  ( 5.664274315459256748, 9.830346811336296398, -0.7998128361456481317 ) ) ;
#57041=CARTESIAN_POINT ( 'NONE',  ( 5.713240515264599750, 7.403118591225121392, -1.316831503761767719 ) ) ;
#57043=CARTESIAN_POINT ( 'NONE',  ( 0.3910849555524695265, 2.914282954768474099, 2.026372354441466683 ) ) ;
#57044=CARTESIAN_POINT ( 'NONE',  ( 3.237364818613055473, 6.998952398349030268, -1.734723475976807094E-15 ) ) ;
#57050=CARTESIAN_POINT ( 'NONE',  ( 5.357406976055401948, 6.279338222599979424, 1.199719254218452935 ) ) ;
#57055=CARTESIAN_POINT ( 'NONE',  ( 3.410758162289653672, 6.136912401716668519, -1.199719254218453823 ) ) ;
#57059=CARTESIAN_POINT ( 'NONE',  ( 5.885648082108190238, 7.959951743916638733, 1.443375672974065660 ) ) ;
#57061=CARTESIAN_POINT ( 'NONE',  ( -6.089547271193396227, 7.133501900260939443, -1.199719254218453823 ) ) ;
#57063=CARTESIAN_POINT ( 'NONE',  ( 5.174371902270911150, 6.065797303184739420, 1.199719254218452047 ) ) ;
#57070=CARTESIAN_POINT ( 'NONE',  ( -4.528121930731268563, 7.284834279576167582, -1.112404534407253953 ) ) ;
#57073=CARTESIAN_POINT ( 'NONE',  ( -3.363304624641834106, 6.081549941127532222, -1.199719254218452047 ) ) ;
#57078=ORIENTED_EDGE ( 'NONE', *, *, #176104, .T. ) ;
#57082=CARTESIAN_POINT ( 'NONE',  ( 0.2892308902501606327, 3.295301175517658443, -2.053744536655083941 ) ) ;
#57091=FACE_OUTER_BOUND ( 'NONE', #62858, .T. ) ;
#57101=CARTESIAN_POINT ( 'NONE',  ( 5.085717018901939390, 5.105960408239938353, 0.000000000000000000 ) ) ;
#57106=CARTESIAN_POINT ( 'NONE',  ( 7.991605200612358573, 8.288237253661408843, 0.7998128361456281477 ) ) ;
#57108=CARTESIAN_POINT ( 'NONE',  ( 7.526711554241970248, 8.810193563817646734, -1.199719254218452047 ) ) ;
#57121=CARTESIAN_POINT ( 'NONE',  ( -6.622231685632140596, 6.690634819517756959, 0.000000000000000000 ) ) ;
#57123=CARTESIAN_POINT ( 'NONE',  ( 6.441532379824158383, 9.568852638886589546, -1.082531754730548412 ) ) ;
#57132=CARTESIAN_POINT ( 'NONE',  ( -5.632486471834530661, 5.535932070087196344, -0.7998128361456362523 ) ) ;
#57140=CARTESIAN_POINT ( 'NONE',  ( -4.553559489343377287, 6.405848385690952718, -1.599625672291271394 ) ) ;
#57150=ADVANCED_FACE ( 'NONE', ( #85448 ), #196633, .T. ) ;
#57166=CARTESIAN_POINT ( 'NONE',  ( -5.926849427829407269, 6.943687749669614995, -1.199719254218453823 ) ) ;
#57168=CARTESIAN_POINT ( 'NONE',  ( -4.842197138736131556, 5.678260079060780008, 1.199719254218452935 ) ) ;
#57178=CARTESIAN_POINT ( 'NONE',  ( -7.065207446497166366, 9.336104335703744539, 0.000000000000000000 ) ) ;
#57179=CARTESIAN_POINT ( 'NONE',  ( -4.787437654953777155, 6.678706214094487947, -1.250000000000001110 ) ) ;
#57193=CARTESIAN_POINT ( 'NONE',  ( -5.224688093219839402, 7.188831756880171397, -1.599625672291271394 ) ) ;
#57194=CARTESIAN_POINT ( 'NONE',  ( 4.010620668045937975, 3.846206254399761715, 2.500000000000000444 ) ) ;
#57202=CARTESIAN_POINT ( 'NONE',  ( 5.994113310573177422, 10.00723293906178846, 0.000000000000000000 ) ) ;
#57209=CARTESIAN_POINT ( 'NONE',  ( -4.204198463910354455, 7.819496816371283465, 0.4055711146801060929 ) ) ;
#57213=CARTESIAN_POINT ( 'NONE',  ( 6.059568310664962709, 6.034194215389424798, 0.7998128361456352531 ) ) ;
#57221=CARTESIAN_POINT ( 'NONE',  ( 7.550965208168244125, 7.774157262476569130, -0.7998128361456341429 ) ) ;
#57223=CARTESIAN_POINT ( 'NONE',  ( 5.155843554946782703, 9.237177590738404831, -0.7998128361456481317 ) ) ;
#57237=CARTESIAN_POINT ( 'NONE',  ( 6.348661983278831578, 6.841051910588018536, 0.6299351563821649069 ) ) ;
#57239=CARTESIAN_POINT ( 'NONE',  ( 4.895902868310594513, 8.725987423088758632, 0.000000000000000000 ) ) ;
#57249=ORIENTED_EDGE ( 'NONE', *, *, #144373, .T. ) ;
#57254=ORIENTED_EDGE ( 'NONE', *, *, #64428, .F. ) ;
#57257=CARTESIAN_POINT ( 'NONE',  ( -3.973948422136968084, 7.650373902552835226, -0.7216878364870458196 ) ) ;
#57261=CARTESIAN_POINT ( 'NONE',  ( 6.749980374757213575, 8.968339418673846097, 1.599625672291268286 ) ) ;
#57279=CARTESIAN_POINT ( 'NONE',  ( 7.340813827156391191, 7.528980651296110160, 0.7998128361456281477 ) ) ;
#57295=CARTESIAN_POINT ( 'NONE',  ( -5.749539660647037032, 8.865490816466966351, 1.199719254218454489 ) ) ;
#57317=CARTESIAN_POINT ( 'NONE',  ( 5.899206235721897507, 6.055031161196562373, 0.000000000000000000 ) ) ;
#57323=CARTESIAN_POINT ( 'NONE',  ( 6.502017186205484300, 9.743381262951846367, -1.199719254218452047 ) ) ;
#57327=CARTESIAN_POINT ( 'NONE',  ( -4.340018570150309785, 7.117086527600392287, -1.082531754730551743 ) ) ;
#57330=ORIENTED_EDGE ( 'NONE', *, *, #62930, .T. ) ;
#57332=CARTESIAN_POINT ( 'NONE',  ( 4.728284716797250375, 8.273450856974118750, 0.7059987189090509707 ) ) ;
#57359=CARTESIAN_POINT ( 'NONE',  ( 5.239300017038202917, 5.077214539491492928, 0.000000000000000000 ) ) ;
#57370=CARTESIAN_POINT ( 'NONE',  ( -7.160114521792834807, 8.486460042580672436, 1.082531754730549078 ) ) ;
#57372=CARTESIAN_POINT ( 'NONE',  ( 5.664274315459256748, 9.830346811336296398, -0.7998128361456481317 ) ) ;
#57386=CARTESIAN_POINT ( 'NONE',  ( 4.523580528814945545, 5.306540700819438960, 1.199719254218452047 ) ) ;
#57388=CARTESIAN_POINT ( 'NONE',  ( -5.167065940583949413, 5.200867483535597913, 0.000000000000000000 ) ) ;
#57403=ORIENTED_EDGE ( 'NONE', *, *, #213637, .F. ) ;
#57414=PRODUCT_DEFINITION_SHAPE ( 'NONE', 'NONE',  #90511 ) ;
#57421=CARTESIAN_POINT ( 'NONE',  ( -7.795011973214244883, 8.058878488363559356, 0.7998128361456341429 ) ) ;
#57424=CARTESIAN_POINT ( 'NONE',  ( -6.608673532018475960, 6.674816973635147477, -0.7998128361456362523 ) ) ;
#57430=CARTESIAN_POINT ( 'NONE',  ( -6.333067150914850174, 8.481940657524365434, 1.443375672974064550 ) ) ;
#57431=CARTESIAN_POINT ( 'NONE',  ( 7.363486825553451354, 8.723727730301414240, -1.082531754730548412 ) ) ;
#57437=CARTESIAN_POINT ( 'NONE',  ( -7.587723245503481095, 8.881373870289390737, 1.199719254218452047 ) ) ;
#57446=CARTESIAN_POINT ( 'NONE',  ( -5.932574734431526942, 9.079031735882207244, 1.199719254218454489 ) ) ;
#57448=CARTESIAN_POINT ( 'NONE',  ( 5.410124943364367667, 7.538760657221164507, -1.247639402986647550 ) ) ;
#57452=CARTESIAN_POINT ( 'NONE',  ( 5.717509255324264572, 7.006698007003683948, 2.500000000000000444 ) ) ;
#57454=CARTESIAN_POINT ( 'NONE',  ( 5.598591087800349086, 5.496387455380669529, -0.7998128361456481317 ) ) ;
#57462=AXIS2_PLACEMENT_3D ( 'NONE', #142368, #208377, #171618 ) ;
#57464=CARTESIAN_POINT ( 'NONE',  ( -6.749980374757255319, 8.968339418673846097, 1.599625672291269396 ) ) ;
#57478=CARTESIAN_POINT ( 'NONE',  ( 8.167861197590044142, 8.493869250135347215, 0.000000000000000000 ) ) ;
#57492=CARTESIAN_POINT ( 'NONE',  ( 6.430738266435902517, 6.882057634903050669, 0.7203813067775278745 ) ) ;
#57494=CARTESIAN_POINT ( 'NONE',  ( -3.797692425159308716, 7.444741906078900406, 0.000000000000000000 ) ) ;
#57522=CARTESIAN_POINT ( 'NONE',  ( 4.095444919779759552, 6.935713618788495793, 1.199719254218451159 ) ) ;
#57542=CARTESIAN_POINT ( 'NONE',  ( -4.959250327548641479, 9.007818825440551791, -0.7998128361456362523 ) ) ;
#57557=CARTESIAN_POINT ( 'NONE',  ( 6.086684617892325733, 6.065829907154645539, -0.7998128361456481317 ) ) ;
#57559=CARTESIAN_POINT ( 'NONE',  ( 7.526184668917440312, 8.913541880892736913, -1.082531754730548412 ) ) ;
#57566=CARTESIAN_POINT ( 'NONE',  ( 4.726673625894836306, 8.212911231124076394, 0.6865719651209405416 ) ) ;
#57568=CARTESIAN_POINT ( 'NONE',  ( 5.417061852544872380, 7.532864896096530316, 1.248242807326222392 ) ) ;
#57586=EDGE_LOOP ( 'NONE', ( #189373, #45539, #134977, #167456 ) ) ;
#57588=CARTESIAN_POINT ( 'NONE',  ( -4.736594563127865420, 6.619389305106191834, -1.599625672291271394 ) ) ;
#57590=CARTESIAN_POINT ( 'NONE',  ( 4.817943484809818600, 6.714296380401858499, 1.599625672291269396 ) ) ;
#57593=CARTESIAN_POINT ( 'NONE',  ( -5.529746549527323474, 7.544733289238903851, -1.599625672291271394 ) ) ;
#57595=CARTESIAN_POINT ( 'NONE',  ( 5.580062740476173566, 8.667767742934335828, 1.199719254218451159 ) ) ;
#57600=CARTESIAN_POINT ( 'NONE',  ( -5.747140441703231240, 7.374164810257596514, -1.320148062302946013 ) ) ;
#57609=CARTESIAN_POINT ( 'NONE',  ( -4.624739795592943459, 6.488892076315448065, -1.443375672974066548 ) ) ;
#57620=CARTESIAN_POINT ( 'NONE',  ( 4.231553341240963384, 7.950912974840849579, -0.7216878364870357165 ) ) ;
#57624=CARTESIAN_POINT ( 'NONE',  ( -7.045397100956844127, 8.248660034984974132, -1.199719254218452047 ) ) ;
#57637=CARTESIAN_POINT ( 'NONE',  ( 4.181342156266883769, 7.197418463578268089, 1.132749409379085748 ) ) ;
#57641=CARTESIAN_POINT ( 'NONE',  ( 5.899733120602060232, 6.912052057904395141, -1.199719254218452047 ) ) ;
#57665=CARTESIAN_POINT ( 'NONE',  ( -5.722950238744243023, 7.770137593325314285, 1.443375672974058777 ) ) ;
#57690=CARTESIAN_POINT ( 'NONE',  ( -7.095713291905736853, 9.371694488680407886, 1.599625672291269396 ) ) ;
#57691=CARTESIAN_POINT ( 'NONE',  ( -5.015590482412729756, 4.816220082428420923, 0.000000000000000000 ) ) ;
#57695=CARTESIAN_POINT ( 'NONE',  ( -5.808742468812186033, 5.741564066561132940, 0.000000000000000000 ) ) ;
#57703=CARTESIAN_POINT ( 'NONE',  ( -3.980200614063634568, 6.801261928786307642, 1.199719254218452935 ) ) ;
#57705=CARTESIAN_POINT ( 'NONE',  ( 6.596403382356258227, 6.772441155557838321, -0.1798620802159808241 ) ) ;
#57709=CARTESIAN_POINT ( 'NONE',  ( 4.179656494762836516, 8.098292687190454586, -0.7998128361456362523 ) ) ;
#57714=CARTESIAN_POINT ( 'NONE',  ( -4.938913097128142304, 8.984092056616635347, -0.7998128361456362523 ) ) ;
#57718=CARTESIAN_POINT ( 'NONE',  ( -3.298376509874564988, 7.070132704820777825, 0.000000000000000000 ) ) ;
#57724=CARTESIAN_POINT ( 'NONE',  ( 6.685579144870162693, 6.972466221869550118, -0.7216878364870458196 ) ) ;
#57725=CARTESIAN_POINT ( 'NONE',  ( -5.817857313595549584, 6.920493299683823096, 1.082531754730549078 ) ) ;
#57732=CARTESIAN_POINT ( 'NONE',  ( 3.553118775233146120, 6.302999783484076524, -1.199719254218453823 ) ) ;
#57742=CARTESIAN_POINT ( 'NONE',  ( 5.323208952783781811, 7.729862296028469970, 1.309151360253474339 ) ) ;
#57751=CARTESIAN_POINT ( 'NONE',  ( 7.035755370848908896, 7.173079118937375931, 0.7998128361456352531 ) ) ;
#57761=CARTESIAN_POINT ( 'NONE',  ( 6.124909263556299166, 6.992440323537196356, 0.9511531368890328020 ) ) ;
#57772=CARTESIAN_POINT ( 'NONE',  ( -4.736138090107036902, 8.221507128720061175, -0.6901939221467829899 ) ) ;
#57778=CARTESIAN_POINT ( 'NONE',  ( -6.740338644649361832, 7.892758502626242567, -1.199719254218452047 ) ) ;
#57791=CARTESIAN_POINT ( 'NONE',  ( 5.851225812749518695, 8.984124660586543243, -1.199719254218452047 ) ) ;
#57795=CARTESIAN_POINT ( 'NONE',  ( -5.608757509018976961, 5.622941248444247364, -0.3933255993917709747 ) ) ;
#57800=CARTESIAN_POINT ( 'NONE',  ( 4.228163802615382494, 6.026220084508304708, -1.599625672291269396 ) ) ;
#57804=CARTESIAN_POINT ( 'NONE',  ( 4.055297343818933697, 5.824542549245813383, 1.443375672974058777 ) ) ;
#57815=CARTESIAN_POINT ( 'NONE',  ( -7.783789588021474692, 8.253711738879413673, 0.7216878364870317197 ) ) ;
#57816=CARTESIAN_POINT ( 'NONE',  ( 4.065465959251388206, 5.836405933916976707, -1.599625672291269396 ) ) ;
#57825=EDGE_LOOP ( 'NONE', ( #126390, #67432, #126270, #25136, #66645, #213616 ) ) ;
#57828=CARTESIAN_POINT ( 'NONE',  ( -5.448397627845328550, 7.449826213943242514, 1.599625672291263179 ) ) ;
#57829=CARTESIAN_POINT ( 'NONE',  ( -4.634908411025374875, 6.500755460986618495, 1.599625672291263179 ) ) ;
#57831=CARTESIAN_POINT ( 'NONE',  ( 7.471952054462754234, 8.850270497362297206, 1.082531754730549078 ) ) ;
#57837=CARTESIAN_POINT ( 'NONE',  ( -3.147653791585956817, 8.919999999999845386, 2.419999999999999485 ) ) ;
#57841=CARTESIAN_POINT ( 'NONE',  ( -5.122256578951685846, 7.813849795838854639, -1.152996464563345924 ) ) ;
#57842=CARTESIAN_POINT ( 'NONE',  ( -6.391719147208884344, 6.567463349398176220, -2.438448605600926467 ) ) ;
#57846=CARTESIAN_POINT ( 'NONE',  ( 4.746763178560254204, 6.631252689777363152, 1.443375672974065660 ) ) ;
#57851=CARTESIAN_POINT ( 'NONE',  ( -7.456058132872594335, 7.663432341298296535, 0.000000000000000000 ) ) ;
#57865=CARTESIAN_POINT ( 'NONE',  ( 5.987861119090863049, 7.014868056141362551, 1.199719254218452047 ) ) ;
#57880=CARTESIAN_POINT ( 'NONE',  ( 4.260029445439537987, 7.236136616047151193, 2.419999999999999485 ) ) ;
#57900=CARTESIAN_POINT ( 'NONE',  ( 5.506019780925567986, 8.477421273504887722, -1.082531754730548412 ) ) ;
#57905=CYLINDRICAL_SURFACE ( 'NONE', #9272, 2.000000000000000000 ) ;
#57906=CARTESIAN_POINT ( 'NONE',  ( 7.824464048418096951, 8.301165276008827476, -0.7216878364870317197 ) ) ;
#57932=CARTESIAN_POINT ( 'NONE',  ( -4.305596300791617814, 7.180890229968955651, 1.199719254218452935 ) ) ;
#57934=CARTESIAN_POINT ( 'NONE',  ( 6.007671464186837618, 6.181573927739029806, 0.7216878364870328300 ) ) ;
#57940=CARTESIAN_POINT ( 'NONE',  ( -4.248501033035892327, 6.049946853332221153, -1.599625672291271394 ) ) ;
#57945=CARTESIAN_POINT ( 'NONE',  ( -6.292392690518209264, 8.434487120394948079, -1.443375672974066548 ) ) ;
#57952=CARTESIAN_POINT ( 'NONE',  ( -6.134138155540168391, 6.121192367743780949, 0.000000000000000000 ) ) ;
#57962=FACE_OUTER_BOUND ( 'NONE', #81494, .T. ) ;
#57964=CARTESIAN_POINT ( 'NONE',  ( -5.478903473698268023, 5.564677938835638216, -0.7216878364870338292 ) ) ;
#57968=CARTESIAN_POINT ( 'NONE',  ( -6.468648687051513413, 7.679749902049126220, 1.082531754730549078 ) ) ;
#57969=CARTESIAN_POINT ( 'NONE',  ( 5.200434439293556643, 8.224868058221247225, -1.199719254218452047 ) ) ;
#57970=CARTESIAN_POINT ( 'NONE',  ( -7.144220599758281054, 7.299621885998258897, 0.7998128361456341429 ) ) ;
#57991=CARTESIAN_POINT ( 'NONE',  ( 7.147083253059300922, 8.367293879104554577, 1.199719254218452935 ) ) ;
#58018=CARTESIAN_POINT ( 'NONE',  ( 5.048745089568936528, 4.904218937602238704, 0.2966393288263181605 ) ) ;
#58026=CARTESIAN_POINT ( 'NONE',  ( 4.899292406491845497, 6.809203455697518947, -1.599625672291273171 ) ) ;
#58029=CARTESIAN_POINT ( 'NONE',  ( -5.002032328799064231, 4.800402236545811441, -0.7998128361456362523 ) ) ;
#58032=CARTESIAN_POINT ( 'NONE',  ( -4.597623488365601752, 8.377994813152914944, 0.7216878364870267237 ) ) ;
#58043=CARTESIAN_POINT ( 'NONE',  ( 3.627688620108284745, 6.389997935838436227, 1.199719254218452047 ) ) ;
#58044=CARTESIAN_POINT ( 'NONE',  ( 6.866278450678116485, 6.975356045404744521, 0.000000000000000000 ) ) ;
#58056=CARTESIAN_POINT ( 'NONE',  ( 5.468734858265785093, 7.473552982767158070, 1.599625672291269396 ) ) ;
#58069=CARTESIAN_POINT ( 'NONE',  ( 5.560252395380198998, 9.501061871336672127, 0.7216878364870317197 ) ) ;
#58070=CARTESIAN_POINT ( 'NONE',  ( -3.336715202739028552, 6.906935146588564223, 0.7216878364870338292 ) ) ;
#58071=CARTESIAN_POINT ( 'NONE',  ( -7.774674742793745708, 8.035151719539642912, 0.7998128361456341429 ) ) ;
#58082=CARTESIAN_POINT ( 'NONE',  ( 7.018280793729500644, 8.217024343219755167, -1.199719254218452047 ) ) ;
#58084=CARTESIAN_POINT ( 'NONE',  ( 5.611095471209277541, 7.639640364534566075, 1.599625672291268286 ) ) ;
#58085=CARTESIAN_POINT ( 'NONE',  ( 7.550965208168244125, 7.774157262476569130, -0.7998128361456341429 ) ) ;
#58088=CARTESIAN_POINT ( 'NONE',  ( 6.933015448541703485, 9.181880338089085214, 1.599625672291268286 ) ) ;
#58107=EDGE_CURVE ( 'NONE', #93276, #24495, #194095, .T. ) ;
#58110=CARTESIAN_POINT ( 'NONE',  ( 3.711900195091365262, 7.552577004240394132, -0.7998128361456362523 ) ) ;
#58114=CARTESIAN_POINT ( 'NONE',  ( 4.603875680292229156, 7.528882839386387360, 1.199719254218452047 ) ) ;
#58119=CARTESIAN_POINT ( 'NONE',  ( 3.573456005653643519, 6.326726552307992080, -1.199719254218453823 ) ) ;
#58123=CARTESIAN_POINT ( 'NONE',  ( 6.712695452541852070, 7.004101914153185504, 0.000000000000000000 ) ) ;
#58126=CARTESIAN_POINT ( 'NONE',  ( -5.143339171537843590, 7.093924681584509173, 1.599625672291263179 ) ) ;
#58127=CARTESIAN_POINT ( 'NONE',  ( 3.691562964670865199, 7.528850235416478576, -0.7998128361456362523 ) ) ;
#58137=CARTESIAN_POINT ( 'NONE',  ( -4.767627293860968507, 5.591261926706423857, -1.199719254218453823 ) ) ;
#58167=CARTESIAN_POINT ( 'NONE',  ( 3.092668437693027794, 6.622213920701574885, -0.7216878364870338292 ) ) ;
#58172=CARTESIAN_POINT ( 'NONE',  ( 6.668631453075247073, 8.873432343378178544, -1.599625672291281386 ) ) ;
#58173=CARTESIAN_POINT ( 'NONE',  ( 3.241808126998965811, 6.796210224891872542, 0.7216878364870257245 ) ) ;
#58186=CARTESIAN_POINT ( 'NONE',  ( -5.773793314573309132, 7.829454515125894964, 1.599625672291263179 ) ) ;
#58188=CARTESIAN_POINT ( 'NONE',  ( 6.983858524370782028, 8.280828045588322084, 1.082531754730549967 ) ) ;
#58198=CARTESIAN_POINT ( 'NONE',  ( -6.147696309153835692, 6.137010213626392208, 0.7998128361456281477 ) ) ;
#58208=CARTESIAN_POINT ( 'NONE',  ( -3.284818356260900796, 7.054314858938165678, 0.7998128361456352531 ) ) ;
#58221=AXIS2_PLACEMENT_3D ( 'NONE', #160311, #45513, #206914 ) ;
#58231=CARTESIAN_POINT ( 'NONE',  ( -4.782994330570982555, 8.802186828966616972, 0.000000000000000000 ) ) ;
#58238=EDGE_LOOP ( 'NONE', ( #12559, #94278, #112828, #132962 ) ) ;
#58245=EDGE_LOOP ( 'NONE', ( #51854, #77240, #15271, #162854 ) ) ;
#58251=CARTESIAN_POINT ( 'NONE',  ( -6.966220764712169000, 6.002124920821316323, -2.420000000000000373 ) ) ;
#58259=CARTESIAN_POINT ( 'NONE',  ( -4.956387674247580755, 7.940146832334256111, 1.199719254218452935 ) ) ;
#58286=CARTESIAN_POINT ( 'NONE',  ( 6.688968683495743583, 8.897159112202094988, -1.599625672291283607 ) ) ;
#58288=CARTESIAN_POINT ( 'NONE',  ( 5.169401708560450004, 9.252995436621013425, 0.000000000000000000 ) ) ;
#58302=CARTESIAN_POINT ( 'NONE',  ( 6.206332990038123221, 6.936436922908462144, -0.8583981852504622978 ) ) ;
#58304=CARTESIAN_POINT ( 'NONE',  ( 6.549997609177859559, 6.814287763561861944, 0.000000000000000000 ) ) ;
#58312=CARTESIAN_POINT ( 'NONE',  ( -4.390861645979385663, 6.216034235099629157, -1.599625672291271394 ) ) ;
#58320=CARTESIAN_POINT ( 'NONE',  ( -7.078765599666485997, 7.431183752465250869, 0.000000000000000000 ) ) ;
#58324=CARTESIAN_POINT ( 'NONE',  ( 6.535912570239620578, 9.782925877658371405, 1.199719254218452047 ) ) ;
#58340=CARTESIAN_POINT ( 'NONE',  ( 7.666209513884374438, 7.908608952478760834, 0.7998128361456281477 ) ) ;
#58358=ORIENTED_EDGE ( 'NONE', *, *, #6353, .T. ) ;
#58361=CARTESIAN_POINT ( 'NONE',  ( -6.017840079619296567, 8.114175741012878973, -1.599625672291271394 ) ) ;
#58366=CARTESIAN_POINT ( 'NONE',  ( -6.492041734278776843, 6.763935894940780180, 0.1675349064616058481 ) ) ;
#58382=CARTESIAN_POINT ( 'NONE',  ( 5.560252395380206991, 7.580323442733986283, 1.443375672974065660 ) ) ;
#58383=ORIENTED_EDGE ( 'NONE', *, *, #61843, .T. ) ;
#58393=CARTESIAN_POINT ( 'NONE',  ( -4.665414256878304577, 5.575976400180357118, -1.082531754730549967 ) ) ;
#58397=AXIS2_PLACEMENT_3D ( 'NONE', #98738, #133399, #14255 ) ;
#58426=CARTESIAN_POINT ( 'NONE',  ( 4.095444919779759552, 6.935713618788495793, 1.199719254218451159 ) ) ;
#58437=CARTESIAN_POINT ( 'NONE',  ( -5.289089323106922258, 9.184704953684462936, 0.7216878364870267237 ) ) ;
#58439=CARTESIAN_POINT ( 'NONE',  ( 5.207740400980577888, 5.248321020665011716, 0.000000000000000000 ) ) ;
#58458=CARTESIAN_POINT ( 'NONE',  ( -3.363831509966360489, 6.938570838353784076, -0.7216878364870458196 ) ) ;
#58488=CARTESIAN_POINT ( 'NONE',  ( -6.474900878978163021, 9.711745571186627402, -1.199719254218452047 ) ) ;
#58491=CARTESIAN_POINT ( 'NONE',  ( -5.478376588373717659, 8.549133898814758936, -1.199719254218452047 ) ) ;
#58493=CARTESIAN_POINT ( 'NONE',  ( -5.983791420057156252, 7.107340751733106643, 1.079986564815892613 ) ) ;
#58496=CARTESIAN_POINT ( 'NONE',  ( -6.577113915960836721, 8.766661883411348555, -1.443375672974066548 ) ) ;
#58499=CARTESIAN_POINT ( 'NONE',  ( -5.164730172163054966, 4.990216387137135889, -0.7998128361456362523 ) ) ;
#58503=CARTESIAN_POINT ( 'NONE',  ( -3.156015896931072540, 6.904045323053366268, 0.000000000000000000 ) ) ;
#58511=CARTESIAN_POINT ( 'NONE',  ( -6.933015448541747006, 9.181880338089085214, 1.599625672291269396 ) ) ;
#58513=CARTESIAN_POINT ( 'NONE',  ( 4.730098472736550264, 8.327237590489470875, -0.7222317683119976461 ) ) ;
#58517=CARTESIAN_POINT ( 'NONE',  ( 4.598150373690133463, 5.393538853173795111, -1.199719254218452047 ) ) ;
#58538=CARTESIAN_POINT ( 'NONE',  ( 5.969332771766739931, 10.18624834369502885, -0.7998128361456481317 ) ) ;
#58554=CARTESIAN_POINT ( 'NONE',  ( 6.548892101489681927, 6.803534504848940401, 0.4251794856353352525 ) ) ;
#58556=CARTESIAN_POINT ( 'NONE',  ( -5.939880696118548187, 6.102484698325975288, 0.000000000000000000 ) ) ;
#58584=CARTESIAN_POINT ( 'NONE',  ( 4.146814880933355596, 5.931313009212638931, 1.599625672291261402 ) ) ;
#58604=CARTESIAN_POINT ( 'NONE',  ( -6.363572996767778100, 8.517530811019446091, -1.599625672291271394 ) ) ;
#58617=CARTESIAN_POINT ( 'NONE',  ( 6.059568310664962709, 6.034194215389424798, 0.7998128361456352531 ) ) ;
#58629=CARTESIAN_POINT ( 'NONE',  ( 4.790043373817672645, 8.140258622390808441, 0.8134525054356611662 ) ) ;
#58630=CARTESIAN_POINT ( 'NONE',  ( -5.112833325684916552, 7.058334528089424076, -1.443375672974066770 ) ) ;
#58631=CARTESIAN_POINT ( 'NONE',  ( 4.978641999450219124, 7.938775605734648799, 1.052364473307040305 ) ) ;
#58632=CARTESIAN_POINT ( 'NONE',  ( 5.309888000197702240, 7.741188690324601218, 1.308016840036421602 ) ) ;
#58646=ORIENTED_EDGE ( 'NONE', *, *, #153640, .F. ) ;
#58651=CARTESIAN_POINT ( 'NONE',  ( -6.168033539574333979, 6.160736982450306876, 0.7998128361456281477 ) ) ;
#58653=CARTESIAN_POINT ( 'NONE',  ( 3.250922972226694352, 7.014770244231638863, 0.7998128361456281477 ) ) ;
#58656=CARTESIAN_POINT ( 'NONE',  ( -5.641074431737709283, 8.738948049406083385, -1.199719254218452047 ) ) ;
#58659=FACE_OUTER_BOUND ( 'NONE', #212607, .T. ) ;
#58664=CARTESIAN_POINT ( 'NONE',  ( -4.671432059311929841, 8.392430178223424520, -0.5935467769075646327 ) ) ;
#58668=EDGE_CURVE ( 'NONE', #40348, #123271, #193955, .T. ) ;
#58674=DIRECTION ( 'NONE',  ( 0.9629573728775006058, 0.2631879969435746425, 0.05869562407617064104 ) ) ;
#58683=CARTESIAN_POINT ( 'NONE',  ( 4.068855497876973537, 7.761098824249525130, -0.7216878364870338292 ) ) ;
#58686=CARTESIAN_POINT ( 'NONE',  ( -7.923814432544069142, 8.209148024248356990, 0.000000000000000000 ) ) ;
#58700=CARTESIAN_POINT ( 'NONE',  ( 4.278479993564246797, 7.149254538203735798, 1.199719254218452047 ) ) ;
#58727=CARTESIAN_POINT ( 'NONE',  ( -4.990809943606269172, 8.836712344267034780, -0.7216878364870338292 ) ) ;
#58750=ORIENTED_EDGE ( 'NONE', *, *, #73552, .F. ) ;
#58751=CARTESIAN_POINT ( 'NONE',  ( -5.921879234118920365, 10.13088588310589699, 0.000000000000000000 ) ) ;
#58752=EDGE_CURVE ( 'NONE', #60255, #112565, #203512, .T. ) ;
#58757=CARTESIAN_POINT ( 'NONE',  ( -3.786470039966538970, 7.639575156594750283, 0.000000000000000000 ) ) ;
#58760=CARTESIAN_POINT ( 'NONE',  ( 6.387299765813869712, 6.624473612970537495, 0.000000000000000000 ) ) ;
#58765=CARTESIAN_POINT ( 'NONE',  ( -6.400331034103001748, 9.624747418832267698, 1.199719254218452935 ) ) ;
#58767=CARTESIAN_POINT ( 'NONE',  ( 6.590809034589254267, 6.776089313701147532, -0.2235409772415736240 ) ) ;
#58771=CARTESIAN_POINT ( 'NONE',  ( 4.878955176071345434, 6.785476686873604280, -1.599625672291269396 ) ) ;
#58778=CARTESIAN_POINT ( 'NONE',  ( -6.994027139803241866, 9.253060644560830994, -1.599625672291271394 ) ) ;
#58781=CARTESIAN_POINT ( 'NONE',  ( -5.581116510680924847, 6.540332679663050541, -1.199719254218453823 ) ) ;
#58786=CARTESIAN_POINT ( 'NONE',  ( 4.516274566683592617, 8.283087737857252719, -0.7216878364870357165 ) ) ;
#58787=CARTESIAN_POINT ( 'NONE',  ( -5.926322542504877333, 7.047036066744706950, -1.082531754730549967 ) ) ;
#58794=CARTESIAN_POINT ( 'NONE',  ( 3.366167277942881064, 7.149221934233827014, -0.7998128361456362523 ) ) ;
#58798=DIRECTION ( 'NONE',  ( -0.6507913734559606089, 0.7592566023653033458, 0.000000000000000000 ) ) ;
#58799=CARTESIAN_POINT ( 'NONE',  ( 2.969872605471104876, 6.605953636086679737, -0.06813560672779371552 ) ) ;
#58806=CARTESIAN_POINT ( 'NONE',  ( 5.678247172832384670, 7.430942480705488684, 1.324022058552588366 ) ) ;
#58826=CARTESIAN_POINT ( 'NONE',  ( 4.594471896879979589, 8.374412622790375238, -0.01639726577711345112 ) ) ;
#58833=CARTESIAN_POINT ( 'NONE',  ( 5.643937085038755797, 9.806620042512378177, -0.7998128361456481317 ) ) ;
#58837=CARTESIAN_POINT ( 'NONE',  ( -4.675522092136524144, 8.294237829558845476, 0.5223692772225538850 ) ) ;
#58843=CARTESIAN_POINT ( 'NONE',  ( -6.794571259104023930, 7.956029886156682274, 1.199719254218452047 ) ) ;
#58857=CARTESIAN_POINT ( 'NONE',  ( 5.027041095616958444, 9.086908054853605421, 0.000000000000000000 ) ) ;
#58865=CARTESIAN_POINT ( 'NONE',  ( 4.041212305325117882, 6.872442235258051646, -1.199719254218448494 ) ) ;
#58868=ADVANCED_FACE ( 'NONE', ( #7458 ), #56231, .F. ) ;
#58869=CARTESIAN_POINT ( 'NONE',  ( 6.360183458142179447, 6.592837920686898556, -0.7216878364870458196 ) ) ;
#58886=CARTESIAN_POINT ( 'NONE',  ( -4.339491684825780737, 7.220434844675483355, -1.199719254218455378 ) ) ;
#58888=CARTESIAN_POINT ( 'NONE',  ( 4.577813143269636065, 5.369812084349879555, -1.199719254218450271 ) ) ;
#58902=CARTESIAN_POINT ( 'NONE',  ( -6.771371375382467583, 6.864631124226471037, -0.7998128361456362523 ) ) ;
#58903=CARTESIAN_POINT ( 'NONE',  ( -5.309953438407606363, 6.223975762010839574, 1.199719254218452935 ) ) ;
#58905=CARTESIAN_POINT ( 'NONE',  ( 7.200788982189461507, 8.533913579710086239, -1.082531754730548412 ) ) ;
#58907=VERTEX_POINT ( 'NONE', #122392 ) ;
#58910=DIRECTION ( 'NONE',  ( -0.3281536732072464768, -0.000000000000000000, 0.9446243521954066358 ) ) ;
#58914=CARTESIAN_POINT ( 'NONE',  ( -5.386282318077409315, 7.574627448853999745, -1.244059264865501557 ) ) ;
#58917=CARTESIAN_POINT ( 'NONE',  ( 5.451787166470912993, 6.493411461371761284, -1.082531754730548412 ) ) ;
#58921=CARTESIAN_POINT ( 'NONE',  ( -7.293360289508603600, 7.473618190706972086, 0.000000000000000000 ) ) ;
#58936=CARTESIAN_POINT ( 'NONE',  ( 6.367489420273535039, 7.457767740854454708, -1.199719254218452047 ) ) ;
#58972=CARTESIAN_POINT ( 'NONE',  ( 7.688882512725796481, 8.142986817701137525, 0.000000000000000000 ) ) ;
#58976=CARTESIAN_POINT ( 'NONE',  ( 6.966220764712121927, 6.002124920821316323, 2.420000000000000373 ) ) ;
#58977=CARTESIAN_POINT ( 'NONE',  ( 5.817857313595521163, 9.801600942587855414, -0.7216878364870458196 ) ) ;
#59001=CARTESIAN_POINT ( 'NONE',  ( -3.481411583659053566, 7.283673624236017830, 0.000000000000000000 ) ) ;
#59003=CARTESIAN_POINT ( 'NONE',  ( 4.706088717274896638, 7.544168365912456764, 1.082531754730548412 ) ) ;
#59008=CARTESIAN_POINT ( 'NONE',  ( -5.010620288702242853, 8.003418215864698482, -1.199719254218453823 ) ) ;
#59012=CARTESIAN_POINT ( 'NONE',  ( -6.116136693540540570, 10.14959355252370266, 0.000000000000000000 ) ) ;
#59019=CARTESIAN_POINT ( 'NONE',  ( -4.960304097753355457, 6.880383762169266504, 1.599625672291263179 ) ) ;
#59027=CARTESIAN_POINT ( 'NONE',  ( -4.930325137224961907, 5.781076077297750970, -1.199719254218453823 ) ) ;
#59030=CARTESIAN_POINT ( 'NONE',  ( -4.326460416536637155, 8.061637896019123062, 0.000000000000000000 ) ) ;
#59031=CARTESIAN_POINT ( 'NONE',  ( -4.624739795592931912, 8.409630504918133909, -0.7216878364870338292 ) ) ;
#59032=CARTESIAN_POINT ( 'NONE',  ( 6.713222337422018349, 7.861122810861019161, -1.199719254218452047 ) ) ;
#59033=CARTESIAN_POINT ( 'NONE',  ( -6.631873415740034083, 7.766215735565355160, 1.199719254218452047 ) ) ;
#59052=CARTESIAN_POINT ( 'NONE',  ( 7.849244587668864348, 8.122149871893999062, 0.7998128361456291469 ) ) ;
#59073=CARTESIAN_POINT ( 'NONE',  ( 4.730098472736550264, 8.327237590489470875, -0.7222317683119976461 ) ) ;
#59078=DIRECTION ( 'NONE',  ( 0.000000000000000000, 1.000000000000000000, 0.000000000000000000 ) ) ;
#59089=CARTESIAN_POINT ( 'NONE',  ( 6.119526231721748033, 8.232809585132461194, 1.599625672291269396 ) ) ;
#59092=FACE_OUTER_BOUND ( 'NONE', #67179, .T. ) ;
#59095=CARTESIAN_POINT ( 'NONE',  ( -5.899206235277530297, 9.896508017883515862, 0.7216878364870267237 ) ) ;
#59106=CARTESIAN_POINT ( 'NONE',  ( 6.481679955784983349, 9.719654494127929922, -1.199719254218452047 ) ) ;
#59107=CARTESIAN_POINT ( 'NONE',  ( 6.391743074199808916, 6.421731439513382433, -0.7998128361456481317 ) ) ;
#59122=CARTESIAN_POINT ( 'NONE',  ( 3.874598038455354665, 7.742391154831717692, -0.7998128361456362523 ) ) ;
#59132=CARTESIAN_POINT ( 'NONE',  ( 6.943184063974162434, 9.193743722760251202, -1.443375672974064550 ) ) ;
#59133=CARTESIAN_POINT ( 'NONE',  ( -3.662110889467009578, 7.286563447771212232, 0.7216878364870338292 ) ) ;
#59135=CARTESIAN_POINT ( 'NONE',  ( -7.435720902452096936, 7.639705572474380091, 0.000000000000000000 ) ) ;
#59143=CARTESIAN_POINT ( 'NONE',  ( 3.719872605471085336, 6.605953636083950364, 2.420000000000000373 ) ) ;
#59147=CARTESIAN_POINT ( 'NONE',  ( 4.667750024854814050, 8.667735138964429709, -0.7998128361456381397 ) ) ;
#59148=CARTESIAN_POINT ( 'NONE',  ( 7.062871678076271920, 7.204714810702593120, -0.7998128361456341429 ) ) ;
#59151=CARTESIAN_POINT ( 'NONE',  ( 5.356880090730874677, 5.422317325373725794, 0.7216878364870328300 ) ) ;
#59167=CARTESIAN_POINT ( 'NONE',  ( 4.492547798081839794, 6.334668079219206049, 1.599625672291262513 ) ) ;
#59171=CARTESIAN_POINT ( 'NONE',  ( 5.387385936583818591, 7.378645907471495846, -1.599625672291283607 ) ) ;
#59175=CARTESIAN_POINT ( 'NONE',  ( 5.993586425693011144, 9.150212042353954800, -1.199719254218452047 ) ) ;
#59176=DIRECTION ( 'NONE',  ( -0.9446243521954068578, 0.000000000000000000, -0.3281536732072456997 ) ) ;
#59184=CARTESIAN_POINT ( 'NONE',  ( 4.855228407469603269, 7.718164671139588151, -1.082531754730548412 ) ) ;
#59186=CARTESIAN_POINT ( 'NONE',  ( -5.224688093219839402, 7.188831756880171397, -1.599625672291271394 ) ) ;
#59187=CARTESIAN_POINT ( 'NONE',  ( 4.390861645979372341, 6.216034235099629157, -1.599625672291269396 ) ) ;
#59196=CARTESIAN_POINT ( 'NONE',  ( -4.502189528189771472, 7.410248995266807803, -1.199719254218453823 ) ) ;
#59223=ORIENTED_EDGE ( 'NONE', *, *, #101206, .T. ) ;
#59227=CARTESIAN_POINT ( 'NONE',  ( 6.831329296439236032, 9.063246493969506545, -1.599625672291267398 ) ) ;
#59228=CARTESIAN_POINT ( 'NONE',  ( 3.051993976407674225, 6.574760382535328240, -0.7216878364870338292 ) ) ;
#59239=CARTESIAN_POINT ( 'NONE',  ( -5.601453741101424022, 6.564059448486966986, -1.199719254218453823 ) ) ;
#59242=CARTESIAN_POINT ( 'NONE',  ( -4.776215253764153346, 8.794277906025310898, -0.7998128361456362523 ) ) ;
#59244=CARTESIAN_POINT ( 'NONE',  ( 5.994113310573177422, 10.00723293906178846, 0.000000000000000000 ) ) ;
#59246=CARTESIAN_POINT ( 'NONE',  ( -3.783109326081552037, 7.353282959184841872, -0.6894747432927388342 ) ) ;
#59253=CARTESIAN_POINT ( 'NONE',  ( -5.204350862799341115, 7.165104988056252289, -1.599625672291271394 ) ) ;
#59261=CARTESIAN_POINT ( 'NONE',  ( -5.533136088152923904, 6.588318536667425285, 1.082531754730549078 ) ) ;
#59266=CARTESIAN_POINT ( 'NONE',  ( -4.437261413422502798, 8.398831758960053406, 0.000000000000000000 ) ) ;
#59290=CARTESIAN_POINT ( 'NONE',  ( -5.108390017298964914, 9.181815130149269422, 0.000000000000000000 ) ) ;
#59292=CARTESIAN_POINT ( 'NONE',  ( -3.305155586681401303, 7.078041627762083898, 0.7998128361456352531 ) ) ;
#59305=ORIENTED_EDGE ( 'NONE', *, *, #185371, .T. ) ;
#59321=CARTESIAN_POINT ( 'NONE',  ( -5.956828388357799042, 8.042995434541133193, 1.599625672291263179 ) ) ;
#59349=CARTESIAN_POINT ( 'NONE',  ( 4.505052181490820651, 8.477920988373101707, -0.7998128361456381397 ) ) ;
#59362=CARTESIAN_POINT ( 'NONE',  ( 5.542547785767838242, 7.428594929708664196, 1.247761615041423244 ) ) ;
#59365=CARTESIAN_POINT ( 'NONE',  ( 7.187230829020129441, 8.518095734345896730, 1.082531754730549967 ) ) ;
#59372=CARTESIAN_POINT ( 'NONE',  ( -6.310394152517827315, 6.326824364217716656, 0.7998128361456281477 ) ) ;
#59381=CARTESIAN_POINT ( 'NONE',  ( -4.787437638956920871, 8.599444655509458357, -0.7216878364870338292 ) ) ;
#59382=CARTESIAN_POINT ( 'NONE',  ( -1.833030277982348411, 0.000000000000000000, 2.500000000000000444 ) ) ;
#59400=CARTESIAN_POINT ( 'NONE',  ( 8.018721507839716267, 8.319872945426633137, -0.7998128361456341429 ) ) ;
#59416=DIRECTION ( 'NONE',  ( -0.5620411653108187133, 0.8271092603133257670, -5.421010862427498504E-15 ) ) ;
#59418=ORIENTED_EDGE ( 'NONE', *, *, #4565, .T. ) ;
#59419=CARTESIAN_POINT ( 'NONE',  ( -7.045397100956844127, 8.248660034984974132, -1.199719254218452047 ) ) ;
#59421=CARTESIAN_POINT ( 'NONE',  ( 6.475954649182838807, 7.584310507915338562, 1.199719254218452047 ) ) ;
#59432=CARTESIAN_POINT ( 'NONE',  ( 4.509216530447271332, 8.500000000000010658, -0.05037230876976211968 ) ) ;
#59441=CARTESIAN_POINT ( 'NONE',  ( 4.421367491832258523, 8.172362817197399210, 0.7216878364870257245 ) ) ;
#59453=CARTESIAN_POINT ( 'NONE',  ( -5.072158865288277418, 7.010880990960010273, 1.443375672974058777 ) ) ;
#59456=CARTESIAN_POINT ( 'NONE',  ( 2.977454500823585093, 6.499579965040511276, -0.5808385047149626779 ) ) ;
#59461=DIRECTION ( 'NONE',  ( 0.000000000000000000, 0.000000000000000000, 1.000000000000000000 ) ) ;
#59462=DIRECTION ( 'NONE',  ( -0.6507913734559688246, -0.7592566023652963514, 0.000000000000000000 ) ) ;
#59483=CARTESIAN_POINT ( 'NONE',  ( 4.903208829997618423, 5.749440385532527564, -1.199719254218450271 ) ) ;
#59493=CARTESIAN_POINT ( 'NONE',  ( -5.587368702607575344, 8.572328348800551723, 1.082531754730550855 ) ) ;
#59495=CARTESIAN_POINT ( 'NONE',  ( 4.380693030546916944, 6.204170850428461392, 1.443375672974058777 ) ) ;
#59515=CARTESIAN_POINT ( 'NONE',  ( 2.969872605471108873, 6.605953636083950364, -2.420000000000002149 ) ) ;
#59543=CARTESIAN_POINT ( 'NONE',  ( -6.071018923869249129, 10.30488218781460574, 0.7998128361456291469 ) ) ;
#59547=CARTESIAN_POINT ( 'NONE',  ( -7.273023059088104425, 7.449891421883056530, 0.000000000000000000 ) ) ;
#59548=CARTESIAN_POINT ( 'NONE',  ( -5.764151584465413869, 6.753873599078290546, -1.199719254218453823 ) ) ;
#59549=CARTESIAN_POINT ( 'NONE',  ( -5.698737662929126202, 7.345098442806643924, 1.271001439489399809 ) ) ;
#59552=CARTESIAN_POINT ( 'NONE',  ( -7.390603132780795725, 8.755363422066633206, -1.082531754730549967 ) ) ;
#59553=CARTESIAN_POINT ( 'NONE',  ( 7.471952054462754234, 8.850270497362297206, 1.082531754730549078 ) ) ;
#59555=FACE_OUTER_BOUND ( 'NONE', #61720, .T. ) ;
#59559=CARTESIAN_POINT ( 'NONE',  ( -4.522526758610270647, 7.433975764090723359, -1.199719254218453823 ) ) ;
#59564=ORIENTED_EDGE ( 'NONE', *, *, #6657, .F. ) ;
#59575=CARTESIAN_POINT ( 'NONE',  ( 5.682802662783380754, 6.658966523782627434, 1.199719254218452935 ) ) ;
#59581=ORIENTED_EDGE ( 'NONE', *, *, #134736, .T. ) ;
#59599=CARTESIAN_POINT ( 'NONE',  ( 4.692003678781083487, 7.631698837623355658, -1.199719254218450271 ) ) ;
#59600=CARTESIAN_POINT ( 'NONE',  ( 3.562760505341037831, 7.378580699531681830, -1.734723475976807094E-15 ) ) ;
#59616=CARTESIAN_POINT ( 'NONE',  ( 6.598740849494261873, 6.770918179921630475, -0.1579934589533253664 ) ) ;
#59618=CARTESIAN_POINT ( 'NONE',  ( -3.472296738431328134, 7.065113604896248845, 0.000000000000000000 ) ) ;
#59619=CARTESIAN_POINT ( 'NONE',  ( -3.128512303076027123, 6.140441835863033049, 0.8630319677947241308 ) ) ;
#59645=CARTESIAN_POINT ( 'NONE',  ( 2.891631901464575272, 6.595597328342462262, 0.000000000000000000 ) ) ;
#59652=EDGE_CURVE ( 'NONE', #52415, #24930, #84973, .T. ) ;
#59664=CARTESIAN_POINT ( 'NONE',  ( -6.282224075085783177, 8.422623735723785643, 1.599625672291269396 ) ) ;
#59673=ORIENTED_EDGE ( 'NONE', *, *, #156259, .T. ) ;
#59678=CARTESIAN_POINT ( 'NONE',  ( 5.734172623936983904, 5.654565914206774124, 0.7998128361456352531 ) ) ;
#59687=CARTESIAN_POINT ( 'NONE',  ( 4.789099507923308963, 8.141322699134850183, 0.8117711051834965996 ) ) ;
#59690=CARTESIAN_POINT ( 'NONE',  ( 1.833030277982334422, 2.531131934864056632, -2.500000000000000444 ) ) ;
#59694=CARTESIAN_POINT ( 'NONE',  ( -3.824766175154623582, 7.348582304423016964, -0.7466790275774716212 ) ) ;
#59710=CARTESIAN_POINT ( 'NONE',  ( -6.330731382938325602, 6.350551133041632212, 0.7998128361456281477 ) ) ;
#59712=CARTESIAN_POINT ( 'NONE',  ( 4.549643065837591038, 7.465611455855944101, -1.199719254218452047 ) ) ;
#59713=CARTESIAN_POINT ( 'NONE',  ( 0.000000000000000000, 8.920000000000001705, 0.000000000000000000 ) ) ;
#59717=CARTESIAN_POINT ( 'NONE',  ( -5.855142236255304944, 7.924361590421551860, -1.599625672291271394 ) ) ;
#59726=CARTESIAN_POINT ( 'NONE',  ( -5.233950224509621663, 7.808013953112580730, -1.290304472045332496 ) ) ;
#59744=CARTESIAN_POINT ( 'NONE',  ( 4.909461021924244051, 6.821066840368686712, 1.443375672974065660 ) ) ;
#59747=CARTESIAN_POINT ( 'NONE',  ( -7.425025402139490360, 8.691559719698066289, 1.199719254218452047 ) ) ;
#59756=CARTESIAN_POINT ( 'NONE',  ( -4.855228407469635243, 4.837057028235559386, 0.7216878364870257245 ) ) ;
#59761=CARTESIAN_POINT ( 'NONE',  ( 3.888156192069020634, 7.758209000714329839, 1.040834085586084257E-14 ) ) ;
#59777=B_SPLINE_CURVE_WITH_KNOTS ( 'NONE', 3,
 ( #131334, #197328, #143301, #127096 ),
 .UNSPECIFIED., .F., .F.,
 ( 4, 4 ),
 ( 0.000000000000000000, 0.0007228752909667262921 ),
 .UNSPECIFIED. ) ;
#59802=EDGE_LOOP ( 'NONE', ( #205695, #113982, #71531, #28758 ) ) ;
#59815=CARTESIAN_POINT ( 'NONE',  ( -4.136646265500970365, 5.919449624541475607, -1.443375672974066548 ) ) ;
#59822=CARTESIAN_POINT ( 'NONE',  ( -3.149236820124241110, 6.896136400112061970, -0.7998128361456481317 ) ) ;
#59830=CARTESIAN_POINT ( 'NONE',  ( -5.978219388983010418, 5.939287140093762574, -0.7998128361456362523 ) ) ;
#59832=CARTESIAN_POINT ( 'NONE',  ( 5.662876554447811017, 7.443216037249618999, -1.326882488215734845 ) ) ;
#59836=CARTESIAN_POINT ( 'NONE',  ( 3.555981428534177091, 7.370671776590375757, 0.7998128361456271485 ) ) ;
#59842=CARTESIAN_POINT ( 'NONE',  ( -8.086512275908061653, 8.398962174839683215, 0.000000000000000000 ) ) ;
#59847=CARTESIAN_POINT ( 'NONE',  ( -6.147696309153835692, 6.137010213626392208, 0.7998128361456281477 ) ) ;
#59851=CARTESIAN_POINT ( 'NONE',  ( 5.858531774436539052, 6.007577623030311287, 0.000000000000000000 ) ) ;
#59852=CARTESIAN_POINT ( 'NONE',  ( -5.980555156959541208, 7.110307450275150210, 1.082531754730549078 ) ) ;
#59856=CARTESIAN_POINT ( 'NONE',  ( -5.207729805571693404, 7.804368671438548510, -1.360913387355301207 ) ) ;
#59860=CARTESIAN_POINT ( 'NONE',  ( 3.770049233051776749, 6.556085317605844232, 1.199719254218451159 ) ) ;
#59868=CARTESIAN_POINT ( 'NONE',  ( 5.204350862799327793, 7.165104988056252289, -1.599625672291281386 ) ) ;
#59890=CARTESIAN_POINT ( 'NONE',  ( 4.646267551848549004, 8.309382712783076386, 0.4446711254955729165 ) ) ;
#59897=CARTESIAN_POINT ( 'NONE',  ( 7.340813827156391191, 7.528980651296110160, 0.7998128361456281477 ) ) ;
#59902=CARTESIAN_POINT ( 'NONE',  ( -4.652699544748355898, 8.322425126176462129, -0.4365168051920116365 ) ) ;
#59907=CARTESIAN_POINT ( 'NONE',  ( -5.935437387732586778, 10.14670372898850381, -0.7998128361456362523 ) ) ;
#59919=CARTESIAN_POINT ( 'NONE',  ( 5.203297092594585393, 9.292540051327542017, 0.7998128361456341429 ) ) ;
#59924=CARTESIAN_POINT ( 'NONE',  ( 7.065207446497155708, 9.336104335703744539, 0.000000000000000000 ) ) ;
#59929=CARTESIAN_POINT ( 'NONE',  ( 2.905190055078214595, 6.611415174225076186, 0.7998128361456271485 ) ) ;
#59932=CARTESIAN_POINT ( 'NONE',  ( 4.489158259456265121, 7.291082831790689056, -1.082531754730548412 ) ) ;
#59939=AXIS2_PLACEMENT_3D ( 'NONE', #82112, #49620, #148205 ) ;
#59941=CARTESIAN_POINT ( 'NONE',  ( -5.568215224448921141, 7.423109701660543180, 1.245465753432648093 ) ) ;
#59947=CARTESIAN_POINT ( 'NONE',  ( -4.146814880933400005, 5.931313009212638931, 1.599625672291270506 ) ) ;
#59948=CARTESIAN_POINT ( 'NONE',  ( 7.512626515748113576, 7.937354821227203594, 0.7216878364870267237 ) ) ;
#59961=CARTESIAN_POINT ( 'NONE',  ( -6.947627372360122955, 7.070263120700404968, 0.000000000000000000 ) ) ;
#59962=CARTESIAN_POINT ( 'NONE',  ( -5.123001941117347080, 7.070197912760590064, 1.599625672291263179 ) ) ;
#59964=CARTESIAN_POINT ( 'NONE',  ( 5.682275777458829502, 9.643422483761748154, 0.7216878364870317197 ) ) ;
#59976=CARTESIAN_POINT ( 'NONE',  ( -6.300768610526733760, 6.888587422923714954, -0.7334343799849201151 ) ) ;
#59977=FACE_BOUND ( 'NONE', #54233, .T. ) ;
#59981=CARTESIAN_POINT ( 'NONE',  ( 4.245111494854632461, 7.966730820723463502, 0.000000000000000000 ) ) ;
#59985=LINE ( 'NONE', #143415, #186772 ) ;
#59986=CARTESIAN_POINT ( 'NONE',  ( -5.661411662158206681, 8.762674818229999829, -1.199719254218452047 ) ) ;
#60002=CARTESIAN_POINT ( 'NONE',  ( 4.857564175446106525, 8.889184981320973122, 0.7998128361456331437 ) ) ;
#60037=CARTESIAN_POINT ( 'NONE',  ( 6.699137298928153683, 7.948653282571920720, 1.082531754730549967 ) ) ;
#60066=CARTESIAN_POINT ( 'NONE',  ( -3.332271893908731464, 7.109677319527304640, -0.7998128361456481317 ) ) ;
#60068=CARTESIAN_POINT ( 'NONE',  ( 5.356880090730863131, 7.343055753976412525, 1.443375672974064550 ) ) ;
#60073=CARTESIAN_POINT ( 'NONE',  ( -5.143339171537843590, 7.093924681584509173, 1.599625672291263179 ) ) ;
#60077=CARTESIAN_POINT ( 'NONE',  ( -4.146814880933400005, 5.931313009212638931, 1.599625672291270506 ) ) ;
#60084=CARTESIAN_POINT ( 'NONE',  ( -5.041653019435350380, 6.975290837464928728, -1.599625672291271394 ) ) ;
#60094=CARTESIAN_POINT ( 'NONE',  ( -5.171509248969888617, 4.998125310078441075, 0.7998128361456281477 ) ) ;
#60099=CARTESIAN_POINT ( 'NONE',  ( -6.021229618244897885, 7.157760988441397743, 1.082531754730548412 ) ) ;
#60100=CARTESIAN_POINT ( 'NONE',  ( -5.275531169048909952, 7.248148678680751189, -1.443375672974066548 ) ) ;
#60101=CARTESIAN_POINT ( 'NONE',  ( 6.547661840756936691, 6.603636667163397256, 0.7998128361456352531 ) ) ;
#60103=CARTESIAN_POINT ( 'NONE',  ( -5.661411662158206681, 8.762674818229999829, -1.199719254218452047 ) ) ;
#60121=CARTESIAN_POINT ( 'NONE',  ( 5.989670002187236442, 10.20997511251894529, -0.7998128361456481317 ) ) ;
#60140=CARTESIAN_POINT ( 'NONE',  ( 4.601768607255383614, 8.481659704624913587, -0.1707596084408805059 ) ) ;
#60155=CARTESIAN_POINT ( 'NONE',  ( 6.713222337422018349, 7.861122810861019161, -1.199719254218452047 ) ) ;
#60158=( BOUNDED_CURVE ( )  B_SPLINE_CURVE ( 2, ( #170233, #5565, #205927, #105260, #171301 ),
 .UNSPECIFIED., .F., .T. ) 
 B_SPLINE_CURVE_WITH_KNOTS ( ( 3, 2, 3 ),
 ( 0.000000000000000000, 0.5732952876205078541, 1.000000000000000000 ),
 .UNSPECIFIED. ) 
 CURVE ( )  GEOMETRIC_REPRESENTATION_ITEM ( )  RATIONAL_B_SPLINE_CURVE ( ( 0.9706336853805221931, 0.9832135787375378966, 1.000000000000000000, 0.9875058365010993544, 0.9773420270535906340 ) ) 
 REPRESENTATION_ITEM ( '' )  );
#60159=CARTESIAN_POINT ( 'NONE',  ( -3.305155586681401303, 7.078041627762083898, 0.7998128361456352531 ) ) ;
#60162=CARTESIAN_POINT ( 'NONE',  ( -6.495764994278840021, 8.671754808115688107, 1.443375672974064550 ) ) ;
#60173=CARTESIAN_POINT ( 'NONE',  ( 7.828907357248368726, 8.098423103070084395, 0.7998128361456281477 ) ) ;
#60174=CARTESIAN_POINT ( 'NONE',  ( 4.342354338126830804, 8.288106837781779035, -0.7998128361456381397 ) ) ;
#60186=CARTESIAN_POINT ( 'NONE',  ( 4.877901405866606588, 8.912911750144889567, 0.7998128361456341429 ) ) ;
#60193=CARTESIAN_POINT ( 'NONE',  ( 0.000000000000000000, 8.999999999999998224, 0.000000000000000000 ) ) ;
#60198=CARTESIAN_POINT ( 'NONE',  ( -4.746763178560296836, 6.631252689777363152, 1.443375672974058777 ) ) ;
#60199=CARTESIAN_POINT ( 'NONE',  ( -6.668631453075260396, 8.873432343378178544, -1.599625672291271394 ) ) ;
#60211=CARTESIAN_POINT ( 'NONE',  ( 4.694866332082116678, 8.699370830729650450, 0.7998128361456341429 ) ) ;
#60212=CARTESIAN_POINT ( 'NONE',  ( 7.361151057576892143, 7.552707420120024828, 0.7998128361456291469 ) ) ;
#60215=CARTESIAN_POINT ( 'NONE',  ( 4.882344714252594642, 4.868692719482363707, 0.000000000000000000 ) ) ;
#60231=DIRECTION ( 'NONE',  ( -0.6507913734559641616, -0.7592566023653004592, 0.000000000000000000 ) ) ;
#60234=CARTESIAN_POINT ( 'NONE',  ( 3.223806664999388172, 6.983134552466421674, -0.7998128361456362523 ) ) ;
#60239=CARTESIAN_POINT ( 'NONE',  ( 4.980641328173811999, 6.904110530993182948, 1.599625672291269396 ) ) ;
#60251=CARTESIAN_POINT ( 'NONE',  ( 6.943184063974162434, 9.193743722760251202, -1.443375672974064550 ) ) ;
#60253=CARTESIAN_POINT ( 'NONE',  ( -6.794571259104023930, 7.956029886156682274, 1.199719254218452047 ) ) ;
#60254=CARTESIAN_POINT ( 'NONE',  ( 5.337069745634900997, 6.255611453776062980, 1.199719254218452047 ) ) ;
#60255=VERTEX_POINT ( 'NONE', #165586 ) ;
#60261=CARTESIAN_POINT ( 'NONE',  ( -4.118112554246268431, 7.605586660457912984, -0.5892100532764152909 ) ) ;
#60264=CARTESIAN_POINT ( 'NONE',  ( -5.483346782084204563, 5.361935765378481378, 0.000000000000000000 ) ) ;
#60292=VECTOR ( 'NONE', #56384, 1000.000000000000000 ) ;
#60298=CARTESIAN_POINT ( 'NONE',  ( 3.892599500454941630, 6.595097612955829192, 1.082531754730549078 ) ) ;
#60308=CARTESIAN_POINT ( 'NONE',  ( -5.167592825464113915, 6.057888380243431570, 1.199719254218452935 ) ) ;
#60310=CARTESIAN_POINT ( 'NONE',  ( -6.947627372360122955, 7.070263120700404968, 0.000000000000000000 ) ) ;
#60321=CARTESIAN_POINT ( 'NONE',  ( -6.608673532018475960, 6.674816973635147477, -0.7998128361456362523 ) ) ;
#60328=CARTESIAN_POINT ( 'NONE',  ( -5.641601317062248988, 6.714861303728305586, -1.082531754730549967 ) ) ;
#60332=CARTESIAN_POINT ( 'NONE',  ( -4.990283058281743678, 7.979691447040783814, -1.199719254218453823 ) ) ;
#60353=CARTESIAN_POINT ( 'NONE',  ( -5.769876891067536206, 8.889217585290882795, 1.199719254218454489 ) ) ;
#60356=CARTESIAN_POINT ( 'NONE',  ( -4.145761110728687804, 8.058748072483927771, -0.7998128361456481317 ) ) ;
#60365=CARTESIAN_POINT ( 'NONE',  ( 6.021229617800532452, 6.197391773621639288, 0.000000000000000000 ) ) ;
#60366=CARTESIAN_POINT ( 'NONE',  ( -5.179808110042967151, 6.342388681160900710, -1.197525655462832406 ) ) ;
#60381=CARTESIAN_POINT ( 'NONE',  ( -6.577640801285370209, 7.702944352034914566, -1.199719254218452047 ) ) ;
#60406=ADVANCED_FACE ( 'NONE', ( #98458, #181817 ), #150421, .F. ) ;
#60411=CARTESIAN_POINT ( 'NONE',  ( 6.505933609711257226, 8.683618192786854095, -1.599625672291281386 ) ) ;
#60425=CARTESIAN_POINT ( 'NONE',  ( 6.059270238282111087, 7.038290852966752276, 1.014332888565868229 ) ) ;
#60427=CARTESIAN_POINT ( 'NONE',  ( 5.560252395380206103, 8.540692657035327429, 1.082531754730547524 ) ) ;
#60433=CARTESIAN_POINT ( 'NONE',  ( -3.962726036944197894, 7.845207153068690431, -0.7998128361456481317 ) ) ;
#60440=CARTESIAN_POINT ( 'NONE',  ( -5.600926855776882540, 8.588146194164741232, -1.082531754730549967 ) ) ;
#60445=CARTESIAN_POINT ( 'NONE',  ( 5.671053392266061977, 9.838255734277600695, 0.7998128361456331437 ) ) ;
#60451=CARTESIAN_POINT ( 'NONE',  ( -4.821859908315634158, 5.654533310236863564, 1.199719254218452935 ) ) ;
#60461=CARTESIAN_POINT ( 'NONE',  ( 3.923105346307896202, 5.670318552149568703, -1.599625672291269396 ) ) ;
#60467=DIRECTION ( 'NONE',  ( 0.000000000000000000, 0.000000000000000000, -1.000000000000000000 ) ) ;
#60478=CARTESIAN_POINT ( 'NONE',  ( -7.099629715411508890, 8.311931418515415615, 1.199719254218452047 ) ) ;
#60480=CARTESIAN_POINT ( 'NONE',  ( 5.006703865196457492, 9.063181286029688977, 0.000000000000000000 ) ) ;
#60482=CIRCLE ( 'NONE', #91613, 0.8299999999999999600 ) ;
#60489=CARTESIAN_POINT ( 'NONE',  ( 5.825163275726873202, 6.825053905550038991, 1.199719254218452047 ) ) ;
#60496=CARTESIAN_POINT ( 'NONE',  ( 3.268924434670684498, 6.827845917175511481, -1.734723475976807094E-15 ) ) ;
#60500=CARTESIAN_POINT ( 'NONE',  ( 6.373741612200174878, 6.608655767087927124, 0.7216878364870328300 ) ) ;
#60501=ORIENTED_EDGE ( 'NONE', *, *, #129048, .F. ) ;
#60511=CARTESIAN_POINT ( 'NONE',  ( -5.316205630334255972, 8.255971431148344308, -1.082531754730549967 ) ) ;
#60517=CARTESIAN_POINT ( 'NONE',  ( 2.975337776247584998, 6.515577267086843705, -0.5540753762497061530 ) ) ;
#60523=CYLINDRICAL_SURFACE ( 'NONE', #112420, 0.4000000000000001332 ) ;
#60547=CARTESIAN_POINT ( 'NONE',  ( 5.415556014015861841, 5.282846535965431300, -0.7998128361456481317 ) ) ;
#60559=CARTESIAN_POINT ( 'NONE',  ( -7.268579750702168774, 7.652633595340216921, -0.7216878364870338292 ) ) ;
#60561=CARTESIAN_POINT ( 'NONE',  ( 4.923019175093585886, 5.876515471431535076, -1.082531754730548412 ) ) ;
#60580=CARTESIAN_POINT ( 'NONE',  ( -4.556949027968976829, 5.449433633119473264, 1.082531754730549078 ) ) ;
#60586=CARTESIAN_POINT ( 'NONE',  ( -5.060975816087005974, 7.500583322029065414, -1.217465846647723282 ) ) ;
#60613=CARTESIAN_POINT ( 'NONE',  ( -7.632314129850253259, 7.869064337772231355, 0.7998128361456341429 ) ) ;
#60616=CARTESIAN_POINT ( 'NONE',  ( -6.882699257592852504, 8.058845884393651460, -1.199719254218452047 ) ) ;
#60617=CARTESIAN_POINT ( 'NONE',  ( -4.681723370323557454, 8.380211346474826684, 0.6239904028470877329 ) ) ;
#60624=CARTESIAN_POINT ( 'NONE',  ( -3.546339698426324460, 6.295090860542775779, -1.199719254218450271 ) ) ;
#60627=CARTESIAN_POINT ( 'NONE',  ( -4.411198876399886615, 6.239761003923544713, -1.599625672291271394 ) ) ;
#60641=CARTESIAN_POINT ( 'NONE',  ( 5.734172623936983904, 5.654565914206774124, 0.7998128361456352531 ) ) ;
#60662=CARTESIAN_POINT ( 'NONE',  ( 4.030516805012513082, 7.924296382481737844, 0.000000000000000000 ) ) ;
#60663=CARTESIAN_POINT ( 'NONE',  ( 4.573896719763862251, 6.429575154514868274, -1.599625672291273171 ) ) ;
#60665=CARTESIAN_POINT ( 'NONE',  ( 3.770049233051776749, 6.556085317605844232, 1.199719254218451159 ) ) ;
#60674=CARTESIAN_POINT ( 'NONE',  ( 0.4461838333974484927, 2.877219473291486640, 1.949594826320268481 ) ) ;
#60678=CARTESIAN_POINT ( 'NONE',  ( 4.595841027163160675, 8.489102040997540399, 0.04885061651019838302 ) ) ;
#60679=CARTESIAN_POINT ( 'NONE',  ( -4.787437638956935082, 6.678706226906775179, -1.443375672974066548 ) ) ;
#60707=CARTESIAN_POINT ( 'NONE',  ( 3.040771591214902259, 6.769593633051179005, -0.7998128361456362523 ) ) ;
#60726=CARTESIAN_POINT ( 'NONE',  ( -4.858757509019083543, 5.629766575900002401, -2.500000000000000444 ) ) ;
#60728=VERTEX_POINT ( 'NONE', #131247 ) ;
#60735=EDGE_LOOP ( 'NONE', ( #162963, #188874, #210804, #205757, #137240, #124223 ) ) ;
#60744=CARTESIAN_POINT ( 'NONE',  ( 4.817943484809818600, 6.714296380401858499, 1.599625672291269396 ) ) ;
#60755=B_SPLINE_CURVE_WITH_KNOTS ( 'NONE', 3,
 ( #105495, #43693, #188847, #156364 ),
 .UNSPECIFIED., .F., .F.,
 ( 4, 4 ),
 ( 0.001768109493081024492, 0.002022414007280575604 ),
 .UNSPECIFIED. ) ;
#60756=AXIS2_PLACEMENT_3D ( 'NONE', #76997, #75944, #158277 ) ;
#60757=CARTESIAN_POINT ( 'NONE',  ( 5.840936731490688594, 7.196517624969346549, 1.161314407385056313 ) ) ;
#60764=CARTESIAN_POINT ( 'NONE',  ( -3.951451420331601128, 7.320064228719081356, -0.7343074186010454252 ) ) ;
#60780=CARTESIAN_POINT ( 'NONE',  ( -4.633854640820660009, 8.628190524257904670, -0.7998128361456362523 ) ) ;
#60782=CARTESIAN_POINT ( 'NONE',  ( 3.888156192069020634, 7.758209000714329839, 1.040834085586084257E-14 ) ) ;
#60786=CARTESIAN_POINT ( 'NONE',  ( -5.738844160334429567, 9.917344963690652548, 0.000000000000000000 ) ) ;
#60794=CARTESIAN_POINT ( 'NONE',  ( -5.645675577465527617, 7.454724071444114308, -1.341317915573495334 ) ) ;
#60811=CARTESIAN_POINT ( 'NONE',  ( 4.855228407469603269, 7.718164671139588151, -1.082531754730548412 ) ) ;
#60830=CARTESIAN_POINT ( 'NONE',  ( 3.739016502318667445, 7.584212696005614873, 0.7998128361456271485 ) ) ;
#60881=CARTESIAN_POINT ( 'NONE',  ( -4.462041952228944730, 7.259447140025469203, -1.082531754730549967 ) ) ;
#60887=CARTESIAN_POINT ( 'NONE',  ( -5.581116510680924847, 6.540332679663050541, -1.199719254218453823 ) ) ;
#60892=ORIENTED_EDGE ( 'NONE', *, *, #76698, .T. ) ;
#60894=CARTESIAN_POINT ( 'NONE',  ( 3.147653791585693028, 8.999999999999998224, 2.419999999999999485 ) ) ;
#60897=CARTESIAN_POINT ( 'NONE',  ( -4.294900800479008574, 8.232744377192641849, 0.000000000000000000 ) ) ;
#60899=ORIENTED_EDGE ( 'NONE', *, *, #147535, .T. ) ;
#60900=CARTESIAN_POINT ( 'NONE',  ( 5.796475149741596056, 7.337953333587568849, -1.293683646293428913 ) ) ;
#60905=CARTESIAN_POINT ( 'NONE',  ( 6.017840079619279692, 8.114175741012878973, -1.599625672291281386 ) ) ;
#60911=CARTESIAN_POINT ( 'NONE',  ( -5.887983850084758330, 10.09134126839936840, 0.7998128361456291469 ) ) ;
#60917=CARTESIAN_POINT ( 'NONE',  ( -5.041653019435350380, 6.975290837464928728, -1.599625672291271394 ) ) ;
#60921=CARTESIAN_POINT ( 'NONE',  ( 4.041739190205284160, 7.729463131965888856, 0.000000000000000000 ) ) ;
#60923=CARTESIAN_POINT ( 'NONE',  ( -4.624739795592931912, 8.409630504918133909, -0.7216878364870338292 ) ) ;
#60931=CARTESIAN_POINT ( 'NONE',  ( 6.066347387471824781, 6.042103138330730872, -0.7998128361456481317 ) ) ;
#60937=CARTESIAN_POINT ( 'NONE',  ( 5.448397627845284141, 7.449826213943242514, 1.599625672291268286 ) ) ;
#60960=CARTESIAN_POINT ( 'NONE',  ( 4.943016831304842817, 7.975319854387232787, 1.017975537214605319 ) ) ;
#60967=CARTESIAN_POINT ( 'NONE',  ( 7.042534447655770080, 7.180988041878682004, -0.7998128361456341429 ) ) ;
#60968=ORIENTED_EDGE ( 'NONE', *, *, #86369, .F. ) ;
#60972=CARTESIAN_POINT ( 'NONE',  ( -4.807049873888117553, 8.139959938814184781, 0.8294007104595437774 ) ) ;
#60980=CARTESIAN_POINT ( 'NONE',  ( -4.950135482320939140, 4.947781948895412008, -0.7216878364870338292 ) ) ;
#60992=CARTESIAN_POINT ( 'NONE',  ( -4.625266680917477835, 5.425174544939014964, -1.199719254218453823 ) ) ;
#60994=CARTESIAN_POINT ( 'NONE',  ( 7.049313524462606395, 7.188896964819984525, 0.000000000000000000 ) ) ;
#61002=CARTESIAN_POINT ( 'NONE',  ( 5.727393547130178675, 5.646656991265468939, 0.000000000000000000 ) ) ;
#61004=CARTESIAN_POINT ( 'NONE',  ( 4.217995187182915551, 7.935095128439824563, 0.7216878364870257245 ) ) ;
#61013=CARTESIAN_POINT ( 'NONE',  ( -5.679286501732877745, 7.334821546209805199, 1.225395024417414103 ) ) ;
#61020=CARTESIAN_POINT ( 'NONE',  ( -5.147255595043616516, 6.034161611419515125, 1.199719254218452935 ) ) ;
#61021=CARTESIAN_POINT ( 'NONE',  ( 6.482206841109512396, 9.616306177052839743, -1.082531754730548412 ) ) ;
#61032=CARTESIAN_POINT ( 'NONE',  ( -5.250750630242457362, 9.347902511916677426, 0.000000000000000000 ) ) ;
#61033=CARTESIAN_POINT ( 'NONE',  ( -3.949167883330528372, 7.829389307186077396, 1.214306433183764966E-14 ) ) ;
#61035=CARTESIAN_POINT ( 'NONE',  ( 7.336370518326124746, 7.731722824234849689, -0.7216878364870317197 ) ) ;
#61047=CARTESIAN_POINT ( 'NONE',  ( -5.717536675473545493, 7.305230138711669596, -1.214019596050613492 ) ) ;
#61052=EDGE_CURVE ( 'NONE', #60728, #156131, #84555, .T. ) ;
#61057=CARTESIAN_POINT ( 'NONE',  ( -8.120407659942227241, 8.438506789546210030, 0.7998128361456341429 ) ) ;
#61073=CARTESIAN_POINT ( 'NONE',  ( 6.638652492546827766, 7.774124658506663010, 1.199719254218452047 ) ) ;
#61107=CARTESIAN_POINT ( 'NONE',  ( 4.415115299905642665, 5.179997933758551554, -1.199719254218450271 ) ) ;
#61135=CARTESIAN_POINT ( 'NONE',  ( -4.980641328173854632, 6.904110530993182948, 1.599625672291263179 ) ) ;
#61137=CARTESIAN_POINT ( 'NONE',  ( 4.516274566683592617, 8.283087737857252719, -0.7216878364870357165 ) ) ;
#61142=CARTESIAN_POINT ( 'NONE',  ( -5.224688093219839402, 7.188831756880171397, -1.599625672291271394 ) ) ;
#61147=CARTESIAN_POINT ( 'NONE',  ( -7.024532985656169792, 9.288650798055913427, 1.443375672974064550 ) ) ;
#61150=CARTESIAN_POINT ( 'NONE',  ( -1.833506991698480526, 2.501547993919093660, 2.496244204820596835 ) ) ;
#61155=CARTESIAN_POINT ( 'NONE',  ( -4.261005416444848315, 8.193199762486115034, 0.7998128361456352531 ) ) ;
#61165=CARTESIAN_POINT ( 'NONE',  ( -4.309512724297390740, 6.121127159803966933, 1.599625672291270506 ) ) ;
#61170=CARTESIAN_POINT ( 'NONE',  ( -6.305950844131887223, 6.529566537674873494, 0.000000000000000000 ) ) ;
#61171=CARTESIAN_POINT ( 'NONE',  ( -6.116136693096208887, 6.308116694799912771, 0.7216878364870257245 ) ) ;
#61172=CARTESIAN_POINT ( 'NONE',  ( 7.035755370848908896, 7.173079118937375931, 0.7998128361456352531 ) ) ;
#61173=CARTESIAN_POINT ( 'NONE',  ( -5.420227550413282636, 9.545625585449309725, 0.7998128361456291469 ) ) ;
#61193=CARTESIAN_POINT ( 'NONE',  ( 7.550965208168244125, 7.774157262476569130, -0.7998128361456341429 ) ) ;
#61213=CARTESIAN_POINT ( 'NONE',  ( 4.628438946891473726, 8.448539137754004003, 0.3726521946380862427 ) ) ;
#61228=CARTESIAN_POINT ( 'NONE',  ( 6.550524494058025837, 7.671308660269694712, -1.199719254218452047 ) ) ;
#61231=CARTESIAN_POINT ( 'NONE',  ( -5.178288325776719603, 5.006034233019745372, 0.000000000000000000 ) ) ;
#61235=CARTESIAN_POINT ( 'NONE',  ( -5.438229012412888252, 9.358701257874761481, -0.7216878364870338292 ) ) ;
#61245=CARTESIAN_POINT ( 'NONE',  ( 5.096939404094710468, 4.911127157724081371, 0.000000000000000000 ) ) ;
#61246=CARTESIAN_POINT ( 'NONE',  ( 6.475954649182838807, 7.584310507915338562, 1.199719254218452047 ) ) ;
#61259=ORIENTED_EDGE ( 'NONE', *, *, #208272, .T. ) ;
#61260=CARTESIAN_POINT ( 'NONE',  ( 5.417364897112183719, 8.477953592343014932, 1.199719254218451159 ) ) ;
#61270=DIRECTION ( 'NONE',  ( 0.000000000000000000, 1.000000000000000000, 0.000000000000000000 ) ) ;
#61273=CARTESIAN_POINT ( 'NONE',  ( -4.909461021924285795, 6.821066840368686712, 1.443375672974058777 ) ) ;
#61274=CARTESIAN_POINT ( 'NONE',  ( -7.370792787684826486, 8.628288336167626582, -1.199719254218452047 ) ) ;
#61283=CARTESIAN_POINT ( 'NONE',  ( 6.197485614778206475, 6.403023770095559009, -0.7216878364870318308 ) ) ;
#61288=CARTESIAN_POINT ( 'NONE',  ( 5.040599249230596435, 9.102725900736217568, 0.7998128361456341429 ) ) ;
#61291=CARTESIAN_POINT ( 'NONE',  ( 7.635176783151273128, 8.936736330878529699, 1.199719254218452935 ) ) ;
#61306=DIRECTION ( 'NONE',  ( -0.000000000000000000, -0.000000000000000000, -1.000000000000000000 ) ) ;
#61307=B_SPLINE_CURVE_WITH_KNOTS ( 'NONE', 3,
 ( #112292, #14701, #196671, #95999, #145831 ),
 .UNSPECIFIED., .F., .F.,
 ( 4, 1, 4 ),
 ( 8.741117365843281861E-19, 5.162781510639185282E-05, 0.0001032556302127828247 ),
 .UNSPECIFIED. ) ;
#61310=ADVANCED_FACE ( 'NONE', ( #202545 ), #120334, .T. ) ;
#61311=CARTESIAN_POINT ( 'NONE',  ( 6.170896192875352959, 7.228408975556602556, 1.199719254218453823 ) ) ;
#61317=CARTESIAN_POINT ( 'NONE',  ( 4.875038752565570732, 7.845239757038595663, -1.199719254218452047 ) ) ;
#61323=CARTESIAN_POINT ( 'NONE',  ( -6.966220764712169000, 6.002124920821316323, -2.420000000000000373 ) ) ;
#61327=EDGE_CURVE ( 'NONE', #9317, #209619, #48947, .T. ) ;
#61328=CARTESIAN_POINT ( 'NONE',  ( 6.156811154381533591, 9.236677875870187293, -1.082531754730548412 ) ) ;
#61330=CARTESIAN_POINT ( 'NONE',  ( -5.271087860662956537, 9.371629280740593870, 0.000000000000000000 ) ) ;
#61331=CARTESIAN_POINT ( 'NONE',  ( 4.258142763143749399, 7.125527769379820242, 1.199719254218451159 ) ) ;
#61341=CARTESIAN_POINT ( 'NONE',  ( -5.469788628470539926, 5.346117919495872783, -0.7998128361456362523 ) ) ;
#61359=ADVANCED_FACE ( 'NONE', ( #39014 ), #8631, .T. ) ;
#61370=CARTESIAN_POINT ( 'NONE',  ( 4.014622883422321209, 5.777089012116397804, -1.443375672974068769 ) ) ;
#61377=CARTESIAN_POINT ( 'NONE',  ( 5.854088466050551887, 10.05179665369283981, 0.7998128361456341429 ) ) ;
#61387=CARTESIAN_POINT ( 'NONE',  ( -6.168033539574333979, 6.160736982450306876, 0.7998128361456281477 ) ) ;
#61389=CARTESIAN_POINT ( 'NONE',  ( -8.072954122294394352, 8.383144328957069291, -0.7998128361456362523 ) ) ;
#61391=CARTESIAN_POINT ( 'NONE',  ( 6.007671464186823407, 9.062681570643055906, 1.082531754730549967 ) ) ;
#61398=CARTESIAN_POINT ( 'NONE',  ( 3.231779075379137556, 6.036511184309971689, -2.420000000000002149 ) ) ;
#61399=CARTESIAN_POINT ( 'NONE',  ( -4.274563570058511175, 8.209017608368725405, 0.000000000000000000 ) ) ;
#61406=CARTESIAN_POINT ( 'NONE',  ( -4.882344714696960075, 5.829061934302122161, 1.082531754730549078 ) ) ;
#61410=CARTESIAN_POINT ( 'NONE',  ( -3.800028193580205382, 7.655393002477360653, -0.7998128361456481317 ) ) ;
#61427=CARTESIAN_POINT ( 'NONE',  ( -7.632314129850253259, 7.869064337772231355, 0.7998128361456341429 ) ) ;
#61429=CARTESIAN_POINT ( 'NONE',  ( -3.467853430045390706, 7.267855778353407459, 0.7998128361456352531 ) ) ;
#61454=CARTESIAN_POINT ( 'NONE',  ( -7.144220599758281054, 7.299621885998258897, 0.7998128361456341429 ) ) ;
#61481=CARTESIAN_POINT ( 'NONE',  ( 8.174640274396848483, 8.501778173076651512, 0.7998128361456291469 ) ) ;
#61483=CARTESIAN_POINT ( 'NONE',  ( 6.994027139803230320, 9.253060644560830994, -1.599625672291267398 ) ) ;
#61495=CARTESIAN_POINT ( 'NONE',  ( 4.920187338115698417, 7.999083482620499730, 0.9937779052983791717 ) ) ;
#61497=CARTESIAN_POINT ( 'NONE',  ( 6.699137298928153683, 7.948653282571920720, 1.082531754730549967 ) ) ;
#61504=CARTESIAN_POINT ( 'NONE',  ( -5.472651281771599763, 6.413789912602166687, 1.199719254218452935 ) ) ;
#61512=CARTESIAN_POINT ( 'NONE',  ( -5.099275172071237705, 8.963255110809500437, 0.000000000000000000 ) ) ;
#61521=CARTESIAN_POINT ( 'NONE',  ( -4.995253251992230581, 4.792493313604505367, 0.000000000000000000 ) ) ;
#61531=CARTESIAN_POINT ( 'NONE',  ( 7.693325821111733021, 7.940244644243982464, -0.7998128361456341429 ) ) ;
#61551=CARTESIAN_POINT ( 'NONE',  ( -7.923814432544069142, 8.209148024248356990, 0.000000000000000000 ) ) ;
#61552=EDGE_CURVE ( 'NONE', #17896, #204026, #16940, .T. ) ;
#61553=CARTESIAN_POINT ( 'NONE',  ( -3.824766175154623582, 7.348582304423016964, -0.7466790275774716212 ) ) ;
#61554=CARTESIAN_POINT ( 'NONE',  ( 5.936491157937257235, 8.019268665717216749, 1.599625672291268286 ) ) ;
#61556=CARTESIAN_POINT ( 'NONE',  ( -5.333877144031607287, 7.620261487198364492, 1.234409035313356107 ) ) ;
#61563=CARTESIAN_POINT ( 'NONE',  ( 5.367048706163317640, 7.354919138647580290, -1.599625672291281386 ) ) ;
#61566=CARTESIAN_POINT ( 'NONE',  ( -5.561826481650498977, 5.891466595178788346, -0.7788020862528137744 ) ) ;
#61571=CARTESIAN_POINT ( 'NONE',  ( 3.119784744920330422, 6.653849612466795627, 0.7216878364870257245 ) ) ;
#61574=CARTESIAN_POINT ( 'NONE',  ( 5.478903473698239601, 7.485416367438324059, -1.443375672974078761 ) ) ;
#61575=ORIENTED_EDGE ( 'NONE', *, *, #13673, .F. ) ;
#61582=DIRECTION ( 'NONE',  ( 0.6507913734559640506, -0.7592566023653003482, 0.000000000000000000 ) ) ;
#61585=CARTESIAN_POINT ( 'NONE',  ( -5.966997003790232235, 7.094489604910957148, -1.082531754730549967 ) ) ;
#61602=CARTESIAN_POINT ( 'NONE',  ( 4.370663978927085580, 5.060324124126027279, 7.500000000000000000 ) ) ;
#61618=CARTESIAN_POINT ( 'NONE',  ( 5.285699784481295183, 7.260012063351913625, 1.599625672291268286 ) ) ;
#61633=CARTESIAN_POINT ( 'NONE',  ( -6.292392690518202159, 9.394856334696294553, -1.082531754730549967 ) ) ;
#61636=CARTESIAN_POINT ( 'NONE',  ( 4.895902867866261055, 4.884510565364971413, -0.7216878364870458196 ) ) ;
#61660=CARTESIAN_POINT ( 'NONE',  ( 3.553238514845298734, 7.337208092372121904, -0.2327671511505452484 ) ) ;
#61661=CIRCLE ( 'NONE', #141333, 4.022469383779238683 ) ;
#61690=CARTESIAN_POINT ( 'NONE',  ( -5.586845290032572464, 7.502486493224762576, 1.347716017753825879 ) ) ;
#61693=ORIENTED_EDGE ( 'NONE', *, *, #40364, .T. ) ;
#61695=FACE_OUTER_BOUND ( 'NONE', #7848, .T. ) ;
#61698=CARTESIAN_POINT ( 'NONE',  ( -3.709037541790315640, 6.484905011134099340, -1.199719254218450271 ) ) ;
#61701=AXIS2_PLACEMENT_3D ( 'NONE', #103577, #169635, #21218 ) ;
#61702=CARTESIAN_POINT ( 'NONE',  ( -3.806807270387036368, 7.663301925418665839, 0.000000000000000000 ) ) ;
#61707=EDGE_LOOP ( 'NONE', ( #109469, #90878, #70491, #174290 ) ) ;
#61715=CARTESIAN_POINT ( 'NONE',  ( 3.711900195091365262, 7.552577004240394132, -0.7998128361456362523 ) ) ;
#61720=EDGE_LOOP ( 'NONE', ( #152806, #144072, #89534, #145480, #137481, #49975, #107044, #86703, #98395, #122164, #23423, #82378, #145777, #10814, #5844, #115042 ) ) ;
#61739=CARTESIAN_POINT ( 'NONE',  ( 4.505052181490820651, 8.477920988373101707, -0.7998128361456381397 ) ) ;
#61740=CARTESIAN_POINT ( 'NONE',  ( 4.706615602599436343, 5.520081620234675412, 1.199719254218452935 ) ) ;
#61747=FACE_OUTER_BOUND ( 'NONE', #170195, .T. ) ;
#61752=VERTEX_POINT ( 'NONE', #56331 ) ;
#61755=CARTESIAN_POINT ( 'NONE',  ( 5.017113787211129328, 8.018716392533608683, 1.139262206072016559 ) ) ;
#61756=CARTESIAN_POINT ( 'NONE',  ( -4.543390873910949423, 6.393985001019784953, 1.443375672974058777 ) ) ;
#61757=CARTESIAN_POINT ( 'NONE',  ( 4.773879485787624333, 4.742149952939897162, -0.7216878364870357165 ) ) ;
#61767=EDGE_CURVE ( 'NONE', #758, #103686, #23810, .T. ) ;
#61771=VERTEX_POINT ( 'NONE', #55264 ) ;
#61786=CARTESIAN_POINT ( 'NONE',  ( 5.065906673361608270, 5.939254536123854677, -1.199719254218450271 ) ) ;
#61803=CARTESIAN_POINT ( 'NONE',  ( -5.596483547390937119, 9.751257581923240991, 0.000000000000000000 ) ) ;
#61805=ORIENTED_EDGE ( 'NONE', *, *, #69350, .F. ) ;
#61814=CARTESIAN_POINT ( 'NONE',  ( 5.879395890181562834, 6.888325289080478697, -1.199719254218452047 ) ) ;
#61820=CARTESIAN_POINT ( 'NONE',  ( 5.631432701629774051, 7.663367133358481631, 1.599625672291269396 ) ) ;
#61830=CARTESIAN_POINT ( 'NONE',  ( 4.631618433768171172, 8.327536854573105884, -0.3785340233409782984 ) ) ;
#61838=CARTESIAN_POINT ( 'NONE',  ( 4.970485548933691433, 6.521808019254549116, 1.328095809470300814 ) ) ;
#61843=EDGE_CURVE ( 'NONE', #47264, #211508, #14560, .T. ) ;
#61849=CARTESIAN_POINT ( 'NONE',  ( -5.631432701629818460, 7.663367133358481631, 1.599625672291263179 ) ) ;
#61851=CARTESIAN_POINT ( 'NONE',  ( 6.235824307642648279, 6.239826211863360506, 0.000000000000000000 ) ) ;
#61855=CARTESIAN_POINT ( 'NONE',  ( -7.533490631048818109, 8.818102486758951031, -1.199719254218452047 ) ) ;
#61858=CIRCLE ( 'NONE', #106903, 4.022469383779238683 ) ;
#61860=CARTESIAN_POINT ( 'NONE',  ( 2.743825832610055748, 3.021665646862250920, -2.500000000000000444 ) ) ;
#61863=ADVANCED_FACE ( 'NONE', ( #179680 ), #128762, .T. ) ;
#61865=CARTESIAN_POINT ( 'NONE',  ( -5.526470424545159688, 7.552361116859303891, -1.349762019914104272 ) ) ;
#61881=CARTESIAN_POINT ( 'NONE',  ( 4.556949027968946631, 8.330541276023501140, -0.7216878364870357165 ) ) ;
#61884=EDGE_CURVE ( 'NONE', #29314, #105686, #39112, .T. ) ;
#61888=EDGE_LOOP ( 'NONE', ( #209065, #212444, #163689, #165072 ) ) ;
#61893=DIRECTION ( 'NONE',  ( 0.7592566023653005702, -0.6507913734559639396, 0.000000000000000000 ) ) ;
#61899=CARTESIAN_POINT ( 'NONE',  ( -3.011319516011047082, 6.527306845405913549, 0.7216878364870328300 ) ) ;
#61903=CARTESIAN_POINT ( 'NONE',  ( 3.725458348705031231, 7.568394850123006279, -1.734723475976807094E-15 ) ) ;
#61906=FACE_OUTER_BOUND ( 'NONE', #57586, .T. ) ;
#61928=CARTESIAN_POINT ( 'NONE',  ( 5.747730777550676073, 5.670383760089384495, 0.000000000000000000 ) ) ;
#61954=CARTESIAN_POINT ( 'NONE',  ( -5.939880696118548187, 6.102484698325975288, 0.000000000000000000 ) ) ;
#61960=ORIENTED_EDGE ( 'NONE', *, *, #91370, .F. ) ;
#61961=CARTESIAN_POINT ( 'NONE',  ( -4.437261413422502798, 8.398831758960053406, 0.000000000000000000 ) ) ;
#61972=CARTESIAN_POINT ( 'NONE',  ( -5.492988512192097161, 6.437516681426083132, 1.199719254218452935 ) ) ;
#61974=ORIENTED_EDGE ( 'NONE', *, *, #88712, .F. ) ;
#61975=CARTESIAN_POINT ( 'NONE',  ( 5.307274686206796765, 7.744096871513173497, 1.304404211447189876 ) ) ;
#61980=CARTESIAN_POINT ( 'NONE',  ( 5.529746549527311039, 7.544733289238903851, -1.599625672291281386 ) ) ;
#61988=CARTESIAN_POINT ( 'NONE',  ( -4.085803189671902480, 5.860132702740892263, -1.599625672291271394 ) ) ;
#61993=CARTESIAN_POINT ( 'NONE',  ( -4.936050443827081580, 7.916420063510339666, 1.199719254218452935 ) ) ;
#61997=CARTESIAN_POINT ( 'NONE',  ( 6.834718834620487016, 7.146462526578263308, 0.000000000000000000 ) ) ;
#61999=CARTESIAN_POINT ( 'NONE',  ( -5.112833325684904118, 8.979072956692109031, -0.7216878364870338292 ) ) ;
#62006=CARTESIAN_POINT ( 'NONE',  ( 5.879395890181562834, 6.888325289080478697, -1.199719254218452047 ) ) ;
#62013=CARTESIAN_POINT ( 'NONE',  ( 4.318600669050584706, 4.999583595936801572, 2.419999999999999485 ) ) ;
#62033=CARTESIAN_POINT ( 'NONE',  ( 3.147653791585803162, 8.919999999999939533, -2.500000000000000444 ) ) ;
#62038=CARTESIAN_POINT ( 'NONE',  ( 5.054560120293923653, 7.862967615930308796, 1.113740650586869219 ) ) ;
#62046=CARTESIAN_POINT ( 'NONE',  ( 5.671053392266061977, 9.838255734277600695, 0.7998128361456331437 ) ) ;
#62051=CARTESIAN_POINT ( 'NONE',  ( -4.712247760717829692, 8.249883430950177399, 0.6303846594760522670 ) ) ;
#62054=ORIENTED_EDGE ( 'NONE', *, *, #56512, .T. ) ;
#62058=CARTESIAN_POINT ( 'NONE',  ( -3.146901051703345331, 6.685485303713597283, 0.000000000000000000 ) ) ;
#62068=CARTESIAN_POINT ( 'NONE',  ( -5.327428015527048366, 5.180030537728460338, -0.7998128361456362523 ) ) ;
#62070=CARTESIAN_POINT ( 'NONE',  ( 6.003228155800906407, 10.22579295840155744, 0.000000000000000000 ) ) ;
#62072=LINE ( 'NONE', #13308, #202886 ) ;
#62077=CARTESIAN_POINT ( 'NONE',  ( 5.499767588998890844, 6.445425604367387429, 1.199719254218451159 ) ) ;
#62080=CARTESIAN_POINT ( 'NONE',  ( 5.139949632912227173, 8.050339434155988627, -1.082531754730548412 ) ) ;
#62086=DIRECTION ( 'NONE',  ( -0.6507913734559641616, -0.7592566023653004592, 0.000000000000000000 ) ) ;
#62087=CARTESIAN_POINT ( 'NONE',  ( -6.344338864096334518, 6.859745832460597548, 0.6559349933493059392 ) ) ;
#62094=CARTESIAN_POINT ( 'NONE',  ( -4.472210567661380587, 6.310941310395290493, 1.599625672291270506 ) ) ;
#62095=CARTESIAN_POINT ( 'NONE',  ( 5.011674058906918638, 5.875983152593414971, 1.199719254218452047 ) ) ;
#62107=CARTESIAN_POINT ( 'NONE',  ( -7.273023059088104425, 7.449891421883056530, 0.000000000000000000 ) ) ;
#62108=CARTESIAN_POINT ( 'NONE',  ( 4.844006021832467646, 8.873367135438366304, 0.000000000000000000 ) ) ;
#62110=CARTESIAN_POINT ( 'NONE',  ( 6.495764994278797388, 8.671754808115688107, 1.443375672974063439 ) ) ;
#62121=CARTESIAN_POINT ( 'NONE',  ( -5.206707715320216145, 7.734635641480951840, -1.194516140545264227 ) ) ;
#62122=DIRECTION ( 'NONE',  ( -0.6507913734559640506, -0.7592566023653003482, 0.000000000000000000 ) ) ;
#62129=CARTESIAN_POINT ( 'NONE',  ( -2.984203208339354152, 6.495671153122273722, 0.000000000000000000 ) ) ;
#62147=CARTESIAN_POINT ( 'NONE',  ( 5.342795052237045539, 8.390955439988655229, -1.199719254218450271 ) ) ;
#62173=ORIENTED_EDGE ( 'NONE', *, *, #79643, .T. ) ;
#62183=CARTESIAN_POINT ( 'NONE',  ( 7.404161286838808920, 8.771181268467660885, -1.082531754730548412 ) ) ;
#62210=EDGE_LOOP ( 'NONE', ( #179478, #52217, #163043, #16766 ) ) ;
#62211=CARTESIAN_POINT ( 'NONE',  ( -5.926849427829407269, 6.943687749669614995, -1.199719254218453823 ) ) ;
#62213=CARTESIAN_POINT ( 'NONE',  ( 6.983858524370782028, 8.280828045588322084, 1.082531754730549967 ) ) ;
#62218=CARTESIAN_POINT ( 'NONE',  ( -5.601453741101424022, 6.564059448486966986, -1.199719254218453823 ) ) ;
#62222=DIRECTION ( 'NONE',  ( -0.000000000000000000, -1.000000000000000000, -0.000000000000000000 ) ) ;
#62223=CARTESIAN_POINT ( 'NONE',  ( -3.135678666510573365, 6.880318554229450712, 0.000000000000000000 ) ) ;
#62229=CARTESIAN_POINT ( 'NONE',  ( -6.283277845290492714, 6.295188672452495915, -0.7998128361456362523 ) ) ;
#62238=CARTESIAN_POINT ( 'NONE',  ( -3.610214042988883598, 7.433943160120816351, 0.7998128361456352531 ) ) ;
#62241=CARTESIAN_POINT ( 'NONE',  ( -6.617788377246204945, 6.893376992974917350, -0.7216878364870338292 ) ) ;
#62242=CARTESIAN_POINT ( 'NONE',  ( -5.248414861821563804, 9.137251415518218067, 0.7216878364870267237 ) ) ;
#62243=CARTESIAN_POINT ( 'NONE',  ( 7.361151057576892143, 7.552707420120024828, 0.7998128361456291469 ) ) ;
#62244=CARTESIAN_POINT ( 'NONE',  ( -6.095272577795516789, 9.268845886473535245, 1.199719254218452047 ) ) ;
#62282=CARTESIAN_POINT ( 'NONE',  ( 4.827426732796687325, 8.217478009653898852, -0.9130428269800896501 ) ) ;
#62292=B_SPLINE_CURVE_WITH_KNOTS ( 'NONE', 3,
 ( #133701, #115348, #82772, #66490, #182392, #97990, #134756, #147795, #67557, #148846, #100095, #198636, #116403 ),
 .UNSPECIFIED., .F., .F.,
 ( 4, 3, 3, 3, 4 ),
 ( 2.035183503902616585E-17, 6.251625766521519618E-05, 0.0001877438076102492463, 0.0003155212742595949371, 0.0004444121044040558622 ),
 .UNSPECIFIED. ) ;
#62296=CARTESIAN_POINT ( 'NONE',  ( 5.631432701629774051, 7.663367133358481631, 1.599625672291269396 ) ) ;
#62299=CARTESIAN_POINT ( 'NONE',  ( -3.983063267364693960, 7.868933921892603323, -0.7998128361456481317 ) ) ;
#62303=CARTESIAN_POINT ( 'NONE',  ( -6.658462837642833421, 8.861568958707010779, 1.443375672974064550 ) ) ;
#62314=CARTESIAN_POINT ( 'NONE',  ( 5.657495238652423097, 9.822437888394988548, 0.000000000000000000 ) ) ;
#62315=CARTESIAN_POINT ( 'NONE',  ( 6.017840079619279692, 8.114175741012878973, -1.599625672291281386 ) ) ;
#62319=CARTESIAN_POINT ( 'NONE',  ( -4.793291032674840579, 4.846031192413886579, -0.3973851993939380156 ) ) ;
#62323=CARTESIAN_POINT ( 'NONE',  ( 4.085803189671889157, 5.860132702740892263, -1.599625672291273171 ) ) ;
#62325=B_SPLINE_CURVE_WITH_KNOTS ( 'NONE', 3,
 ( #86140, #197749, #33129, #181501, #149007, #183633, #152211, #201981, #16851, #151154 ),
 .UNSPECIFIED., .F., .F.,
 ( 4, 2, 2, 2, 4 ),
 ( 0.000000000000000000, 0.1250610353511166506, 0.2501220707022333012, 0.3751831060533499240, 0.5002441414044666024 ),
 .UNSPECIFIED. ) ;
#62330=CARTESIAN_POINT ( 'NONE',  ( 5.189738938980948291, 9.276722205444929870, 0.000000000000000000 ) ) ;
#62331=ORIENTED_EDGE ( 'NONE', *, *, #82621, .T. ) ;
#62336=CARTESIAN_POINT ( 'NONE',  ( 3.719872605471109761, 6.605953636083950364, -2.420000000000002149 ) ) ;
#62342=CARTESIAN_POINT ( 'NONE',  ( -5.370438244788932280, 6.398504386076097283, 1.082531754730549078 ) ) ;
#62343=CARTESIAN_POINT ( 'NONE',  ( -5.901542003698421190, 10.10715911428198055, 0.000000000000000000 ) ) ;
#62353=CARTESIAN_POINT ( 'NONE',  ( -4.065465959251405081, 5.836405933916976707, -1.599625672291271394 ) ) ;
#62354=CARTESIAN_POINT ( 'NONE',  ( 5.363132282657546490, 8.414682208812571673, -1.199719254218452047 ) ) ;
#62357=CARTESIAN_POINT ( 'NONE',  ( 5.207740400980577888, 5.248321020665011716, 0.000000000000000000 ) ) ;
#62370=CARTESIAN_POINT ( 'NONE',  ( -0.4000000000000243916, 3.000000000000566214, -2.023857702507757317 ) ) ;
#62372=CARTESIAN_POINT ( 'NONE',  ( 4.525389411911321602, 8.501647757197021704, -0.7998128361456381397 ) ) ;
#62374=CARTESIAN_POINT ( 'NONE',  ( -3.709037541790315640, 6.484905011134099340, -1.199719254218450271 ) ) ;
#62385=CARTESIAN_POINT ( 'NONE',  ( 6.021229618244865023, 10.03886863134542828, -0.7216878364870458196 ) ) ;
#62387=CARTESIAN_POINT ( 'NONE',  ( -6.770317605177755382, 8.992066187497757213, 1.599625672291269396 ) ) ;
#62388=CARTESIAN_POINT ( 'NONE',  ( 4.908934136599710563, 7.884784371745123366, 1.199719254218451159 ) ) ;
#62400=CARTESIAN_POINT ( 'NONE',  ( -4.634908411025374875, 6.500755460986618495, 1.599625672291263179 ) ) ;
#62428=CARTESIAN_POINT ( 'NONE',  ( 4.041739190649647817, 6.769093918182960579, -1.082531754730548412 ) ) ;
#62434=CARTESIAN_POINT ( 'NONE',  ( 4.055297343818923039, 7.745280977848496562, 0.7216878364870257245 ) ) ;
#62446=CARTESIAN_POINT ( 'NONE',  ( -4.959250327548641479, 9.007818825440551791, -0.7998128361456362523 ) ) ;
#62448=CARTESIAN_POINT ( 'NONE',  ( -7.937372586157736443, 8.224965870130965584, 0.7998128361456341429 ) ) ;
#62454=CARTESIAN_POINT ( 'NONE',  ( 3.542963271983512463, 7.334866628692126689, -0.05839583369298829985 ) ) ;
#62455=CARTESIAN_POINT ( 'NONE',  ( 6.502017186205484300, 9.743381262951846367, -1.199719254218452047 ) ) ;
#62462=CARTESIAN_POINT ( 'NONE',  ( -5.855142236255304944, 7.924361590421551860, -1.599625672291271394 ) ) ;
#62468=CARTESIAN_POINT ( 'NONE',  ( -3.499413046103020175, 7.096749297179887783, 0.7216878364870338292 ) ) ;
#62472=CARTESIAN_POINT ( 'NONE',  ( -4.827585214917754719, 7.789877296449459365, -1.199719254218453823 ) ) ;
#62486=DIRECTION ( 'NONE',  ( 0.7592566023653004592, 0.6507913734559639396, 0.000000000000000000 ) ) ;
#62491=CARTESIAN_POINT ( 'NONE',  ( -7.767895665986912057, 8.027242796598338614, -0.7998128361456362523 ) ) ;
#62492=CARTESIAN_POINT ( 'NONE',  ( -5.666381855868691808, 5.575476684793721383, 0.000000000000000000 ) ) ;
#62518=CARTESIAN_POINT ( 'NONE',  ( -6.740338644649361832, 7.892758502626242567, -1.199719254218452047 ) ) ;
#62542=CARTESIAN_POINT ( 'NONE',  ( 7.364013710877980401, 8.620379413226322285, -1.199719254218452047 ) ) ;
#62543=CARTESIAN_POINT ( 'NONE',  ( 6.481679955784983349, 9.719654494127929922, -1.199719254218452047 ) ) ;
#62555=CARTESIAN_POINT ( 'NONE',  ( 5.510920874727778696, 7.454463421478725316, 1.249874847645112697 ) ) ;
#62557=CARTESIAN_POINT ( 'NONE',  ( 7.363486825997814123, 7.763358516518489516, 0.000000000000000000 ) ) ;
#62563=CARTESIAN_POINT ( 'NONE',  ( -5.255720823952942489, 6.160704378480398979, -1.199719254218453823 ) ) ;
#62569=CARTESIAN_POINT ( 'NONE',  ( -5.763624699140882157, 7.817591130454727200, -1.443375672974066548 ) ) ;
#62571=CARTESIAN_POINT ( 'NONE',  ( -4.108375792757257727, 7.564741050373271491, 0.6295801075443598904 ) ) ;
#62577=CARTESIAN_POINT ( 'NONE',  ( -4.146814880933400005, 5.931313009212638931, 1.599625672291270506 ) ) ;
#62587=CARTESIAN_POINT ( 'NONE',  ( 6.318982112420993502, 9.529840343536603697, -1.199719254218452047 ) ) ;
#62605=CARTESIAN_POINT ( 'NONE',  ( -7.208094944320834863, 8.438474185576302133, -1.199719254218452047 ) ) ;
#62608=CARTESIAN_POINT ( 'NONE',  ( 7.503511670520385479, 7.718794801887437274, 0.7998128361456281477 ) ) ;
#62611=CARTESIAN_POINT ( 'NONE',  ( -5.679286501732877745, 7.334821546209805199, 1.225395024417414103 ) ) ;
#62617=CARTESIAN_POINT ( 'NONE',  ( 4.960304097753311936, 6.880383762169266504, 1.599625672291268286 ) ) ;
#62626=CARTESIAN_POINT ( 'NONE',  ( 5.641601317062233001, 7.675230518029648508, -1.443375672974078761 ) ) ;
#62638=CARTESIAN_POINT ( 'NONE',  ( -6.780486220610195680, 7.083191143566240910, -0.7216878364870338292 ) ) ;
#62661=CARTESIAN_POINT ( 'NONE',  ( 6.034787771414189095, 6.213209619504255876, -0.7216878364870512597 ) ) ;
#62671=CARTESIAN_POINT ( 'NONE',  ( 4.532168488718122390, 8.509556680138327778, 0.7998128361456271485 ) ) ;
#62673=CARTESIAN_POINT ( 'NONE',  ( 7.035755370848908896, 7.173079118937375931, 0.7998128361456352531 ) ) ;
#62684=CARTESIAN_POINT ( 'NONE',  ( -4.995253251992230581, 4.792493313604505367, 0.000000000000000000 ) ) ;
#62687=CARTESIAN_POINT ( 'NONE',  ( 5.989670002187236442, 10.20997511251894529, -0.7998128361456481317 ) ) ;
#62702=CARTESIAN_POINT ( 'NONE',  ( -6.780486220610195680, 7.083191143566240910, -0.7216878364870338292 ) ) ;
#62704=CARTESIAN_POINT ( 'NONE',  ( -5.831415467653581430, 5.975941931783510519, 0.7216878364870257245 ) ) ;
#62708=DIRECTION ( 'NONE',  ( 0.000000000000000000, 1.000000000000000000, 0.000000000000000000 ) ) ;
#62718=CIRCLE ( 'NONE', #142250, 2.000000000000000000 ) ;
#62742=CARTESIAN_POINT ( 'NONE',  ( -6.936931872047518155, 8.122117267924091166, 1.199719254218452047 ) ) ;
#62743=CARTESIAN_POINT ( 'NONE',  ( -5.689102680971802606, 7.419971068449684459, 1.333831099742349480 ) ) ;
#62751=CARTESIAN_POINT ( 'NONE',  ( -3.305155586681401303, 7.078041627762083898, 0.7998128361456352531 ) ) ;
#62754=CARTESIAN_POINT ( 'NONE',  ( -4.492547798081878874, 6.334668079219206049, 1.599625672291263179 ) ) ;
#62766=CARTESIAN_POINT ( 'NONE',  ( 5.306037014901791693, 7.283738832175834510, 1.599625672291269396 ) ) ;
#62771=ADVANCED_FACE ( 'NONE', ( #115030, #14237 ), #31596, .F. ) ;
#62791=CARTESIAN_POINT ( 'NONE',  ( 6.066347387471824781, 6.042103138330730872, -0.7998128361456481317 ) ) ;
#62792=CARTESIAN_POINT ( 'NONE',  ( 4.115782150200256950, 6.959440387612411349, 1.199719254218452047 ) ) ;
#62794=CARTESIAN_POINT ( 'NONE',  ( 3.932747076415766596, 6.745899468197171345, 1.199719254218451159 ) ) ;
#62808=CARTESIAN_POINT ( 'NONE',  ( 4.672271667806711548, 8.395315985019093930, 0.5582388282892002396 ) ) ;
#62809=CARTESIAN_POINT ( 'NONE',  ( -4.462041952228942954, 8.219816354326809460, -0.7216878364870338292 ) ) ;
#62838=CARTESIAN_POINT ( 'NONE',  ( 6.540882763950133238, 6.595727744222092959, 0.000000000000000000 ) ) ;
#62841=CARTESIAN_POINT ( 'NONE',  ( 3.400062661977048428, 7.188766548940353829, -1.734723475976807094E-15 ) ) ;
#62843=EDGE_CURVE ( 'NONE', #162782, #192662, #22799, .T. ) ;
#62856=CARTESIAN_POINT ( 'NONE',  ( -6.851666526859749418, 9.086973262793417661, -1.599625672291271394 ) ) ;
#62858=EDGE_LOOP ( 'NONE', ( #139635, #210844, #88485, #170784, #112955, #173895, #43996 ) ) ;
#62867=CARTESIAN_POINT ( 'NONE',  ( 4.854701522145073334, 7.821512988214679218, -1.199719254218450271 ) ) ;
#62873=CARTESIAN_POINT ( 'NONE',  ( 6.574778147984297938, 6.635272358928617997, -0.7998128361456481317 ) ) ;
#62878=EDGE_LOOP ( 'NONE', ( #172630, #24222, #185088, #198284, #84076 ) ) ;
#62884=CARTESIAN_POINT ( 'NONE',  ( 4.666668778386947380, 8.284408874816399759, 0.5204741841226891985 ) ) ;
#62898=CARTESIAN_POINT ( 'NONE',  ( -6.249896535389937391, 6.922618705386589077, 0.8105719012266124901 ) ) ;
#62901=ORIENTED_EDGE ( 'NONE', *, *, #50156, .T. ) ;
#62905=CARTESIAN_POINT ( 'NONE',  ( -5.794130544993808307, 7.853181283949808744, 1.599625672291263179 ) ) ;
#62907=CARTESIAN_POINT ( 'NONE',  ( 5.091969210384201361, 8.098325291160362482, 1.199719254218452047 ) ) ;
#62912=CARTESIAN_POINT ( 'NONE',  ( -6.343235766347277149, 8.493804042195527870, -1.599625672291271394 ) ) ;
#62921=CARTESIAN_POINT ( 'NONE',  ( -6.489832820117282353, 6.840411167308092288, -0.6218019135817691723 ) ) ;
#62930=EDGE_CURVE ( 'NONE', #95923, #61752, #173862, .T. ) ;
#62939=CARTESIAN_POINT ( 'NONE',  ( 5.045042558060919724, 8.899983727797476263, -0.7216878364870458196 ) ) ;
#62946=DIRECTION ( 'NONE',  ( -0.6507913734559641616, -0.7592566023653004592, 0.000000000000000000 ) ) ;
#62952=CARTESIAN_POINT ( 'NONE',  ( -4.285785955695645910, 7.053815144069948140, 1.082531754730549967 ) ) ;
#62956=CARTESIAN_POINT ( 'NONE',  ( 5.224688093219824303, 7.188831756880171397, -1.599625672291283607 ) ) ;
#62962=CARTESIAN_POINT ( 'NONE',  ( -1.833030277982346634, 9.001999999999998892, -2.499999999999998668 ) ) ;
#62975=CARTESIAN_POINT ( 'NONE',  ( 6.983858524370782028, 8.280828045588322084, 1.082531754730549967 ) ) ;
#63000=CARTESIAN_POINT ( 'NONE',  ( 4.014622883422321209, 5.777089012116397804, -1.443375672974068769 ) ) ;
#63005=APPLICATION_CONTEXT ( 'automotive_design' ) ;
#63010=CARTESIAN_POINT ( 'NONE',  ( -5.438229012412903352, 6.477593614970734492, -1.082531754730549967 ) ) ;
#63015=EDGE_CURVE ( 'NONE', #158170, #206605, #134452, .T. ) ;
#63017=CARTESIAN_POINT ( 'NONE',  ( -6.635789839245807897, 6.706452665400368218, 0.7998128361456341429 ) ) ;
#63019=CIRCLE ( 'NONE', #18001, 2.080000000000000071 ) ;
#63029=CARTESIAN_POINT ( 'NONE',  ( -3.983063267364693960, 7.868933921892603323, -0.7998128361456481317 ) ) ;
#63032=CARTESIAN_POINT ( 'NONE',  ( 6.218145995260431214, 7.027935176161393294, 1.016989286988238206 ) ) ;
#63035=CARTESIAN_POINT ( 'NONE',  ( 2.984786552656538472, 6.457129931797648048, 0.3969071495571047103 ) ) ;
#63037=CARTESIAN_POINT ( 'NONE',  ( 6.367489420273535039, 7.457767740854454708, -1.199719254218452047 ) ) ;
#63043=DIRECTION ( 'NONE',  ( -0.000000000000000000, -0.000000000000000000, 1.000000000000000000 ) ) ;
#63044=CARTESIAN_POINT ( 'NONE',  ( -3.169574050544739841, 6.919863168935977527, -0.7998128361456481317 ) ) ;
#63051=CARTESIAN_POINT ( 'NONE',  ( -5.971440312176176768, 5.931378217152456500, 0.000000000000000000 ) ) ;
#63054=CARTESIAN_POINT ( 'NONE',  ( 7.309254211098767051, 7.700087132469628948, 0.7216878364870267237 ) ) ;
#63056=CARTESIAN_POINT ( 'NONE',  ( -5.248414861821563804, 9.137251415518218067, 0.7216878364870267237 ) ) ;
#63063=CARTESIAN_POINT ( 'NONE',  ( 4.342354338126830804, 8.288106837781779035, -0.7998128361456381397 ) ) ;
#63064=VERTEX_POINT ( 'NONE', #100838 ) ;
#63093=CARTESIAN_POINT ( 'NONE',  ( 5.220047253295719614, 7.706380104734268599, 1.202949228536150938 ) ) ;
#63101=CARTESIAN_POINT ( 'NONE',  ( 6.318982112420993502, 9.529840343536603697, -1.199719254218452047 ) ) ;
#63102=ORIENTED_EDGE ( 'NONE', *, *, #88807, .T. ) ;
#63106=CARTESIAN_POINT ( 'NONE',  ( -5.206707715320216145, 7.734635641480951840, -1.194516140545264227 ) ) ;
#63115=CARTESIAN_POINT ( 'NONE',  ( -3.323157048681004699, 6.891117300187535655, -0.7216878364870458196 ) ) ;
#63126=CARTESIAN_POINT ( 'NONE',  ( -4.679499295372141709, 5.488445928469455559, 1.199719254218452935 ) ) ;
#63139=CARTESIAN_POINT ( 'NONE',  ( 4.258142763143749399, 7.125527769379820242, 1.199719254218451159 ) ) ;
#63142=CARTESIAN_POINT ( 'NONE',  ( 6.346625304528514810, 6.577020074804287297, 0.000000000000000000 ) ) ;
#63155=CARTESIAN_POINT ( 'NONE',  ( -4.716257332707368910, 6.595662536282280719, -1.599625672291271394 ) ) ;
#63156=CARTESIAN_POINT ( 'NONE',  ( 5.551137550152489553, 5.441024994791534120, 0.7998128361456352531 ) ) ;
#63166=CARTESIAN_POINT ( 'NONE',  ( -6.099189001301292379, 8.209082816308541197, 1.599625672291263179 ) ) ;
#63167=CARTESIAN_POINT ( 'NONE',  ( 7.354371980770088690, 7.544798497178720531, 0.000000000000000000 ) ) ;
#63169=CARTESIAN_POINT ( 'NONE',  ( -3.177206141917424009, 8.963489737286273851, -2.500000000000001332 ) ) ;
#63173=CARTESIAN_POINT ( 'NONE',  ( 4.686278372178935392, 5.496354851410763409, 1.199719254218452047 ) ) ;
#63181=CARTESIAN_POINT ( 'NONE',  ( -6.486551268120854807, 6.767445667853342783, -0.2095380678983837508 ) ) ;
#63188=CARTESIAN_POINT ( 'NONE',  ( -3.133342898089680695, 6.669667457830990465, 0.7216878364870338292 ) ) ;
#63189=CIRCLE ( 'NONE', #18167, 0.4800000000000000933 ) ;
#63204=CARTESIAN_POINT ( 'NONE',  ( 7.354371980770088690, 7.544798497178720531, 0.000000000000000000 ) ) ;
#63239=CARTESIAN_POINT ( 'NONE',  ( 3.878514461961128479, 6.682628084666728085, -1.199719254218448494 ) ) ;
#63270=CARTESIAN_POINT ( 'NONE',  ( -6.143779885648060102, 7.196773283791382703, 1.199719254218452047 ) ) ;
#63272=CARTESIAN_POINT ( 'NONE',  ( 7.173672674962134899, 7.541908673643526129, -0.7216878364870317197 ) ) ;
#63277=CARTESIAN_POINT ( 'NONE',  ( -4.359828915246279024, 7.244161613499399799, -1.199719254218455378 ) ) ;
#63283=CARTESIAN_POINT ( 'NONE',  ( -4.472210567661380587, 6.310941310395290493, 1.599625672291270506 ) ) ;
#63290=CARTESIAN_POINT ( 'NONE',  ( -4.125423880308188629, 8.035021303660014880, -0.7998128361456481317 ) ) ;
#63300=CARTESIAN_POINT ( 'NONE',  ( -4.339491684825780737, 7.220434844675483355, -1.199719254218455378 ) ) ;
#63303=CARTESIAN_POINT ( 'NONE',  ( -5.126391479742927970, 8.994890803093138487, 0.7216878364870267237 ) ) ;
#63304=CARTESIAN_POINT ( 'NONE',  ( -5.872089928050201024, 8.904503111816948646, 1.082531754730550855 ) ) ;
#63305=CARTESIAN_POINT ( 'NONE',  ( 6.230854113932139171, 9.427024345299638952, 1.199719254218452047 ) ) ;
#63306=CARTESIAN_POINT ( 'NONE',  ( -6.363572996767778100, 8.517530811019446091, -1.599625672291271394 ) ) ;
#63346=CARTESIAN_POINT ( 'NONE',  ( 4.614865537624940117, 8.465324746759504748, 0.2878883051726736086 ) ) ;
#63363=CARTESIAN_POINT ( 'NONE',  ( 4.850785098639300408, 8.881276058379668825, -0.7998128361456481317 ) ) ;
#63366=CARTESIAN_POINT ( 'NONE',  ( -5.666381855868691808, 5.575476684793721383, 0.000000000000000000 ) ) ;
#63370=CARTESIAN_POINT ( 'NONE',  ( -6.414416072596837104, 9.537216947121368804, -1.082531754730549967 ) ) ;
#63381=CARTESIAN_POINT ( 'NONE',  ( 4.549643065837591038, 7.465611455855944101, -1.199719254218452047 ) ) ;
#63383=CARTESIAN_POINT ( 'NONE',  ( 7.452141709366786770, 8.723195411463290583, 1.199719254218452047 ) ) ;
#63390=ORIENTED_EDGE ( 'NONE', *, *, #171151, .T. ) ;
#63397=CARTESIAN_POINT ( 'NONE',  ( 5.363132282657546490, 8.414682208812571673, -1.199719254218452047 ) ) ;
#63406=CARTESIAN_POINT ( 'NONE',  ( 4.908293137491657632, 4.795002863307560759, 0.000000000000000000 ) ) ;
#63410=CARTESIAN_POINT ( 'NONE',  ( -3.824808732831001201, 7.476377598362539345, 0.7216878364870338292 ) ) ;
#63411=CARTESIAN_POINT ( 'NONE',  ( 6.048345925472191631, 7.189396680206621149, 1.082531754730549967 ) ) ;
#63423=CARTESIAN_POINT ( 'NONE',  ( -7.458393901293492334, 7.874083437696761223, 0.7216878364870317197 ) ) ;
#63427=CARTESIAN_POINT ( 'NONE',  ( 7.095713291905693332, 9.371694488680407886, 1.599625672291268286 ) ) ;
#63442=CARTESIAN_POINT ( 'NONE',  ( -5.993453320721772393, 6.500486263839809098, 0.7145505879262403770 ) ) ;
#63444=CARTESIAN_POINT ( 'NONE',  ( 5.306037014901791693, 7.283738832175834510, 1.599625672291269396 ) ) ;
#63446=CARTESIAN_POINT ( 'NONE',  ( -6.005335696210345020, 5.970922831858983315, 0.7998128361456281477 ) ) ;
#63458=CARTESIAN_POINT ( 'NONE',  ( 7.187230829020130329, 7.557726520044554697, 0.7216878364870267237 ) ) ;
#63460=CARTESIAN_POINT ( 'NONE',  ( -6.149505192250180663, 9.332117270003974951, -1.199719254218452047 ) ) ;
#63461=CARTESIAN_POINT ( 'NONE',  ( 6.527324610336440180, 6.579909898339485252, 0.7998128361456331437 ) ) ;
#63470=CARTESIAN_POINT ( 'NONE',  ( -4.797606254389363833, 6.690569611577942943, 1.599625672291263179 ) ) ;
#63500=CIRCLE ( 'NONE', #15077, 0.08000000000000041800 ) ;
#63501=CARTESIAN_POINT ( 'NONE',  ( 4.800995793014950941, 5.734154859006458160, -1.082531754730548412 ) ) ;
#63507=CARTESIAN_POINT ( 'NONE',  ( 4.217995187182920880, 6.974725914138481642, 1.082531754730549078 ) ) ;
#63518=AXIS2_PLACEMENT_3D ( 'NONE', #204869, #85815, #69538 ) ;
#63522=CARTESIAN_POINT ( 'NONE',  ( -5.794130544993808307, 7.853181283949808744, 1.599625672291263179 ) ) ;
#63524=CARTESIAN_POINT ( 'NONE',  ( -6.454563648557663846, 9.688018802362710957, -1.199719254218452047 ) ) ;
#63529=CARTESIAN_POINT ( 'NONE',  ( 3.079110283634975964, 6.606396074300548982, 0.7216878364870257245 ) ) ;
#63534=CARTESIAN_POINT ( 'NONE',  ( -5.315678745009726924, 8.359319748223434487, -1.199719254218453823 ) ) ;
#63540=CARTESIAN_POINT ( 'NONE',  ( -4.990809943606286048, 5.955604701363006015, -1.082531754730549967 ) ) ;
#63543=CARTESIAN_POINT ( 'NONE',  ( -4.610654757099099221, 7.536791762327691657, 1.199719254218452935 ) ) ;
#63561=ORIENTED_EDGE ( 'NONE', *, *, #50156, .F. ) ;
#63562=CARTESIAN_POINT ( 'NONE',  ( -7.608060475923978494, 8.905100639113307182, 1.199719254218452047 ) ) ;
#63563=CARTESIAN_POINT ( 'NONE',  ( 3.088225128862704949, 6.824956093640315302, 0.7998128361456281477 ) ) ;
#63564=CARTESIAN_POINT ( 'NONE',  ( -5.991777542596674166, 5.955104985976372944, 0.000000000000000000 ) ) ;
#63569=EDGE_CURVE ( 'NONE', #173630, #109313, #118410, .T. ) ;
#63584=CARTESIAN_POINT ( 'NONE',  ( 4.858757509019057785, 5.629766575900002401, -2.420000000000000373 ) ) ;
#63590=CARTESIAN_POINT ( 'NONE',  ( -6.526270840131767059, 8.707344961610770540, -1.599625672291271394 ) ) ;
#63617=CARTESIAN_POINT ( 'NONE',  ( 7.340813827156391191, 7.528980651296110160, 0.7998128361456281477 ) ) ;
#63618=LINE ( 'NONE', #65711, #76019 ) ;
#63632=CARTESIAN_POINT ( 'NONE',  ( 5.732961426666957294, 7.278201736375829789, 1.206439608388230500 ) ) ;
#63634=CARTESIAN_POINT ( 'NONE',  ( 5.072158865288222351, 8.931619419562697004, 0.7216878364870317197 ) ) ;
#63639=CARTESIAN_POINT ( 'NONE',  ( -3.610214042988883598, 7.433943160120816351, 0.7998128361456352531 ) ) ;
#63655=CARTESIAN_POINT ( 'NONE',  ( -5.984998465789844069, 5.947196063035064206, 0.7998128361456281477 ) ) ;
#63665=CARTESIAN_POINT ( 'NONE',  ( 3.223806664999388172, 6.983134552466421674, -0.7998128361456362523 ) ) ;
#63685=CARTESIAN_POINT ( 'NONE',  ( 4.993145711582793744, 9.047363440147082159, -0.7998128361456481317 ) ) ;
#63687=CARTESIAN_POINT ( 'NONE',  ( -5.472807559815892731, 7.501441282320147508, 1.250076539767187578 ) ) ;
#63695=CARTESIAN_POINT ( 'NONE',  ( 5.337069745634900997, 6.255611453776062980, 1.199719254218452047 ) ) ;
#63701=FACE_OUTER_BOUND ( 'NONE', #207342, .T. ) ;
#63703=CARTESIAN_POINT ( 'NONE',  ( 6.211043768836173484, 8.339580045099285854, 1.443375672974065660 ) ) ;
#63714=CARTESIAN_POINT ( 'NONE',  ( -4.638297949650955765, 8.425448351319163365, 0.7216878364870267237 ) ) ;
#63742=ORIENTED_EDGE ( 'NONE', *, *, #149120, .F. ) ;
#63746=CARTESIAN_POINT ( 'NONE',  ( 5.448397627845284141, 7.449826213943242514, 1.599625672291268286 ) ) ;
#63748=CARTESIAN_POINT ( 'NONE',  ( 4.929271367020211514, 7.908511140569038922, 1.199719254218452047 ) ) ;
#63760=CARTESIAN_POINT ( 'NONE',  ( -4.981695098378565945, 4.776675467721892332, -0.7998128361456362523 ) ) ;
#63763=CARTESIAN_POINT ( 'NONE',  ( 3.879041346841291649, 7.539648981374564407, 1.040834085586084257E-14 ) ) ;
#63777=CARTESIAN_POINT ( 'NONE',  ( -5.153507786970262572, 9.026526494858359229, -0.7216878364870338292 ) ) ;
#63779=CARTESIAN_POINT ( 'NONE',  ( -3.526529353330350336, 7.128384988945109413, -0.7216878364870458196 ) ) ;
#63780=CARTESIAN_POINT ( 'NONE',  ( 4.393008644795362905, 7.016788222801661590, 1.284222742053114041 ) ) ;
#63797=VERTEX_POINT ( 'NONE', #40720 ) ;
#63807=CARTESIAN_POINT ( 'NONE',  ( -4.329849954717889915, 6.144853928627882489, 1.599625672291270506 ) ) ;
#63814=CARTESIAN_POINT ( 'NONE',  ( -5.606595252507366567, 5.572856915785063592, -0.3451608010808376870 ) ) ;
#63819=CARTESIAN_POINT ( 'NONE',  ( -5.966470118465691641, 9.118576350588734059, -1.199719254218452047 ) ) ;
#63820=CARTESIAN_POINT ( 'NONE',  ( -5.137161949866410282, 7.898551110135567654, 1.241398918778359173 ) ) ;
#63829=CARTESIAN_POINT ( 'NONE',  ( -5.655686355556086120, 6.627330832017406692, 1.199719254218452935 ) ) ;
#63835=CARTESIAN_POINT ( 'NONE',  ( -6.328041841479842056, 6.870487382198048998, 0.6860574420480938240 ) ) ;
#63841=CARTESIAN_POINT ( 'NONE',  ( 4.362691568547328202, 8.311833606605697256, -0.7998128361456381397 ) ) ;
#63866=CARTESIAN_POINT ( 'NONE',  ( 4.420840606507738357, 7.315341919971147355, 1.199719254218451159 ) ) ;
#63867=CARTESIAN_POINT ( 'NONE',  ( 5.086243903782109221, 5.962981304947771122, -1.199719254218452047 ) ) ;
#63869=CARTESIAN_POINT ( 'NONE',  ( 5.063044020060520900, 4.871582543017558109, 0.7998128361456352531 ) ) ;
#63881=CARTESIAN_POINT ( 'NONE',  ( 5.469253881944042384, 7.602781119232224327, 1.336104631850141944 ) ) ;
#63882=CARTESIAN_POINT ( 'NONE',  ( -4.950135482320918712, 7.828889591799445213, -1.082531754730549967 ) ) ;
#63895=ORIENTED_EDGE ( 'NONE', *, *, #72507, .F. ) ;
#63908=CARTESIAN_POINT ( 'NONE',  ( 5.499767588998890844, 6.445425604367387429, 1.199719254218451159 ) ) ;
#63927=CARTESIAN_POINT ( 'NONE',  ( -7.781453819600577582, 8.043060642480948985, 0.000000000000000000 ) ) ;
#63939=ORIENTED_EDGE ( 'NONE', *, *, #137980, .T. ) ;
#63940=CARTESIAN_POINT ( 'NONE',  ( 5.529746549527311039, 7.544733289238903851, -1.599625672291281386 ) ) ;
#63944=CARTESIAN_POINT ( 'NONE',  ( 4.715203562502613188, 8.723097599553565118, 0.7998128361456341429 ) ) ;
#63953=VECTOR ( 'NONE', #149804, 1000.000000000000114 ) ;
#63956=CARTESIAN_POINT ( 'NONE',  ( 4.644395130292630292, 8.311692339142366492, -0.4369040224408097250 ) ) ;
#63967=CARTESIAN_POINT ( 'NONE',  ( -6.305925513666572613, 6.529536985466737775, -1.006778644550405474E-06 ) ) ;
#63972=CARTESIAN_POINT ( 'NONE',  ( -6.097415271940877624, 7.027018469112610077, 0.9862998271150682505 ) ) ;
#63982=CARTESIAN_POINT ( 'NONE',  ( -6.954406449166956605, 7.078172043641714595, -0.7998128361456362523 ) ) ;
#63984=CARTESIAN_POINT ( 'NONE',  ( 6.574778147984297938, 6.635272358928617997, -0.7998128361456481317 ) ) ;
#63988=CARTESIAN_POINT ( 'NONE',  ( -7.587723245503481095, 8.881373870289390737, 1.199719254218452047 ) ) ;
#63995=CARTESIAN_POINT ( 'NONE',  ( -6.218052724642120666, 7.025831364812846758, -1.032658732443512584 ) ) ;
#64013=CARTESIAN_POINT ( 'NONE',  ( 6.712695452541852070, 7.004101914153185504, 0.000000000000000000 ) ) ;
#64030=CARTESIAN_POINT ( 'NONE',  ( -4.014622883422322985, 7.697827440719083647, -0.7216878364870458196 ) ) ;
#64032=CARTESIAN_POINT ( 'NONE',  ( 5.040599249230596435, 9.102725900736217568, 0.7998128361456341429 ) ) ;
#64036=DIRECTION ( 'NONE',  ( 0.6507913734559641616, -0.7592566023653004592, 0.000000000000000000 ) ) ;
#64077=CARTESIAN_POINT ( 'NONE',  ( 3.553645660557675612, 6.199651466408984568, -1.082531754730549967 ) ) ;
#64084=CARTESIAN_POINT ( 'NONE',  ( -4.163763581353360443, 7.871824920094959488, -5.011504818508299590E-05 ) ) ;
#64086=ORIENTED_EDGE ( 'NONE', *, *, #172230, .F. ) ;
#64087=CARTESIAN_POINT ( 'NONE',  ( -3.811250578772977349, 7.460559751961507224, -0.7216878364870458196 ) ) ;
#64095=CARTESIAN_POINT ( 'NONE',  ( -4.827585214917754719, 7.789877296449459365, -1.199719254218453823 ) ) ;
#64104=CARTESIAN_POINT ( 'NONE',  ( -3.820365424000704557, 7.679119771301277098, -0.7998128361456481317 ) ) ;
#64107=CARTESIAN_POINT ( 'NONE',  ( 5.502223863662048409, 7.574938096329499437, 1.338028725624084148 ) ) ;
#64112=CARTESIAN_POINT ( 'NONE',  ( 5.017399365509065845, 8.011327138806002779, -1.199719254218450271 ) ) ;
#64120=CARTESIAN_POINT ( 'NONE',  ( -5.652823702255029836, 5.559658838911111900, -0.7998128361456362523 ) ) ;
#64125=CARTESIAN_POINT ( 'NONE',  ( -6.798487682609798632, 6.896266815991691779, 0.7998128361456341429 ) ) ;
#64129=CARTESIAN_POINT ( 'NONE',  ( 6.997416677984476863, 7.336276677169590421, 0.000000000000000000 ) ) ;
#64131=CARTESIAN_POINT ( 'NONE',  ( -6.305950843687521790, 7.489935751457798219, 1.082531754730548412 ) ) ;
#64137=CARTESIAN_POINT ( 'NONE',  ( 6.378184920586140727, 6.405913593630768510, 0.000000000000000000 ) ) ;
#64140=DIRECTION ( 'NONE',  ( 0.000000000000000000, 0.000000000000000000, 1.000000000000000000 ) ) ;
#64167=CARTESIAN_POINT ( 'NONE',  ( 4.675188888464441028, 8.274035074156913083, -0.5495550137140058355 ) ) ;
#64182=CARTESIAN_POINT ( 'NONE',  ( -5.591215426272092337, 7.404592667505576209, -1.242541652263975172 ) ) ;
#64190=CARTESIAN_POINT ( 'NONE',  ( -4.380693030546956912, 6.204170850428461392, 1.443375672974065660 ) ) ;
#64201=CARTESIAN_POINT ( 'NONE',  ( -5.340986169140711226, 5.195848383611072485, 0.000000000000000000 ) ) ;
#64211=CARTESIAN_POINT ( 'NONE',  ( 4.044074958626150185, 7.940114228364351767, 0.7998128361456271485 ) ) ;
#64215=CARTESIAN_POINT ( 'NONE',  ( 5.167065940139554669, 9.042344340222555843, -0.7216878364870458196 ) ) ;
#64218=ORIENTED_EDGE ( 'NONE', *, *, #116473, .F. ) ;
#64228=CARTESIAN_POINT ( 'NONE',  ( -6.286140498591554326, 7.362860665558790707, 1.199719254218452047 ) ) ;
#64229=CARTESIAN_POINT ( 'NONE',  ( 4.366607992053101128, 7.252070536440704096, -1.199719254218448494 ) ) ;
#64239=CARTESIAN_POINT ( 'NONE',  ( -5.562588163356775972, 9.711712967216715953, 0.7998128361456291469 ) ) ;
#64240=CARTESIAN_POINT ( 'NONE',  ( 5.830888582329017744, 8.960397891762626799, -1.199719254218452047 ) ) ;
#64247=CARTESIAN_POINT ( 'NONE',  ( 5.903649544107831382, 5.852288987739402870, -0.7998128361456481317 ) ) ;
#64254=CARTESIAN_POINT ( 'NONE',  ( -6.468510628652166972, 6.779004017053734898, -0.3101152288892006781 ) ) ;
#64263=CARTESIAN_POINT ( 'NONE',  ( -7.944151662964566540, 8.232874793072271657, 0.000000000000000000 ) ) ;
#64303=ORIENTED_EDGE ( 'NONE', *, *, #181711, .F. ) ;
#64311=CARTESIAN_POINT ( 'NONE',  ( 2.905190055078214595, 6.611415174225076186, 0.7998128361456271485 ) ) ;
#64312=CARTESIAN_POINT ( 'NONE',  ( -4.665414256878304577, 5.575976400180357118, -1.082531754730549967 ) ) ;
#64317=EDGE_CURVE ( 'NONE', #130628, #175863, #202393, .T. ) ;
#64327=ADVANCED_FACE ( 'NONE', ( #103867 ), #134653, .T. ) ;
#64343=CARTESIAN_POINT ( 'NONE',  ( -4.471156797456668386, 8.438376373666578445, -0.7998128361456362523 ) ) ;
#64345=CARTESIAN_POINT ( 'NONE',  ( 6.848276988234151652, 7.162280372460873679, -0.7216878364870317197 ) ) ;
#64350=CARTESIAN_POINT ( 'NONE',  ( -6.119526231721793330, 8.232809585132461194, 1.599625672291263179 ) ) ;
#64358=CARTESIAN_POINT ( 'NONE',  ( -6.635789839245807897, 6.706452665400368218, 0.7998128361456341429 ) ) ;
#64369=CARTESIAN_POINT ( 'NONE',  ( -6.310394152517827315, 6.326824364217716656, 0.7998128361456281477 ) ) ;
#64372=CARTESIAN_POINT ( 'NONE',  ( -5.641601317062239218, 8.635599732330991429, -1.082531754730549967 ) ) ;
#64373=CARTESIAN_POINT ( 'NONE',  ( -7.078765599666485997, 7.431183752465250869, 0.000000000000000000 ) ) ;
#64374=CARTESIAN_POINT ( 'NONE',  ( 6.363572996767764778, 8.517530811019446091, -1.599625672291283607 ) ) ;
#64375=CARTESIAN_POINT ( 'NONE',  ( -7.944151662964566540, 8.232874793072271657, 0.000000000000000000 ) ) ;
#64413=CARTESIAN_POINT ( 'NONE',  ( 5.694759483343039719, 7.307619849039811655, -1.219011658351103478 ) ) ;
#64428=EDGE_CURVE ( 'NONE', #112384, #13123, #108336, .T. ) ;
#64432=CARTESIAN_POINT ( 'NONE',  ( -3.494969737272722643, 7.299491470118629088, -0.7998128361456481317 ) ) ;
#64446=CARTESIAN_POINT ( 'NONE',  ( 4.573896719763862251, 6.429575154514868274, -1.599625672291273171 ) ) ;
#64448=CARTESIAN_POINT ( 'NONE',  ( 6.801350335910821165, 7.963938809097990124, 1.199719254218452047 ) ) ;
#64454=( BOUNDED_SURFACE ( )  B_SPLINE_SURFACE ( 3, 2, ( 
 ( #40850, #20293, #172982 ),
 ( #202229, #37625, #104779 ),
 ( #139414, #73311, #56016 ),
 ( #57082, #103705, #21343 ),
 ( #87453, #8320, #153520 ),
 ( #6166, #188136, #122170 ),
 ( #5089, #123247, #71164 ),
 ( #39767, #72235, #74405 ),
 ( #105872, #23495, #89601 ),
 ( #155652, #24561, #137281 ) ),
 .UNSPECIFIED., .F., .F., .T. ) 
 B_SPLINE_SURFACE_WITH_KNOTS ( ( 4, 2, 2, 2, 4 ),
 ( 3, 3 ),
 ( 0.000000000000000000, 0.0003762496586418675494, 0.0007524993172837350988, 0.001128748975925602648, 0.001504998634567470198 ),
 ( 0.000000000000000000, 1.000000000000000000 ),
 .UNSPECIFIED. ) 
 GEOMETRIC_REPRESENTATION_ITEM ( )  RATIONAL_B_SPLINE_SURFACE ( (
 ( 1.000000000000000000, 0.7127558927793078425, 1.000000000000000000),
 ( 1.000000000000000000, 0.7005070939717433776, 1.000000000000000000),
 ( 1.000000000000000000, 0.7091518804501668605, 1.000000000000000000),
 ( 1.000000000000000000, 0.7448155602382602325, 1.000000000000000000),
 ( 1.000000000000000000, 0.7694546621959588162, 1.000000000000000000),
 ( 1.000000000000000000, 0.7891761707070057419, 1.000000000000000000),
 ( 1.000000000000000000, 0.7831667280482919047, 1.000000000000000000),
 ( 1.000000000000000000, 0.7490304966219030192, 1.000000000000000000),
 ( 1.000000000000000000, 0.7236037604914373755, 1.000000000000000000),
 ( 1.000000000000000000, 0.7127552757490021040, 1.000000000000000000) ) ) 
 REPRESENTATION_ITEM ( '' )  SURFACE ( )  );
#64462=CARTESIAN_POINT ( 'NONE',  ( 6.225128807330042591, 7.291680359087043151, -1.199719254218452047 ) ) ;
#64477=CARTESIAN_POINT ( 'NONE',  ( -6.021229618244897885, 7.157760988441397743, 1.082531754730548412 ) ) ;
#64478=CARTESIAN_POINT ( 'NONE',  ( 5.397554552016216256, 7.390509292142662723, 1.443375672974065660 ) ) ;
#64488=CARTESIAN_POINT ( 'NONE',  ( -6.672020991700860826, 7.917017590806697314, 1.082531754730549078 ) ) ;
#64492=CARTESIAN_POINT ( 'NONE',  ( 4.624739795592929248, 6.488892076315451618, -1.443375672974068769 ) ) ;
#64507=CARTESIAN_POINT ( 'NONE',  ( 5.682802662783380754, 6.658966523782627434, 1.199719254218452935 ) ) ;
#64509=CARTESIAN_POINT ( 'NONE',  ( -5.340986169140711226, 5.195848383611072485, 0.000000000000000000 ) ) ;
#64522=CARTESIAN_POINT ( 'NONE',  ( 6.129694847154206983, 8.244672969803623630, -1.443375672974078761 ) ) ;
#64525=CARTESIAN_POINT ( 'NONE',  ( -6.363572996767778100, 8.517530811019446091, -1.599625672291271394 ) ) ;
#64526=CARTESIAN_POINT ( 'NONE',  ( 6.866278450678116485, 6.975356045404744521, 0.000000000000000000 ) ) ;
#64535=CARTESIAN_POINT ( 'NONE',  ( -5.152980901645737077, 8.169505597632108262, -1.199719254218453823 ) ) ;
#64546=EDGE_CURVE ( 'NONE', #194727, #77529, #177408, .T. ) ;
#64552=ORIENTED_EDGE ( 'NONE', *, *, #122982, .T. ) ;
#64562=CARTESIAN_POINT ( 'NONE',  ( 4.258669648468281110, 6.061810238003387141, 1.443375672974058777 ) ) ;
#64569=CARTESIAN_POINT ( 'NONE',  ( 4.950135482320912494, 6.868520377498098739, -1.443375672974068769 ) ) ;
#64582=CARTESIAN_POINT ( 'NONE',  ( -5.119085517611572378, 8.129960982925583224, 1.199719254218452935 ) ) ;
#64584=CARTESIAN_POINT ( 'NONE',  ( -7.259464905474441565, 7.434073576000447048, -0.7998128361456362523 ) ) ;
#64592=CARTESIAN_POINT ( 'NONE',  ( 5.501576472095266901, 9.640532660744973725, -0.7998128361456481317 ) ) ;
#64596=CARTESIAN_POINT ( 'NONE',  ( -5.611095471209320174, 7.639640364534566075, 1.599625672291263179 ) ) ;
#64602=CARTESIAN_POINT ( 'NONE',  ( -6.468648687495877958, 6.719380688266201496, 0.000000000000000000 ) ) ;
#64606=CARTESIAN_POINT ( 'NONE',  ( -6.069210040772897052, 7.109775131437022999, -1.199719254218453823 ) ) ;
#64627=CARTESIAN_POINT ( 'NONE',  ( -6.071018923869249129, 10.30488218781460574, 0.7998128361456291469 ) ) ;
#64628=CARTESIAN_POINT ( 'NONE',  ( 5.259637247458703868, 5.100941308315409373, 0.000000000000000000 ) ) ;
#64629=CARTESIAN_POINT ( 'NONE',  ( -5.336015975430226099, 8.383046517047350932, -1.199719254218453823 ) ) ;
#64647=CARTESIAN_POINT ( 'NONE',  ( 4.990809943606266508, 6.915973915664348937, -1.443375672974068769 ) ) ;
#64651=CARTESIAN_POINT ( 'NONE',  ( -5.257529707049291900, 9.355811434857983500, 0.7998128361456291469 ) ) ;
#64675=CARTESIAN_POINT ( 'NONE',  ( 5.110497557708379546, 4.926945003606695295, -0.7998128361456481317 ) ) ;
#64688=CARTESIAN_POINT ( 'NONE',  ( 4.794097012578165007, 8.135614534340449566, -0.8214339667521903809 ) ) ;
#64690=CARTESIAN_POINT ( 'NONE',  ( 6.021229618244865023, 10.03886863134542828, -0.7216878364870458196 ) ) ;
#64695=CARTESIAN_POINT ( 'NONE',  ( -6.069210040772897052, 7.109775131437022999, -1.199719254218453823 ) ) ;
#64704=CARTESIAN_POINT ( 'NONE',  ( -4.041773898501059392, 7.631402218382003610, 0.4027767917945597742 ) ) ;
#64710=CARTESIAN_POINT ( 'NONE',  ( -5.472651281771599763, 6.413789912602166687, 1.199719254218452935 ) ) ;
#64720=CARTESIAN_POINT ( 'NONE',  ( 3.237364818613055473, 6.998952398349030268, -1.734723475976807094E-15 ) ) ;
#64743=CARTESIAN_POINT ( 'NONE',  ( -5.725286006720766707, 9.901527117808042178, 0.7998128361456291469 ) ) ;
#64753=CARTESIAN_POINT ( 'NONE',  ( 5.123001941117305336, 7.070197912760590064, 1.599625672291268286 ) ) ;
#64765=CARTESIAN_POINT ( 'NONE',  ( 7.349928672384120176, 7.747540670635879145, 0.7216878364870267237 ) ) ;
#64766=ORIENTED_EDGE ( 'NONE', *, *, #156259, .F. ) ;
#64776=CARTESIAN_POINT ( 'NONE',  ( -6.129694847154220305, 8.244672969803623630, -1.443375672974066548 ) ) ;
#64798=CARTESIAN_POINT ( 'NONE',  ( 5.596450457127522427, 5.765155227950554462, 0.6767625585771692709 ) ) ;
#64808=CARTESIAN_POINT ( 'NONE',  ( 6.201928923608456046, 6.200281597156833691, 0.7998128361456352531 ) ) ;
#64810=CARTESIAN_POINT ( 'NONE',  ( 4.376249722160992839, 8.327651452488305850, 0.000000000000000000 ) ) ;
#64822=CARTESIAN_POINT ( 'NONE',  ( -5.334207092333882017, 5.187939460669764635, 0.7998128361456281477 ) ) ;
#64827=CARTESIAN_POINT ( 'NONE',  ( 4.380693030546905398, 8.124909279031149012, 0.7216878364870247253 ) ) ;
#64839=CARTESIAN_POINT ( 'NONE',  ( -5.397554552016258889, 7.390509292142662723, 1.443375672974058777 ) ) ;
#64841=CARTESIAN_POINT ( 'NONE',  ( -5.641601317062248988, 6.714861303728305586, -1.082531754730549967 ) ) ;
#64845=CARTESIAN_POINT ( 'NONE',  ( 0.000000000000000000, 8.920000000000001705, 0.000000000000000000 ) ) ;
#64855=EDGE_CURVE ( 'NONE', #148211, #99015, #197205, .T. ) ;
#64857=CIRCLE ( 'NONE', #40769, 2.000000000000000000 ) ;
#64859=CARTESIAN_POINT ( 'NONE',  ( -2.972980823146582186, 6.690504403638126263, 0.000000000000000000 ) ) ;
#64870=CARTESIAN_POINT ( 'NONE',  ( -4.679499295372141709, 5.488445928469455559, 1.199719254218452935 ) ) ;
#64879=CARTESIAN_POINT ( 'NONE',  ( -5.887983850084758330, 10.09134126839936840, 0.7998128361456291469 ) ) ;
#64880=CARTESIAN_POINT ( 'NONE',  ( -4.804518813248800591, 8.239360463340183571, 0.8967481634083998010 ) ) ;
#64899=CARTESIAN_POINT ( 'NONE',  ( 7.361151057576892143, 7.552707420120024828, 0.7998128361456291469 ) ) ;
#64921=CARTESIAN_POINT ( 'NONE',  ( 6.964048179274811012, 8.153752959689313684, 1.199719254218452047 ) ) ;
#64922=CARTESIAN_POINT ( 'NONE',  ( 5.574337433874081427, 6.532423756721743580, -1.199719254218452047 ) ) ;
#64925=CARTESIAN_POINT ( 'NONE',  ( 3.553118775233146120, 6.302999783484076524, -1.199719254218453823 ) ) ;
#64935=CARTESIAN_POINT ( 'NONE',  ( 4.601164721245145195, 8.482418317249249995, 0.1585857521721554253 ) ) ;
#64936=CARTESIAN_POINT ( 'NONE',  ( -4.285785955251283141, 8.014184357852876417, 0.000000000000000000 ) ) ;
#64937=CARTESIAN_POINT ( 'NONE',  ( 5.234856708652233515, 6.240325927249993576, 1.082531754730549078 ) ) ;
#64959=CARTESIAN_POINT ( 'NONE',  ( 4.854701522145073334, 7.821512988214679218, -1.199719254218450271 ) ) ;
#64961=CARTESIAN_POINT ( 'NONE',  ( 3.464990776744291345, 6.200183785247111778, 1.199719254218452047 ) ) ;
#64977=CARTESIAN_POINT ( 'NONE',  ( -6.957269102468015554, 8.145844036748005834, 1.199719254218452047 ) ) ;
#64987=CARTESIAN_POINT ( 'NONE',  ( 7.015418140428412386, 7.149352350113456822, 0.7998128361456331437 ) ) ;
#64990=AXIS2_PLACEMENT_3D ( 'NONE', #113887, #47773, #30439 ) ;
#64992=CARTESIAN_POINT ( 'NONE',  ( 5.387385936583818591, 7.378645907471495846, -1.599625672291283607 ) ) ;
#65002=CARTESIAN_POINT ( 'NONE',  ( -1.919948509414037163, 8.999999999999998224, 0.7750000000000013545 ) ) ;
#65004=CARTESIAN_POINT ( 'NONE',  ( 4.693755526227673336, 8.251780594207492214, -0.6034641085399840010 ) ) ;
#65019=CARTESIAN_POINT ( 'NONE',  ( 4.934241560730721510, 4.721313007132757811, 0.000000000000000000 ) ) ;
#65025=CARTESIAN_POINT ( 'NONE',  ( -6.903036488013351679, 8.082572653217566128, -1.199719254218452047 ) ) ;
#65027=CARTESIAN_POINT ( 'NONE',  ( 6.062430963966053632, 7.101866208495718702, -1.199719254218452047 ) ) ;
#65031=CARTESIAN_POINT ( 'NONE',  ( -5.413448473606448985, 9.537716662508005427, 0.000000000000000000 ) ) ;
#65040=CARTESIAN_POINT ( 'NONE',  ( -6.175853536056814086, 7.055546168579414079, -1.074032317439767903 ) ) ;
#65052=ORIENTED_EDGE ( 'NONE', *, *, #40506, .T. ) ;
#65055=CARTESIAN_POINT ( 'NONE',  ( 5.722950238744198614, 8.730506807626655430, 1.082531754730549967 ) ) ;
#65058=CARTESIAN_POINT ( 'NONE',  ( -7.533490631048818109, 8.818102486758951031, -1.199719254218452047 ) ) ;
#65069=CARTESIAN_POINT ( 'NONE',  ( -3.350273356352693188, 6.922752992471175482, 0.000000000000000000 ) ) ;
#65072=CARTESIAN_POINT ( 'NONE',  ( 6.225128807330042591, 7.291680359087043151, -1.199719254218452047 ) ) ;
#65090=CARTESIAN_POINT ( 'NONE',  ( 8.122743427918724279, 8.649157885426255632, 0.7216878364870267237 ) ) ;
#65114=CARTESIAN_POINT ( 'NONE',  ( 6.116136693540529912, 10.14959355252369910, 1.530808498934192557E-16 ) ) ;
#65119=CARTESIAN_POINT ( 'NONE',  ( 3.542423274920540432, 7.354853930707762721, -1.734723475976807094E-15 ) ) ;
#65122=CARTESIAN_POINT ( 'NONE',  ( -1.807716826991530024, 2.517780620582464213, 2.499994708711103630 ) ) ;
#65123=ORIENTED_EDGE ( 'NONE', *, *, #173439, .F. ) ;
#65124=CARTESIAN_POINT ( 'NONE',  ( -4.272227801637618505, 7.998366511970260717, 0.7216878364870338292 ) ) ;
#65130=CARTESIAN_POINT ( 'NONE',  ( -6.296835998904160014, 6.311006518335105397, 0.000000000000000000 ) ) ;
#65138=AXIS2_PLACEMENT_3D ( 'NONE', #202485, #50938, #134354 ) ;
#65139=CARTESIAN_POINT ( 'NONE',  ( -6.469175572376043348, 7.576401584974034265, 1.199719254218452047 ) ) ;
#65141=CARTESIAN_POINT ( 'NONE',  ( 6.582202237817778467, 6.781708767774706104, 0.2773405359152263383 ) ) ;
#65146=CARTESIAN_POINT ( 'NONE',  ( 5.668190738965027897, 8.770583741171307679, -1.199719254218452047 ) ) ;
#65153=CARTESIAN_POINT ( 'NONE',  ( -3.630551273409382329, 7.457669928944732796, 0.7998128361456352531 ) ) ;
#65159=CARTESIAN_POINT ( 'NONE',  ( -5.098748287191073203, 8.106234214101666780, 1.199719254218452935 ) ) ;
#65162=CARTESIAN_POINT ( 'NONE',  ( -3.618674974218159868, 7.443814246554973479, 0.3006916729143232492 ) ) ;
#65163=CARTESIAN_POINT ( 'NONE',  ( 6.224601922005513543, 7.395028676162137771, -1.082531754730548412 ) ) ;
#65165=CARTESIAN_POINT ( 'NONE',  ( -6.034787771414192648, 9.094317262408276648, 1.082531754730549967 ) ) ;
#65171=CARTESIAN_POINT ( 'NONE',  ( 4.532168488718122390, 8.509556680138327778, 0.7998128361456271485 ) ) ;
#65172=EDGE_LOOP ( 'NONE', ( #202957, #52644, #59305, #7216 ) ) ;
#65180=CARTESIAN_POINT ( 'NONE',  ( -2.744103632728948305, 3.021832644587346017, -2.500000000000000444 ) ) ;
#65195=CARTESIAN_POINT ( 'NONE',  ( 5.495418255317095380, 6.026204583819558813, -0.7979391942483995415 ) ) ;
#65200=CARTESIAN_POINT ( 'NONE',  ( 4.794097012578165007, 8.135614534340449566, -0.8214339667521903809 ) ) ;
#65208=CARTESIAN_POINT ( 'NONE',  ( 7.991605200612358573, 8.288237253661408843, 0.7998128361456281477 ) ) ;
#65214=CARTESIAN_POINT ( 'NONE',  ( -5.575295409310188965, 7.417394932307940003, -1.244639187630245170 ) ) ;
#65233=CARTESIAN_POINT ( 'NONE',  ( -3.305155586681401303, 7.078041627762083898, 0.7998128361456352531 ) ) ;
#65239=ORIENTED_EDGE ( 'NONE', *, *, #202346, .T. ) ;
#65240=VERTEX_POINT ( 'NONE', #149532 ) ;
#65243=CARTESIAN_POINT ( 'NONE',  ( 5.987861119090863049, 7.014868056141362551, 1.199719254218452047 ) ) ;
#65244=CARTESIAN_POINT ( 'NONE',  ( 5.553597010146855695, 5.912075037831448832, 0.6282849591137803502 ) ) ;
#65247=CARTESIAN_POINT ( 'NONE',  ( 5.302647476276220573, 8.240153584747313076, -1.082531754730548412 ) ) ;
#65263=CARTESIAN_POINT ( 'NONE',  ( -4.447956913735107598, 7.346977611736363656, 1.199719254218452935 ) ) ;
#65264=CARTESIAN_POINT ( 'NONE',  ( 5.401997860402196316, 5.267028690082820930, 0.000000000000000000 ) ) ;
#65273=CARTESIAN_POINT ( 'NONE',  ( -3.169574050544739841, 6.919863168935977527, -0.7998128361456481317 ) ) ;
#65274=CARTESIAN_POINT ( 'NONE',  ( 5.494797395288433250, 9.632623737803665875, 0.000000000000000000 ) ) ;
#65280=CARTESIAN_POINT ( 'NONE',  ( 4.848976215542928792, 5.686169002002086970, 1.199719254218452047 ) ) ;
#65286=CARTESIAN_POINT ( 'NONE',  ( -6.564228937702958788, 6.791309396811020527, 0.4070866938790471679 ) ) ;
#65294=CARTESIAN_POINT ( 'NONE',  ( -7.095713291905736853, 9.371694488680407886, 1.599625672291269396 ) ) ;
#65295=CARTESIAN_POINT ( 'NONE',  ( -7.930593509350902792, 8.217056947189661287, -0.7998128361456362523 ) ) ;
#65305=DIRECTION ( 'NONE',  ( 0.6507913734559658270, -0.7592566023652989049, 0.000000000000000000 ) ) ;
#65307=CARTESIAN_POINT ( 'NONE',  ( -3.809456170543987330, 8.470288933811271903, 2.500000000000000444 ) ) ;
#65344=CARTESIAN_POINT ( 'NONE',  ( 8.000720045840086669, 8.506797273001177828, 0.7216878364870267237 ) ) ;
#65372=CARTESIAN_POINT ( 'NONE',  ( -5.143339171537843590, 7.093924681584509173, 1.599625672291263179 ) ) ;
#65374=CARTESIAN_POINT ( 'NONE',  ( 6.495764994278797388, 8.671754808115688107, 1.443375672974063439 ) ) ;
#65380=CARTESIAN_POINT ( 'NONE',  ( -5.271087860662956537, 9.371629280740593870, 0.000000000000000000 ) ) ;
#65384=DIRECTION ( 'NONE',  ( 0.000000000000000000, 0.000000000000000000, -1.000000000000000000 ) ) ;
#65388=CARTESIAN_POINT ( 'NONE',  ( -5.773793314573309132, 7.829454515125894964, 1.599625672291263179 ) ) ;
#65401=CARTESIAN_POINT ( 'NONE',  ( -4.613517410400161722, 8.604463755433990002, -0.7998128361456362523 ) ) ;
#65404=CARTESIAN_POINT ( 'NONE',  ( -6.211043768836215229, 8.339580045099285854, 1.443375672974064550 ) ) ;
#65406=CARTESIAN_POINT ( 'NONE',  ( -7.227905289416814760, 7.605180057173966723, -0.7216878364870338292 ) ) ;
#65407=CARTESIAN_POINT ( 'NONE',  ( 5.854088466050551887, 10.05179665369283981, 0.7998128361456341429 ) ) ;
#65408=CARTESIAN_POINT ( 'NONE',  ( -4.624739795592943459, 6.488892076315448065, -1.443375672974066548 ) ) ;
#65427=CARTESIAN_POINT ( 'NONE',  ( 6.548892101489681927, 6.803534504848940401, 0.4251794856353352525 ) ) ;
#65445=CARTESIAN_POINT ( 'NONE',  ( 6.053075614097062740, 7.042710966267798689, -1.019147762646470001 ) ) ;
#65460=CARTESIAN_POINT ( 'NONE',  ( 7.686546744304875389, 7.932335721302671949, 0.7998128361456291469 ) ) ;
#65463=CARTESIAN_POINT ( 'NONE',  ( -4.685224601974262271, 7.623789914682047808, -1.199719254218453823 ) ) ;
#65467=CARTESIAN_POINT ( 'NONE',  ( -6.238160075619175515, 10.29195416494877513, 0.000000000000000000 ) ) ;
#65478=CARTESIAN_POINT ( 'NONE',  ( 3.250922972226694352, 7.014770244231638863, 0.7998128361456281477 ) ) ;
#65480=CARTESIAN_POINT ( 'NONE',  ( 5.722423353419669567, 8.833855124701747386, 1.199719254218451159 ) ) ;
#65488=CARTESIAN_POINT ( 'NONE',  ( -5.709392084686210289, 8.714688961225625974, 1.082531754730550855 ) ) ;
#65494=VERTEX_POINT ( 'NONE', #171105 ) ;
#65495=CARTESIAN_POINT ( 'NONE',  ( 7.014364370223726830, 9.276787413384745662, -1.599625672291269396 ) ) ;
#65499=CARTESIAN_POINT ( 'NONE',  ( 1.843739406749204335, 8.920000000000001705, 0.7750000000000004663 ) ) ;
#65508=CARTESIAN_POINT ( 'NONE',  ( -4.665414256878287702, 8.457084043084382330, -0.7216878364870338292 ) ) ;
#65509=CARTESIAN_POINT ( 'NONE',  ( 5.777182853198898904, 6.873039762554409293, -1.082531754730548412 ) ) ;
#65520=CARTESIAN_POINT ( 'NONE',  ( -5.008811405605897882, 4.808311159487113073, 0.7998128361456281477 ) ) ;
#65521=CARTESIAN_POINT ( 'NONE',  ( -6.617788377246196951, 7.853746207276256719, -1.082531754730549967 ) ) ;
#65522=CARTESIAN_POINT ( 'NONE',  ( 1.834945990282811579, 2.515477056191848249, -2.498594247320889306 ) ) ;
#65526=CARTESIAN_POINT ( 'NONE',  ( 4.190878879955609371, 7.903459436674603822, -0.7216878364870338292 ) ) ;
#65541=AXIS2_PLACEMENT_3D ( 'NONE', #31946, #212802, #195510 ) ;
#65543=CARTESIAN_POINT ( 'NONE',  ( -5.276058054373441664, 6.184431147304315424, -1.199719254218453823 ) ) ;
#65554=CARTESIAN_POINT ( 'NONE',  ( 8.014278199453778839, 8.522615118883788199, 0.000000000000000000 ) ) ;
#65557=CARTESIAN_POINT ( 'NONE',  ( 4.844006021832467646, 8.873367135438366304, 0.000000000000000000 ) ) ;
#65565=CARTESIAN_POINT ( 'NONE',  ( -6.123442655227560927, 7.173046514967467147, 1.199719254218452047 ) ) ;
#65580=ORIENTED_EDGE ( 'NONE', *, *, #143009, .F. ) ;
#65590=CARTESIAN_POINT ( 'NONE',  ( 4.421367491832270957, 6.251624388594711590, 1.443375672974058777 ) ) ;
#65596=CARTESIAN_POINT ( 'NONE',  ( 5.858531774436539052, 6.007577623030311287, 0.000000000000000000 ) ) ;
#65607=CARTESIAN_POINT ( 'NONE',  ( -5.281783360975562225, 8.319775133516907673, 1.199719254218452935 ) ) ;
#65609=CARTESIAN_POINT ( 'NONE',  ( -6.720001414228860881, 7.869031733802326123, -1.199719254218452047 ) ) ;
#65617=CARTESIAN_POINT ( 'NONE',  ( 5.840530312436913007, 10.03597880781023299, 0.000000000000000000 ) ) ;
#65623=CARTESIAN_POINT ( 'NONE',  ( -5.608135385276092677, 5.599224824533729716, 0.4022279080854191391 ) ) ;
#65624=CARTESIAN_POINT ( 'NONE',  ( -6.994027139803241866, 9.253060644560830994, -1.599625672291271394 ) ) ;
#65630=( BOUNDED_CURVE ( )  B_SPLINE_CURVE ( 2, ( #66737, #55597, #31103, #64647, #116651, #33209, #83016 ),
 .UNSPECIFIED., .F., .T. ) 
 B_SPLINE_CURVE_WITH_KNOTS ( ( 3, 2, 2, 3 ),
 ( 0.3500000000000000888, 0.3583333333333333925, 0.3666666666666665853, 0.3749999999999998890 ),
 .UNSPECIFIED. ) 
 CURVE ( )  GEOMETRIC_REPRESENTATION_ITEM ( )  RATIONAL_B_SPLINE_CURVE ( ( 0.9999999999999982236, 0.8660254037844404840, 1.000000000000000000, 0.8660254037844387076, 1.000000000000000000, 0.8660254037844404840, 0.9999999999999982236 ) ) 
 REPRESENTATION_ITEM ( '' )  );
#65632=CARTESIAN_POINT ( 'NONE',  ( -6.305950844131887223, 6.529566537674873494, 0.000000000000000000 ) ) ;
#65635=CARTESIAN_POINT ( 'NONE',  ( -5.529746549527323474, 7.544733289238903851, -1.599625672291271394 ) ) ;
#65652=CARTESIAN_POINT ( 'NONE',  ( -6.504227504688391726, 6.823496289112537916, 0.6761912409562121917 ) ) ;
#65655=CARTESIAN_POINT ( 'NONE',  ( -5.329763783947941036, 5.390681634126922361, 0.000000000000000000 ) ) ;
#65657=CARTESIAN_POINT ( 'NONE',  ( -4.136646265500970365, 5.919449624541475607, -1.443375672974066548 ) ) ;
#65658=CARTESIAN_POINT ( 'NONE',  ( 3.573456005653643519, 6.326726552307992080, -1.199719254218453823 ) ) ;
#65659=CARTESIAN_POINT ( 'NONE',  ( -6.818824913030298696, 6.919993584815607335, 0.7998128361456341429 ) ) ;
#65660=ORIENTED_EDGE ( 'NONE', *, *, #199073, .T. ) ;
#65709=CARTESIAN_POINT ( 'NONE',  ( 3.953084306836263995, 6.769626237021087789, 1.199719254218452047 ) ) ;
#65711=CARTESIAN_POINT ( 'NONE',  ( -4.207966135563095733, 7.175396087857926375, 7.500000000000000000 ) ) ;
#65722=CARTESIAN_POINT ( 'NONE',  ( 4.614363445337835934, 8.349151705029461468, -0.2795175495247017583 ) ) ;
#65724=CARTESIAN_POINT ( 'NONE',  ( 4.065465959251388206, 5.836405933916976707, -1.599625672291269396 ) ) ;
#65725=ADVANCED_FACE ( 'NONE', ( #213967 ), #100246, .F. ) ;
#65731=CARTESIAN_POINT ( 'NONE',  ( -6.771371375382467583, 6.864631124226471037, -0.7998128361456362523 ) ) ;
#65736=CARTESIAN_POINT ( 'NONE',  ( -8.041394506236766659, 8.554250810130591631, -0.7216878364870338292 ) ) ;
#65745=EDGE_CURVE ( 'NONE', #40807, #198442, #19718, .T. ) ;
#65747=CARTESIAN_POINT ( 'NONE',  ( -5.147255595043616516, 6.034161611419515125, 1.199719254218452935 ) ) ;
#65757=CARTESIAN_POINT ( 'NONE',  ( 5.520104819419390907, 6.469152373191302985, 1.199719254218452935 ) ) ;
#65785=CARTESIAN_POINT ( 'NONE',  ( 6.343235766347262938, 8.493804042195527870, -1.599625672291281386 ) ) ;
#65786=CARTESIAN_POINT ( 'NONE',  ( 3.719872605471106208, 6.605953636083950364, 7.500000000000000000 ) ) ;
#65791=B_SPLINE_SURFACE_WITH_KNOTS ( 'NONE', 1, 3, ( 
 ( #107176, #142848, #123464, #41069, #43206, #72462, #93020, #208852, #173202, #58366, #124519, #158016, #56234, #138562, #190477, #42136, #108251, #174272, #25847, #91955, #17848, #79929, #194750, #29062, #2660, #178515, #94087, #83933, #163331, #144979, #167334, #128772, #127722, #150022, #134854, #177449, #51453, #44258, #13853, #160127, #193681, #95146, #30126, #162266, #176385, #161197, #68733, #35174, #209918, #110381, #210983, #96215, #146035, #101251, #1592, #46386, #62611, #27991, #112504, #11726, #129843, #212048, #12784, #78857, #63687, #77802, #18920, #45324, #61556, #67653, #133799, #111444, #199809, #195825, #47464, #113579, #143922, #179581, #31203, #117573, #183568, #97277, #85005, #151096, #69795, #89296, #74101, #119709, #205136, #200860, #170519, #102321, #135904, #185691, #186766, #104472, #118640, #103395, #156424, #188902, #152150, #52507, #87140, #38392, #22101, #40544, #23181, #203001, #4781, #184625, #153211, #36242, #71931, #88214, #37321, #169456, #54641, #19991, #106648, #201922, #3720, #6930, #171588, #56779, #154285, #21043, #53575, #70859, #122945, #136974, #5859, #105553, #55706, #24252, #90356, #168394, #139108, #120789, #138041, #155347, #86075, #172675, #204054, #121860, #187831, #39458, #73009, #8010, #126130, #142335, #158553, #178009, #57841, #109870, #91437, #62121, #25336, #206215, #107734, #93571, #94640, #92514, #58914, #124004, #110929, #209402, #29626, #128281, #144478, #157498, #159616, #193175, #189971, #175883, #42694, #61047, #41620, #9093, #10149, #194243, #208345, #45887, #75169, #141279, #12279, #161764, #112008, #95711, #207287, #26403, #191027, #44824, #125070, #13356, #108800, #210484, #140193, #11213, #173759, #76224, #174826, #192090, #59976, #43757, #27473, #77294, #143406, #127207, #176934, #28551, #160684, #78357, #100999, #64254, #99948, #33870, #130397, #63181 ),
 ( #181189, #198489, #148702, #117323, #183321, #195323, #17598, #180136, #131433, #50134, #211545, #51201, #31764, #129345, #81559, #146596, #271, #82617, #65286, #147643, #97834, #34925, #46954, #49076, #30699, #1346, #179077, #145548, #113072, #32816, #166012, #163899, #212614, #96780, #116256, #66342, #167088, #67408, #83682, #162831, #98890, #132487, #14409, #115196, #196387, #182245, #80499, #48030, #15475, #133549, #213661, #199557, #114144, #197435, #149771, #79430, #164943, #16535, #85826, #119458, #69546, #71683, #118390, #72765, #35997, #89048, #188659, #137796, #121615, #102078, #203815, #54402, #169208, #3479, #40288, #152962, #68486, #55460, #187584, #185445, #138864, #103147, #168146, #39210, #106398, #151905, #22932, #18679, #202749, #134613, #19746, #135656, #4536, #136725, #150845, #201679, #84758, #6690, #184378, #2409, #105301, #171338, #53325, #155105, #120541, #20799, #37066, #200616, #70610, #52263, #204882, #56534, #86895, #122696, #186520, #38150, #104222, #170269, #21854, #87961, #154035, #5601, #73847, #107484, #91184, #158313, #75980, #90113, #74917, #128030, #160429, #123759, #172422, #58664, #9904, #142083, #12034, #209155, #174576, #190778, #156180, #124815, #24012, #43506, #208098, #8838, #157245, #26153, #205968, #78106, #41373, #189721, #192912, #143161, #176682, #59726, #207034, #173509, #25082, #28294, #141027, #125885, #77033, #27218, #210227, #61865, #139941, #110684, #42441, #191843, #60794, #7759, #144233, #108545, #57600, #92267, #109627, #93324, #175632, #159360, #10958, #126953, #193984, #44568, #94390, #45632, #33620, #211297, #177755, #79175, #65040, #66086, #63995, #30443, #95466, #82364, #180935, #149510, #99691, #116000, #129089, #131195, #164692, #161514, #81313, #14150, #32556, #29370, #62921, #196137, #165761, #113890, #17346, #46699, #112816, #198238, #133291, #83428 ) ),
 .UNSPECIFIED., .F., .T., .F.,
 ( 2, 2 ),
 ( 4, 2, 2, 2, 2, 2, 2, 2, 2, 2, 2, 2, 2, 2, 2, 2, 2, 2, 2, 2, 2, 2, 2, 2, 2, 2, 2, 2, 2, 2, 2, 2, 2, 2, 2, 2, 2, 2, 2, 2, 2, 2, 2, 2, 2, 2, 2, 2, 2, 2, 2, 2, 2, 2, 2, 2, 2, 2, 2, 2, 2, 2, 2, 2, 2, 2, 2, 2, 2, 2, 2, 2, 2, 2, 2, 2, 2, 2, 2, 2, 2, 2, 2, 2, 2, 2, 2, 2, 2, 2, 2, 2, 2, 2, 2, 2, 2, 2, 2, 2, 2, 2, 2, 2, 2, 2, 2, 2, 4 ),
 ( 0.000000000000000000, 1.000000000000000000 ),
 ( -5.017377349295429334E-06, 6.045441312669188748E-05, 0.0001259262036026792043, 0.0002568697845546538379, 0.0003878133655066284716, 0.0004205492607446221706, 0.0004532851559826158155, 0.0005187569464586031052, 0.0005842287369345903949, 0.0006497005274105776846, 0.0007806441083625523724, 0.0008461158988385397706, 0.0009115876893145270603, 0.0009770594797905143500, 0.001042531270266501640, 0.001173474851218476219, 0.001238946641694463509, 0.001304418432170450799, 0.001369890222646438088, 0.001435362013122425378, 0.001500833803598412668, 0.001566305594074400174, 0.001631777384550387681, 0.001697249175026374970, 0.001762720965502362260, 0.001828192755978349550, 0.001893664546454336840, 0.001959136336930324129, 0.002090079917882298709, 0.002155551708358285998, 0.002221023498834273288, 0.002286495289310260578, 0.002351967079786247868, 0.002482910660738222447, 0.002548382451214209737, 0.002613854241690197026, 0.002679326032166184316, 0.002744797822642171606, 0.002810269613118158896, 0.002875741403594146185, 0.003006684984546120765, 0.003072156775022108488, 0.003137628565498095778, 0.003203100355974083067, 0.003268572146450070791, 0.003399515727402045370, 0.003530459308354019950, 0.003563195203592013811, 0.003595931098830007239, 0.003661402889305994529, 0.003726874679781981819, 0.003792346470257969109, 0.003923290051209943688, 0.003988761841685931411, 0.004054233632161918267, 0.004119705422637905123, 0.004185177213113892847, 0.004250649003589880570, 0.004316120794065867426, 0.004381592584541854282, 0.004447064375017842006, 0.004578007955969816585, 0.004643479746445803441, 0.004708951536921791164, 0.004774423327397778888, 0.004839895117873765744, 0.004970838698825740323, 0.005101782279777714903, 0.005232725860729689482, 0.005363669441681664062, 0.005494613022633638641, 0.005625556603585613220, 0.005691028394061600076, 0.005756500184537587800, 0.005821971975013575523, 0.005887443765489562379, 0.006018387346441536959, 0.006083859136917524682, 0.006149330927393512405, 0.006214802717869500129, 0.006280274508345486985, 0.006411218089297461564, 0.006476689879773449288, 0.006542161670249437011, 0.006607633460725424734, 0.006673105251201411590, 0.006738577041677398446, 0.006804048832153386170, 0.006869520622629373893, 0.006934992413105360749, 0.007000464203581347605, 0.007065935994057335329, 0.007131407784533323052, 0.007196879575009309908, 0.007327823155961284488, 0.007393294946437272211, 0.007458766736913259067, 0.007491502632151252061, 0.007524238527389245923, 0.007589710317865233646, 0.007720653898817208226, 0.007786125689293195082, 0.007851597479769182805, 0.007917069270245168794, 0.007982541060721156517, 0.008113484641673131964, 0.008244428222625107411, 0.008309900013101095134, 0.008375371803577081123 ),
 .UNSPECIFIED. ) ;
#65793=CARTESIAN_POINT ( 'NONE',  ( 4.231553341240963384, 7.950912974840849579, -0.7216878364870357165 ) ) ;
#65797=CARTESIAN_POINT ( 'NONE',  ( 5.994113311017540191, 9.046863725278862844, -1.082531754730548412 ) ) ;
#65798=ORIENTED_EDGE ( 'NONE', *, *, #10571, .T. ) ;
#65806=DIRECTION ( 'NONE',  ( -0.6507913734559559460, 0.7592566023653074536, 0.000000000000000000 ) ) ;
#65809=CARTESIAN_POINT ( 'NONE',  ( -7.593975437430151132, 8.032261896522864930, -0.7216878364870338292 ) ) ;
#65836=CARTESIAN_POINT ( 'NONE',  ( 4.190878879955592495, 7.903459436674620697, -0.7216878364870198403 ) ) ;
#65839=CARTESIAN_POINT ( 'NONE',  ( 1.843739406749228538, 9.999999999999998224, -0.7749999999999996891 ) ) ;
#65846=CARTESIAN_POINT ( 'NONE',  ( 4.583538449871731757, 7.505156070562471804, 1.199719254218451159 ) ) ;
#65848=CARTESIAN_POINT ( 'NONE',  ( 5.550083779947807550, 7.568460058062819407, -1.599625672291283607 ) ) ;
#65859=CARTESIAN_POINT ( 'NONE',  ( -4.821859908315634158, 5.654533310236863564, 1.199719254218452935 ) ) ;
#65862=CARTESIAN_POINT ( 'NONE',  ( 5.844973620822844218, 5.991759777147701804, 0.7216878364870328300 ) ) ;
#65871=CARTESIAN_POINT ( 'NONE',  ( -5.469788628470539926, 5.346117919495872783, -0.7998128361456362523 ) ) ;
#65878=CARTESIAN_POINT ( 'NONE',  ( -7.756673280794142755, 8.222076047114187602, -0.7216878364870338292 ) ) ;
#65880=CARTESIAN_POINT ( 'NONE',  ( -4.326460416536637155, 8.061637896019123062, 0.000000000000000000 ) ) ;
#65893=EDGE_CURVE ( 'NONE', #164262, #44, #98147, .T. ) ;
#65908=CARTESIAN_POINT ( 'NONE',  ( -3.980200614063634568, 6.801261928786307642, 1.199719254218452935 ) ) ;
#65918=CARTESIAN_POINT ( 'NONE',  ( 3.633153978699183995, 3.497932562452356731, -2.447764766412549697 ) ) ;
#65919=CARTESIAN_POINT ( 'NONE',  ( -4.620524454801235414, 8.454239455966142458, -0.3877863265914320845 ) ) ;
#65921=FACE_OUTER_BOUND ( 'NONE', #65172, .T. ) ;
#65935=CARTESIAN_POINT ( 'NONE',  ( 5.040599249230596435, 9.102725900736217568, 0.7998128361456341429 ) ) ;
#65952=CARTESIAN_POINT ( 'NONE',  ( 7.041790712887754822, 6.002124920821316323, 2.446252293856579829 ) ) ;
#65959=CARTESIAN_POINT ( 'NONE',  ( 6.099189001301251523, 8.209082816308541197, 1.599625672291268286 ) ) ;
#65960=CARTESIAN_POINT ( 'NONE',  ( 6.886615681098613884, 6.999082814228660077, 0.000000000000000000 ) ) ;
#65962=CARTESIAN_POINT ( 'NONE',  ( 3.718679271898170491, 7.560485927181699317, 0.7998128361456271485 ) ) ;
#65972=CARTESIAN_POINT ( 'NONE',  ( 4.639288533706844575, 8.435234533841581950, -0.4270733708018232822 ) ) ;
#65974=CARTESIAN_POINT ( 'NONE',  ( -6.739811759324840779, 7.035737605399991601, -0.7216878364870338292 ) ) ;
#65975=CARTESIAN_POINT ( 'NONE',  ( 4.909461021924254709, 5.860697626067345567, 1.082531754730549078 ) ) ;
#66000=CARTESIAN_POINT ( 'NONE',  ( 4.583538449871731757, 7.505156070562471804, 1.199719254218451159 ) ) ;
#66002=CARTESIAN_POINT ( 'NONE',  ( 5.259637247458703868, 5.100941308315409373, 0.000000000000000000 ) ) ;
#66013=DIRECTION ( 'NONE',  ( 0.6507913734559775953, 0.7592566023652888019, 0.000000000000000000 ) ) ;
#66022=CARTESIAN_POINT ( 'NONE',  ( -4.195212134638190982, 7.860597793832757141, -0.3698817738262829558 ) ) ;
#66032=CARTESIAN_POINT ( 'NONE',  ( 6.554440917563797875, 6.611545590104705994, -0.7998128361456481317 ) ) ;
#66037=CARTESIAN_POINT ( 'NONE',  ( -6.497544600628390121, 6.760421010857692536, 0.1165534177344582784 ) ) ;
#66038=CARTESIAN_POINT ( 'NONE',  ( 7.062871678076271920, 7.204714810702593120, -0.7998128361456341429 ) ) ;
#66050=CARTESIAN_POINT ( 'NONE',  ( 4.784634885068531851, 8.146353749921887655, 0.8039021629790907841 ) ) ;
#66060=CARTESIAN_POINT ( 'NONE',  ( 5.279289720117871454, 6.257118729668095902, 1.159094902893437196 ) ) ;
#66065=CARTESIAN_POINT ( 'NONE',  ( -6.090138087829436664, 7.032093901976294248, 0.9931326435281346843 ) ) ;
#66072=CARTESIAN_POINT ( 'NONE',  ( -5.447343857640614573, 9.577261277214532242, -0.7998128361456362523 ) ) ;
#66074=CARTESIAN_POINT ( 'NONE',  ( 7.049313524462606395, 7.188896964819984525, 0.000000000000000000 ) ) ;
#66078=CARTESIAN_POINT ( 'NONE',  ( -4.841670253855968831, 4.821239182352949904, 0.000000000000000000 ) ) ;
#66086=CARTESIAN_POINT ( 'NONE',  ( -6.204128743306504212, 7.035606015609114472, -1.046755002246579469 ) ) ;
#66104=CARTESIAN_POINT ( 'NONE',  ( 6.211043768836173484, 8.339580045099285854, 1.443375672974065660 ) ) ;
#66116=CARTESIAN_POINT ( 'NONE',  ( -3.526529353330350336, 7.128384988945109413, -0.7216878364870458196 ) ) ;
#66118=CARTESIAN_POINT ( 'NONE',  ( 5.417364897112183719, 8.477953592343014932, 1.199719254218451159 ) ) ;
#66121=CARTESIAN_POINT ( 'NONE',  ( -5.908321080505254841, 10.11506803722328129, 0.7998128361456291469 ) ) ;
#66123=CARTESIAN_POINT ( 'NONE',  ( -4.462568837553487100, 5.235360394347691404, -1.199719254218453823 ) ) ;
#66125=CARTESIAN_POINT ( 'NONE',  ( 1.854512760316388897, 9.001999999999998892, 2.484105960264901825 ) ) ;
#66161=CARTESIAN_POINT ( 'NONE',  ( 4.773879485787624333, 4.742149952939897162, -0.7216878364870357165 ) ) ;
#66167=CARTESIAN_POINT ( 'NONE',  ( 3.528865121306874464, 7.339036084825155015, -0.7998128361456362523 ) ) ;
#66173=CARTESIAN_POINT ( 'NONE',  ( -5.438229012412890917, 8.398332043573416783, -1.082531754730549967 ) ) ;
#66180=CARTESIAN_POINT ( 'NONE',  ( -5.074494633264801990, 9.142270515442742607, 0.7998128361456291469 ) ) ;
#66187=DIRECTION ( 'NONE',  ( 0.000000000000000000, -1.496258514059622730E-16, 1.000000000000000000 ) ) ;
#66190=CARTESIAN_POINT ( 'NONE',  ( -4.932134020321308654, 8.976183133675331050, 0.7998128361456291469 ) ) ;
#66192=CARTESIAN_POINT ( 'NONE',  ( 6.592372495380235620, 6.775069446727209233, 0.2122460957004346782 ) ) ;
#66198=CARTESIAN_POINT ( 'NONE',  ( 7.693325821111733021, 7.940244644243982464, -0.7998128361456341429 ) ) ;
#66204=CARTESIAN_POINT ( 'NONE',  ( -4.305596300791617814, 7.180890229968955651, 1.199719254218452935 ) ) ;
#66209=CARTESIAN_POINT ( 'NONE',  ( -6.180537922983287302, 8.303989891604203422, -1.599625672291271394 ) ) ;
#66213=CARTESIAN_POINT ( 'NONE',  ( 6.577113915960825175, 8.766661883411348555, -1.443375672974078761 ) ) ;
#66215=CARTESIAN_POINT ( 'NONE',  ( -7.580417283372126391, 8.016444050121833698, 0.7216878364870317197 ) ) ;
#66222=CARTESIAN_POINT ( 'NONE',  ( 6.879836604291781121, 6.991173891287354003, -0.7998128361456341429 ) ) ;
#66236=CARTESIAN_POINT ( 'NONE',  ( 6.435676556713933572, 6.878741676577107889, -0.7109887800627444632 ) ) ;
#66265=CARTESIAN_POINT ( 'NONE',  ( -6.074251926901598431, 7.043194046877760961, -1.007762736454496988 ) ) ;
#66285=CARTESIAN_POINT ( 'NONE',  ( -6.154475385960665790, 6.144919136567696505, 0.000000000000000000 ) ) ;
#66300=CARTESIAN_POINT ( 'NONE',  ( 4.518610335104485287, 8.493738834255713854, 0.000000000000000000 ) ) ;
#66303=CARTESIAN_POINT ( 'NONE',  ( 5.844973620822830895, 8.872867420051733234, 1.082531754730549967 ) ) ;
#66307=VECTOR ( 'NONE', #49329, 1000.000000000000000 ) ;
#66311=CARTESIAN_POINT ( 'NONE',  ( 3.906157654512973920, 7.571284673658210451, -0.7216878364870253915 ) ) ;
#66319=CARTESIAN_POINT ( 'NONE',  ( -5.957882158562513908, 5.915560371269843465, -0.7998128361456362523 ) ) ;
#66320=CARTESIAN_POINT ( 'NONE',  ( 4.686278372178935392, 5.496354851410763409, 1.199719254218452047 ) ) ;
#66325=VERTEX_POINT ( 'NONE', #44882 ) ;
#66328=CARTESIAN_POINT ( 'NONE',  ( -5.340986169140711226, 5.195848383611072485, 0.000000000000000000 ) ) ;
#66329=CARTESIAN_POINT ( 'NONE',  ( 7.126746022638799971, 8.343567110280638133, 1.199719254218452047 ) ) ;
#66330=CARTESIAN_POINT ( 'NONE',  ( -6.343417644159658586, 6.506394916542938667, -2.500000000000000444 ) ) ;
#66335=CARTESIAN_POINT ( 'NONE',  ( 5.713835393516482952, 5.630839145382857680, 0.7998128361456352531 ) ) ;
#66342=CARTESIAN_POINT ( 'NONE',  ( -6.253183873137761140, 7.001293123865100831, 0.9949814792902436089 ) ) ;
#66353=CARTESIAN_POINT ( 'NONE',  ( -5.935437387732586778, 10.14670372898850381, -0.7998128361456362523 ) ) ;
#66362=CARTESIAN_POINT ( 'NONE',  ( -4.524619481383255426, 4.928362264877893750, 0.8618174646245332360 ) ) ;
#66382=CARTESIAN_POINT ( 'NONE',  ( 5.411639590510088027, 6.342609606130419131, -1.199719254218452047 ) ) ;
#66392=ORIENTED_EDGE ( 'NONE', *, *, #55251, .F. ) ;
#66403=CARTESIAN_POINT ( 'NONE',  ( 6.039231080244466199, 6.010467446565510130, 0.7998128361456352531 ) ) ;
#66404=CARTESIAN_POINT ( 'NONE',  ( -4.855228407469635243, 4.837057028235559386, 0.7216878364870257245 ) ) ;
#66417=FACE_OUTER_BOUND ( 'NONE', #141091, .T. ) ;
#66429=CARTESIAN_POINT ( 'NONE',  ( -5.281783360975562225, 8.319775133516907673, 1.199719254218452935 ) ) ;
#66430=CARTESIAN_POINT ( 'NONE',  ( 6.577113915960825175, 8.766661883411348555, -1.443375672974078761 ) ) ;
#66436=CARTESIAN_POINT ( 'NONE',  ( -5.824109505522200081, 8.952488968821326054, -1.199719254218452047 ) ) ;
#66437=CARTESIAN_POINT ( 'NONE',  ( -2.823841133396259639, 6.516508098929413961, -0.7998128361456481317 ) ) ;
#66445=CARTESIAN_POINT ( 'NONE',  ( -5.586841817283045408, 8.675676665875643678, 1.199719254218454489 ) ) ;
#66452=CARTESIAN_POINT ( 'NONE',  ( 6.076298462418691315, 7.128931413452940014, -1.143247356662546732 ) ) ;
#66457=CARTESIAN_POINT ( 'NONE',  ( -4.111865726694519552, 8.019203457777400956, 0.000000000000000000 ) ) ;
#66460=CARTESIAN_POINT ( 'NONE',  ( -6.943184063974175757, 9.193743722760251202, -1.443375672974066548 ) ) ;
#66462=CARTESIAN_POINT ( 'NONE',  ( -5.546694241322218666, 8.524874810634301525, 1.082531754730550855 ) ) ;
#66463=CARTESIAN_POINT ( 'NONE',  ( 5.826972158823246595, 10.02016096192762085, -0.7998128361456481317 ) ) ;
#66464=CARTESIAN_POINT ( 'NONE',  ( -3.485854892044998543, 6.120562236477518070, -1.082531754730546636 ) ) ;
#66479=CARTESIAN_POINT ( 'NONE',  ( -0.3857294007042892936, 3.105957228677906024, 1.963430320088064063 ) ) ;
#66484=CARTESIAN_POINT ( 'NONE',  ( 6.569431593124095414, 6.790062804044275424, 0.3413723397009699734 ) ) ;
#66490=CARTESIAN_POINT ( 'NONE',  ( 5.607153537668954968, 7.478697956109829903, -1.381574923128374044 ) ) ;
#66504=CARTESIAN_POINT ( 'NONE',  ( 5.599868899865946936, 7.382462344760764239, -1.240035354157904779 ) ) ;
#66516=CARTESIAN_POINT ( 'NONE',  ( 6.013923656113508542, 9.173938811177871244, -1.199719254218452047 ) ) ;
#66519=CARTESIAN_POINT ( 'NONE',  ( -5.276058054373441664, 6.184431147304315424, -1.199719254218453823 ) ) ;
#66529=EDGE_CURVE ( 'NONE', #83476, #122390, #66786, .T. ) ;
#66534=CARTESIAN_POINT ( 'NONE',  ( 5.435893244436359240, 5.306573304789342416, -0.7998128361456481317 ) ) ;
#66535=VECTOR ( 'NONE', #500, 1000.000000000000000 ) ;
#66537=CARTESIAN_POINT ( 'NONE',  ( 5.806634928402749196, 9.996434193103704402, -0.7998128361456481317 ) ) ;
#66541=CARTESIAN_POINT ( 'NONE',  ( -6.739811759324828344, 8.956476034002674780, -1.443375672974066548 ) ) ;
#66546=CARTESIAN_POINT ( 'NONE',  ( 7.364013710877980401, 8.620379413226322285, -1.199719254218452047 ) ) ;
#66561=CARTESIAN_POINT ( 'NONE',  ( -6.807602527837528505, 7.114826835331461652, 0.7216878364870317197 ) ) ;
#66562=CARTESIAN_POINT ( 'NONE',  ( 5.560252395380215873, 6.619954228432645138, 1.082531754730549078 ) ) ;
#66572=CARTESIAN_POINT ( 'NONE',  ( -5.171509248969888617, 4.998125310078441075, 0.7998128361456281477 ) ) ;
#66573=CARTESIAN_POINT ( 'NONE',  ( -6.780486220610186798, 8.043560357867583832, -1.082531754730549967 ) ) ;
#66574=CARTESIAN_POINT ( 'NONE',  ( 7.472478939787284169, 8.746922180287201698, 1.199719254218452935 ) ) ;
#66577=CARTESIAN_POINT ( 'NONE',  ( 6.170369307550831017, 6.371388078330353366, 0.7216878364870328300 ) ) ;
#66592=CARTESIAN_POINT ( 'NONE',  ( 2.943528747942701695, 6.448217615992859919, 0.000000000000000000 ) ) ;
#66595=CARTESIAN_POINT ( 'NONE',  ( -4.950662367645459305, 5.804802846121667415, -1.199719254218453823 ) ) ;
#66605=CARTESIAN_POINT ( 'NONE',  ( 5.090160327287878594, 4.903218234782778850, -0.7998128361456481317 ) ) ;
#66644=CARTESIAN_POINT ( 'NONE',  ( 5.722950238744211937, 5.849399164722627553, 0.7216878364870328300 ) ) ;
#66645=ORIENTED_EDGE ( 'NONE', *, *, #146400, .F. ) ;
#66650=CARTESIAN_POINT ( 'NONE',  ( 6.672020991256494504, 6.956648375986938859, 0.000000000000000000 ) ) ;
#66663=CARTESIAN_POINT ( 'NONE',  ( -7.293360289508603600, 7.473618190706972086, 0.000000000000000000 ) ) ;
#66673=CARTESIAN_POINT ( 'NONE',  ( 7.095713291905693332, 9.371694488680407886, 1.599625672291268286 ) ) ;
#66680=CARTESIAN_POINT ( 'NONE',  ( -7.273023059088104425, 7.449891421883056530, 0.000000000000000000 ) ) ;
#66686=CARTESIAN_POINT ( 'NONE',  ( -6.292392690518214593, 7.474117906093608710, -1.082531754730549967 ) ) ;
#66689=CARTESIAN_POINT ( 'NONE',  ( -4.776215253764153346, 8.794277906025310898, -0.7998128361456362523 ) ) ;
#66710=ORIENTED_EDGE ( 'NONE', *, *, #175830, .T. ) ;
#66711=CARTESIAN_POINT ( 'NONE',  ( -6.474900878978163021, 9.711745571186627402, -1.199719254218452047 ) ) ;
#66713=CARTESIAN_POINT ( 'NONE',  ( 2.911969131885072670, 6.619324097166378706, 0.000000000000000000 ) ) ;
#66714=CARTESIAN_POINT ( 'NONE',  ( -5.010620288702242853, 8.003418215864698482, -1.199719254218453823 ) ) ;
#66730=CARTESIAN_POINT ( 'NONE',  ( -3.147653791585727667, 8.920000000000001705, -2.499999999999998668 ) ) ;
#66732=CARTESIAN_POINT ( 'NONE',  ( -5.538461698019560231, 5.946930065481515371, -0.9078598751902633435 ) ) ;
#66737=CARTESIAN_POINT ( 'NONE',  ( 5.899206235721897507, 6.055031161196562373, 0.000000000000000000 ) ) ;
#66761=CARTESIAN_POINT ( 'NONE',  ( 4.370663978927065152, 5.060324124126027279, 2.420000000000000373 ) ) ;
#66769=CARTESIAN_POINT ( 'NONE',  ( 3.736153849017632922, 6.516540702899320081, -1.199719254218453823 ) ) ;
#66782=CARTESIAN_POINT ( 'NONE',  ( 4.625518323863472503, 8.335144253906971556, 0.3473850511846506839 ) ) ;
#66784=CARTESIAN_POINT ( 'NONE',  ( 5.388439706788500594, 5.251210844200210559, 0.7998128361456352531 ) ) ;
#66786=CIRCLE ( 'NONE', #149877, 2.080000000000000071 ) ;
#66791=CARTESIAN_POINT ( 'NONE',  ( -5.315678745009726924, 8.359319748223434487, -1.199719254218453823 ) ) ;
#66796=CARTESIAN_POINT ( 'NONE',  ( -6.251718229232846369, 9.347402796530044355, -1.082531754730549967 ) ) ;
#66798=CARTESIAN_POINT ( 'NONE',  ( -5.155907263950760822, 7.611285832944477470, 1.217474411562294190 ) ) ;
#66803=CARTESIAN_POINT ( 'NONE',  ( 5.668717624289557833, 8.667235424096215723, -1.082531754730548412 ) ) ;
#66806=CARTESIAN_POINT ( 'NONE',  ( -5.309953438407606363, 6.223975762010839574, 1.199719254218452935 ) ) ;
#66817=CARTESIAN_POINT ( 'NONE',  ( 4.095444919779759552, 6.935713618788495793, 1.199719254218451159 ) ) ;
#66818=CARTESIAN_POINT ( 'NONE',  ( 4.923546060418115822, 5.773167154356443120, -1.199719254218452047 ) ) ;
#66842=CARTESIAN_POINT ( 'NONE',  ( 5.996449078994045223, 10.21788403546024782, 0.7998128361456331437 ) ) ;
#66850=CARTESIAN_POINT ( 'NONE',  ( 4.694866332082116678, 8.699370830729650450, 0.7998128361456341429 ) ) ;
#66857=CARTESIAN_POINT ( 'NONE',  ( 5.424670859243587273, 5.501406555305196733, -0.7216878364870458196 ) ) ;
#66861=CARTESIAN_POINT ( 'NONE',  ( 6.211043768836170820, 9.299949259400630552, 1.082531754730549967 ) ) ;
#66873=CARTESIAN_POINT ( 'NONE',  ( -6.970300371201519241, 7.304640985922785212, 0.7216878364870317197 ) ) ;
#66877=CARTESIAN_POINT ( 'NONE',  ( 3.147653791585699690, 8.920000000000010587, 2.500000000000000444 ) ) ;
#66901=CARTESIAN_POINT ( 'NONE',  ( 4.380693030546913391, 7.164540064729805202, 1.082531754730549078 ) ) ;
#66911=CARTESIAN_POINT ( 'NONE',  ( 7.517069824134078537, 7.734612647770044092, 0.000000000000000000 ) ) ;
#66913=CARTESIAN_POINT ( 'NONE',  ( 6.384963997392946844, 6.413822516572072807, 0.7998128361456352531 ) ) ;
#66928=CARTESIAN_POINT ( 'NONE',  ( -4.767627293860968507, 5.591261926706423857, -1.199719254218453823 ) ) ;
#66930=CARTESIAN_POINT ( 'NONE',  ( 5.356880090730863131, 7.343055753976412525, 1.443375672974064550 ) ) ;
#66941=AXIS2_PLACEMENT_3D ( 'NONE', #121800, #187767, #7947 ) ;
#66946=CARTESIAN_POINT ( 'NONE',  ( -6.238160076063538284, 9.331584951165851294, 1.082531754730549967 ) ) ;
#66948=CARTESIAN_POINT ( 'NONE',  ( -5.370438244788932280, 6.398504386076097283, 1.082531754730549078 ) ) ;
#66976=CARTESIAN_POINT ( 'NONE',  ( -5.167592825464113915, 6.057888380243431570, 1.199719254218452935 ) ) ;
#66988=CARTESIAN_POINT ( 'NONE',  ( -5.679622069920094773, 7.427521650927588759, -1.335666627332438683 ) ) ;
#67006=CARTESIAN_POINT ( 'NONE',  ( 7.225569521440261767, 7.394528961293920233, -0.7998128361456341429 ) ) ;
#67029=CARTESIAN_POINT ( 'NONE',  ( 6.424584688029230328, 8.588711117491191871, 1.599625672291268286 ) ) ;
#67030=CARTESIAN_POINT ( 'NONE',  ( 4.603875680292229156, 7.528882839386387360, 1.199719254218452047 ) ) ;
#67032=CARTESIAN_POINT ( 'NONE',  ( 3.555981428534177091, 7.370671776590375757, 0.7998128361456271485 ) ) ;
#67045=CARTESIAN_POINT ( 'NONE',  ( 5.694759483343039719, 7.307619849039811655, -1.219011658351103478 ) ) ;
#67046=CARTESIAN_POINT ( 'NONE',  ( -4.624739795592936353, 7.449261290616792763, -1.082531754730549967 ) ) ;
#67047=CARTESIAN_POINT ( 'NONE',  ( 4.746763178560254204, 6.631252689777363152, 1.443375672974065660 ) ) ;
#67071=CARTESIAN_POINT ( 'NONE',  ( 3.854260808034858155, 7.718664386007802136, -0.7998128361456362523 ) ) ;
#67072=CARTESIAN_POINT ( 'NONE',  ( 5.408776937209000657, 5.274937613024121674, 0.7998128361456352531 ) ) ;
#67097=DIRECTION ( 'NONE',  ( 1.000000000000000000, 0.000000000000000000, 0.000000000000000000 ) ) ;
#67101=CARTESIAN_POINT ( 'NONE',  ( 5.671053392266061977, 9.838255734277600695, 0.7998128361456331437 ) ) ;
#67105=CARTESIAN_POINT ( 'NONE',  ( -5.773214272755326171, 7.262619621122762048, 1.194638459467006530 ) ) ;
#67106=CARTESIAN_POINT ( 'NONE',  ( 7.700104897918568447, 7.948153567185284096, 0.000000000000000000 ) ) ;
#67118=CARTESIAN_POINT ( 'NONE',  ( -1.880823357903582460, 8.986349088233119176, 0.7750000000000013545 ) ) ;
#67120=CARTESIAN_POINT ( 'NONE',  ( 1.854512760316388897, 2.488359591189891251, 2.484105960264901825 ) ) ;
#67142=CARTESIAN_POINT ( 'NONE',  ( -5.607179047703544583, 8.699403434699558346, 1.199719254218454489 ) ) ;
#67144=CARTESIAN_POINT ( 'NONE',  ( 7.713663051532233972, 7.963971413067895355, -0.7998128361456341429 ) ) ;
#67155=CARTESIAN_POINT ( 'NONE',  ( 0.003603623020859416434, 2.503419261533966100, -2.003492231431212467 ) ) ;
#67163=CARTESIAN_POINT ( 'NONE',  ( 7.289443866002793371, 8.533381260871966134, 1.199719254218452047 ) ) ;
#67174=CARTESIAN_POINT ( 'NONE',  ( 7.377044979611483200, 7.779176362401098999, -0.7216878364870317197 ) ) ;
#67179=EDGE_LOOP ( 'NONE', ( #32515, #117241 ) ) ;
#67188=CARTESIAN_POINT ( 'NONE',  ( -4.340018570150309785, 7.117086527600392287, -1.082531754730551743 ) ) ;
#67190=CARTESIAN_POINT ( 'NONE',  ( 5.631432701629774051, 7.663367133358481631, 1.599625672291269396 ) ) ;
#67193=CARTESIAN_POINT ( 'NONE',  ( -6.312203035614172286, 9.521931420595302953, -1.199719254218452047 ) ) ;
#67195=CARTESIAN_POINT ( 'NONE',  ( -4.573896719763875574, 6.429575154514868274, -1.599625672291271394 ) ) ;
#67204=ORIENTED_EDGE ( 'NONE', *, *, #130004, .T. ) ;
#67207=CARTESIAN_POINT ( 'NONE',  ( 3.840479349152599919, 7.346192795665340114, 0.4818892653144311033 ) ) ;
#67242=CARTESIAN_POINT ( 'NONE',  ( 5.225741863424510747, 5.061396693608882558, 0.7998128361456352531 ) ) ;
#67244=CARTESIAN_POINT ( 'NONE',  ( -5.418418667316934112, 6.350518529071726981, -1.199719254218453823 ) ) ;
#67248=CARTESIAN_POINT ( 'NONE',  ( -6.590672069574513792, 6.861741300691274859, 0.000000000000000000 ) ) ;
#67253=CARTESIAN_POINT ( 'NONE',  ( -7.747558435566414659, 8.003516027774422170, -0.7998128361456362523 ) ) ;
#67260=CARTESIAN_POINT ( 'NONE',  ( -5.281783360975562225, 8.319775133516907673, 1.199719254218452935 ) ) ;
#67262=CARTESIAN_POINT ( 'NONE',  ( 4.655672573246532941, 8.415299432525721102, 0.4976263304441782553 ) ) ;
#67267=CARTESIAN_POINT ( 'NONE',  ( 5.318541398310776103, 9.426991741329731056, -0.7998128361456481317 ) ) ;
#67275=CARTESIAN_POINT ( 'NONE',  ( -4.492547798081878874, 6.334668079219206049, 1.599625672291263179 ) ) ;
#67279=CARTESIAN_POINT ( 'NONE',  ( -5.237192476628793614, 9.332084666034067055, 0.7998128361456291469 ) ) ;
#67281=CARTESIAN_POINT ( 'NONE',  ( 6.346625304528514810, 6.577020074804287297, 0.000000000000000000 ) ) ;
#67285=CARTESIAN_POINT ( 'NONE',  ( -7.892254816486440561, 8.380254505421877553, 0.000000000000000000 ) ) ;
#67291=CARTESIAN_POINT ( 'NONE',  ( 6.852720297064418986, 6.959538199522133262, 0.7998128361456331437 ) ) ;
#67299=CARTESIAN_POINT ( 'NONE',  ( -5.100224957694119432, 6.410602811745620855, 1.321793204645645980 ) ) ;
#67304=CARTESIAN_POINT ( 'NONE',  ( 5.253852870291571442, 7.792406146126436006, -1.285611862062207011 ) ) ;
#67318=CARTESIAN_POINT ( 'NONE',  ( -4.570507181138272479, 7.385989907086349504, 1.082531754730549967 ) ) ;
#67332=CARTESIAN_POINT ( 'NONE',  ( -5.826481282663010575, 7.222486169913409526, -1.172043233395845485 ) ) ;
#67349=CARTESIAN_POINT ( 'NONE',  ( -3.955946960137363799, 7.837298230127379917, 0.7998128361456352531 ) ) ;
#67360=VERTEX_POINT ( 'NONE', #121168 ) ;
#67364=CARTESIAN_POINT ( 'NONE',  ( 6.424584688029230328, 8.588711117491191871, 1.599625672291268286 ) ) ;
#67367=CARTESIAN_POINT ( 'NONE',  ( 5.356880090730850696, 9.263794182579101033, 0.7216878364870317197 ) ) ;
#67384=CARTESIAN_POINT ( 'NONE',  ( -4.125423880308188629, 8.035021303660014880, -0.7998128361456481317 ) ) ;
#67385=CARTESIAN_POINT ( 'NONE',  ( 4.355912491740495440, 8.303924683664389406, 0.000000000000000000 ) ) ;
#67389=EDGE_CURVE ( 'NONE', #80820, #58907, #17150, .T. ) ;
#67394=CARTESIAN_POINT ( 'NONE',  ( -8.086512275908061653, 8.398962174839683215, 0.000000000000000000 ) ) ;
#67395=CARTESIAN_POINT ( 'NONE',  ( 7.614839552730775729, 8.913009562054615031, 1.199719254218452047 ) ) ;
#67397=CARTESIAN_POINT ( 'NONE',  ( -5.717509255324293882, 7.006698007003660855, -2.500000000000000444 ) ) ;
#67403=CARTESIAN_POINT ( 'NONE',  ( 5.740951700743842423, 5.662474837148078421, -0.7998128361456481317 ) ) ;
#67408=CARTESIAN_POINT ( 'NONE',  ( -6.212075186202199006, 7.030024481103895440, 1.038766164041710738 ) ) ;
#67417=CARTESIAN_POINT ( 'NONE',  ( -3.648552735408990166, 6.310376387068841630, -1.082531754730546636 ) ) ;
#67432=ORIENTED_EDGE ( 'NONE', *, *, #177718, .T. ) ;
#67443=CARTESIAN_POINT ( 'NONE',  ( -1.886825320689270225, 2.480000000000016858, 2.459652456995881753 ) ) ;
#67468=CARTESIAN_POINT ( 'NONE',  ( 5.337069745634900997, 6.255611453776062980, 1.199719254218452047 ) ) ;
#67469=CARTESIAN_POINT ( 'NONE',  ( -5.329763783947941036, 5.390681634126922361, 0.000000000000000000 ) ) ;
#67499=CARTESIAN_POINT ( 'NONE',  ( -6.469175572376043348, 7.576401584974034265, 1.199719254218452047 ) ) ;
#67511=CARTESIAN_POINT ( 'NONE',  ( -6.831329296439251131, 9.063246493969506545, -1.599625672291271394 ) ) ;
#67513=CARTESIAN_POINT ( 'NONE',  ( 5.396826230253299883, 7.665096674459883630, -1.326205021280580265 ) ) ;
#67523=CARTESIAN_POINT ( 'NONE',  ( -6.459533842268148973, 6.500820668926428958, 0.000000000000000000 ) ) ;
#67528=CARTESIAN_POINT ( 'NONE',  ( -7.593975437430151132, 8.032261896522864930, -0.7216878364870338292 ) ) ;
#67531=CARTESIAN_POINT ( 'NONE',  ( 3.879041346841291649, 7.539648981374564407, 1.040834085586084257E-14 ) ) ;
#67533=CARTESIAN_POINT ( 'NONE',  ( -3.458738584817664385, 7.049295759013638474, 0.7216878364870338292 ) ) ;
#67535=ORIENTED_EDGE ( 'NONE', *, *, #99878, .F. ) ;
#67546=CARTESIAN_POINT ( 'NONE',  ( -0.4771755680234849861, 3.000978323161636485, 1.942502113148306231 ) ) ;
#67551=CARTESIAN_POINT ( 'NONE',  ( 6.564609147483420060, 6.793222102749934876, 0.3624652974001541517 ) ) ;
#67556=CARTESIAN_POINT ( 'NONE',  ( -4.913752204202785023, 4.881785571126718182, -0.5639616748225815268 ) ) ;
#67557=CARTESIAN_POINT ( 'NONE',  ( 5.769883596960928784, 7.349226441320860559, -1.350955626351646233 ) ) ;
#67571=CARTESIAN_POINT ( 'NONE',  ( 6.396603524444617328, 6.809554808131969672, -0.5206029305389828776 ) ) ;
#67585=CARTESIAN_POINT ( 'NONE',  ( 7.364013710877980401, 8.620379413226322285, -1.199719254218452047 ) ) ;
#67588=CARTESIAN_POINT ( 'NONE',  ( -4.633854640820660009, 8.628190524257904670, -0.7998128361456362523 ) ) ;
#67600=CARTESIAN_POINT ( 'NONE',  ( 5.910428620914669473, 5.860197910680708944, 0.000000000000000000 ) ) ;
#67602=CARTESIAN_POINT ( 'NONE',  ( 5.885121196783658526, 9.023669275293071834, 1.199719254218452047 ) ) ;
#67608=CARTESIAN_POINT ( 'NONE',  ( -6.821160681006823268, 9.051383109298335228, 1.443375672974064550 ) ) ;
#67609=ORIENTED_EDGE ( 'NONE', *, *, #17759, .F. ) ;
#67613=CARTESIAN_POINT ( 'NONE',  ( 8.188198428010544205, 8.517596018959260107, 0.000000000000000000 ) ) ;
#67627=CARTESIAN_POINT ( 'NONE',  ( -5.302647476720585118, 9.200522799567075083, 0.000000000000000000 ) ) ;
#67628=CARTESIAN_POINT ( 'NONE',  ( 5.397554552016226914, 6.430140077841320689, 1.082531754730549078 ) ) ;
#67632=ORIENTED_EDGE ( 'NONE', *, *, #207750, .T. ) ;
#67636=ORIENTED_EDGE ( 'NONE', *, *, #48644, .T. ) ;
#67637=CARTESIAN_POINT ( 'NONE',  ( -3.149236820124241110, 6.896136400112061970, -0.7998128361456481317 ) ) ;
#67638=CARTESIAN_POINT ( 'NONE',  ( -6.943184063974178422, 8.233374508458908281, -1.082531754730549967 ) ) ;
#67639=CARTESIAN_POINT ( 'NONE',  ( 1.859876166164115219, 2.485118833786766679, -2.480102205501340418 ) ) ;
#67642=CARTESIAN_POINT ( 'NONE',  ( 4.489158259456265121, 7.291082831790689056, -1.082531754730548412 ) ) ;
#67653=CARTESIAN_POINT ( 'NONE',  ( -5.303700083894403505, 7.646886670761364968, 1.227282432737321294 ) ) ;
#67658=CARTESIAN_POINT ( 'NONE',  ( 5.099275172515607579, 5.121778254122544283, -0.7216878364870458196 ) ) ;
#67661=CARTESIAN_POINT ( 'NONE',  ( -4.620296487206990932, 8.612372678375294299, 0.000000000000000000 ) ) ;
#67674=CARTESIAN_POINT ( 'NONE',  ( 3.379725431556547477, 7.165039780116438273, -1.734723475976807094E-15 ) ) ;
#67686=CARTESIAN_POINT ( 'NONE',  ( 3.004449694157372175, 6.376150746295683014, 0.4906582928672916788 ) ) ;
#67696=CARTESIAN_POINT ( 'NONE',  ( -1.854512760316423536, 0.000000000000000000, 2.484105960264900936 ) ) ;
#67710=CARTESIAN_POINT ( 'NONE',  ( 6.387299765813869712, 6.624473612970537495, 0.000000000000000000 ) ) ;
#67711=ORIENTED_EDGE ( 'NONE', *, *, #42400, .T. ) ;
#67716=CARTESIAN_POINT ( 'NONE',  ( 6.346625304528514810, 6.577020074804287297, 0.000000000000000000 ) ) ;
#67739=CARTESIAN_POINT ( 'NONE',  ( 4.041739190205284160, 7.729463131965888856, 0.000000000000000000 ) ) ;
#67741=CARTESIAN_POINT ( 'NONE',  ( 3.892599500454941630, 6.595097612955829192, 1.082531754730549078 ) ) ;
#67747=CARTESIAN_POINT ( 'NONE',  ( -6.882699257592852504, 8.058845884393651460, -1.199719254218452047 ) ) ;
#67753=CARTESIAN_POINT ( 'NONE',  ( -4.475600106286965918, 8.235634200727838916, 0.7216878364870338292 ) ) ;
#67756=CARTESIAN_POINT ( 'NONE',  ( -6.622231685632140596, 6.690634819517756959, 0.000000000000000000 ) ) ;
#67778=CARTESIAN_POINT ( 'NONE',  ( -3.851925040058337579, 6.547644075826416277, -1.082531754730546636 ) ) ;
#67779=ORIENTED_EDGE ( 'NONE', *, *, #193855, .F. ) ;
#67780=CARTESIAN_POINT ( 'NONE',  ( -4.950135482320929370, 5.908151163196758482, -1.082531754730549967 ) ) ;
#67781=CARTESIAN_POINT ( 'NONE',  ( 2.925527285498711549, 6.635141943048991742, 0.7998128361456281477 ) ) ;
#67782=CARTESIAN_POINT ( 'NONE',  ( -5.330290668828105538, 6.247702530834755130, 1.199719254218452935 ) ) ;
#67783=CARTESIAN_POINT ( 'NONE',  ( -4.959250327548641479, 9.007818825440551791, -0.7998128361456362523 ) ) ;
#67839=CARTESIAN_POINT ( 'NONE',  ( 3.923105346307896202, 5.670318552149568703, -1.599625672291269396 ) ) ;
#67841=CARTESIAN_POINT ( 'NONE',  ( 6.189608320745400682, 5.317548586107500697, -2.438128985384273140 ) ) ;
#67852=CARTESIAN_POINT ( 'NONE',  ( 4.664027441776592120, 8.287593892024585074, -0.5126927951675692707 ) ) ;
#67855=CARTESIAN_POINT ( 'NONE',  ( 5.252858170651868441, 5.093032385374103299, -0.7998128361456481317 ) ) ;
#67858=EDGE_LOOP ( 'NONE', ( #47193, #124650, #40021, #45385 ) ) ;
#67859=CARTESIAN_POINT ( 'NONE',  ( -5.960744811863571968, 6.983232364376142698, 1.199719254218452935 ) ) ;
#67865=CARTESIAN_POINT ( 'NONE',  ( -6.075462232255183892, 10.10214001435745246, 0.000000000000000000 ) ) ;
#67869=CARTESIAN_POINT ( 'NONE',  ( 5.872089928050245433, 6.023395468912886130, -0.7216878364870151774 ) ) ;
#67873=CARTESIAN_POINT ( 'NONE',  ( 5.316205630334249754, 7.295602216847000498, -1.443375672974078761 ) ) ;
#67876=CARTESIAN_POINT ( 'NONE',  ( -5.418418667316934112, 6.350518529071726981, -1.199719254218453823 ) ) ;
#67889=CARTESIAN_POINT ( 'NONE',  ( 4.258142763143749399, 7.125527769379820242, 1.199719254218451159 ) ) ;
#67890=CARTESIAN_POINT ( 'NONE',  ( 4.760848217054122422, 5.583353003765119560, -1.199719254218452047 ) ) ;
#67902=ORIENTED_EDGE ( 'NONE', *, *, #200488, .T. ) ;
#67914=CARTESIAN_POINT ( 'NONE',  ( 7.506374323821472849, 8.786466794993730289, -1.199719254218452047 ) ) ;
#67920=EDGE_CURVE ( 'NONE', #156131, #111968, #21345, .T. ) ;
#67923=CARTESIAN_POINT ( 'NONE',  ( 6.852720297064418986, 6.959538199522133262, 0.7998128361456331437 ) ) ;
#67927=CARTESIAN_POINT ( 'NONE',  ( 5.560252395380215873, 6.619954228432645138, 1.082531754730549078 ) ) ;
#67930=CARTESIAN_POINT ( 'NONE',  ( 5.560252395380198998, 9.501061871336672127, 0.7216878364870317197 ) ) ;
#67942=CARTESIAN_POINT ( 'NONE',  ( 6.485343392949857844, 6.752073445700102816, -0.1478272009810890908 ) ) ;
#67943=CARTESIAN_POINT ( 'NONE',  ( -7.160114521792834807, 8.486460042580672436, 1.082531754730549078 ) ) ;
#67979=CARTESIAN_POINT ( 'NONE',  ( 6.801350335910821165, 7.963938809097990124, 1.199719254218452047 ) ) ;
#67981=CARTESIAN_POINT ( 'NONE',  ( 6.068156270568149324, 9.237210194708310951, 1.199719254218452047 ) ) ;
#67989=SURFACE_STYLE_USAGE ( .BOTH. , #120052 ) ;
#67996=CARTESIAN_POINT ( 'NONE',  ( -6.296835998904160014, 6.311006518335105397, 0.000000000000000000 ) ) ;
#67998=CARTESIAN_POINT ( 'NONE',  ( 5.872089928050205465, 6.023395468912922546, -0.7216878364870458196 ) ) ;
#68013=CARTESIAN_POINT ( 'NONE',  ( -7.783789588021474692, 8.253711738879413673, 0.7216878364870317197 ) ) ;
#68015=CARTESIAN_POINT ( 'NONE',  ( -5.722950238744243023, 7.770137593325314285, 1.443375672974058777 ) ) ;
#68040=CARTESIAN_POINT ( 'NONE',  ( -2.979759899953417612, 6.698413326579433225, 0.7998128361456352531 ) ) ;
#68041=EDGE_CURVE ( 'NONE', #123271, #101393, #96063, .T. ) ;
#68051=CARTESIAN_POINT ( 'NONE',  ( -4.671432059311929841, 8.392430178223424520, -0.5935467769075646327 ) ) ;
#68055=ORIENTED_EDGE ( 'NONE', *, *, #164497, .T. ) ;
#68071=CARTESIAN_POINT ( 'NONE',  ( 4.864343252252968597, 8.897093904262280972, 0.000000000000000000 ) ) ;
#68095=CARTESIAN_POINT ( 'NONE',  ( 5.993586425693011144, 9.150212042353954800, -1.199719254218452047 ) ) ;
#68096=CARTESIAN_POINT ( 'NONE',  ( 5.306037014901791693, 7.283738832175834510, 1.599625672291269396 ) ) ;
#68098=CARTESIAN_POINT ( 'NONE',  ( 6.052789233858158369, 6.026285292448116948, 0.000000000000000000 ) ) ;
#68102=CARTESIAN_POINT ( 'NONE',  ( -6.180810755953226376, 5.328981043924833294, -2.500000000000671019 ) ) ;
#68111=CARTESIAN_POINT ( 'NONE',  ( 4.681345713234763117, 8.384430392927429310, -0.5894114041281351968 ) ) ;
#68112=CARTESIAN_POINT ( 'NONE',  ( -5.383996397958228819, 8.335060660042973524, 1.082531754730550855 ) ) ;
#68113=CARTESIAN_POINT ( 'NONE',  ( 3.879041347285658414, 6.579279767591636130, -1.082531754730548412 ) ) ;
#68137=CARTESIAN_POINT ( 'NONE',  ( -4.055297343818976330, 5.824542549245813383, 1.443375672974065660 ) ) ;
#68142=CARTESIAN_POINT ( 'NONE',  ( 6.313256805818848960, 7.394496357324014113, 1.199719254218452047 ) ) ;
#68147=ADVANCED_FACE ( 'NONE', ( #174667 ), #120904, .T. ) ;
#68172=CARTESIAN_POINT ( 'NONE',  ( 3.719872605471109761, 6.605953636083950364, -2.420000000000002149 ) ) ;
#68174=CARTESIAN_POINT ( 'NONE',  ( 5.508355548902068577, 9.648441583686274470, 0.7998128361456331437 ) ) ;
#68178=CARTESIAN_POINT ( 'NONE',  ( -5.288707357724018898, 7.660230058424141397, 1.223219983389673748 ) ) ;
#68179=CARTESIAN_POINT ( 'NONE',  ( 7.147083253059300922, 8.367293879104554577, 1.199719254218452935 ) ) ;
#68201=EDGE_CURVE ( 'NONE', #53040, #12133, #155503, .T. ) ;
#68211=CARTESIAN_POINT ( 'NONE',  ( -5.772739544368596043, 9.956889578397179363, -0.7998128361456362523 ) ) ;
#68214=CARTESIAN_POINT ( 'NONE',  ( 6.713222337422018349, 7.861122810861019161, -1.199719254218452047 ) ) ;
#68231=CARTESIAN_POINT ( 'NONE',  ( -3.838364070418780027, 7.492192144726518954, 0.0001517565043702621237 ) ) ;
#68235=CARTESIAN_POINT ( 'NONE',  ( 5.494797395288433250, 9.632623737803665875, 0.000000000000000000 ) ) ;
#68244=CARTESIAN_POINT ( 'NONE',  ( 5.994113311017540191, 9.046863725278862844, -1.082531754730548412 ) ) ;
#68258=CARTESIAN_POINT ( 'NONE',  ( -4.936577329151611515, 7.813071746435248599, 1.082531754730549967 ) ) ;
#68261=CARTESIAN_POINT ( 'NONE',  ( 4.552505719138623341, 8.533283448962240669, 0.7998128361456341429 ) ) ;
#68266=CARTESIAN_POINT ( 'NONE',  ( -5.015590482412729756, 4.816220082428420923, 0.000000000000000000 ) ) ;
#68276=ORIENTED_EDGE ( 'NONE', *, *, #164365, .F. ) ;
#68278=CARTESIAN_POINT ( 'NONE',  ( 3.740030321153864801, 7.357464482200652078, -0.2303333660634114821 ) ) ;
#68281=CARTESIAN_POINT ( 'NONE',  ( 3.809144859872759525, 7.350721511173911260, -0.4830196155153026472 ) ) ;
#68308=CARTESIAN_POINT ( 'NONE',  ( 3.933273961740296087, 6.642551151122080277, 1.082531754730549078 ) ) ;
#68313=CARTESIAN_POINT ( 'NONE',  ( 3.715816618597135523, 6.492813934075403637, -1.199719254218453823 ) ) ;
#68316=CARTESIAN_POINT ( 'NONE',  ( -3.935609729716867289, 7.813571461303467913, 0.7998128361456352531 ) ) ;
#68320=CARTESIAN_POINT ( 'NONE',  ( -4.624739795592931912, 8.409630504918133909, -0.7216878364870338292 ) ) ;
#68326=CARTESIAN_POINT ( 'NONE',  ( -7.259464905474441565, 7.434073576000447048, -0.7998128361456362523 ) ) ;
#68330=VERTEX_POINT ( 'NONE', #34917 ) ;
#68333=CARTESIAN_POINT ( 'NONE',  ( 7.065207446497155708, 9.336104335703744539, 0.000000000000000000 ) ) ;
#68334=CARTESIAN_POINT ( 'NONE',  ( -4.471156797456668386, 8.438376373666578445, -0.7998128361456362523 ) ) ;
#68336=CARTESIAN_POINT ( 'NONE',  ( 4.817101577040221905, 8.228953320636518853, 0.8951067572735508238 ) ) ;
#68341=CARTESIAN_POINT ( 'NONE',  ( 5.643937085038755797, 9.806620042512378177, -0.7998128361456481317 ) ) ;
#68348=CARTESIAN_POINT ( 'NONE',  ( -3.980200614063634568, 6.801261928786307642, 1.199719254218452935 ) ) ;
#68352=CARTESIAN_POINT ( 'NONE',  ( -7.110325215724114578, 7.260077271291732082, 0.000000000000000000 ) ) ;
#68358=CARTESIAN_POINT ( 'NONE',  ( -8.054952659850432184, 8.570068656013202002, 0.000000000000000000 ) ) ;
#68364=CARTESIAN_POINT ( 'NONE',  ( 7.018280793729500644, 8.217024343219755167, -1.199719254218452047 ) ) ;
#68379=EDGE_CURVE ( 'NONE', #38381, #26620, #149763, .T. ) ;
#68380=CARTESIAN_POINT ( 'NONE',  ( 6.328358748234019338, 6.951510624437585939, -0.8854765018257749754 ) ) ;
#68388=CARTESIAN_POINT ( 'NONE',  ( -2.974588534184118949, 6.690032103375380679, 0.07232793336444105770 ) ) ;
#68394=ORIENTED_EDGE ( 'NONE', *, *, #205051, .F. ) ;
#68409=CARTESIAN_POINT ( 'NONE',  ( -6.602617837901656017, 6.766230214585198688, 0.2136612715164920018 ) ) ;
#68428=CARTESIAN_POINT ( 'NONE',  ( -6.140917232347002042, 6.129101290685087911, -0.7998128361456362523 ) ) ;
#68438=EDGE_LOOP ( 'NONE', ( #176637, #191786, #32731, #211080 ) ) ;
#68441=ORIENTED_EDGE ( 'NONE', *, *, #169486, .T. ) ;
#68444=CARTESIAN_POINT ( 'NONE',  ( 5.830888582329017744, 8.960397891762626799, -1.199719254218452047 ) ) ;
#68445=CARTESIAN_POINT ( 'NONE',  ( 4.085803189671889157, 5.860132702740892263, -1.599625672291273171 ) ) ;
#68447=CARTESIAN_POINT ( 'NONE',  ( 5.655159470231527763, 9.611786791996525636, -0.7216878364870458196 ) ) ;
#68462=CARTESIAN_POINT ( 'NONE',  ( -4.827585214917754719, 7.789877296449459365, -1.199719254218453823 ) ) ;
#68463=CARTESIAN_POINT ( 'NONE',  ( 4.206772801990143584, 8.129928378955675328, 0.7998128361456271485 ) ) ;
#68466=EDGE_CURVE ( 'NONE', #53040, #118869, #186702, .T. ) ;
#68472=CARTESIAN_POINT ( 'NONE',  ( -6.912678218121246942, 9.158153569265168770, 1.599625672291269396 ) ) ;
#68473=CARTESIAN_POINT ( 'NONE',  ( 3.061108821635398769, 6.793320401875094561, -0.7998128361456362523 ) ) ;
#68480=CARTESIAN_POINT ( 'NONE',  ( 5.468734858265785093, 7.473552982767158070, 1.599625672291269396 ) ) ;
#68486=CARTESIAN_POINT ( 'NONE',  ( -5.181409149560055383, 7.856748536063159705, 1.265847179423916335 ) ) ;
#68496=CARTESIAN_POINT ( 'NONE',  ( -4.977251789548269301, 4.979417640660637190, 0.7216878364870257245 ) ) ;
#68499=CARTESIAN_POINT ( 'NONE',  ( -4.053528829375205866, 3.783736749027349244, 2.445701138906847039 ) ) ;
#68504=CARTESIAN_POINT ( 'NONE',  ( 2.929970594329034395, 6.432399770110250437, -0.7216878364870338292 ) ) ;
#68515=CARTESIAN_POINT ( 'NONE',  ( -6.633258869711600170, 6.703499867610458018, -0.5492115505440260392 ) ) ;
#68523=CARTESIAN_POINT ( 'NONE',  ( 3.739016502318667445, 7.584212696005614873, 0.7998128361456271485 ) ) ;
#68545=CARTESIAN_POINT ( 'NONE',  ( 5.564695703766185275, 5.456842840674144490, 0.000000000000000000 ) ) ;
#68548=CARTESIAN_POINT ( 'NONE',  ( -3.987506576194992824, 7.666191748953863794, 0.7216878364870338292 ) ) ;
#68571=CARTESIAN_POINT ( 'NONE',  ( -5.596483547390937119, 9.751257581923240991, 0.000000000000000000 ) ) ;
#68585=CARTESIAN_POINT ( 'NONE',  ( -6.587282531393266360, 8.778525268082516320, 1.599625672291269396 ) ) ;
#68600=CARTESIAN_POINT ( 'NONE',  ( -6.771371375382467583, 6.864631124226471037, -0.7998128361456362523 ) ) ;
#68603=CARTESIAN_POINT ( 'NONE',  ( -5.465345320084574965, 9.390336950158399532, 0.000000000000000000 ) ) ;
#68607=CARTESIAN_POINT ( 'NONE',  ( 4.380693030546916944, 6.204170850428461392, 1.443375672974058777 ) ) ;
#68608=CARTESIAN_POINT ( 'NONE',  ( -7.608060475923978494, 8.905100639113307182, 1.199719254218452047 ) ) ;
#68621=CARTESIAN_POINT ( 'NONE',  ( -0.1942909893604273797, 2.636497617442806529, 1.993158123458445230 ) ) ;
#68626=CARTESIAN_POINT ( 'NONE',  ( 6.459053645710411296, 6.863086831863287607, 0.6637952124323226455 ) ) ;
#68646=CARTESIAN_POINT ( 'NONE',  ( 5.880365472892705725, 7.167286867907723291, -1.140585135024022811 ) ) ;
#68664=CARTESIAN_POINT ( 'NONE',  ( -6.577640801285370209, 7.702944352034914566, -1.199719254218452047 ) ) ;
#68677=CARTESIAN_POINT ( 'NONE',  ( 6.387826650694035990, 7.481494509678370264, -1.199719254218452047 ) ) ;
#68686=CARTESIAN_POINT ( 'NONE',  ( -5.411112705185557203, 9.327065566109540740, 0.7216878364870267237 ) ) ;
#68687=ORIENTED_EDGE ( 'NONE', *, *, #82785, .T. ) ;
#68691=CARTESIAN_POINT ( 'NONE',  ( 6.230854113932139171, 9.427024345299638952, 1.199719254218452047 ) ) ;
#68696=VECTOR ( 'NONE', #12839, 1000.000000000000000 ) ;
#68698=DIRECTION ( 'NONE',  ( -0.000000000000000000, -1.000000000000000000, -0.000000000000000000 ) ) ;
#68702=EDGE_CURVE ( 'NONE', #41289, #129277, #73813, .T. ) ;
#68704=CARTESIAN_POINT ( 'NONE',  ( -5.587368702607575344, 8.572328348800551723, 1.082531754730550855 ) ) ;
#68705=CARTESIAN_POINT ( 'NONE',  ( 5.966997003790217136, 8.054858819212300958, -1.443375672974078761 ) ) ;
#68711=CARTESIAN_POINT ( 'NONE',  ( -3.179715765502671321, 5.975770656120749535, -2.499999999999998668 ) ) ;
#68715=B_SPLINE_CURVE_WITH_KNOTS ( 'NONE', 3,
 ( #120149, #170953, #6299, #153651, #85436, #152571 ),
 .UNSPECIFIED., .F., .F.,
 ( 4, 2, 4 ),
 ( 1.748223473168672935E-18, 0.0003191287515899651349, 0.0006382575031799285351 ),
 .UNSPECIFIED. ) ;
#68717=CARTESIAN_POINT ( 'NONE',  ( -4.634908411025374875, 6.500755460986618495, 1.599625672291263179 ) ) ;
#68718=CARTESIAN_POINT ( 'NONE',  ( -4.604929450496978660, 5.401447776115099408, -1.199719254218453823 ) ) ;
#68720=CARTESIAN_POINT ( 'NONE',  ( 3.865483193227626124, 7.523831135491951372, -0.7216878364870338292 ) ) ;
#68733=CARTESIAN_POINT ( 'NONE',  ( -5.941092982759174745, 7.138105816550336158, 1.109076209742832164 ) ) ;
#68737=CARTESIAN_POINT ( 'NONE',  ( -0.1216878429548678975, 3.463015919485879834, -1.996294584693599994 ) ) ;
#68738=CARTESIAN_POINT ( 'NONE',  ( 4.760321332173959696, 4.726332107057286791, 0.000000000000000000 ) ) ;
#68741=CARTESIAN_POINT ( 'NONE',  ( -6.656127069666307072, 6.730179434224282886, 0.7998128361456341429 ) ) ;
#68753=CARTESIAN_POINT ( 'NONE',  ( 8.000720045840086669, 8.506797273001177828, 0.7216878364870267237 ) ) ;
#68758=( BOUNDED_CURVE ( )  B_SPLINE_CURVE ( 2, ( #20310, #152464, #66901, #136225, #169772, #69048, #199041 ),
 .UNSPECIFIED., .F., .T. ) 
 B_SPLINE_CURVE_WITH_KNOTS ( ( 3, 2, 2, 3 ),
 ( 0.2750000000000000222, 0.2833333333333331039, 0.2916666666666662966, 0.2999999999999993783 ),
 .UNSPECIFIED. ) 
 CURVE ( )  GEOMETRIC_REPRESENTATION_ITEM ( )  RATIONAL_B_SPLINE_CURVE ( ( 1.000000000000000000, 0.8660254037844387076, 1.000000000000000000, 0.8660254037844387076, 1.000000000000000000, 0.8660254037844484776, 0.9999999999999902300 ) ) 
 REPRESENTATION_ITEM ( '' )  );
#68791=CARTESIAN_POINT ( 'NONE',  ( 6.265276383290871109, 7.442482214328385304, -1.082531754730548412 ) ) ;
#68796=CARTESIAN_POINT ( 'NONE',  ( 6.658462837642799670, 6.940830530104329377, 0.7216878364870328300 ) ) ;
#68810=CARTESIAN_POINT ( 'NONE',  ( -7.957709816578236506, 8.248692638954882028, 0.7998128361456341429 ) ) ;
#68820=CARTESIAN_POINT ( 'NONE',  ( 3.540087506499646874, 7.144202834309300698, -0.7216878364870338292 ) ) ;
#68826=CARTESIAN_POINT ( 'NONE',  ( -7.761116589180078407, 8.019333873657032541, 0.000000000000000000 ) ) ;
#68831=CARTESIAN_POINT ( 'NONE',  ( -6.048345925472225382, 8.149765894507963182, 1.443375672974058777 ) ) ;
#68836=CARTESIAN_POINT ( 'NONE',  ( -5.264308783856126439, 9.363720357799287797, -0.7998128361456362523 ) ) ;
#68844=CARTESIAN_POINT ( 'NONE',  ( -3.960390268523300339, 7.634556056670224855, 1.214306433183764966E-14 ) ) ;
#68858=CARTESIAN_POINT ( 'NONE',  ( -5.628043163004235794, 5.738674243025936761, 0.7216878364870257245 ) ) ;
#68860=CARTESIAN_POINT ( 'NONE',  ( 5.845500506147374153, 6.848780674373954547, 1.199719254218453823 ) ) ;
#68861=CARTESIAN_POINT ( 'NONE',  ( -4.468294144155606773, 7.370704380560280100, 1.199719254218452935 ) ) ;
#68862=CARTESIAN_POINT ( 'NONE',  ( -4.308458954092677651, 8.248562223075252220, -0.7998128361456362523 ) ) ;
#68881=STYLED_ITEM ( 'NONE', ( #10044 ), #23845 ) ;
#68886=CARTESIAN_POINT ( 'NONE',  ( -6.071018923869249129, 10.30488218781460574, 0.7998128361456291469 ) ) ;
#68906=CARTESIAN_POINT ( 'NONE',  ( -4.983766652555303267, 4.889725027032487681, 0.3176639355364049844 ) ) ;
#68914=CARTESIAN_POINT ( 'NONE',  ( 5.761288931164342486, 5.686201605971993978, -0.7998128361456481317 ) ) ;
#68928=CARTESIAN_POINT ( 'NONE',  ( 4.597294405107005488, 8.370805622008914426, 0.1071034531749150143 ) ) ;
#68931=CARTESIAN_POINT ( 'NONE',  ( 4.686278372178935392, 5.496354851410763409, 1.199719254218452047 ) ) ;
#68937=CARTESIAN_POINT ( 'NONE',  ( -6.286140498591554326, 7.362860665558790707, 1.199719254218452047 ) ) ;
#68950=CARTESIAN_POINT ( 'NONE',  ( 5.560252395380206103, 8.540692657035327429, 1.082531754730547524 ) ) ;
#68953=CARTESIAN_POINT ( 'NONE',  ( -5.478376588373717659, 8.549133898814758936, -1.199719254218452047 ) ) ;
#68966=CARTESIAN_POINT ( 'NONE',  ( 4.366607992053101128, 7.252070536440704096, -1.199719254218448494 ) ) ;
#68967=CARTESIAN_POINT ( 'NONE',  ( 5.712781623311797397, 7.758274208654143855, -1.599625672291283607 ) ) ;
#68987=FACE_OUTER_BOUND ( 'NONE', #58245, .T. ) ;
#68991=CARTESIAN_POINT ( 'NONE',  ( 4.951193585101709260, 7.980601645383334386, 1.044180363230226893 ) ) ;
#68993=CARTESIAN_POINT ( 'NONE',  ( 7.991605200612358573, 8.288237253661408843, 0.7998128361456281477 ) ) ;
#68995=ADVANCED_FACE ( 'NONE', ( #106584 ), #55644, .F. ) ;
#69002=CARTESIAN_POINT ( 'NONE',  ( 6.801350335910821165, 7.963938809097990124, 1.199719254218452047 ) ) ;
#69007=CARTESIAN_POINT ( 'NONE',  ( 6.075462232699553766, 6.260663157670496304, -0.7216878364870458196 ) ) ;
#69010=CARTESIAN_POINT ( 'NONE',  ( 3.444653546323793947, 6.176457016423196222, 1.199719254218451159 ) ) ;
#69022=CARTESIAN_POINT ( 'NONE',  ( 6.381672224870991172, 6.819330018336470012, -0.5576268912585117254 ) ) ;
#69023=CARTESIAN_POINT ( 'NONE',  ( -6.536439455564198475, 8.719208346281938304, 1.443375672974064550 ) ) ;
#69031=CARTESIAN_POINT ( 'NONE',  ( -5.570361349191150779, 5.866663122702686195, 0.5491554309224304653 ) ) ;
#69048=CARTESIAN_POINT ( 'NONE',  ( 5.844973620822802474, 5.991759777147735555, 0.7216878364870634721 ) ) ;
#69056=CARTESIAN_POINT ( 'NONE',  ( 7.340813827156391191, 7.528980651296110160, 0.7998128361456281477 ) ) ;
#69058=CARTESIAN_POINT ( 'NONE',  ( 5.365994935958575240, 9.482354201918870018, 0.7998128361456341429 ) ) ;
#69072=CARTESIAN_POINT ( 'NONE',  ( -5.798046968499580345, 6.793418213784815585, 1.199719254218452935 ) ) ;
#69074=CARTESIAN_POINT ( 'NONE',  ( 5.017926250389229459, 8.868348035513836436, 0.000000000000000000 ) ) ;
#69083=CARTESIAN_POINT ( 'NONE',  ( -5.144392941742557568, 4.966489618313220333, -0.7998128361456362523 ) ) ;
#69089=CARTESIAN_POINT ( 'NONE',  ( -7.621091744657483069, 8.063897588288083895, 0.7216878364870317197 ) ) ;
#69091=CARTESIAN_POINT ( 'NONE',  ( -6.468648687495877958, 6.719380688266201496, 0.000000000000000000 ) ) ;
#69115=CARTESIAN_POINT ( 'NONE',  ( -6.493429226302317225, 6.540365283632955773, 0.7998128361456341429 ) ) ;
#69125=CARTESIAN_POINT ( 'NONE',  ( 5.300027894412070673, 4.752150942167815195, -2.500000000000000444 ) ) ;
#69126=CARTESIAN_POINT ( 'NONE',  ( -5.345048817422858534, 7.707963373851138833, -1.327269471787644317 ) ) ;
#69150=CARTESIAN_POINT ( 'NONE',  ( 1.880823357903570248, 8.986349088233119176, -0.7749999999999996891 ) ) ;
#69165=CARTESIAN_POINT ( 'NONE',  ( 5.397027666691686321, 8.454226823519094935, 1.199719254218451159 ) ) ;
#69166=CARTESIAN_POINT ( 'NONE',  ( 4.715203562502613188, 8.723097599553565118, 0.7998128361456341429 ) ) ;
#69168=CARTESIAN_POINT ( 'NONE',  ( 4.878955176071345434, 6.785476686873604280, -1.599625672291269396 ) ) ;
#69172=CARTESIAN_POINT ( 'NONE',  ( -3.627759838191260577, 3.517451378710267029, -2.499999999999886757 ) ) ;
#69181=CARTESIAN_POINT ( 'NONE',  ( 4.701115458738250652, 8.361069499448168685, -0.6471830670988186762 ) ) ;
#69183=CARTESIAN_POINT ( 'NONE',  ( -6.739811759324840779, 7.035737605399991601, -0.7216878364870338292 ) ) ;
#69184=CARTESIAN_POINT ( 'NONE',  ( 5.750066545971570520, 5.881034856487848295, -0.7216878364870458196 ) ) ;
#69204=CARTESIAN_POINT ( 'NONE',  ( -4.299344108864953995, 7.069632989434141201, -1.082531754730551743 ) ) ;
#69209=CARTESIAN_POINT ( 'NONE',  ( 7.205232291019763480, 7.370802192470005565, -0.7998128361456341429 ) ) ;
#69211=ORIENTED_EDGE ( 'NONE', *, *, #145312, .F. ) ;
#69217=DIRECTION ( 'NONE',  ( 1.000000000000000000, -0.000000000000000000, 1.224646799147353207E-16 ) ) ;
#69238=CARTESIAN_POINT ( 'NONE',  ( 6.373214726875630731, 9.593111727067046957, 1.199719254218452047 ) ) ;
#69242=CARTESIAN_POINT ( 'NONE',  ( 6.013923656113508542, 9.173938811177871244, -1.199719254218452047 ) ) ;
#69268=CARTESIAN_POINT ( 'NONE',  ( 3.255366281057017197, 6.812028071292901998, -0.7216878364870338292 ) ) ;
#69273=CARTESIAN_POINT ( 'NONE',  ( -6.312203035614172286, 9.521931420595302953, -1.199719254218452047 ) ) ;
#69275=CARTESIAN_POINT ( 'NONE',  ( 7.309781096423290769, 8.557108029695882578, 1.199719254218452935 ) ) ;
#69279=CARTESIAN_POINT ( 'NONE',  ( -4.014622883422336308, 5.777089012116397804, -1.443375672974066548 ) ) ;
#69284=CYLINDRICAL_SURFACE ( 'NONE', #103195, 0.07999999999999954370 ) ;
#69298=CARTESIAN_POINT ( 'NONE',  ( 7.452141709366786770, 8.723195411463290583, 1.199719254218452047 ) ) ;
#69308=CARTESIAN_POINT ( 'NONE',  ( 6.617788377246179188, 8.814115421577600529, -1.443375672974078761 ) ) ;
#69321=CARTESIAN_POINT ( 'NONE',  ( -6.129694847154231852, 6.323934541200937787, -0.7216878364870338292 ) ) ;
#69324=CARTESIAN_POINT ( 'NONE',  ( 7.686546744304875389, 7.932335721302671949, 0.7998128361456291469 ) ) ;
#69327=CARTESIAN_POINT ( 'NONE',  ( -6.851666526859749418, 9.086973262793417661, -1.599625672291271394 ) ) ;
#69329=CARTESIAN_POINT ( 'NONE',  ( -3.923105346307911745, 5.670318552149568703, -1.599625672291283607 ) ) ;
#69342=CARTESIAN_POINT ( 'NONE',  ( -4.733205024502264102, 7.575804057677677505, 1.082531754730549967 ) ) ;
#69345=CARTESIAN_POINT ( 'NONE',  ( 3.846074041338778393, 7.345424771109255957, -0.6475569374996810179 ) ) ;
#69350=EDGE_CURVE ( 'NONE', #207685, #63797, #177653, .T. ) ;
#69373=CARTESIAN_POINT ( 'NONE',  ( 3.594320121398666856, 7.207474218358159490, -1.734723475976807094E-15 ) ) ;
#69380=CARTESIAN_POINT ( 'NONE',  ( -5.147255595043616516, 6.034161611419515125, 1.199719254218452935 ) ) ;
#69383=VERTEX_POINT ( 'NONE', #59690 ) ;
#69384=CARTESIAN_POINT ( 'NONE',  ( -4.923019175093582334, 8.757623114335565617, 0.7216878364870267237 ) ) ;
#69389=ORIENTED_EDGE ( 'NONE', *, *, #6353, .F. ) ;
#69390=CARTESIAN_POINT ( 'NONE',  ( -7.435720902452096936, 7.639705572474380091, 0.000000000000000000 ) ) ;
#69397=CARTESIAN_POINT ( 'NONE',  ( 4.766981195426724938, 4.885374124022287212, -0.7701443108643934998 ) ) ;
#69398=CARTESIAN_POINT ( 'NONE',  ( -1.886825320689270225, 2.480000000000016858, 2.459652456995881753 ) ) ;
#69399=CARTESIAN_POINT ( 'NONE',  ( -5.926849427829407269, 6.943687749669614995, -1.199719254218453823 ) ) ;
#69401=CARTESIAN_POINT ( 'NONE',  ( 4.641544345285703699, 8.432478572106539616, -0.4375188090333537727 ) ) ;
#69407=CARTESIAN_POINT ( 'NONE',  ( 7.126746022638799971, 8.343567110280638133, 1.199719254218452047 ) ) ;
#69418=CARTESIAN_POINT ( 'NONE',  ( -7.262327558775498737, 8.501745569106741840, 1.199719254218452047 ) ) ;
#69432=CARTESIAN_POINT ( 'NONE',  ( 6.424584688029230328, 8.588711117491191871, 1.599625672291268286 ) ) ;
#69444=CARTESIAN_POINT ( 'NONE',  ( 6.212391540903618115, 7.031971956796816414, -1.022972206104319826 ) ) ;
#69454=CARTESIAN_POINT ( 'NONE',  ( -2.974698719455045381, 6.690899969729074748, -0.05384663926280564006 ) ) ;
#69474=CARTESIAN_POINT ( 'NONE',  ( -6.600870636098118638, 6.767368133241304484, -0.2259646751960984468 ) ) ;
#69487=CARTESIAN_POINT ( 'NONE',  ( 3.556032804726692920, 7.337844839197152247, -0.2427830827038110206 ) ) ;
#69492=CARTESIAN_POINT ( 'NONE',  ( -4.899292406491858820, 6.809203455697518947, -1.599625672291271394 ) ) ;
#69508=CARTESIAN_POINT ( 'NONE',  ( -5.346851039111045978, 6.199209027673974859, 1.173132900504408438 ) ) ;
#69517=CARTESIAN_POINT ( 'NONE',  ( 5.736508392357904107, 5.865217010605237924, 0.000000000000000000 ) ) ;
#69525=CARTESIAN_POINT ( 'NONE',  ( -5.562588163356775972, 9.711712967216715953, 0.7998128361456291469 ) ) ;
#69527=CARTESIAN_POINT ( 'NONE',  ( 4.342354338126830804, 8.288106837781779035, -0.7998128361456381397 ) ) ;
#69535=CARTESIAN_POINT ( 'NONE',  ( -7.761116589180078407, 8.019333873657032541, 0.000000000000000000 ) ) ;
#69536=CARTESIAN_POINT ( 'NONE',  ( 8.018721507839716267, 8.319872945426633137, -0.7998128361456341429 ) ) ;
#69538=DIRECTION ( 'NONE',  ( 1.000000000000000000, 0.000000000000000000, 0.000000000000000000 ) ) ;
#69542=CIRCLE ( 'NONE', #266, 2.080000000000000071 ) ;
#69543=CARTESIAN_POINT ( 'NONE',  ( 6.607619761813720238, 8.802252036906432764, 1.599625672291268286 ) ) ;
#69546=CARTESIAN_POINT ( 'NONE',  ( -5.621078624820424530, 7.474595091574217420, 1.344519841555512629 ) ) ;
#69558=CARTESIAN_POINT ( 'NONE',  ( -4.299344108864961989, 6.109263775132799168, -1.443375672974066548 ) ) ;
#69561=CARTESIAN_POINT ( 'NONE',  ( -2.734094378161644023, 2.930569811600738817, 2.453211638583631782 ) ) ;
#69567=CARTESIAN_POINT ( 'NONE',  ( 4.746763178560261309, 5.670883475476017566, 1.082531754730549078 ) ) ;
#69571=CARTESIAN_POINT ( 'NONE',  ( -6.798487682609798632, 6.896266815991691779, 0.7998128361456341429 ) ) ;
#69612=CARTESIAN_POINT ( 'NONE',  ( 3.555981428534177091, 7.370671776590375757, 0.7998128361456271485 ) ) ;
#69613=CARTESIAN_POINT ( 'NONE',  ( -3.689227196694341515, 7.318199139536432973, -0.7216878364870458196 ) ) ;
#69638=CARTESIAN_POINT ( 'NONE',  ( -5.956828388357799042, 8.042995434541133193, 1.599625672291263179 ) ) ;
#69653=CARTESIAN_POINT ( 'NONE',  ( -5.074494633264801990, 9.142270515442742607, 0.7998128361456291469 ) ) ;
#69655=CARTESIAN_POINT ( 'NONE',  ( 4.913571454530422322, 8.125067815752732514, -1.031885869761673069 ) ) ;
#69660=CARTESIAN_POINT ( 'NONE',  ( 5.415556014015861841, 5.282846535965431300, -0.7998128361456481317 ) ) ;
#69665=CARTESIAN_POINT ( 'NONE',  ( -7.208094944320834863, 8.438474185576302133, -1.199719254218452047 ) ) ;
#69669=CARTESIAN_POINT ( 'NONE',  ( -6.238160076063538284, 9.331584951165851294, 1.082531754730549967 ) ) ;
#69674=CARTESIAN_POINT ( 'NONE',  ( 4.597623488365603528, 5.496887170248887067, -1.082531754730548412 ) ) ;
#69675=CARTESIAN_POINT ( 'NONE',  ( -5.112833325684928987, 5.137596099486740897, -0.7216878364870338292 ) ) ;
#69694=CARTESIAN_POINT ( 'NONE',  ( 6.578229047358968629, 6.784305542873760864, 0.2988042929856441488 ) ) ;
#69699=CARTESIAN_POINT ( 'NONE',  ( 4.370663978927085580, 5.060324124126027279, -2.420000000000000373 ) ) ;
#69715=CARTESIAN_POINT ( 'NONE',  ( 5.779562687394081522, 7.242644825714458001, 1.188994900607452054 ) ) ;
#69732=CARTESIAN_POINT ( 'NONE',  ( -5.121948170912633991, 9.197632976031879792, -0.7998128361456362523 ) ) ;
#69743=CARTESIAN_POINT ( 'NONE',  ( 6.574778147984297938, 6.635272358928617997, -0.7998128361456481317 ) ) ;
#69751=CARTESIAN_POINT ( 'NONE',  ( -6.658462837642833421, 8.861568958707010779, 1.443375672974064550 ) ) ;
#69757=CARTESIAN_POINT ( 'NONE',  ( 6.984385409695311964, 8.177479728513226576, 1.199719254218452935 ) ) ;
#69770=CARTESIAN_POINT ( 'NONE',  ( -6.536439455564198475, 8.719208346281938304, 1.443375672974064550 ) ) ;
#69771=CARTESIAN_POINT ( 'NONE',  ( 5.058600711674583472, 8.915801573680086634, 0.000000000000000000 ) ) ;
#69780=CARTESIAN_POINT ( 'NONE',  ( -3.610214042988883598, 7.433943160120816351, 0.7998128361456352531 ) ) ;
#69781=CARTESIAN_POINT ( 'NONE',  ( -2.972980823146582186, 6.690504403638126263, 0.000000000000000000 ) ) ;
#69784=CARTESIAN_POINT ( 'NONE',  ( 5.180624093753221970, 9.058162186105164437, 0.000000000000000000 ) ) ;
#69788=CARTESIAN_POINT ( 'NONE',  ( -5.586581854188635177, 5.810800913040471194, -0.4357733342581562863 ) ) ;
#69795=CARTESIAN_POINT ( 'NONE',  ( -4.964107424972056037, 7.970992240003957008, 1.031144368780096965 ) ) ;
#69802=CARTESIAN_POINT ( 'NONE',  ( -5.712781623311813384, 7.758274208654143855, -1.599625672291271394 ) ) ;
#69815=CARTESIAN_POINT ( 'NONE',  ( 3.555981428534177091, 7.370671776590375757, 0.7998128361456271485 ) ) ;
#69825=CARTESIAN_POINT ( 'NONE',  ( 3.152240666618498555, 6.104686963247638154, 0.9091918461422390241 ) ) ;
#69840=VERTEX_POINT ( 'NONE', #60894 ) ;
#69851=CARTESIAN_POINT ( 'NONE',  ( 4.394251184604957672, 8.140727125432173139, -0.7216878364870357165 ) ) ;
#69856=CARTESIAN_POINT ( 'NONE',  ( 5.031484404002878996, 7.923796667095108326, 1.082531754730548412 ) ) ;
#69858=CARTESIAN_POINT ( 'NONE',  ( -3.940069096733920251, 8.986657997193951530, 0.7749999999999996891 ) ) ;
#69871=CARTESIAN_POINT ( 'NONE',  ( -5.610041701004606196, 9.767075427805856691, -0.7998128361456362523 ) ) ;
#69882=CARTESIAN_POINT ( 'NONE',  ( 3.865483193227626124, 7.523831135491951372, -0.7216878364870338292 ) ) ;
#69887=CARTESIAN_POINT ( 'NONE',  ( -5.749539660647037032, 8.865490816466966351, 1.199719254218454489 ) ) ;
#69893=CARTESIAN_POINT ( 'NONE',  ( -6.672020991700860826, 7.917017590806697314, 1.082531754730549078 ) ) ;
#69897=CARTESIAN_POINT ( 'NONE',  ( -6.749980374757255319, 8.968339418673846097, 1.599625672291269396 ) ) ;
#69903=CARTESIAN_POINT ( 'NONE',  ( -4.604929450496978660, 5.401447776115099408, -1.199719254218453823 ) ) ;
#69917=CARTESIAN_POINT ( 'NONE',  ( -5.167065940583949413, 5.200867483535597913, 0.000000000000000000 ) ) ;
#69918=ADVANCED_FACE ( 'NONE', ( #148555 ), #132332, .F. ) ;
#69920=CARTESIAN_POINT ( 'NONE',  ( -3.648552735408985725, 7.270745601370182776, -0.7216878364870458196 ) ) ;
#69921=CARTESIAN_POINT ( 'NONE',  ( 5.737035277238070385, 6.722237907313067140, -1.199719254218452047 ) ) ;
#69922=CARTESIAN_POINT ( 'NONE',  ( -4.950662367645459305, 5.804802846121667415, -1.199719254218453823 ) ) ;
#69923=CARTESIAN_POINT ( 'NONE',  ( -5.447343857640614573, 9.577261277214532242, -0.7998128361456362523 ) ) ;
#69970=CARTESIAN_POINT ( 'NONE',  ( -4.955972296452688219, 4.884889769079732602, -0.3912739104816483349 ) ) ;
#69978=CARTESIAN_POINT ( 'NONE',  ( 6.384963997392946844, 6.413822516572072807, 0.7998128361456352531 ) ) ;
#69995=CARTESIAN_POINT ( 'NONE',  ( 3.854260808034858155, 7.718664386007802136, -0.7998128361456362523 ) ) ;
#70000=CARTESIAN_POINT ( 'NONE',  ( -5.966470118465691641, 9.118576350588734059, -1.199719254218452047 ) ) ;
#70009=CARTESIAN_POINT ( 'NONE',  ( -5.861933645127444414, 6.964938855919925231, 1.092222976013698332 ) ) ;
#70014=CARTESIAN_POINT ( 'NONE',  ( 4.719646871332936477, 8.520355426614829142, -0.7216878364870357165 ) ) ;
#70017=CARTESIAN_POINT ( 'NONE',  ( -6.459533842268148973, 6.500820668926428958, 0.000000000000000000 ) ) ;
#70029=CARTESIAN_POINT ( 'NONE',  ( 3.217027588192558074, 6.975225629525113824, -1.734723475976807094E-15 ) ) ;
#70030=CARTESIAN_POINT ( 'NONE',  ( 6.398522151006641678, 6.429640362454684954, 0.000000000000000000 ) ) ;
#70051=CARTESIAN_POINT ( 'NONE',  ( 5.763319317650291040, 7.363698819737331647, -1.304181885133362195 ) ) ;
#70053=ORIENTED_EDGE ( 'NONE', *, *, #7244, .T. ) ;
#70061=CARTESIAN_POINT ( 'NONE',  ( 3.088225128862704949, 6.824956093640315302, 0.7998128361456281477 ) ) ;
#70066=CARTESIAN_POINT ( 'NONE',  ( 6.690022453700429139, 6.769724048930809701, 0.7998128361456331437 ) ) ;
#70071=CARTESIAN_POINT ( 'NONE',  ( 4.963693636378940788, 5.923969009597785274, -1.082531754730548412 ) ) ;
#70075=CARTESIAN_POINT ( 'NONE',  ( 6.373741612200160667, 9.489763409991955001, 1.082531754730549078 ) ) ;
#70086=CARTESIAN_POINT ( 'NONE',  ( 6.400493444083267036, 6.807005473012165631, 0.5116258143813920967 ) ) ;
#70087=CARTESIAN_POINT ( 'NONE',  ( -4.442231607132987925, 5.211633625523774960, -1.199719254218453823 ) ) ;
#70116=CARTESIAN_POINT ( 'NONE',  ( 5.346851039111009563, 6.199209027673978412, 1.092492203018504471 ) ) ;
#70118=EDGE_LOOP ( 'NONE', ( #100372, #30464, #71104, #169663 ) ) ;
#70122=CARTESIAN_POINT ( 'NONE',  ( 5.885121196783658526, 9.023669275293071834, 1.199719254218452047 ) ) ;
#70124=CARTESIAN_POINT ( 'NONE',  ( 5.528692779322568640, 9.672168352510192690, 0.7998128361456341429 ) ) ;
#70139=CARTESIAN_POINT ( 'NONE',  ( -3.959863383643135393, 6.777535159962392086, 1.199719254218452935 ) ) ;
#70141=CARTESIAN_POINT ( 'NONE',  ( 6.089020385868848528, 8.197219431637373432, -1.443375672974078761 ) ) ;
#70151=CARTESIAN_POINT ( 'NONE',  ( -3.984117037569407938, 5.741498858621315371, 1.599625672291270506 ) ) ;
#70158=CARTESIAN_POINT ( 'NONE',  ( -5.157951095356222204, 4.982307464195829816, 0.000000000000000000 ) ) ;
#70160=CARTESIAN_POINT ( 'NONE',  ( -5.804299160426242388, 6.904675454319632699, -1.082531754730549967 ) ) ;
#70182=EDGE_CURVE ( 'NONE', #65240, #2249, #89167, .T. ) ;
#70183=CARTESIAN_POINT ( 'NONE',  ( -6.656127069666307072, 6.730179434224282886, 0.7998128361456341429 ) ) ;
#70193=CARTESIAN_POINT ( 'NONE',  ( -4.593509350353649268, 8.487843406384373068, -0.1931319778552646749 ) ) ;
#70208=CARTESIAN_POINT ( 'NONE',  ( 3.578681416171143770, 3.551814636441959383, 2.500000000000000444 ) ) ;
#70214=EDGE_CURVE ( 'NONE', #79190, #115058, #166639, .T. ) ;
#70216=CARTESIAN_POINT ( 'NONE',  ( 4.599659039672021166, 8.466119764437587847, 0.4625730637407374779 ) ) ;
#70218=CARTESIAN_POINT ( 'NONE',  ( 1.909527279894939422, 8.998253746724575564, -0.7749999999999996891 ) ) ;
#70227=CARTESIAN_POINT ( 'NONE',  ( 4.441177836928239309, 7.339068688795062911, 1.199719254218452047 ) ) ;
#70234=CARTESIAN_POINT ( 'NONE',  ( 7.225569521440261767, 7.394528961293920233, -0.7998128361456341429 ) ) ;
#70236=CARTESIAN_POINT ( 'NONE',  ( 5.204350862799327793, 7.165104988056252289, -1.599625672291281386 ) ) ;
#70249=CARTESIAN_POINT ( 'NONE',  ( 4.985841187518467166, 7.931359929992748192, -1.059499378661461710 ) ) ;
#70250=VECTOR ( 'NONE', #146610, 1000.000000000000000 ) ;
#70252=CARTESIAN_POINT ( 'NONE',  ( -4.950135482320918712, 7.828889591799445213, -1.082531754730549967 ) ) ;
#70253=CARTESIAN_POINT ( 'NONE',  ( 5.180624094197585627, 8.097792972322238825, -1.082531754730548412 ) ) ;
#70260=CARTESIAN_POINT ( 'NONE',  ( -2.823841133396259639, 6.516508098929413961, -0.7998128361456481317 ) ) ;
#70261=CARTESIAN_POINT ( 'NONE',  ( 3.658644423338138107, 7.354739799217567153, 0.2810151790806048044 ) ) ;
#70270=CARTESIAN_POINT ( 'NONE',  ( -5.438229012412903352, 6.477593614970734492, -1.082531754730549967 ) ) ;
#70275=CARTESIAN_POINT ( 'NONE',  ( 6.879836604291781121, 6.991173891287354003, -0.7998128361456341429 ) ) ;
#70282=DIRECTION ( 'NONE',  ( -0.7978120914393174168, 0.6029061840396252592, 6.536721945407052908E-15 ) ) ;
#70283=AXIS2_PLACEMENT_3D ( 'NONE', #38529, #186897, #91574 ) ;
#70297=ORIENTED_EDGE ( 'NONE', *, *, #47358, .F. ) ;
#70304=CARTESIAN_POINT ( 'NONE',  ( 5.820193082016415609, 10.01225203898631655, 0.000000000000000000 ) ) ;
#70333=CARTESIAN_POINT ( 'NONE',  ( 4.909461021924254709, 5.860697626067345567, 1.082531754730549078 ) ) ;
#70340=CARTESIAN_POINT ( 'NONE',  ( 5.189738938980948291, 9.276722205444929870, 0.000000000000000000 ) ) ;
#70344=CARTESIAN_POINT ( 'NONE',  ( -4.177320726786319049, 6.927272377009067839, -1.082531754730551743 ) ) ;
#70349=CARTESIAN_POINT ( 'NONE',  ( 0.4917504562594980921, 10.46609003534429405, 2.420000000000000373 ) ) ;
#70355=CARTESIAN_POINT ( 'NONE',  ( -4.955918092712652268, 4.886086657537050293, 0.4932186882876873901 ) ) ;
#70364=CARTESIAN_POINT ( 'NONE',  ( 7.828907357248368726, 8.098423103070084395, 0.7998128361456281477 ) ) ;
#70370=ORIENTED_EDGE ( 'NONE', *, *, #86369, .T. ) ;
#70373=CARTESIAN_POINT ( 'NONE',  ( 7.851580356089786328, 8.332800968292465527, 0.000000000000000000 ) ) ;
#70385=CARTESIAN_POINT ( 'NONE',  ( -4.665414256878293031, 7.496714828783040296, -1.082531754730549967 ) ) ;
#70387=CARTESIAN_POINT ( 'NONE',  ( 8.011942431032855083, 8.311964022485323511, 0.7998128361456291469 ) ) ;
#70392=CARTESIAN_POINT ( 'NONE',  ( -6.005335696210345020, 5.970922831858983315, 0.7998128361456281477 ) ) ;
#70394=CARTESIAN_POINT ( 'NONE',  ( 3.920443345323491258, 7.328669659756545940, -0.8660684152334082730 ) ) ;
#70437=CARTESIAN_POINT ( 'NONE',  ( -5.956828388357799042, 8.042995434541133193, 1.599625672291263179 ) ) ;
#70441=CARTESIAN_POINT ( 'NONE',  ( -6.296835998904160014, 6.311006518335105397, 0.000000000000000000 ) ) ;
#70442=CARTESIAN_POINT ( 'NONE',  ( -5.819596349002143398, 5.754226926782749274, -0.5594349688150419553 ) ) ;
#70446=CARTESIAN_POINT ( 'NONE',  ( -6.305950843687521790, 7.489935751457798219, 1.082531754730548412 ) ) ;
#70449=CARTESIAN_POINT ( 'NONE',  ( -4.785408264436112447, 4.881506149194969169, -0.5627276081983053624 ) ) ;
#70453=CARTESIAN_POINT ( 'NONE',  ( -5.250750630242457362, 9.347902511916677426, 0.000000000000000000 ) ) ;
#70460=CARTESIAN_POINT ( 'NONE',  ( -7.795011973214244883, 8.058878488363559356, 0.7998128361456341429 ) ) ;
#70462=CARTESIAN_POINT ( 'NONE',  ( 5.141188686642438554, 7.897460914975725998, 1.230089993873971999 ) ) ;
#70465=CARTESIAN_POINT ( 'NONE',  ( 5.765600714192121501, 7.067438534624141511, 2.440103264412639472 ) ) ;
#70467=CARTESIAN_POINT ( 'NONE',  ( 3.400062661977048428, 7.188766548940353829, -1.734723475976807094E-15 ) ) ;
#70479=CARTESIAN_POINT ( 'NONE',  ( -6.587282531393266360, 8.778525268082516320, 1.599625672291269396 ) ) ;
#70490=CARTESIAN_POINT ( 'NONE',  ( 5.505492895601038938, 8.580769590579979678, -1.199719254218452047 ) ) ;
#70491=ORIENTED_EDGE ( 'NONE', *, *, #58107, .T. ) ;
#70504=CARTESIAN_POINT ( 'NONE',  ( 5.911136963822321455, 7.250628055112136039, -1.245581879728396846 ) ) ;
#70517=ORIENTED_EDGE ( 'NONE', *, *, #202346, .F. ) ;
#70526=CARTESIAN_POINT ( 'NONE',  ( -5.384964389648357219, 7.561047897801473461, -1.247881146202101776 ) ) ;
#70531=CARTESIAN_POINT ( 'NONE',  ( -6.458928793950097891, 6.861006557743732692, 0.6885227102202008398 ) ) ;
#70550=CARTESIAN_POINT ( 'NONE',  ( -5.387385936583832802, 7.378645907471495846, -1.599625672291271394 ) ) ;
#70566=CARTESIAN_POINT ( 'NONE',  ( 4.167152111353856547, 5.955039778036558040, 1.599625672291262513 ) ) ;
#70568=CARTESIAN_POINT ( 'NONE',  ( 6.658462837642789012, 9.821938173008357253, 1.082531754730549078 ) ) ;
#70576=CARTESIAN_POINT ( 'NONE',  ( -6.438543648255500962, 6.869506004301173085, 0.7833520578412848101 ) ) ;
#70584=CARTESIAN_POINT ( 'NONE',  ( -5.088052786878465739, 9.158088361325352977, 0.000000000000000000 ) ) ;
#70587=CARTESIAN_POINT ( 'NONE',  ( 4.667750024854814050, 8.667735138964429709, -0.7998128361456381397 ) ) ;
#70598=CARTESIAN_POINT ( 'NONE',  ( -5.601453741101424022, 6.564059448486966986, -1.199719254218453823 ) ) ;
#70599=CARTESIAN_POINT ( 'NONE',  ( 5.273195401072370281, 5.116759154198018855, -0.7998128361456481317 ) ) ;
#70605=CARTESIAN_POINT ( 'NONE',  ( 5.040599249230596435, 9.102725900736217568, 0.7998128361456341429 ) ) ;
#70610=CARTESIAN_POINT ( 'NONE',  ( -4.618765760061220860, 8.456409177651165621, 0.3783674834792974950 ) ) ;
#70620=CARTESIAN_POINT ( 'NONE',  ( -4.462041952228944730, 7.259447140025469203, -1.082531754730549967 ) ) ;
#70625=CARTESIAN_POINT ( 'NONE',  ( -1.802380875475197541, 2.439898602870748778, 2.460315029152825961 ) ) ;
#70632=CARTESIAN_POINT ( 'NONE',  ( 5.234856708652235291, 5.279956712948652431, 0.7216878364870338292 ) ) ;
#70636=CARTESIAN_POINT ( 'NONE',  ( -6.459533842268148973, 6.500820668926428958, 0.000000000000000000 ) ) ;
#70642=CARTESIAN_POINT ( 'NONE',  ( -4.955918092712652268, 4.886086657537050293, 0.4932186882876873901 ) ) ;
#70649=CARTESIAN_POINT ( 'NONE',  ( 5.110497557708379546, 4.926945003606695295, -0.7998128361456481317 ) ) ;
#70673=CARTESIAN_POINT ( 'NONE',  ( -0.1033001855874529917, 3.400480225852400729, 1.999524373000333144 ) ) ;
#70676=CARTESIAN_POINT ( 'NONE',  ( -6.143253000767895600, 6.339752387083549934, 0.000000000000000000 ) ) ;
#70697=CARTESIAN_POINT ( 'NONE',  ( -6.740338644649361832, 7.892758502626242567, -1.199719254218452047 ) ) ;
#70713=CARTESIAN_POINT ( 'NONE',  ( -2.979759899953417612, 6.698413326579433225, 0.7998128361456352531 ) ) ;
#70715=CARTESIAN_POINT ( 'NONE',  ( 5.092389439195339484, 7.944299729584391123, -1.199137415704543130 ) ) ;
#70719=CARTESIAN_POINT ( 'NONE',  ( 3.067887898442204442, 6.801229324816399746, 0.7998128361456271485 ) ) ;
#70724=CARTESIAN_POINT ( 'NONE',  ( -5.074494633264801990, 9.142270515442742607, 0.7998128361456291469 ) ) ;
#70729=CARTESIAN_POINT ( 'NONE',  ( -3.637330350216213759, 7.465578851886037093, -0.7998128361456481317 ) ) ;
#70732=CARTESIAN_POINT ( 'NONE',  ( 6.061904079085887354, 6.244845311787889486, 0.000000000000000000 ) ) ;
#70733=CARTESIAN_POINT ( 'NONE',  ( 4.055297343818933697, 5.824542549245813383, 1.443375672974058777 ) ) ;
#70734=CARTESIAN_POINT ( 'NONE',  ( -5.275531169048909952, 7.248148678680751189, -1.443375672974066548 ) ) ;
#70750=CARTESIAN_POINT ( 'NONE',  ( 5.499767588998890844, 6.445425604367387429, 1.199719254218451159 ) ) ;
#70755=CARTESIAN_POINT ( 'NONE',  ( 6.148788998471866662, 7.076870205577955986, 1.084632487400632339 ) ) ;
#70763=CARTESIAN_POINT ( 'NONE',  ( 5.013482942003290255, 9.071090208970993274, -0.7998128361456481317 ) ) ;
#70774=CARTESIAN_POINT ( 'NONE',  ( 6.426609430950597890, 6.789993649951097332, 0.4362094596595481599 ) ) ;
#70789=CIRCLE ( 'NONE', #84577, 3.970406073902761790 ) ;
#70793=CARTESIAN_POINT ( 'NONE',  ( -6.479871072688648148, 6.524547437750345402, 0.000000000000000000 ) ) ;
#70806=CARTESIAN_POINT ( 'NONE',  ( 5.875479466675786355, 7.948088359245467416, -1.599625672291283607 ) ) ;
#70813=CARTESIAN_POINT ( 'NONE',  ( -7.146556367734805626, 9.431011410480991231, 1.443375672974064550 ) ) ;
#70814=VERTEX_POINT ( 'NONE', #94235 ) ;
#70818=CARTESIAN_POINT ( 'NONE',  ( 4.543390873910906791, 6.393985001019784953, 1.443375672974065660 ) ) ;
#70819=CARTESIAN_POINT ( 'NONE',  ( 5.607077132713799372, 5.680974216569005364, -0.2743783134233104826 ) ) ;
#70831=CARTESIAN_POINT ( 'NONE',  ( -7.431277594066152403, 8.802816960232885179, -1.082531754730549967 ) ) ;
#70833=CARTESIAN_POINT ( 'NONE',  ( 5.831415467653547680, 8.857049574687536619, -1.082531754730548412 ) ) ;
#70843=CARTESIAN_POINT ( 'NONE',  ( -5.984998465789844069, 5.947196063035064206, 0.7998128361456281477 ) ) ;
#70844=CARTESIAN_POINT ( 'NONE',  ( -5.307090785106547415, 5.156303768904543894, -0.7998128361456362523 ) ) ;
#70847=CARTESIAN_POINT ( 'NONE',  ( 4.529832720297257254, 8.298905583739861314, 0.000000000000000000 ) ) ;
#70859=CARTESIAN_POINT ( 'NONE',  ( -4.626128544448885549, 8.355821839108529048, -0.2988314032242797569 ) ) ;
#70863=CARTESIAN_POINT ( 'NONE',  ( 4.584065335196271462, 5.481069324884694005, 1.082531754730549078 ) ) ;
#70867=CARTESIAN_POINT ( 'NONE',  ( -4.308458954092677651, 8.248562223075252220, -0.7998128361456362523 ) ) ;
#70875=EDGE_CURVE ( 'NONE', #169159, #113379, #97426, .T. ) ;
#70881=CARTESIAN_POINT ( 'NONE',  ( 3.705121118284530279, 7.544668081299086282, -1.734723475976807094E-15 ) ) ;
#70918=CARTESIAN_POINT ( 'NONE',  ( 6.875393295905841917, 7.193916064744513506, 0.000000000000000000 ) ) ;
#70923=FACE_OUTER_BOUND ( 'NONE', #1953, .T. ) ;
#70924=CARTESIAN_POINT ( 'NONE',  ( 6.007671464186825183, 8.102312356341712984, 1.443375672974064550 ) ) ;
#70940=CARTESIAN_POINT ( 'NONE',  ( -6.312203035614172286, 9.521931420595302953, -1.199719254218452047 ) ) ;
#70952=CARTESIAN_POINT ( 'NONE',  ( 4.299344108864946890, 6.109263775132799168, -1.443375672974068769 ) ) ;
#70958=CARTESIAN_POINT ( 'NONE',  ( -4.142898457427624415, 6.991076079377632091, 1.199719254218452935 ) ) ;
#70963=CARTESIAN_POINT ( 'NONE',  ( -5.641601317062233001, 9.595968946632336127, -0.7216878364870338292 ) ) ;
#70966=CARTESIAN_POINT ( 'NONE',  ( -6.668631453075260396, 8.873432343378178544, -1.599625672291271394 ) ) ;
#70971=FACE_OUTER_BOUND ( 'NONE', #84667, .T. ) ;
#70974=DIRECTION ( 'NONE',  ( 0.000000000000000000, -1.000000000000000000, 0.000000000000000000 ) ) ;
#70979=CARTESIAN_POINT ( 'NONE',  ( 0.000000000000000000, 8.980740528189222971, 0.000000000000000000 ) ) ;
#70980=CARTESIAN_POINT ( 'NONE',  ( -4.496464221587651799, 5.274905009054215554, 1.199719254218452935 ) ) ;
#70985=CARTESIAN_POINT ( 'NONE',  ( -5.994113311017573054, 6.165756082374834079, 0.7216878364870257245 ) ) ;
#70987=CARTESIAN_POINT ( 'NONE',  ( -4.082413651046300274, 6.816547455312373494, 1.082531754730549967 ) ) ;
#70988=CARTESIAN_POINT ( 'NONE',  ( 5.357406976055401948, 6.279338222599979424, 1.199719254218452935 ) ) ;
#70989=CARTESIAN_POINT ( 'NONE',  ( -4.980641328173854632, 6.904110530993182948, 1.599625672291263179 ) ) ;
#70990=CARTESIAN_POINT ( 'NONE',  ( -6.119526231721793330, 8.232809585132461194, 1.599625672291263179 ) ) ;
#71014=CARTESIAN_POINT ( 'NONE',  ( -5.698619510900288176, 7.404755683226262875, -1.372140228778085502 ) ) ;
#71027=EDGE_CURVE ( 'NONE', #44793, #142253, #156293, .T. ) ;
#71037=CYLINDRICAL_SURFACE ( 'NONE', #11254, 1.250000000000000000 ) ;
#71047=CARTESIAN_POINT ( 'NONE',  ( 6.412080304620304538, 6.445458208337293549, -0.7998128361456481317 ) ) ;
#71063=CARTESIAN_POINT ( 'NONE',  ( 3.555981428534177091, 7.370671776590375757, 0.7998128361456271485 ) ) ;
#71070=CARTESIAN_POINT ( 'NONE',  ( -6.936931872047518155, 8.122117267924091166, 1.199719254218452047 ) ) ;
#71074=CARTESIAN_POINT ( 'NONE',  ( 3.711900195091365262, 7.552577004240394132, -0.7998128361456362523 ) ) ;
#71082=CARTESIAN_POINT ( 'NONE',  ( 4.028181036591608866, 7.713645286083285590, -0.7216878364870253915 ) ) ;
#71086=CARTESIAN_POINT ( 'NONE',  ( 4.733205024946604667, 8.536173272497439513, 0.000000000000000000 ) ) ;
#71088=CARTESIAN_POINT ( 'NONE',  ( -5.017926250833627755, 5.026871178826882947, 0.7216878364870257245 ) ) ;
#71090=CARTESIAN_POINT ( 'NONE',  ( -6.635789839245807897, 6.706452665400368218, 0.7998128361456341429 ) ) ;
#71102=CARTESIAN_POINT ( 'NONE',  ( 3.867818961648523235, 7.734482231890414283, 1.040834085586084257E-14 ) ) ;
#71103=CARTESIAN_POINT ( 'NONE',  ( 4.050854035433010480, 7.948023151305657841, 0.000000000000000000 ) ) ;
#71104=ORIENTED_EDGE ( 'NONE', *, *, #213238, .F. ) ;
#71122=CARTESIAN_POINT ( 'NONE',  ( 5.494857653270467601, 7.581134149042087600, -1.337725346733337872 ) ) ;
#71128=CARTESIAN_POINT ( 'NONE',  ( 4.746763178560250651, 7.591621904078704297, 1.082531754730549078 ) ) ;
#71130=CARTESIAN_POINT ( 'NONE',  ( 3.711900195091365262, 7.552577004240394132, -0.7998128361456362523 ) ) ;
#71134=CARTESIAN_POINT ( 'NONE',  ( 6.481679955784983349, 9.719654494127929922, -1.199719254218452047 ) ) ;
#71140=CARTESIAN_POINT ( 'NONE',  ( 4.909461021924240498, 7.781436054670031410, 1.082531754730549078 ) ) ;
#71143=CARTESIAN_POINT ( 'NONE',  ( 3.040771591214902259, 6.769593633051179005, -0.7998128361456362523 ) ) ;
#71154=CARTESIAN_POINT ( 'NONE',  ( 5.997574213172828905, 7.082153300894140635, -1.064076030282636420 ) ) ;
#71155=CARTESIAN_POINT ( 'NONE',  ( -3.634467696915153034, 6.397906858779740524, 1.199719254218452935 ) ) ;
#71164=CARTESIAN_POINT ( 'NONE',  ( 0.4608211143923647835, 2.871031678985719537, -1.947158891359296540 ) ) ;
#71181=AXIS2_PLACEMENT_3D ( 'NONE', #111032, #62222, #213761 ) ;
#71190=CARTESIAN_POINT ( 'NONE',  ( 7.367930134383754215, 7.560616343061329125, -0.7998128361456341429 ) ) ;
#71192=CARTESIAN_POINT ( 'NONE',  ( 5.905458427204159477, 9.047396044116986502, 1.199719254218452047 ) ) ;
#71206=CARTESIAN_POINT ( 'NONE',  ( -3.461074353238556167, 7.259946855412102273, 0.000000000000000000 ) ) ;
#71208=CARTESIAN_POINT ( 'NONE',  ( 6.387299765369506055, 7.584842826753462219, -1.082531754730548412 ) ) ;
#71217=CARTESIAN_POINT ( 'NONE',  ( -5.285699784481336927, 7.260012063351913625, 1.599625672291263179 ) ) ;
#71221=CARTESIAN_POINT ( 'NONE',  ( -4.828112100242303306, 4.805421336470338645, -0.7216878364870338292 ) ) ;
#71225=CARTESIAN_POINT ( 'NONE',  ( -5.093022980588950865, 5.970890227889075419, -1.199719254218453823 ) ) ;
#71227=CARTESIAN_POINT ( 'NONE',  ( -6.183927461608886844, 7.347575139032721303, 1.082531754730548412 ) ) ;
#71236=CARTESIAN_POINT ( 'NONE',  ( 4.871153761480781164, 8.051123856976298399, 0.9350251597124116243 ) ) ;
#71251=CARTESIAN_POINT ( 'NONE',  ( -6.143779885648060102, 7.196773283791382703, 1.199719254218452047 ) ) ;
#71253=CARTESIAN_POINT ( 'NONE',  ( -4.004454267989906668, 5.765225627445230927, 1.599625672291270506 ) ) ;
#71262=CARTESIAN_POINT ( 'NONE',  ( -6.026230196168996578, 7.163122537909742071, -1.192248477780058380 ) ) ;
#71282=CARTESIAN_POINT ( 'NONE',  ( 4.641416471958547341, 8.415375545968219129, 0.6158420707860997600 ) ) ;
#71285=CARTESIAN_POINT ( 'NONE',  ( 2.969872605471104876, 6.605953636086679737, -0.06813560672779371552 ) ) ;
#71293=CARTESIAN_POINT ( 'NONE',  ( 5.910428620914669473, 5.860197910680708944, 0.000000000000000000 ) ) ;
#71301=CARTESIAN_POINT ( 'NONE',  ( 6.068156270568149324, 9.237210194708310951, 1.199719254218452047 ) ) ;
#71303=CARTESIAN_POINT ( 'NONE',  ( 6.690022453700429139, 6.769724048930809701, 0.7998128361456331437 ) ) ;
#71317=CARTESIAN_POINT ( 'NONE',  ( 6.423677080210483226, 6.791898735554919853, -0.4454198846488600649 ) ) ;
#71319=CARTESIAN_POINT ( 'NONE',  ( 4.855228407469603269, 7.718164671139588151, -1.082531754730548412 ) ) ;
#71327=CARTESIAN_POINT ( 'NONE',  ( -3.471769853551161411, 6.208092708188416076, 1.199719254218452935 ) ) ;
#71332=CARTESIAN_POINT ( 'NONE',  ( 0.4437637753827078924, 3.174217730513756663, -1.950200034575564123 ) ) ;
#71337=CARTESIAN_POINT ( 'NONE',  ( -5.817857313595549584, 6.920493299683823096, 1.082531754730549078 ) ) ;
#71343=CARTESIAN_POINT ( 'NONE',  ( 6.638652492546827766, 7.774124658506663010, 1.199719254218452047 ) ) ;
#71401=ORIENTED_EDGE ( 'NONE', *, *, #33667, .F. ) ;
#71402=CARTESIAN_POINT ( 'NONE',  ( 4.746763178560254204, 6.631252689777363152, 1.443375672974065660 ) ) ;
#71404=VERTEX_POINT ( 'NONE', #201273 ) ;
#71408=CARTESIAN_POINT ( 'NONE',  ( -6.933015448541747006, 9.181880338089085214, 1.599625672291269396 ) ) ;
#71410=CARTESIAN_POINT ( 'NONE',  ( 6.875920180786008196, 8.050936961452347163, -1.199719254218452047 ) ) ;
#71415=CARTESIAN_POINT ( 'NONE',  ( -3.987506576194992824, 7.666191748953863794, 0.7216878364870338292 ) ) ;
#71435=CARTESIAN_POINT ( 'NONE',  ( 6.210516883511641772, 9.403297576475722508, 1.199719254218452047 ) ) ;
#71446=CARTESIAN_POINT ( 'NONE',  ( 6.211043768836170820, 9.299949259400630552, 1.082531754730549967 ) ) ;
#71458=CARTESIAN_POINT ( 'NONE',  ( -4.611181642423629157, 7.433443445252599702, 1.082531754730549967 ) ) ;
#71460=CARTESIAN_POINT ( 'NONE',  ( 5.677832469072920496, 9.846164657218904992, 0.000000000000000000 ) ) ;
#71465=CARTESIAN_POINT ( 'NONE',  ( -3.630551273409382329, 7.457669928944732796, 0.7998128361456352531 ) ) ;
#71470=B_SPLINE_CURVE_WITH_KNOTS ( 'NONE', 3,
 ( #197194, #150601, #15235, #46713, #112826, #178842, #31520, #96539 ),
 .UNSPECIFIED., .F., .F.,
 ( 4, 2, 2, 4 ),
 ( 0.000000000000000000, 0.001562990337899492670, 0.003125980675798985340, 0.006251961351597973282 ),
 .UNSPECIFIED. ) ;
#71508=CARTESIAN_POINT ( 'NONE',  ( 3.580761967785000888, 7.191656372475549119, -0.7216878364870338292 ) ) ;
#71511=CARTESIAN_POINT ( 'NONE',  ( -5.108390017298964914, 9.181815130149269422, 0.000000000000000000 ) ) ;
#71515=CARTESIAN_POINT ( 'NONE',  ( -5.971440312176176768, 5.931378217152456500, 0.000000000000000000 ) ) ;
#71516=CARTESIAN_POINT ( 'NONE',  ( -5.514013019825418915, 5.994650414344389056, -0.9619886414689112764 ) ) ;
#71518=ORIENTED_EDGE ( 'NONE', *, *, #106930, .T. ) ;
#71520=CARTESIAN_POINT ( 'NONE',  ( -7.241463443030476732, 7.620997903056574430, 0.000000000000000000 ) ) ;
#71521=CARTESIAN_POINT ( 'NONE',  ( 7.824464048418096951, 8.301165276008827476, -0.7216878364870317197 ) ) ;
#71527=CARTESIAN_POINT ( 'NONE',  ( -6.749980374757255319, 8.968339418673846097, 1.599625672291269396 ) ) ;
#71531=ORIENTED_EDGE ( 'NONE', *, *, #149705, .F. ) ;
#71533=CARTESIAN_POINT ( 'NONE',  ( -1.869747205843177662, 2.481503150524173140, 2.472679675789646314 ) ) ;
#71535=CARTESIAN_POINT ( 'NONE',  ( -7.632314129850253259, 7.869064337772231355, 0.7998128361456341429 ) ) ;
#71537=CARTESIAN_POINT ( 'NONE',  ( 4.628438946891473726, 8.448539137754004003, 0.3726521946380862427 ) ) ;
#71540=LINE ( 'NONE', #103003, #60292 ) ;
#71542=CARTESIAN_POINT ( 'NONE',  ( 4.329849954717849947, 6.144853928627882489, 1.599625672291262513 ) ) ;
#71546=AXIS2_PLACEMENT_3D ( 'NONE', #195968, #82195, #200200 ) ;
#71554=CARTESIAN_POINT ( 'NONE',  ( -5.752402313948099533, 9.933162809573264695, -0.7998128361456362523 ) ) ;
#71567=CARTESIAN_POINT ( 'NONE',  ( 4.004454267989866700, 5.765225627445230927, 1.599625672291262513 ) ) ;
#71575=DIRECTION ( 'NONE',  ( 2.168404344971003188E-14, 1.000000000000000000, 0.000000000000000000 ) ) ;
#71580=CARTESIAN_POINT ( 'NONE',  ( 6.440439394220377700, 6.875545743132385645, 0.7017714770480776298 ) ) ;
#71586=CARTESIAN_POINT ( 'NONE',  ( -2.974862185324181674, 6.692333939762660222, -0.03304652273056766371 ) ) ;
#71606=CARTESIAN_POINT ( 'NONE',  ( -5.939261241470221719, 7.227352081167748743, 1.243796156610659454 ) ) ;
#71609=VERTEX_POINT ( 'NONE', #56123 ) ;
#71625=CARTESIAN_POINT ( 'NONE',  ( -5.108390017298964914, 9.181815130149269422, 0.000000000000000000 ) ) ;
#71627=ORIENTED_EDGE ( 'NONE', *, *, #134258, .T. ) ;
#71640=ORIENTED_EDGE ( 'NONE', *, *, #16540, .T. ) ;
#71642=CARTESIAN_POINT ( 'NONE',  ( 3.736153849017632922, 6.516540702899320081, -1.199719254218453823 ) ) ;
#71644=CARTESIAN_POINT ( 'NONE',  ( 5.994113310573177422, 10.00723293906178846, 0.000000000000000000 ) ) ;
#71658=CARTESIAN_POINT ( 'NONE',  ( 5.017399365509065845, 8.011327138806002779, -1.199719254218450271 ) ) ;
#71668=CARTESIAN_POINT ( 'NONE',  ( -4.817943484809863008, 6.714296380401858499, 1.599625672291263179 ) ) ;
#71669=CARTESIAN_POINT ( 'NONE',  ( 4.085803189671889157, 5.860132702740892263, -1.599625672291273171 ) ) ;
#71674=CARTESIAN_POINT ( 'NONE',  ( -4.936050443827081580, 7.916420063510339666, 1.199719254218452935 ) ) ;
#71677=CARTESIAN_POINT ( 'NONE',  ( 7.198453214212898743, 7.362893269528701268, 0.7998128361456291469 ) ) ;
#71683=CARTESIAN_POINT ( 'NONE',  ( -5.586845290032572464, 7.502486493224762576, 1.347716017753825879 ) ) ;
#71693=CARTESIAN_POINT ( 'NONE',  ( -6.251718229232867685, 6.466295153626015590, -0.7216878364870338292 ) ) ;
#71694=EDGE_CURVE ( 'NONE', #206450, #23400, #121207, .T. ) ;
#71706=CARTESIAN_POINT ( 'NONE',  ( 5.040435666063417308, 4.901720900707255524, -0.1634480055122013165 ) ) ;
#71707=CARTESIAN_POINT ( 'NONE',  ( -4.274563570058511175, 8.209017608368725405, 0.000000000000000000 ) ) ;
#71711=VERTEX_POINT ( 'NONE', #122281 ) ;
#71746=CARTESIAN_POINT ( 'NONE',  ( -4.123088112331656951, 6.864000993478624579, 1.082531754730549967 ) ) ;
#71770=CARTESIAN_POINT ( 'NONE',  ( -6.967964602780620353, 7.093989889524320525, 0.000000000000000000 ) ) ;
#71772=CARTESIAN_POINT ( 'NONE',  ( 7.797347741190739256, 8.269529584243604958, 0.7216878364870267237 ) ) ;
#71777=CARTESIAN_POINT ( 'NONE',  ( -3.474632506852224356, 7.275764701294714420, -0.7998128361456481317 ) ) ;
#71785=CARTESIAN_POINT ( 'NONE',  ( -6.050681693448748177, 10.28115541899069463, 0.7998128361456291469 ) ) ;
#71791=CARTESIAN_POINT ( 'NONE',  ( 4.797606254389322089, 6.690569611577942943, 1.599625672291268286 ) ) ;
#71797=CARTESIAN_POINT ( 'NONE',  ( -7.110325215724114578, 7.260077271291732082, 0.000000000000000000 ) ) ;
#71799=CIRCLE ( 'NONE', #147908, 0.8299999999999999600 ) ;
#71802=CARTESIAN_POINT ( 'NONE',  ( -5.469788628470539926, 5.346117919495872783, -0.7998128361456362523 ) ) ;
#71806=CARTESIAN_POINT ( 'NONE',  ( 3.702785349863636277, 7.334016984900627811, -0.7216878364870338292 ) ) ;
#71807=CARTESIAN_POINT ( 'NONE',  ( -3.946832114909637479, 7.618738210787614484, 0.7216878364870338292 ) ) ;
#71811=CARTESIAN_POINT ( 'NONE',  ( -5.743814354044916470, 6.730146830254374990, -1.199719254218453823 ) ) ;
#71814=CARTESIAN_POINT ( 'NONE',  ( 5.713835393516482952, 5.630839145382857680, 0.7998128361456352531 ) ) ;
#71820=CARTESIAN_POINT ( 'NONE',  ( 6.052789233858158369, 6.026285292448116948, 0.000000000000000000 ) ) ;
#71825=CARTESIAN_POINT ( 'NONE',  ( 5.803742400754204667, 7.332416669035665358, 1.290654366993408297 ) ) ;
#71836=CARTESIAN_POINT ( 'NONE',  ( 4.864343252252968597, 8.897093904262280972, 0.000000000000000000 ) ) ;
#71839=EDGE_CURVE ( 'NONE', #111999, #10691, #104118, .T. ) ;
#71848=CARTESIAN_POINT ( 'NONE',  ( 6.162627863271451290, 6.966383021533493647, 0.9102919922300183320 ) ) ;
#71863=CARTESIAN_POINT ( 'NONE',  ( -6.469175572376043348, 7.576401584974034265, 1.199719254218452047 ) ) ;
#71868=CARTESIAN_POINT ( 'NONE',  ( -3.721290253490582955, 7.355952296265487078, 0.5966894627213925606 ) ) ;
#71877=CARTESIAN_POINT ( 'NONE',  ( 4.389807875774629942, 8.343469298370917997, 0.7998128361456271485 ) ) ;
#71887=CARTESIAN_POINT ( 'NONE',  ( 4.415115299905642665, 5.179997933758551554, -1.199719254218450271 ) ) ;
#71890=CARTESIAN_POINT ( 'NONE',  ( 4.923019175093585886, 5.876515471431535076, -1.082531754730548412 ) ) ;
#71892=DIRECTION ( 'NONE',  ( -0.000000000000000000, -1.000000000000000000, -0.000000000000000000 ) ) ;
#71905=CARTESIAN_POINT ( 'NONE',  ( -7.322812365156824654, 8.676274193172000437, 1.082531754730549078 ) ) ;
#71906=CARTESIAN_POINT ( 'NONE',  ( 6.373741612200162443, 8.529394195690610303, 1.443375672974065660 ) ) ;
#71916=CARTESIAN_POINT ( 'NONE',  ( -4.274563570058511175, 8.209017608368725405, 0.000000000000000000 ) ) ;
#71917=CARTESIAN_POINT ( 'NONE',  ( -4.472210567661380587, 6.310941310395290493, 1.599625672291270506 ) ) ;
#71919=CARTESIAN_POINT ( 'NONE',  ( 5.628043163004202931, 8.619781885929965526, -1.082531754730548412 ) ) ;
#71927=CARTESIAN_POINT ( 'NONE',  ( -5.688757509019083614, 5.629766575900002401, -2.420000000000000373 ) ) ;
#71931=CARTESIAN_POINT ( 'NONE',  ( -4.616709804987970678, 8.367809121204862421, 0.2297300046584915267 ) ) ;
#71935=CARTESIAN_POINT ( 'NONE',  ( 6.048345925472191631, 6.229027465905275562, 0.7216878364870328300 ) ) ;
#71939=CARTESIAN_POINT ( 'NONE',  ( -6.317173229324657413, 6.334733287159020954, 0.000000000000000000 ) ) ;
#71952=CARTESIAN_POINT ( 'NONE',  ( 4.716257332707354699, 6.595662536282280719, -1.599625672291269396 ) ) ;
#71966=CARTESIAN_POINT ( 'NONE',  ( -4.787437654953776267, 6.678706214094487947, -1.250000000000001110 ) ) ;
#71973=CARTESIAN_POINT ( 'NONE',  ( -0.4800000000000000933, 2.999999999999999112, -2.500000000000000444 ) ) ;
#71990=CARTESIAN_POINT ( 'NONE',  ( 5.858531774880875176, 9.849054480754103835, -0.7216878364870458196 ) ) ;
#71994=FACE_OUTER_BOUND ( 'NONE', #140926, .T. ) ;
#71995=CARTESIAN_POINT ( 'NONE',  ( 6.333067150914805765, 9.442309871825708356, 1.082531754730549967 ) ) ;
#72009=CARTESIAN_POINT ( 'NONE',  ( -5.759181390754928742, 9.941071732514568993, 0.000000000000000000 ) ) ;
#72020=CARTESIAN_POINT ( 'NONE',  ( 3.702785349863636277, 7.334016984900627811, -0.7216878364870338292 ) ) ;
#72027=CARTESIAN_POINT ( 'NONE',  ( -2.844178363816758814, 6.540234867753325076, -0.7998128361456481317 ) ) ;
#72032=CARTESIAN_POINT ( 'NONE',  ( -6.943184063974178422, 8.233374508458908281, -1.082531754730549967 ) ) ;
#72035=CARTESIAN_POINT ( 'NONE',  ( -5.901542003698421190, 10.10715911428198055, 0.000000000000000000 ) ) ;
#72040=CARTESIAN_POINT ( 'NONE',  ( -5.971440312176176768, 5.931378217152456500, 0.000000000000000000 ) ) ;
#72056=CARTESIAN_POINT ( 'NONE',  ( -4.502716413514310290, 6.346531463890372926, -1.443375672974066548 ) ) ;
#72058=CARTESIAN_POINT ( 'NONE',  ( -5.614485009390564940, 5.722856397143323726, 0.000000000000000000 ) ) ;
#72059=CARTESIAN_POINT ( 'NONE',  ( 5.896870467300973750, 5.844380064798101237, 0.7998128361456352531 ) ) ;
#72061=CARTESIAN_POINT ( 'NONE',  ( -4.945692173934974178, 8.992000979557944973, 0.000000000000000000 ) ) ;
#72062=CARTESIAN_POINT ( 'NONE',  ( -7.442499979258930587, 7.647614495415686164, -0.7998128361456362523 ) ) ;
#72082=CARTESIAN_POINT ( 'NONE',  ( 6.737475991348287785, 6.825086509519945999, -0.7998128361456481317 ) ) ;
#72104=CIRCLE ( 'NONE', #30709, 0.07999999999999983513 ) ;
#72111=CARTESIAN_POINT ( 'NONE',  ( -1.872340672757990321, 8.979957301293506333, -0.7749999999999996891 ) ) ;
#72122=CARTESIAN_POINT ( 'NONE',  ( 6.086684617892325733, 6.065829907154645539, -0.7998128361456481317 ) ) ;
#72123=CARTESIAN_POINT ( 'NONE',  ( 5.526144005543697446, 7.442112546579989996, -1.248357989223557452 ) ) ;
#72139=CARTESIAN_POINT ( 'NONE',  ( 4.366607992053101128, 7.252070536440704096, -1.199719254218448494 ) ) ;
#72144=CARTESIAN_POINT ( 'NONE',  ( -5.752402313948099533, 9.933162809573264695, -0.7998128361456362523 ) ) ;
#72149=CARTESIAN_POINT ( 'NONE',  ( 5.682802662783380754, 6.658966523782627434, 1.199719254218452935 ) ) ;
#72159=CARTESIAN_POINT ( 'NONE',  ( 7.377044979611483200, 7.779176362401098999, -0.7216878364870317197 ) ) ;
#72160=CARTESIAN_POINT ( 'NONE',  ( -4.421367491832313590, 6.251624388594711590, 1.443375672974065660 ) ) ;
#72161=CARTESIAN_POINT ( 'NONE',  ( -4.423703259808839938, 8.383013913077441259, 0.7998128361456352531 ) ) ;
#72169=ORIENTED_EDGE ( 'NONE', *, *, #165318, .F. ) ;
#72173=ORIENTED_EDGE ( 'NONE', *, *, #81808, .T. ) ;
#72174=CARTESIAN_POINT ( 'NONE',  ( 6.201928923608456046, 6.200281597156833691, 0.7998128361456352531 ) ) ;
#72175=CARTESIAN_POINT ( 'NONE',  ( 5.550083779947807550, 7.568460058062819407, -1.599625672291283607 ) ) ;
#72201=CARTESIAN_POINT ( 'NONE',  ( 5.248941747146098180, 6.152795455539095570, -1.199719254218452047 ) ) ;
#72205=CARTESIAN_POINT ( 'NONE',  ( 7.614839552730775729, 8.913009562054615031, 1.199719254218452047 ) ) ;
#72210=CARTESIAN_POINT ( 'NONE',  ( 6.224601922449876312, 6.434659462379210382, 0.000000000000000000 ) ) ;
#72212=CARTESIAN_POINT ( 'NONE',  ( -5.764151584465413869, 6.753873599078290546, -1.199719254218453823 ) ) ;
#72214=CARTESIAN_POINT ( 'NONE',  ( 5.872089928494542477, 9.864872326636710653, 0.000000000000000000 ) ) ;
#72215=ORIENTED_EDGE ( 'NONE', *, *, #88807, .F. ) ;
#72225=CARTESIAN_POINT ( 'NONE',  ( 6.080034374691865473, 7.023743017405461586, -0.9950221519831742301 ) ) ;
#72226=CARTESIAN_POINT ( 'NONE',  ( -6.102578539926875933, 10.13377570664109051, 0.7216878364870267237 ) ) ;
#72235=CARTESIAN_POINT ( 'NONE',  ( 0.2875577598566471660, 2.700852594506745863, -1.980716517367338891 ) ) ;
#72240=CIRCLE ( 'NONE', #27263, 0.08000000000000041800 ) ;
#72253=EDGE_CURVE ( 'NONE', #65494, #24495, #149096, .T. ) ;
#72261=CARTESIAN_POINT ( 'NONE',  ( 7.856023664475727308, 8.130058794835305136, -0.7998128361456341429 ) ) ;
#72263=CARTESIAN_POINT ( 'NONE',  ( 7.062871678076271920, 7.204714810702593120, -0.7998128361456341429 ) ) ;
#72277=CARTESIAN_POINT ( 'NONE',  ( -5.088052786878465739, 9.158088361325352977, 0.000000000000000000 ) ) ;
#72279=CARTESIAN_POINT ( 'NONE',  ( 6.495764994278809823, 7.711385593814346073, 1.082531754730549967 ) ) ;
#72289=CARTESIAN_POINT ( 'NONE',  ( -4.610654757099099221, 7.536791762327691657, 1.199719254218452935 ) ) ;
#72293=CARTESIAN_POINT ( 'NONE',  ( -3.851925040058337579, 6.547644075826416277, -1.082531754730546636 ) ) ;
#72297=CARTESIAN_POINT ( 'NONE',  ( -7.024532985656169792, 9.288650798055913427, 1.443375672974064550 ) ) ;
#72322=CARTESIAN_POINT ( 'NONE',  ( -5.978219388983010418, 5.939287140093762574, -0.7998128361456362523 ) ) ;
#72335=CARTESIAN_POINT ( 'NONE',  ( -5.929989559956849732, 7.234276776666978215, -1.248630897662094563 ) ) ;
#72350=CARTESIAN_POINT ( 'NONE',  ( -5.926849427829407269, 6.943687749669614995, -1.199719254218453823 ) ) ;
#72351=FACE_OUTER_BOUND ( 'NONE', #125636, .T. ) ;
#72372=CARTESIAN_POINT ( 'NONE',  ( 5.411639590510088027, 6.342609606130419131, -1.199719254218452047 ) ) ;
#72381=CARTESIAN_POINT ( 'NONE',  ( 7.062871678076271920, 7.204714810702593120, -0.7998128361456341429 ) ) ;
#72383=CARTESIAN_POINT ( 'NONE',  ( 4.518610335104485287, 8.493738834255713854, 0.000000000000000000 ) ) ;
#72396=CARTESIAN_POINT ( 'NONE',  ( 6.483128551184942800, 6.753495492978965231, -0.1682882784904728146 ) ) ;
#72398=CARTESIAN_POINT ( 'NONE',  ( 6.211043768836185031, 6.418841616496599123, 0.7216878364870328300 ) ) ;
#72405=CARTESIAN_POINT ( 'NONE',  ( -3.688700311369816909, 6.461178242310183784, -1.199719254218450271 ) ) ;
#72415=CARTESIAN_POINT ( 'NONE',  ( -3.811250578772977349, 7.460559751961507224, -0.7216878364870458196 ) ) ;
#72419=CARTESIAN_POINT ( 'NONE',  ( 4.518610335104485287, 8.493738834255713854, 0.000000000000000000 ) ) ;
#72436=CARTESIAN_POINT ( 'NONE',  ( 4.993145711582793744, 9.047363440147082159, -0.7998128361456481317 ) ) ;
#72440=ORIENTED_EDGE ( 'NONE', *, *, #146351, .F. ) ;
#72462=CARTESIAN_POINT ( 'NONE',  ( -6.501436840734760914, 6.757938919538193367, -0.04654198066046839888 ) ) ;
#72468=DIRECTION ( 'NONE',  ( 0.7592566023652995710, 0.6507913734559650498, 0.000000000000000000 ) ) ;
#72470=DIRECTION ( 'NONE',  ( 1.000000000000000000, 0.000000000000000000, 0.000000000000000000 ) ) ;
#72477=ORIENTED_EDGE ( 'NONE', *, *, #186745, .T. ) ;
#72478=CARTESIAN_POINT ( 'NONE',  ( 4.638297949650961982, 5.544340708415133712, -1.082531754730548412 ) ) ;
#72483=CARTESIAN_POINT ( 'NONE',  ( -8.106849506328558164, 8.422688943663599659, 0.000000000000000000 ) ) ;
#72485=CARTESIAN_POINT ( 'NONE',  ( 6.003228155800906407, 10.22579295840155744, 0.000000000000000000 ) ) ;
#72489=CARTESIAN_POINT ( 'NONE',  ( -4.990809943606286048, 5.955604701363006015, -1.082531754730549967 ) ) ;
#72494=EDGE_CURVE ( 'NONE', #51039, #56474, #65630, .T. ) ;
#72503=DIRECTION ( 'NONE',  ( 0.7592566023652995710, -0.6507913734559651608, 8.881784197001252323E-16 ) ) ;
#72507=EDGE_CURVE ( 'NONE', #157478, #71404, #76485, .T. ) ;
#72511=TOROIDAL_SURFACE ( 'NONE', #103778, 0.4800000000000000933, 0.08000000000000000167 ) ;
#72524=CARTESIAN_POINT ( 'NONE',  ( 4.553559489343365740, 6.405848385690952718, -1.599625672291269396 ) ) ;
#72536=CARTESIAN_POINT ( 'NONE',  ( -5.804299160426237059, 7.865044668620976509, -1.443375672974066548 ) ) ;
#72537=ORIENTED_EDGE ( 'NONE', *, *, #171627, .F. ) ;
#72539=CARTESIAN_POINT ( 'NONE',  ( 7.388267364804250725, 7.584343111885245570, -0.7998128361456341429 ) ) ;
#72544=CARTESIAN_POINT ( 'NONE',  ( -5.438755897737433287, 6.374245297895642537, -1.199719254218453823 ) ) ;
#72556=ORIENTED_EDGE ( 'NONE', *, *, #72719, .T. ) ;
#72584=CARTESIAN_POINT ( 'NONE',  ( 5.072158865288245444, 5.090142562357324429, 0.7216878364870338292 ) ) ;
#72591=CARTESIAN_POINT ( 'NONE',  ( -6.771371375382467583, 6.864631124226471037, -0.7998128361456362523 ) ) ;
#72596=CARTESIAN_POINT ( 'NONE',  ( -5.587368702163209910, 9.532697562583475559, 0.000000000000000000 ) ) ;
#72598=CARTESIAN_POINT ( 'NONE',  ( 6.170369307550806148, 10.21286493553572328, 0.7216878364870317197 ) ) ;
#72604=CARTESIAN_POINT ( 'NONE',  ( -6.237633190739009237, 9.434933268240943249, 1.199719254218452047 ) ) ;
#72610=( BOUNDED_SURFACE ( )  B_SPLINE_SURFACE ( 1, 2, ( 
 ( #208605, #107999, #192356, #74367, #140469, #141542, #91709, #206482, #93839, #42956, #44013, #110133, #176144, #45088, #27744, #159878, #11483, #111197, #80767, #163092, #197692, #198742, #132739, #13617, #144741, #46151, #62374, #146856, #79690, #49337, #64509, #33074, #130653, #28816, #30965, #97040, #99152, #194504, #14673, #78616, #66595, #212876, #196645, #48285, #131689, #114397, #50389, #15736, #179343, #180393, #115455, #32016, #164150, #113336, #98099, #165203, #210751, #81822, #94900, #116510, #160951, #47220, #147904, #213921, #65543, #16795, #181445, #82878, #148956, #12542, #128536, #526, #112264, #178278, #29888, #95973, #162026, #145802, #211808, #63446, #129598, #195585, #3729, #166266, #22110, #19999, #88222, #18928, #4789, #136982, #104481, #200870, #51461, #52514, #36250, #154292, #119717, #183576, #17856, #117583, #83941, #133806, #71939, #35182, #185698, #87147, #2668, #1601, #120798, #70867, #150031, #101259, #153219, #151104, #5867, #34130, #85014, #168403, #184633, #102329, #203009, #170527, #182499, #103404, #138049, #167342, #53583, #68741, #134863, #118648, #86083, #54649, #67661, #152159, #186775, #69802, #135910, #169465, #201928, #204063, #21050, #37330, #38401, #55715, #100200, #199817, #155353, #92524, #174833, #8019, #121868, #39466, #75178, #76237, #41631, #105562, #189979, #90367, #206225, #208354, #26412, #6938, #93583, #175892, #74110, #109880, #27483, #205144, #158563, #25346, #59986, #171595, #156434, #73019, #58921, #107745, #91445, #141288, #106657, #23189, #172684, #139116, #173769, #89304, #124012, #157506, #57851, #207297, #10161, #9102, #56786, #122954, #125080, #191036, #42703, #108810, #188914, #159628, #142346, #11222, #24261, #126139, #192101, #43767, #140203, #40553, #77304, #143416, #209410, #187839, #78367, #193184, #12286, #110939, #94649, #81568, #144487, #30707, #80507, #45895, #176944, #48039, #64263, #28560, #210494, #146604, #112016, #15483, #127216, #128290, #145556, #161772, #13365, #196396, #180146, #61057, #212622, #65294, #178016, #96790, #95720 ),
 ( #62129, #31772, #147654, #160693, #162840, #130408, #213670, #29634, #79439, #44832, #163907, #63188, #194252, #211555, #14418, #114153, #129353, #195332, #46962, #113080, #179085, #97842, #23904, #175520, #43391, #27108, #205861, #93217, #158206, #139833, #106294, #73736, #140913, #44458, #9795, #125774, #59618, #42329, #141977, #10848, #173393, #108444, #127925, #172314, #143048, #61756, #41263, #76922, #109512, #192799, #176577, #160323, #209043, #94283, #77999, #28186, #75870, #191735, #206926, #159248, #57494, #40180, #174464, #60679, #26040, #207989, #126841, #24976, #90009, #91079, #123654, #92153, #11927, #156063, #110575, #7652, #144122, #189616, #58556, #124709, #190668, #210116, #107372, #157139, #8731, #74812, #67046, #95352, #196027, #15112, #130036, #147279, #164582, #47663, #161402, #29260, #64936, #131086, #113774, #81201, #177651, #33511, #31395, #99584, #30331, #16167, #148343, #115890, #212248, #62809, #63882, #179777, #165648, #197076, #194950, #12986, #128971, #79060, #145179, #83312, #46586, #48713, #98520, #14040, #211184, #132122, #82252, #112705, #178715, #214344, #162465, #17237, #45524, #96415, #97469, #163526, #213311, #65974, #181875, #193877, #114826, #149398, #80126, #180825, #146231, #32451, #198133, #49764, #981, #111640, #151047, #15680, #166209, #52464, #102272, #180340, #199762, #101201, #168350, #165148, #99095, #3674, #117526, #115401, #183520, #114343, #65488, #213865, #118590, #84958, #31961, #184578, #116454, #2615, #98044, #35129, #167288, #18875, #131635, #68686, #17799, #197637, #164097, #147847, #474, #36197, #83885, #51407, #133753, #182447, #81767, #49282, #181394, #19943, #134808, #33018, #86029, #34075, #200814, #16739, #152103, #69751, #135856, #82824, #201877, #149976, #148900, #66541, #132682, #198690, #50334, #1546, #100144, #67608, #55659, #155302, #24205, #186719, #121816, #141230, #119660, #156378, #75120, #54597, #90308, #122901, #206168, #189926, #173714, #7961, #107685, #91390, #41571, #23133, #139066, #154237, #205092, #70813, #53526, #187784, #137995 ) ),
 .UNSPECIFIED., .F., .F., .F. ) 
 B_SPLINE_SURFACE_WITH_KNOTS ( ( 2, 2 ),
 ( 3, 2, 2, 2, 2, 2, 2, 2, 2, 2, 2, 2, 2, 2, 2, 2, 2, 2, 2, 2, 2, 2, 2, 2, 2, 2, 2, 2, 2, 2, 2, 2, 2, 2, 2, 2, 2, 2, 2, 2, 2, 2, 2, 2, 2, 2, 2, 2, 2, 2, 2, 2, 2, 2, 2, 2, 2, 2, 2, 2, 2, 2, 2, 2, 2, 2, 2, 2, 2, 2, 2, 2, 2, 2, 2, 2, 2, 2, 2, 2, 2, 2, 2, 2, 2, 2, 2, 2, 2, 2, 2, 2, 2, 2, 2, 2, 2, 2, 2, 2, 2, 2, 2, 2, 2, 2, 2, 2, 2, 2, 2, 2, 2, 2, 2, 2, 2, 2, 2, 2, 3 ),
 ( 0.000000000000000000, 1.000000000000000000 ),
 ( 0.000000000000000000, 0.008333333333333333218, 0.01666666666666666644, 0.02500000000000000139, 0.03333333333333333287, 0.04166666666666666435, 0.05000000000000000278, 0.05833333333333333426, 0.06666666666666666574, 0.07499999999999999722, 0.08333333333333332871, 0.09166666666666666019, 0.1000000000000000056, 0.1083333333333333370, 0.1166666666666666685, 0.1250000000000000000, 0.1333333333333333315, 0.1416666666666666630, 0.1499999999999999944, 0.1583333333333333259, 0.1666666666666666574, 0.1749999999999999889, 0.1833333333333333204, 0.1916666666666666796, 0.2000000000000000111, 0.2083333333333333426, 0.2166666666666666741, 0.2250000000000000056, 0.2333333333333333370, 0.2416666666666666685, 0.2500000000000000000, 0.2583333333333333592, 0.2666666666666666630, 0.2750000000000000222, 0.2833333333333333259, 0.2916666666666666852, 0.2999999999999999889, 0.3083333333333333481, 0.3166666666666666519, 0.3250000000000000111, 0.3333333333333333148, 0.3416666666666666741, 0.3499999999999999778, 0.3583333333333333370, 0.3666666666666666408, 0.3750000000000000000, 0.3833333333333333592, 0.3916666666666666630, 0.4000000000000000222, 0.4083333333333333259, 0.4166666666666666852, 0.4249999999999999889, 0.4333333333333333481, 0.4416666666666666519, 0.4500000000000000111, 0.4583333333333333148, 0.4666666666666666741, 0.4749999999999999778, 0.4833333333333333370, 0.4916666666666666408, 0.5000000000000000000, 0.5083333333333333037, 0.5166666666666667185, 0.5250000000000000222, 0.5333333333333333259, 0.5416666666666666297, 0.5500000000000000444, 0.5583333333333333481, 0.5666666666666666519, 0.5749999999999999556, 0.5833333333333333703, 0.5916666666666666741, 0.5999999999999999778, 0.6083333333333332815, 0.6166666666666666963, 0.6250000000000000000, 0.6333333333333333037, 0.6416666666666667185, 0.6500000000000000222, 0.6583333333333333259, 0.6666666666666666297, 0.6750000000000000444, 0.6833333333333333481, 0.6916666666666666519, 0.6999999999999999556, 0.7083333333333333703, 0.7166666666666666741, 0.7249999999999999778, 0.7333333333333332815, 0.7416666666666666963, 0.7500000000000000000, 0.7583333333333333037, 0.7666666666666667185, 0.7750000000000000222, 0.7833333333333333259, 0.7916666666666666297, 0.8000000000000000444, 0.8083333333333333481, 0.8166666666666666519, 0.8249999999999999556, 0.8333333333333333703, 0.8416666666666666741, 0.8499999999999999778, 0.8583333333333332815, 0.8666666666666666963, 0.8750000000000000000, 0.8833333333333333037, 0.8916666666666667185, 0.9000000000000000222, 0.9083333333333333259, 0.9166666666666666297, 0.9250000000000000444, 0.9333333333333333481, 0.9416666666666666519, 0.9499999999999999556, 0.9583333333333333703, 0.9666666666666666741, 0.9749999999999999778, 0.9833333333333332815, 0.9916666666666666963, 1.000000000000000000 ),
 .UNSPECIFIED. ) 
 GEOMETRIC_REPRESENTATION_ITEM ( )  RATIONAL_B_SPLINE_SURFACE ( (
 ( 1.000000000000000000, 0.8660254037844387076, 1.000000000000000000, 0.8660254037844387076, 1.000000000000000000, 0.8660254037844387076, 1.000000000000000000, 0.8660254037844387076, 1.000000000000000000, 0.8660254037844387076, 1.000000000000000000, 0.8660254037844387076, 1.000000000000000000, 0.8660254037844387076, 1.000000000000000000, 0.8660254037844387076, 1.000000000000000000, 0.8660254037844387076, 1.000000000000000000, 0.8660254037844387076, 1.000000000000000000, 0.8660254037844387076, 1.000000000000000000, 0.8660254037844387076, 1.000000000000000000, 0.8660254037844387076, 1.000000000000000000, 0.8660254037844387076, 1.000000000000000000, 0.8660254037844387076, 1.000000000000000000, 0.8660254037844387076, 1.000000000000000000, 0.8660254037844387076, 1.000000000000000000, 0.8660254037844387076, 1.000000000000000000, 0.8660254037844387076, 1.000000000000000000, 0.8660254037844387076, 1.000000000000000000, 0.8660254037844387076, 1.000000000000000000, 0.8660254037844387076, 1.000000000000000000, 0.8660254037844387076, 1.000000000000000000, 0.8660254037844387076, 1.000000000000000000, 0.8660254037844387076, 1.000000000000000000, 0.8660254037844387076, 1.000000000000000000, 0.8660254037844387076, 1.000000000000000000, 0.8660254037844387076, 1.000000000000000000, 0.8660254037844387076, 1.000000000000000000, 0.8660254037844387076, 1.000000000000000000, 0.8660254037844387076, 1.000000000000000000, 0.8660254037844387076, 1.000000000000000000, 0.8660254037844387076, 1.000000000000000000, 0.8660254037844387076, 1.000000000000000000, 0.8660254037844387076, 1.000000000000000000, 0.8660254037844387076, 1.000000000000000000, 0.8660254037844387076, 1.000000000000000000, 0.8660254037844387076, 1.000000000000000000, 0.8660254037844387076, 1.000000000000000000, 0.8660254037844387076, 1.000000000000000000, 0.8660254037844387076, 1.000000000000000000, 0.8660254037844387076, 1.000000000000000000, 0.8660254037844387076, 1.000000000000000000, 0.8660254037844387076, 1.000000000000000000, 0.8660254037844387076, 1.000000000000000000, 0.8660254037844387076, 1.000000000000000000, 0.8660254037844387076, 1.000000000000000000, 0.8660254037844387076, 1.000000000000000000, 0.8660254037844387076, 1.000000000000000000, 0.8660254037844387076, 1.000000000000000000, 0.8660254037844387076, 1.000000000000000000, 0.8660254037844387076, 1.000000000000000000, 0.8660254037844387076, 1.000000000000000000, 0.8660254037844387076, 1.000000000000000000, 0.8660254037844387076, 1.000000000000000000, 0.8660254037844387076, 1.000000000000000000, 0.8660254037844387076, 1.000000000000000000, 0.8660254037844387076, 1.000000000000000000, 0.8660254037844387076, 1.000000000000000000, 0.8660254037844387076, 1.000000000000000000, 0.8660254037844387076, 1.000000000000000000, 0.8660254037844387076, 1.000000000000000000, 0.8660254037844387076, 1.000000000000000000, 0.8660254037844387076, 1.000000000000000000, 0.8660254037844387076, 1.000000000000000000, 0.8660254037844387076, 1.000000000000000000, 0.8660254037844387076, 1.000000000000000000, 0.8660254037844387076, 1.000000000000000000, 0.8660254037844387076, 1.000000000000000000, 0.8660254037844387076, 1.000000000000000000, 0.8660254037844387076, 1.000000000000000000, 0.8660254037844387076, 1.000000000000000000, 0.8660254037844387076, 1.000000000000000000, 0.8660254037844387076, 1.000000000000000000, 0.8660254037844387076, 1.000000000000000000, 0.8660254037844387076, 1.000000000000000000, 0.8660254037844387076, 1.000000000000000000, 0.8660254037844387076, 1.000000000000000000, 0.8660254037844387076, 1.000000000000000000, 0.8660254037844387076, 1.000000000000000000, 0.8660254037844387076, 1.000000000000000000, 0.8660254037844387076, 1.000000000000000000, 0.8660254037844387076, 1.000000000000000000, 0.8660254037844387076, 1.000000000000000000, 0.8660254037844387076, 1.000000000000000000, 0.8660254037844387076, 1.000000000000000000, 0.8660254037844387076, 1.000000000000000000, 0.8660254037844387076, 1.000000000000000000, 0.8660254037844387076, 1.000000000000000000, 0.8660254037844387076, 1.000000000000000000, 0.8660254037844387076, 1.000000000000000000, 0.8660254037844387076, 1.000000000000000000, 0.8660254037844387076, 1.000000000000000000, 0.8660254037844387076, 1.000000000000000000, 0.8660254037844387076, 1.000000000000000000, 0.8660254037844387076, 1.000000000000000000, 0.8660254037844387076, 1.000000000000000000, 0.8660254037844387076, 1.000000000000000000, 0.8660254037844387076, 1.000000000000000000, 0.8660254037844387076, 1.000000000000000000, 0.8660254037844387076, 1.000000000000000000, 0.8660254037844387076, 1.000000000000000000, 0.8660254037844387076, 1.000000000000000000, 0.8660254037844387076, 1.000000000000000000, 0.8660254037844387076, 1.000000000000000000, 0.8660254037844387076, 1.000000000000000000, 0.8660254037844387076, 1.000000000000000000, 0.8660254037844387076, 1.000000000000000000, 0.8660254037844387076, 1.000000000000000000, 0.8660254037844387076, 1.000000000000000000, 0.8660254037844387076, 1.000000000000000000, 0.8660254037844387076, 1.000000000000000000, 0.8660254037844387076, 1.000000000000000000, 0.8660254037844387076, 1.000000000000000000, 0.8660254037844387076, 1.000000000000000000, 0.8660254037844387076, 1.000000000000000000, 0.8660254037844387076, 1.000000000000000000, 0.8660254037844387076, 1.000000000000000000, 0.8660254037844387076, 1.000000000000000000, 0.8660254037844387076, 1.000000000000000000),
 ( 1.000000000000000000, 0.8660254037844387076, 1.000000000000000000, 0.8660254037844387076, 1.000000000000000000, 0.8660254037844387076, 1.000000000000000000, 0.8660254037844387076, 1.000000000000000000, 0.8660254037844387076, 1.000000000000000000, 0.8660254037844387076, 1.000000000000000000, 0.8660254037844387076, 1.000000000000000000, 0.8660254037844387076, 1.000000000000000000, 0.8660254037844387076, 1.000000000000000000, 0.8660254037844387076, 1.000000000000000000, 0.8660254037844387076, 1.000000000000000000, 0.8660254037844387076, 1.000000000000000000, 0.8660254037844387076, 1.000000000000000000, 0.8660254037844387076, 1.000000000000000000, 0.8660254037844387076, 1.000000000000000000, 0.8660254037844387076, 1.000000000000000000, 0.8660254037844387076, 1.000000000000000000, 0.8660254037844387076, 1.000000000000000000, 0.8660254037844387076, 1.000000000000000000, 0.8660254037844387076, 1.000000000000000000, 0.8660254037844387076, 1.000000000000000000, 0.8660254037844387076, 1.000000000000000000, 0.8660254037844387076, 1.000000000000000000, 0.8660254037844387076, 1.000000000000000000, 0.8660254037844387076, 1.000000000000000000, 0.8660254037844387076, 1.000000000000000000, 0.8660254037844387076, 1.000000000000000000, 0.8660254037844387076, 1.000000000000000000, 0.8660254037844387076, 1.000000000000000000, 0.8660254037844387076, 1.000000000000000000, 0.8660254037844387076, 1.000000000000000000, 0.8660254037844387076, 1.000000000000000000, 0.8660254037844387076, 1.000000000000000000, 0.8660254037844387076, 1.000000000000000000, 0.8660254037844387076, 1.000000000000000000, 0.8660254037844387076, 1.000000000000000000, 0.8660254037844387076, 1.000000000000000000, 0.8660254037844387076, 1.000000000000000000, 0.8660254037844387076, 1.000000000000000000, 0.8660254037844387076, 1.000000000000000000, 0.8660254037844387076, 1.000000000000000000, 0.8660254037844387076, 1.000000000000000000, 0.8660254037844387076, 1.000000000000000000, 0.8660254037844387076, 1.000000000000000000, 0.8660254037844387076, 1.000000000000000000, 0.8660254037844387076, 1.000000000000000000, 0.8660254037844387076, 1.000000000000000000, 0.8660254037844387076, 1.000000000000000000, 0.8660254037844387076, 1.000000000000000000, 0.8660254037844387076, 1.000000000000000000, 0.8660254037844387076, 1.000000000000000000, 0.8660254037844387076, 1.000000000000000000, 0.8660254037844387076, 1.000000000000000000, 0.8660254037844387076, 1.000000000000000000, 0.8660254037844387076, 1.000000000000000000, 0.8660254037844387076, 1.000000000000000000, 0.8660254037844387076, 1.000000000000000000, 0.8660254037844387076, 1.000000000000000000, 0.8660254037844387076, 1.000000000000000000, 0.8660254037844387076, 1.000000000000000000, 0.8660254037844387076, 1.000000000000000000, 0.8660254037844387076, 1.000000000000000000, 0.8660254037844387076, 1.000000000000000000, 0.8660254037844387076, 1.000000000000000000, 0.8660254037844387076, 1.000000000000000000, 0.8660254037844387076, 1.000000000000000000, 0.8660254037844387076, 1.000000000000000000, 0.8660254037844387076, 1.000000000000000000, 0.8660254037844387076, 1.000000000000000000, 0.8660254037844387076, 1.000000000000000000, 0.8660254037844387076, 1.000000000000000000, 0.8660254037844387076, 1.000000000000000000, 0.8660254037844387076, 1.000000000000000000, 0.8660254037844387076, 1.000000000000000000, 0.8660254037844387076, 1.000000000000000000, 0.8660254037844387076, 1.000000000000000000, 0.8660254037844387076, 1.000000000000000000, 0.8660254037844387076, 1.000000000000000000, 0.8660254037844387076, 1.000000000000000000, 0.8660254037844387076, 1.000000000000000000, 0.8660254037844387076, 1.000000000000000000, 0.8660254037844387076, 1.000000000000000000, 0.8660254037844387076, 1.000000000000000000, 0.8660254037844387076, 1.000000000000000000, 0.8660254037844387076, 1.000000000000000000, 0.8660254037844387076, 1.000000000000000000, 0.8660254037844387076, 1.000000000000000000, 0.8660254037844387076, 1.000000000000000000, 0.8660254037844387076, 1.000000000000000000, 0.8660254037844387076, 1.000000000000000000, 0.8660254037844387076, 1.000000000000000000, 0.8660254037844387076, 1.000000000000000000, 0.8660254037844387076, 1.000000000000000000, 0.8660254037844387076, 1.000000000000000000, 0.8660254037844387076, 1.000000000000000000, 0.8660254037844387076, 1.000000000000000000, 0.8660254037844387076, 1.000000000000000000, 0.8660254037844387076, 1.000000000000000000, 0.8660254037844387076, 1.000000000000000000, 0.8660254037844387076, 1.000000000000000000, 0.8660254037844387076, 1.000000000000000000, 0.8660254037844387076, 1.000000000000000000, 0.8660254037844387076, 1.000000000000000000, 0.8660254037844387076, 1.000000000000000000, 0.8660254037844387076, 1.000000000000000000, 0.8660254037844387076, 1.000000000000000000, 0.8660254037844387076, 1.000000000000000000, 0.8660254037844387076, 1.000000000000000000, 0.8660254037844387076, 1.000000000000000000, 0.8660254037844387076, 1.000000000000000000, 0.8660254037844387076, 1.000000000000000000, 0.8660254037844387076, 1.000000000000000000, 0.8660254037844387076, 1.000000000000000000, 0.8660254037844387076, 1.000000000000000000, 0.8660254037844387076, 1.000000000000000000, 0.8660254037844387076, 1.000000000000000000, 0.8660254037844387076, 1.000000000000000000, 0.8660254037844387076, 1.000000000000000000, 0.8660254037844387076, 1.000000000000000000, 0.8660254037844387076, 1.000000000000000000) ) ) 
 REPRESENTATION_ITEM ( '' )  SURFACE ( )  );
#72613=CARTESIAN_POINT ( 'NONE',  ( -6.312203035614172286, 9.521931420595302953, -1.199719254218452047 ) ) ;
#72615=CARTESIAN_POINT ( 'NONE',  ( 4.827426732796687325, 8.217478009653898852, -0.9130428269800896501 ) ) ;
#72618=CARTESIAN_POINT ( 'NONE',  ( 6.966220764712121927, 6.002124920821316323, 2.500000000000000444 ) ) ;
#72620=CARTESIAN_POINT ( 'NONE',  ( 2.911969131885072670, 6.619324097166378706, 0.000000000000000000 ) ) ;
#72630=CARTESIAN_POINT ( 'NONE',  ( -6.668631453075260396, 8.873432343378178544, -1.599625672291271394 ) ) ;
#72645=CARTESIAN_POINT ( 'NONE',  ( 3.061108821635398769, 6.793320401875094561, -0.7998128361456362523 ) ) ;
#72659=CARTESIAN_POINT ( 'NONE',  ( 5.853046489161108035, 7.294594176516559614, 1.271900669079442325 ) ) ;
#72675=AXIS2_PLACEMENT_3D ( 'NONE', #177195, #61306, #158812 ) ;
#72682=EDGE_CURVE ( 'NONE', #53161, #22926, #26576, .T. ) ;
#72688=CARTESIAN_POINT ( 'NONE',  ( -6.382290003970109815, 6.834844811514095397, -0.5765442458998057962 ) ) ;
#72706=CARTESIAN_POINT ( 'NONE',  ( -5.281783360975562225, 8.319775133516907673, 1.199719254218452935 ) ) ;
#72719=EDGE_CURVE ( 'NONE', #95923, #210733, #131883, .T. ) ;
#72724=CARTESIAN_POINT ( 'NONE',  ( 4.655245641445829641, 6.524482229810530498, 1.599625672291269396 ) ) ;
#72734=CARTESIAN_POINT ( 'NONE',  ( 5.107728353013315292, 7.811434107096660640, 1.148430247377411728 ) ) ;
#72752=CARTESIAN_POINT ( 'NONE',  ( -5.061990249855848667, 6.999017606288844284, -1.599625672291271394 ) ) ;
#72754=CARTESIAN_POINT ( 'NONE',  ( 4.386945222473598527, 7.275797305264619652, -1.199719254218452047 ) ) ;
#72757=CARTESIAN_POINT ( 'NONE',  ( -6.720001414228860881, 7.869031733802326123, -1.199719254218452047 ) ) ;
#72760=CARTESIAN_POINT ( 'NONE',  ( 6.444921918449731280, 8.612437886315108315, 1.599625672291268286 ) ) ;
#72765=CARTESIAN_POINT ( 'NONE',  ( -5.535867093699859964, 7.544539992772745229, 1.349747212490030046 ) ) ;
#72775=CARTESIAN_POINT ( 'NONE',  ( -4.950135482320926705, 6.868520377498098739, -1.443375672974066548 ) ) ;
#72784=CARTESIAN_POINT ( 'NONE',  ( 3.594320121398666856, 7.207474218358159490, -1.734723475976807094E-15 ) ) ;
#72787=CARTESIAN_POINT ( 'NONE',  ( -5.562588163356775972, 9.711712967216715953, 0.7998128361456291469 ) ) ;
#72789=EDGE_LOOP ( 'NONE', ( #53079, #63390, #74983, #11267, #156014, #117231 ) ) ;
#72827=CARTESIAN_POINT ( 'NONE',  ( -5.817857314039913241, 5.960124085900898372, 0.000000000000000000 ) ) ;
#72849=CARTESIAN_POINT ( 'NONE',  ( -7.553827861469316396, 8.841829255582865699, -1.199719254218452047 ) ) ;
#72854=CARTESIAN_POINT ( 'NONE',  ( -5.971440312176176768, 5.931378217152456500, 0.000000000000000000 ) ) ;
#72857=DIRECTION ( 'NONE',  ( -1.000000000000000000, 0.000000000000000000, 0.000000000000000000 ) ) ;
#72864=CARTESIAN_POINT ( 'NONE',  ( -7.425025402139490360, 8.691559719698066289, 1.199719254218452047 ) ) ;
#72866=CARTESIAN_POINT ( 'NONE',  ( 6.599791786788117953, 6.770233575417231364, 0.1470628079319712123 ) ) ;
#72870=CARTESIAN_POINT ( 'NONE',  ( 5.065906673361608270, 5.939254536123854677, -1.199719254218450271 ) ) ;
#72875=CARTESIAN_POINT ( 'NONE',  ( -7.611976899429754084, 7.845337568948314022, 0.7998128361456341429 ) ) ;
#72878=CARTESIAN_POINT ( 'NONE',  ( -3.135678666510573365, 6.880318554229450712, 0.000000000000000000 ) ) ;
#72882=EDGE_CURVE ( 'NONE', #135497, #130628, #36932, .T. ) ;
#72885=CARTESIAN_POINT ( 'NONE',  ( 4.204437033569277560, 7.919277282557212416, 0.000000000000000000 ) ) ;
#72886=CARTESIAN_POINT ( 'NONE',  ( -5.628043163004235794, 5.738674243025936761, 0.7216878364870257245 ) ) ;
#72890=CARTESIAN_POINT ( 'NONE',  ( -6.147696309153835692, 6.137010213626393096, 0.7998128361456282587 ) ) ;
#72893=CARTESIAN_POINT ( 'NONE',  ( 5.740951700743842423, 5.662474837148078421, -0.7998128361456481317 ) ) ;
#72898=CARTESIAN_POINT ( 'NONE',  ( -4.492037202130076068, 8.252031063672584210, -0.07255873971346314677 ) ) ;
#72901=CARTESIAN_POINT ( 'NONE',  ( 5.123001941117305336, 7.070197912760590064, 1.599625672291268286 ) ) ;
#72906=CARTESIAN_POINT ( 'NONE',  ( 4.802592184731321545, 8.245026257381830703, 0.8702854636597904259 ) ) ;
#72911=CARTESIAN_POINT ( 'NONE',  ( 5.962700214836534229, 7.205731455156047183, -1.256203146960620076 ) ) ;
#72915=CARTESIAN_POINT ( 'NONE',  ( 5.525830126021535449, 8.604496359403894346, -1.199719254218452047 ) ) ;
#72925=CARTESIAN_POINT ( 'NONE',  ( 5.370783296855561773, 7.572579728427998091, 1.242435897699250891 ) ) ;
#72943=CARTESIAN_POINT ( 'NONE',  ( -7.469616286486262524, 7.679250187180907794, 0.7998128361456341429 ) ) ;
#72949=CARTESIAN_POINT ( 'NONE',  ( -8.014278199453791274, 8.522615118883788199, 1.530808498934192557E-16 ) ) ;
#72956=CARTESIAN_POINT ( 'NONE',  ( 5.794130544993763898, 7.853181283949808744, 1.599625672291269396 ) ) ;
#72964=CARTESIAN_POINT ( 'NONE',  ( 4.472210567661338843, 6.310941310395290493, 1.599625672291261402 ) ) ;
#72967=CARTESIAN_POINT ( 'NONE',  ( 5.695833931072550094, 5.817763472438987726, 0.000000000000000000 ) ) ;
#72976=CARTESIAN_POINT ( 'NONE',  ( 5.553597010146855695, 5.912075037831448832, 0.6282849591137803502 ) ) ;
#72981=CARTESIAN_POINT ( 'NONE',  ( -5.912764389335557702, 8.951956649983198844, 1.082531754730550855 ) ) ;
#72982=CARTESIAN_POINT ( 'NONE',  ( 6.916067756746836714, 8.201738816693689316, -1.082531754730548412 ) ) ;
#72992=CARTESIAN_POINT ( 'NONE',  ( -4.936050443827081580, 7.916420063510339666, 1.199719254218452935 ) ) ;
#72993=CARTESIAN_POINT ( 'NONE',  ( -5.320648938720212051, 5.172121614787156929, 0.000000000000000000 ) ) ;
#72995=CARTESIAN_POINT ( 'NONE',  ( 6.685579144870162693, 6.972466221869550118, -0.7216878364870458196 ) ) ;
#73001=CARTESIAN_POINT ( 'NONE',  ( -2.428612866367529932E-14, 2.999999999999999112, 2.500000000000000444 ) ) ;
#73009=CARTESIAN_POINT ( 'NONE',  ( -4.981341760169012645, 7.953289812593539843, -1.047584607753747399 ) ) ;
#73013=CARTESIAN_POINT ( 'NONE',  ( 6.075462232699553766, 6.260663157670496304, -0.7216878364870458196 ) ) ;
#73019=CARTESIAN_POINT ( 'NONE',  ( -7.279802135894939852, 7.457800344824362604, -0.7998128361456362523 ) ) ;
#73031=CARTESIAN_POINT ( 'NONE',  ( 5.367048706163317640, 7.354919138647580290, -1.599625672291281386 ) ) ;
#73066=CARTESIAN_POINT ( 'NONE',  ( 5.722950238744198614, 8.730506807626655430, 1.082531754730549967 ) ) ;
#73070=CARTESIAN_POINT ( 'NONE',  ( 7.146556367734771875, 8.470642196179646533, 1.082531754730549967 ) ) ;
#73094=CARTESIAN_POINT ( 'NONE',  ( -5.004894982100124068, 5.868074229652107121, 1.199719254218452935 ) ) ;
#73096=CARTESIAN_POINT ( 'NONE',  ( 4.353576723319599218, 8.093273587265928271, -0.7216878364870357165 ) ) ;
#73102=CARTESIAN_POINT ( 'NONE',  ( -3.817502770699643388, 6.611447778194983194, 1.199719254218452935 ) ) ;
#73107=CARTESIAN_POINT ( 'NONE',  ( -6.292392690518202159, 9.394856334696294553, -1.082531754730549967 ) ) ;
#73115=CARTESIAN_POINT ( 'NONE',  ( -5.483346782084204563, 5.361935765378481378, 0.000000000000000000 ) ) ;
#73123=DIRECTION ( 'NONE',  ( 1.000000000000000000, 0.000000000000000000, 0.000000000000000000 ) ) ;
#73124=CARTESIAN_POINT ( 'NONE',  ( -4.442231607132987925, 5.211633625523774960, -1.199719254218453823 ) ) ;
#73127=CARTESIAN_POINT ( 'NONE',  ( -5.370438244788932280, 6.398504386076097283, 1.082531754730549078 ) ) ;
#73129=CARTESIAN_POINT ( 'NONE',  ( -5.438229012412890917, 8.398332043573416783, -1.082531754730549967 ) ) ;
#73130=CARTESIAN_POINT ( 'NONE',  ( 4.037295881819344956, 7.932205305423046582, -0.7998128361456362523 ) ) ;
#73131=CARTESIAN_POINT ( 'NONE',  ( -4.796552484184649856, 8.818004674849227342, -0.7998128361456362523 ) ) ;
#73132=CARTESIAN_POINT ( 'NONE',  ( -7.282664789195997912, 8.525472337930658284, 1.199719254218452047 ) ) ;
#73152=CARTESIAN_POINT ( 'NONE',  ( 5.851225812749518695, 8.984124660586543243, -1.199719254218452047 ) ) ;
#73176=CARTESIAN_POINT ( 'NONE',  ( -3.147653791585727667, 8.920000000000001705, 2.419999999999999485 ) ) ;
#73192=CARTESIAN_POINT ( 'NONE',  ( 6.398522151006641678, 6.429640362454684954, 0.000000000000000000 ) ) ;
#73209=CARTESIAN_POINT ( 'NONE',  ( 4.030516805012513082, 7.924296382481737844, 0.000000000000000000 ) ) ;
#73217=CARTESIAN_POINT ( 'NONE',  ( -7.425025402139490360, 8.691559719698066289, 1.199719254218452047 ) ) ;
#73221=CARTESIAN_POINT ( 'NONE',  ( 5.194709132691408549, 6.089524072008651423, 1.199719254218452935 ) ) ;
#73232=CARTESIAN_POINT ( 'NONE',  ( 7.363486825997814123, 7.763358516518489516, 0.000000000000000000 ) ) ;
#73233=CARTESIAN_POINT ( 'NONE',  ( -5.329763783947941036, 5.390681634126922361, 0.000000000000000000 ) ) ;
#73234=CARTESIAN_POINT ( 'NONE',  ( -6.231907884136888676, 7.299589282028351001, -1.199719254218453823 ) ) ;
#73236=CARTESIAN_POINT ( 'NONE',  ( -5.546112223000226216, 5.929839062422638918, -0.8878705470019981894 ) ) ;
#73246=CARTESIAN_POINT ( 'NONE',  ( 5.662465432362883355, 6.635239754958710989, 1.199719254218451159 ) ) ;
#73247=CARTESIAN_POINT ( 'NONE',  ( 6.225128807330042591, 7.291680359087043151, -1.199719254218452047 ) ) ;
#73250=CARTESIAN_POINT ( 'NONE',  ( 5.189738938980948291, 9.276722205444929870, 0.000000000000000000 ) ) ;
#73266=CARTESIAN_POINT ( 'NONE',  ( 5.316739912341137853, 7.735632174496787528, -1.307268462668280673 ) ) ;
#73269=CARTESIAN_POINT ( 'NONE',  ( 3.810548893104170887, 8.469546410357008170, -2.500000000000001776 ) ) ;
#73271=CARTESIAN_POINT ( 'NONE',  ( 5.598591087800349086, 5.496387455380669529, -0.7998128361456481317 ) ) ;
#73273=CARTESIAN_POINT ( 'NONE',  ( -6.966220764712169000, 6.002124920821316323, -2.420000000000000373 ) ) ;
#73275=CARTESIAN_POINT ( 'NONE',  ( 3.739016502318667445, 7.584212696005614873, 0.7998128361456271485 ) ) ;
#73280=CARTESIAN_POINT ( 'NONE',  ( 4.947799714344386146, 4.737130853015369958, -0.7998128361456481317 ) ) ;
#73285=CARTESIAN_POINT ( 'NONE',  ( 4.584065335196252811, 8.362176967788721882, 0.7216878364870328300 ) ) ;
#73287=CARTESIAN_POINT ( 'NONE',  ( -4.633854640820660009, 8.628190524257904670, -0.7998128361456362523 ) ) ;
#73289=CARTESIAN_POINT ( 'NONE',  ( 6.034787771858531435, 10.05468647722803865, 0.000000000000000000 ) ) ;
#73301=CARTESIAN_POINT ( 'NONE',  ( -3.135678666510573365, 6.880318554229450712, 0.000000000000000000 ) ) ;
#73311=CARTESIAN_POINT ( 'NONE',  ( 0.1003079426142767377, 3.401198454231973756, -1.999680697241537741 ) ) ;
#73331=CARTESIAN_POINT ( 'NONE',  ( 5.072158865288245444, 5.090142562357324429, 0.7216878364870338292 ) ) ;
#73339=CARTESIAN_POINT ( 'NONE',  ( 3.377389663135653031, 6.954388683717978026, -0.7216878364870338292 ) ) ;
#73352=CARTESIAN_POINT ( 'NONE',  ( -4.911796789900812144, 8.952456364851418158, 0.7998128361456291469 ) ) ;
#73354=CARTESIAN_POINT ( 'NONE',  ( 5.790741006368192778, 8.809596036521288198, -1.082531754730548412 ) ) ;
#73365=CARTESIAN_POINT ( 'NONE',  ( -3.786470039966538970, 7.639575156594750283, 0.000000000000000000 ) ) ;
#73370=CARTESIAN_POINT ( 'NONE',  ( -3.174017359375036929, 6.717120995997236221, 0.7216878364870338292 ) ) ;
#73374=CARTESIAN_POINT ( 'NONE',  ( -5.469788628470539926, 5.346117919495872783, -0.7998128361456362523 ) ) ;
#73386=VECTOR ( 'NONE', #158171, 1000.000000000000114 ) ;
#73399=CARTESIAN_POINT ( 'NONE',  ( -3.969505113751027547, 7.853116076009993840, 1.214306433183764966E-14 ) ) ;
#73401=CARTESIAN_POINT ( 'NONE',  ( -5.340986169140711226, 5.195848383611072485, 0.000000000000000000 ) ) ;
#73427=CARTESIAN_POINT ( 'NONE',  ( -4.620296487206990932, 8.612372678375294299, 0.000000000000000000 ) ) ;
#73434=DIRECTION ( 'NONE',  ( 0.000000000000000000, 0.000000000000000000, 1.000000000000000000 ) ) ;
#73441=CARTESIAN_POINT ( 'NONE',  ( -5.618858236835076347, 6.511109054719892875, 1.020627645029206443 ) ) ;
#73445=CARTESIAN_POINT ( 'NONE',  ( 3.250922972226694352, 7.014770244231638863, 0.7998128361456281477 ) ) ;
#73449=B_SPLINE_CURVE_WITH_KNOTS ( 'NONE', 3,
 ( #37848, #118102, #4248, #106913, #134321, #151614, #102854, #83389, #199260, #20513 ),
 .UNSPECIFIED., .F., .F.,
 ( 4, 3, 3, 4 ),
 ( -1.883571653736190889E-06, 0.000000000000000000, 1.648379509549351119E-05, 5.799965632663460626E-05 ),
 .UNSPECIFIED. ) ;
#73455=CARTESIAN_POINT ( 'NONE',  ( 7.147083253059300922, 8.367293879104554577, 1.199719254218452935 ) ) ;
#73457=CARTESIAN_POINT ( 'NONE',  ( 7.191674137406095291, 7.354984346587396082, 0.000000000000000000 ) ) ;
#73459=( BOUNDED_SURFACE ( )  B_SPLINE_SURFACE ( 1, 2, ( 
 ( #183278, #168108, #186473, #87919, #20760, #150804, #55418, #117280, #2368, #3441, #185405, #169165, #202710, #137755, #86854, #68445, #153993, #200575, #152919, #4498, #118350, #70566, #136685, #38109, #170230, #39174, #21815, #5561, #71642, #203774, #121572, #187543, #105257, #171298, #89005, #175583, #176640, #173460, #91141, #90070, #41326, #188613, #156133, #106356, #124773, #40245, #74873, #110638, #208051, #7715, #107436, #8794, #190732, #138818, #192865, #172379, #75934, #72724, #73799, #59678, #27173, #123714, #158269, #209106, #140979, #189676, #42395, #25040, #9858, #60744, #157197, #108505, #142035, #23968, #139893, #191796, #174528, #26106, #92218, #125838, #205924, #43458, #206988, #58617, #93277, #57557, #109579, #159315, #204839, #56492, #10912, #76988, #126906, #143115, #44521, #28252, #94345, #122650, #160387, #32510, #16230, #11987, #177713, #111704, #82314, #29322, #14102, #80192, #163593, #146297, #211248, #64992, #195017, #48774, #179838, #13048, #144188, #95416, #78063, #45588, #112772, #62873, #178783, #129040, #127987, #79127, #212309, #99643, #46649, #61820, #30397, #147342, #180888, #113842, #161468, #148408, #210180, #193941, #96483, #63944, #130099, #81263, #214407, #31459, #145243, #98585, #162530, #196093, #47726, #97536, #15176, #213370, #131146, #197135, #132185, #114889, #164647, #66038, #198191, #49826, #115951, #181941, #33571, #85517, #133242, #149460, #171839, #105813, #55957, #1043, #199247, #156670, #74346, #34633, #73250, #17299, #50894, #190208, #106898, #41868, #138286, #23432, #89543, #100704, #184077, #118092, #155594, #183016, #35696, #205387, #101772, #19437, #117019, #7179, #139357, #151603, #69242, #204301, #2105, #84453, #122110, #165710, #68179, #83377, #67106, #167840, #188075, #166780, #18376, #57026, #3171, #123193, #189154, #134310, #150541, #40793, #39704, #172924, #24500, #90611, #200317, #51968, #8262, #140450, #206461, #58088, #124250, #208582, #28796, #129579, #107977, #77534, #78599, #43994, #175062, #127452, #29870, #63427, #61291, #145786, #12526 ),
 ( #60215, #193423, #95953, #126376, #11461, #111178, #9338, #191267, #144719, #143655, #209650, #45067, #177180, #141524, #94880, #158794, #142575, #210731, #42933, #75411, #10391, #25577, #174006, #192335, #62357, #162008, #194486, #160932, #92750, #128518, #91688, #27723, #46129, #112246, #157741, #59151, #13597, #109043, #178257, #207532, #125309, #195566, #79671, #26649, #211789, #76466, #110112, #176123, #93817, #159858, #116493, #64492, #131671, #83920, #213903, #115435, #146836, #50370, #182482, #181426, #165183, #82861, #98080, #180375, #16777, #68720, #164135, #134842, #163073, #49318, #148937, #47202, #113317, #34110, #33056, #166247, #67642, #15719, #212855, #150011, #509, #100182, #133789, #99134, #179323, #30944, #17837, #1581, #183556, #65526, #130634, #147887, #199797, #97019, #14654, #66577, #51442, #197674, #114380, #132719, #35163, #2647, #198724, #84992, #117561, #101239, #167321, #18908, #151083, #80748, #196626, #48266, #31999, #81804, #70847, #186756, #122934, #53563, #136962, #19978, #38379, #88201, #52496, #56768, #202989, #89286, #103383, #24240, #153198, #155334, #4769, #3707, #6918, #72995, #169445, #21030, #23171, #90342, #54629, #87128, #86062, #74090, #156411, #7998, #120776, #105540, #36229, #104460, #200845, #118626, #154274, #170507, #5849, #135892, #168382, #22089, #152139, #184612, #204043, #138029, #71919, #102308, #69784, #188891, #171574, #139097, #55693, #201910, #205124, #121848, #187819, #40532, #39446, #119696, #185680, #106636, #172664, #37309, #158541, #9082, #26390, #61035, #161753, #140181, #109858, #110917, #76213, #207274, #159602, #62110, #95698, #93558, #177999, #44813, #10138, #78345, #77281, #176923, #11200, #59964, #209391, #29613, #210472, #142323, #126119, #128269, #58905, #208333, #173748, #192079, #27460, #206203, #194231, #43745, #28538, #42681, #13344, #92502, #94630, #175872, #157487, #160673, #12268, #108788, #174814, #144468, #57831, #143393, #127196, #25325, #123992, #189960, #41610, #193163, #45875, #107721, #111997, #91426, #75156, #141266, #125058 ) ),
 .UNSPECIFIED., .F., .F., .T. ) 
 B_SPLINE_SURFACE_WITH_KNOTS ( ( 2, 2 ),
 ( 3, 2, 2, 2, 2, 2, 2, 2, 2, 2, 2, 2, 2, 2, 2, 2, 2, 2, 2, 2, 2, 2, 2, 2, 2, 2, 2, 2, 2, 2, 2, 2, 2, 2, 2, 2, 2, 2, 2, 2, 2, 2, 2, 2, 2, 2, 2, 2, 2, 2, 2, 2, 2, 2, 2, 2, 2, 2, 2, 2, 2, 2, 2, 2, 2, 2, 2, 2, 2, 2, 2, 2, 2, 2, 2, 2, 2, 2, 2, 2, 2, 2, 2, 2, 2, 2, 2, 2, 2, 2, 2, 2, 2, 2, 2, 2, 2, 2, 2, 2, 2, 2, 2, 2, 2, 2, 2, 2, 2, 2, 2, 2, 2, 2, 2, 2, 2, 2, 2, 2, 3 ),
 ( 0.000000000000000000, 1.000000000000000000 ),
 ( 0.000000000000000000, 0.008333333333333333218, 0.01666666666666666644, 0.02500000000000000139, 0.03333333333333333287, 0.04166666666666666435, 0.05000000000000000278, 0.05833333333333333426, 0.06666666666666666574, 0.07499999999999999722, 0.08333333333333332871, 0.09166666666666666019, 0.1000000000000000056, 0.1083333333333333370, 0.1166666666666666685, 0.1250000000000000000, 0.1333333333333333315, 0.1416666666666666630, 0.1499999999999999944, 0.1583333333333333259, 0.1666666666666666574, 0.1749999999999999889, 0.1833333333333333204, 0.1916666666666666796, 0.2000000000000000111, 0.2083333333333333426, 0.2166666666666666741, 0.2250000000000000056, 0.2333333333333333370, 0.2416666666666666685, 0.2500000000000000000, 0.2583333333333333592, 0.2666666666666666630, 0.2750000000000000222, 0.2833333333333333259, 0.2916666666666666852, 0.2999999999999999889, 0.3083333333333333481, 0.3166666666666666519, 0.3250000000000000111, 0.3333333333333333148, 0.3416666666666666741, 0.3499999999999999778, 0.3583333333333333370, 0.3666666666666666408, 0.3750000000000000000, 0.3833333333333333592, 0.3916666666666666630, 0.4000000000000000222, 0.4083333333333333259, 0.4166666666666666852, 0.4249999999999999889, 0.4333333333333333481, 0.4416666666666666519, 0.4500000000000000111, 0.4583333333333333148, 0.4666666666666666741, 0.4749999999999999778, 0.4833333333333333370, 0.4916666666666666408, 0.5000000000000000000, 0.5083333333333333037, 0.5166666666666667185, 0.5250000000000000222, 0.5333333333333333259, 0.5416666666666666297, 0.5500000000000000444, 0.5583333333333333481, 0.5666666666666666519, 0.5749999999999999556, 0.5833333333333333703, 0.5916666666666666741, 0.5999999999999999778, 0.6083333333333332815, 0.6166666666666666963, 0.6250000000000000000, 0.6333333333333333037, 0.6416666666666667185, 0.6500000000000000222, 0.6583333333333333259, 0.6666666666666666297, 0.6750000000000000444, 0.6833333333333333481, 0.6916666666666666519, 0.6999999999999999556, 0.7083333333333333703, 0.7166666666666666741, 0.7249999999999999778, 0.7333333333333332815, 0.7416666666666666963, 0.7500000000000000000, 0.7583333333333333037, 0.7666666666666667185, 0.7750000000000000222, 0.7833333333333333259, 0.7916666666666666297, 0.8000000000000000444, 0.8083333333333333481, 0.8166666666666666519, 0.8249999999999999556, 0.8333333333333333703, 0.8416666666666666741, 0.8499999999999999778, 0.8583333333333332815, 0.8666666666666666963, 0.8750000000000000000, 0.8833333333333333037, 0.8916666666666667185, 0.9000000000000000222, 0.9083333333333333259, 0.9166666666666666297, 0.9250000000000000444, 0.9333333333333333481, 0.9416666666666666519, 0.9499999999999999556, 0.9583333333333333703, 0.9666666666666666741, 0.9749999999999999778, 0.9833333333333332815, 0.9916666666666666963, 1.000000000000000000 ),
 .UNSPECIFIED. ) 
 GEOMETRIC_REPRESENTATION_ITEM ( )  RATIONAL_B_SPLINE_SURFACE ( (
 ( 1.000000000000000000, 0.8660254037844387076, 1.000000000000000000, 0.8660254037844387076, 1.000000000000000000, 0.8660254037844387076, 1.000000000000000000, 0.8660254037844387076, 1.000000000000000000, 0.8660254037844387076, 1.000000000000000000, 0.8660254037844387076, 1.000000000000000000, 0.8660254037844387076, 1.000000000000000000, 0.8660254037844387076, 1.000000000000000000, 0.8660254037844387076, 1.000000000000000000, 0.8660254037844387076, 1.000000000000000000, 0.8660254037844387076, 1.000000000000000000, 0.8660254037844387076, 1.000000000000000000, 0.8660254037844387076, 1.000000000000000000, 0.8660254037844387076, 1.000000000000000000, 0.8660254037844387076, 1.000000000000000000, 0.8660254037844387076, 1.000000000000000000, 0.8660254037844387076, 1.000000000000000000, 0.8660254037844387076, 1.000000000000000000, 0.8660254037844387076, 1.000000000000000000, 0.8660254037844387076, 1.000000000000000000, 0.8660254037844387076, 1.000000000000000000, 0.8660254037844387076, 1.000000000000000000, 0.8660254037844387076, 1.000000000000000000, 0.8660254037844387076, 1.000000000000000000, 0.8660254037844387076, 1.000000000000000000, 0.8660254037844387076, 1.000000000000000000, 0.8660254037844387076, 1.000000000000000000, 0.8660254037844387076, 1.000000000000000000, 0.8660254037844387076, 1.000000000000000000, 0.8660254037844387076, 1.000000000000000000, 0.8660254037844387076, 1.000000000000000000, 0.8660254037844387076, 1.000000000000000000, 0.8660254037844387076, 1.000000000000000000, 0.8660254037844387076, 1.000000000000000000, 0.8660254037844387076, 1.000000000000000000, 0.8660254037844387076, 1.000000000000000000, 0.8660254037844387076, 1.000000000000000000, 0.8660254037844387076, 1.000000000000000000, 0.8660254037844387076, 1.000000000000000000, 0.8660254037844387076, 1.000000000000000000, 0.8660254037844387076, 1.000000000000000000, 0.8660254037844387076, 1.000000000000000000, 0.8660254037844387076, 1.000000000000000000, 0.8660254037844387076, 1.000000000000000000, 0.8660254037844387076, 1.000000000000000000, 0.8660254037844387076, 1.000000000000000000, 0.8660254037844387076, 1.000000000000000000, 0.8660254037844387076, 1.000000000000000000, 0.8660254037844387076, 1.000000000000000000, 0.8660254037844387076, 1.000000000000000000, 0.8660254037844387076, 1.000000000000000000, 0.8660254037844387076, 1.000000000000000000, 0.8660254037844387076, 1.000000000000000000, 0.8660254037844387076, 1.000000000000000000, 0.8660254037844387076, 1.000000000000000000, 0.8660254037844387076, 1.000000000000000000, 0.8660254037844387076, 1.000000000000000000, 0.8660254037844387076, 1.000000000000000000, 0.8660254037844387076, 1.000000000000000000, 0.8660254037844387076, 1.000000000000000000, 0.8660254037844387076, 1.000000000000000000, 0.8660254037844387076, 1.000000000000000000, 0.8660254037844387076, 1.000000000000000000, 0.8660254037844387076, 1.000000000000000000, 0.8660254037844387076, 1.000000000000000000, 0.8660254037844387076, 1.000000000000000000, 0.8660254037844387076, 1.000000000000000000, 0.8660254037844387076, 1.000000000000000000, 0.8660254037844387076, 1.000000000000000000, 0.8660254037844387076, 1.000000000000000000, 0.8660254037844387076, 1.000000000000000000, 0.8660254037844387076, 1.000000000000000000, 0.8660254037844387076, 1.000000000000000000, 0.8660254037844387076, 1.000000000000000000, 0.8660254037844387076, 1.000000000000000000, 0.8660254037844387076, 1.000000000000000000, 0.8660254037844387076, 1.000000000000000000, 0.8660254037844387076, 1.000000000000000000, 0.8660254037844387076, 1.000000000000000000, 0.8660254037844387076, 1.000000000000000000, 0.8660254037844387076, 1.000000000000000000, 0.8660254037844387076, 1.000000000000000000, 0.8660254037844387076, 1.000000000000000000, 0.8660254037844387076, 1.000000000000000000, 0.8660254037844387076, 1.000000000000000000, 0.8660254037844387076, 1.000000000000000000, 0.8660254037844387076, 1.000000000000000000, 0.8660254037844387076, 1.000000000000000000, 0.8660254037844387076, 1.000000000000000000, 0.8660254037844387076, 1.000000000000000000, 0.8660254037844387076, 1.000000000000000000, 0.8660254037844387076, 1.000000000000000000, 0.8660254037844387076, 1.000000000000000000, 0.8660254037844387076, 1.000000000000000000, 0.8660254037844387076, 1.000000000000000000, 0.8660254037844387076, 1.000000000000000000, 0.8660254037844387076, 1.000000000000000000, 0.8660254037844387076, 1.000000000000000000, 0.8660254037844387076, 1.000000000000000000, 0.8660254037844387076, 1.000000000000000000, 0.8660254037844387076, 1.000000000000000000, 0.8660254037844387076, 1.000000000000000000, 0.8660254037844387076, 1.000000000000000000, 0.8660254037844387076, 1.000000000000000000, 0.8660254037844387076, 1.000000000000000000, 0.8660254037844387076, 1.000000000000000000, 0.8660254037844387076, 1.000000000000000000, 0.8660254037844387076, 1.000000000000000000, 0.8660254037844387076, 1.000000000000000000, 0.8660254037844387076, 1.000000000000000000, 0.8660254037844387076, 1.000000000000000000, 0.8660254037844387076, 1.000000000000000000, 0.8660254037844387076, 1.000000000000000000, 0.8660254037844387076, 1.000000000000000000, 0.8660254037844387076, 1.000000000000000000, 0.8660254037844387076, 1.000000000000000000, 0.8660254037844387076, 1.000000000000000000, 0.8660254037844387076, 1.000000000000000000, 0.8660254037844387076, 1.000000000000000000, 0.8660254037844387076, 1.000000000000000000),
 ( 1.000000000000000000, 0.8660254037844387076, 1.000000000000000000, 0.8660254037844387076, 1.000000000000000000, 0.8660254037844387076, 1.000000000000000000, 0.8660254037844387076, 1.000000000000000000, 0.8660254037844387076, 1.000000000000000000, 0.8660254037844387076, 1.000000000000000000, 0.8660254037844387076, 1.000000000000000000, 0.8660254037844387076, 1.000000000000000000, 0.8660254037844387076, 1.000000000000000000, 0.8660254037844387076, 1.000000000000000000, 0.8660254037844387076, 1.000000000000000000, 0.8660254037844387076, 1.000000000000000000, 0.8660254037844387076, 1.000000000000000000, 0.8660254037844387076, 1.000000000000000000, 0.8660254037844387076, 1.000000000000000000, 0.8660254037844387076, 1.000000000000000000, 0.8660254037844387076, 1.000000000000000000, 0.8660254037844387076, 1.000000000000000000, 0.8660254037844387076, 1.000000000000000000, 0.8660254037844387076, 1.000000000000000000, 0.8660254037844387076, 1.000000000000000000, 0.8660254037844387076, 1.000000000000000000, 0.8660254037844387076, 1.000000000000000000, 0.8660254037844387076, 1.000000000000000000, 0.8660254037844387076, 1.000000000000000000, 0.8660254037844387076, 1.000000000000000000, 0.8660254037844387076, 1.000000000000000000, 0.8660254037844387076, 1.000000000000000000, 0.8660254037844387076, 1.000000000000000000, 0.8660254037844387076, 1.000000000000000000, 0.8660254037844387076, 1.000000000000000000, 0.8660254037844387076, 1.000000000000000000, 0.8660254037844387076, 1.000000000000000000, 0.8660254037844387076, 1.000000000000000000, 0.8660254037844387076, 1.000000000000000000, 0.8660254037844387076, 1.000000000000000000, 0.8660254037844387076, 1.000000000000000000, 0.8660254037844387076, 1.000000000000000000, 0.8660254037844387076, 1.000000000000000000, 0.8660254037844387076, 1.000000000000000000, 0.8660254037844387076, 1.000000000000000000, 0.8660254037844387076, 1.000000000000000000, 0.8660254037844387076, 1.000000000000000000, 0.8660254037844387076, 1.000000000000000000, 0.8660254037844387076, 1.000000000000000000, 0.8660254037844387076, 1.000000000000000000, 0.8660254037844387076, 1.000000000000000000, 0.8660254037844387076, 1.000000000000000000, 0.8660254037844387076, 1.000000000000000000, 0.8660254037844387076, 1.000000000000000000, 0.8660254037844387076, 1.000000000000000000, 0.8660254037844387076, 1.000000000000000000, 0.8660254037844387076, 1.000000000000000000, 0.8660254037844387076, 1.000000000000000000, 0.8660254037844387076, 1.000000000000000000, 0.8660254037844387076, 1.000000000000000000, 0.8660254037844387076, 1.000000000000000000, 0.8660254037844387076, 1.000000000000000000, 0.8660254037844387076, 1.000000000000000000, 0.8660254037844387076, 1.000000000000000000, 0.8660254037844387076, 1.000000000000000000, 0.8660254037844387076, 1.000000000000000000, 0.8660254037844387076, 1.000000000000000000, 0.8660254037844387076, 1.000000000000000000, 0.8660254037844387076, 1.000000000000000000, 0.8660254037844387076, 1.000000000000000000, 0.8660254037844387076, 1.000000000000000000, 0.8660254037844387076, 1.000000000000000000, 0.8660254037844387076, 1.000000000000000000, 0.8660254037844387076, 1.000000000000000000, 0.8660254037844387076, 1.000000000000000000, 0.8660254037844387076, 1.000000000000000000, 0.8660254037844387076, 1.000000000000000000, 0.8660254037844387076, 1.000000000000000000, 0.8660254037844387076, 1.000000000000000000, 0.8660254037844387076, 1.000000000000000000, 0.8660254037844387076, 1.000000000000000000, 0.8660254037844387076, 1.000000000000000000, 0.8660254037844387076, 1.000000000000000000, 0.8660254037844387076, 1.000000000000000000, 0.8660254037844387076, 1.000000000000000000, 0.8660254037844387076, 1.000000000000000000, 0.8660254037844387076, 1.000000000000000000, 0.8660254037844387076, 1.000000000000000000, 0.8660254037844387076, 1.000000000000000000, 0.8660254037844387076, 1.000000000000000000, 0.8660254037844387076, 1.000000000000000000, 0.8660254037844387076, 1.000000000000000000, 0.8660254037844387076, 1.000000000000000000, 0.8660254037844387076, 1.000000000000000000, 0.8660254037844387076, 1.000000000000000000, 0.8660254037844387076, 1.000000000000000000, 0.8660254037844387076, 1.000000000000000000, 0.8660254037844387076, 1.000000000000000000, 0.8660254037844387076, 1.000000000000000000, 0.8660254037844387076, 1.000000000000000000, 0.8660254037844387076, 1.000000000000000000, 0.8660254037844387076, 1.000000000000000000, 0.8660254037844387076, 1.000000000000000000, 0.8660254037844387076, 1.000000000000000000, 0.8660254037844387076, 1.000000000000000000, 0.8660254037844387076, 1.000000000000000000, 0.8660254037844387076, 1.000000000000000000, 0.8660254037844387076, 1.000000000000000000, 0.8660254037844387076, 1.000000000000000000, 0.8660254037844387076, 1.000000000000000000, 0.8660254037844387076, 1.000000000000000000, 0.8660254037844387076, 1.000000000000000000, 0.8660254037844387076, 1.000000000000000000, 0.8660254037844387076, 1.000000000000000000, 0.8660254037844387076, 1.000000000000000000, 0.8660254037844387076, 1.000000000000000000, 0.8660254037844387076, 1.000000000000000000, 0.8660254037844387076, 1.000000000000000000, 0.8660254037844387076, 1.000000000000000000, 0.8660254037844387076, 1.000000000000000000, 0.8660254037844387076, 1.000000000000000000, 0.8660254037844387076, 1.000000000000000000, 0.8660254037844387076, 1.000000000000000000, 0.8660254037844387076, 1.000000000000000000) ) ) 
 REPRESENTATION_ITEM ( '' )  SURFACE ( )  );
#73462=CARTESIAN_POINT ( 'NONE',  ( -1.793747577714859487, 2.512287210193241194, -2.500000000000000444 ) ) ;
#73471=CARTESIAN_POINT ( 'NONE',  ( 6.361499291607088935, 6.832587723092125032, 0.6030276918116053153 ) ) ;
#73473=CARTESIAN_POINT ( 'NONE',  ( 5.343321937561575474, 8.287607122913563273, -1.082531754730548412 ) ) ;
#73478=VECTOR ( 'NONE', #37004, 1000.000000000000000 ) ;
#73482=CARTESIAN_POINT ( 'NONE',  ( -4.442231607132987925, 5.211633625523774960, -1.199719254218453823 ) ) ;
#73483=CARTESIAN_POINT ( 'NONE',  ( 3.634019179650556097, 7.351260730161411239, -0.2183562399340302218 ) ) ;
#73493=CARTESIAN_POINT ( 'NONE',  ( -5.031484404002922517, 6.963427452793760963, 1.443375672974058777 ) ) ;
#73497=CARTESIAN_POINT ( 'NONE',  ( 7.180978637093494044, 8.406838493811077839, -1.199719254218452047 ) ) ;
#73515=CARTESIAN_POINT ( 'NONE',  ( 4.681308178468477799, 8.683552984847038303, 0.000000000000000000 ) ) ;
#73522=AXIS2_PLACEMENT_3D ( 'NONE', #184094, #72468, #136441 ) ;
#73531=EDGE_CURVE ( 'NONE', #44, #210733, #62718, .T. ) ;
#73552=EDGE_CURVE ( 'NONE', #182199, #45216, #155871, .T. ) ;
#73558=CARTESIAN_POINT ( 'NONE',  ( 5.885648082108200896, 6.039213315313952002, 0.7216878364870328300 ) ) ;
#73568=CARTESIAN_POINT ( 'NONE',  ( -4.882344714696960075, 5.829061934302122161, 1.082531754730549078 ) ) ;
#73599=CARTESIAN_POINT ( 'NONE',  ( 5.876533236880477240, 5.820653295974182129, 0.7998128361456352531 ) ) ;
#73602=CARTESIAN_POINT ( 'NONE',  ( -9.336326716892651589, 8.920000000000001705, 2.500000000000000444 ) ) ;
#73613=CARTESIAN_POINT ( 'NONE',  ( -6.780486220610186798, 8.043560357867583832, -1.082531754730549967 ) ) ;
#73615=CARTESIAN_POINT ( 'NONE',  ( 5.176180785367283654, 9.260904359562321275, -0.7998128361456481317 ) ) ;
#73627=VECTOR ( 'NONE', #50437, 1000.000000000000000 ) ;
#73633=CARTESIAN_POINT ( 'NONE',  ( 4.927462483923885195, 4.713404084191450849, -0.7998128361456481317 ) ) ;
#73635=CARTESIAN_POINT ( 'NONE',  ( -4.340018570150322219, 5.196348098997705556, -1.082531754730551743 ) ) ;
#73651=ORIENTED_EDGE ( 'NONE', *, *, #47472, .T. ) ;
#73666=CARTESIAN_POINT ( 'NONE',  ( -8.093291352714894415, 8.406871097780989288, -0.7998128361456362523 ) ) ;
#73669=CARTESIAN_POINT ( 'NONE',  ( -5.088052786878465739, 9.158088361325352977, 0.000000000000000000 ) ) ;
#73670=CARTESIAN_POINT ( 'NONE',  ( -5.608413262169404945, 5.655525674710887962, 0.4595228360113173260 ) ) ;
#73674=CARTESIAN_POINT ( 'NONE',  ( -7.092323753280154186, 7.447001598347859463, 0.7216878364870317197 ) ) ;
#73680=CARTESIAN_POINT ( 'NONE',  ( -3.383641855062333281, 6.105276709951447778, -1.199719254218452047 ) ) ;
#73688=CARTESIAN_POINT ( 'NONE',  ( -1.880721860161314041, 2.480169305151522341, 2.464325445266503323 ) ) ;
#73689=CARTESIAN_POINT ( 'NONE',  ( -7.456058132872594335, 7.663432341298296535, 0.000000000000000000 ) ) ;
#73691=CARTESIAN_POINT ( 'NONE',  ( 4.807910157829258679, 8.239027388120819140, -0.8806314816870459694 ) ) ;
#73696=CARTESIAN_POINT ( 'NONE',  ( 5.982890925380405456, 10.20206618957764100, 0.000000000000000000 ) ) ;
#73719=CARTESIAN_POINT ( 'NONE',  ( 7.452141709366786770, 8.723195411463290583, 1.199719254218452047 ) ) ;
#73735=CARTESIAN_POINT ( 'NONE',  ( 5.652821694808577213, 7.451312062667313718, 1.328372732707931103 ) ) ;
#73736=CARTESIAN_POINT ( 'NONE',  ( -5.302647476276252547, 5.359045941843285199, 0.7216878364870257245 ) ) ;
#73763=CARTESIAN_POINT ( 'NONE',  ( 4.903208829997618423, 5.749440385532527564, -1.199719254218450271 ) ) ;
#73780=CARTESIAN_POINT ( 'NONE',  ( -6.469175572376043348, 7.576401584974034265, 1.199719254218452047 ) ) ;
#73791=DIRECTION ( 'NONE',  ( 0.7927788072564095900, 0.000000000000000000, -0.6095094443608766177 ) ) ;
#73799=CARTESIAN_POINT ( 'NONE',  ( 5.194709132691408549, 6.089524072008651423, 1.199719254218452935 ) ) ;
#73801=CARTESIAN_POINT ( 'NONE',  ( 5.980555156959511898, 9.991415093179179863, -0.7216878364870458196 ) ) ;
#73810=B_SPLINE_CURVE_WITH_KNOTS ( 'NONE', 3,
 ( #45905, #129359, #13371, #32829 ),
 .UNSPECIFIED., .F., .F.,
 ( 4, 4 ),
 ( 0.000000000000000000, 0.0002847049822659113399 ),
 .UNSPECIFIED. ) ;
#73811=CARTESIAN_POINT ( 'NONE',  ( 5.916355900263067014, 7.140870225795406867, 1.119544393390920600 ) ) ;
#73813=B_SPLINE_CURVE_WITH_KNOTS ( 'NONE', 3,
 ( #26337, #5791, #173697, #104407, #208279, #170456, #71868, #142268, #41556, #25273 ),
 .UNSPECIFIED., .F., .F.,
 ( 4, 3, 3, 4 ),
 ( 1.740265443795535820E-15, 3.125156195614331076E-05, 5.753630127952281341E-05, 8.382839040627577314E-05 ),
 .UNSPECIFIED. ) ;
#73814=CARTESIAN_POINT ( 'NONE',  ( -6.329301559086026430, 6.910747120380293929, 0.8034454130101459368 ) ) ;
#73832=CARTESIAN_POINT ( 'NONE',  ( -5.330290668828105538, 6.247702530834755130, 1.199719254218452935 ) ) ;
#73834=CARTESIAN_POINT ( 'NONE',  ( 5.032011289327418702, 5.899709921417326974, 1.199719254218452935 ) ) ;
#73837=CARTESIAN_POINT ( 'NONE',  ( -5.101610940492132151, 9.173906207207963348, -0.7998128361456362523 ) ) ;
#73841=CARTESIAN_POINT ( 'NONE',  ( 7.035755370848908896, 7.173079118937375931, 0.7998128361456352531 ) ) ;
#73842=CYLINDRICAL_SURFACE ( 'NONE', #186052, 1.250000000000000000 ) ;
#73847=CARTESIAN_POINT ( 'NONE',  ( -4.588266729941921973, 8.494429388143421633, -0.1275441020149002680 ) ) ;
#73855=CARTESIAN_POINT ( 'NONE',  ( -4.706088717274938382, 6.583799151611112954, 1.443375672974058777 ) ) ;
#73856=VECTOR ( 'NONE', #83577, 1000.000000000000000 ) ;
#73866=CARTESIAN_POINT ( 'NONE',  ( 3.743459811148990291, 7.381470523066878009, -0.7216878364870338292 ) ) ;
#73871=CARTESIAN_POINT ( 'NONE',  ( -6.720001414228860881, 7.869031733802326123, -1.199719254218452047 ) ) ;
#73887=CARTESIAN_POINT ( 'NONE',  ( 4.085803189671889157, 5.860132702740892263, -1.599625672291273171 ) ) ;
#73914=CARTESIAN_POINT ( 'NONE',  ( -6.617788377246204945, 6.893376992974917350, -0.7216878364870338292 ) ) ;
#73936=CARTESIAN_POINT ( 'NONE',  ( -4.841670253411603397, 5.781608396135871075, 1.082531754730549078 ) ) ;
#73937=CARTESIAN_POINT ( 'NONE',  ( -4.462568837553487100, 5.235360394347691404, -1.199719254218453823 ) ) ;
#73941=CARTESIAN_POINT ( 'NONE',  ( -3.447516199624892419, 7.244129009529488350, 0.7998128361456352531 ) ) ;
#73952=CARTESIAN_POINT ( 'NONE',  ( -5.915100157312088491, 10.12297696016459092, -0.7998128361456362523 ) ) ;
#73954=CARTESIAN_POINT ( 'NONE',  ( 6.454497976780569246, 6.866128686250288382, -0.6735470152485992790 ) ) ;
#73958=CARTESIAN_POINT ( 'NONE',  ( 5.204350862799327793, 7.165104988056252289, -1.599625672291281386 ) ) ;
#73963=CARTESIAN_POINT ( 'NONE',  ( -6.129167961829681488, 9.308390501180058507, -1.199719254218452047 ) ) ;
#73967=CARTESIAN_POINT ( 'NONE',  ( -4.604929450496978660, 5.401447776115099408, -1.199719254218453823 ) ) ;
#73972=CARTESIAN_POINT ( 'NONE',  ( 6.658462837642799670, 6.940830530104329377, 0.7216878364870328300 ) ) ;
#73973=CARTESIAN_POINT ( 'NONE',  ( -5.112833325684916552, 7.058334528089422300, -1.443375672974066548 ) ) ;
#73976=CARTESIAN_POINT ( 'NONE',  ( -3.772911886352873445, 7.623757310712139912, 0.7998128361456350310 ) ) ;
#73980=CARTESIAN_POINT ( 'NONE',  ( 5.252858170651868441, 5.093032385374103299, -0.7998128361456481317 ) ) ;
#73987=DIRECTION ( 'NONE',  ( 0.6507913734559641616, 0.7592566023653004592, 0.000000000000000000 ) ) ;
#73989=VECTOR ( 'NONE', #78006, 1000.000000000000114 ) ;
#73992=CARTESIAN_POINT ( 'NONE',  ( 5.371503168974233411, 7.687194297833679357, 1.321221623412481394 ) ) ;
#74001=CARTESIAN_POINT ( 'NONE',  ( 5.417364897112183719, 8.477953592343014932, 1.199719254218451159 ) ) ;
#74012=CARTESIAN_POINT ( 'NONE',  ( 6.476386945563378461, 6.757828299745357370, 0.2189195654383000456 ) ) ;
#74015=ADVANCED_FACE ( 'NONE', ( #178702 ), #207991, .T. ) ;
#74025=CARTESIAN_POINT ( 'NONE',  ( -4.620365152176808543, 8.363145938788004941, -0.2588828456067792660 ) ) ;
#74033=CARTESIAN_POINT ( 'NONE',  ( -7.605197822622922210, 7.837428646007010613, -0.7998128361456362523 ) ) ;
#74047=CARTESIAN_POINT ( 'NONE',  ( 7.713663051532233972, 7.963971413067895355, -0.7998128361456341429 ) ) ;
#74054=CARTESIAN_POINT ( 'NONE',  ( 3.366167277942881064, 7.149221934233827014, -0.7998128361456362523 ) ) ;
#74057=CARTESIAN_POINT ( 'NONE',  ( 3.553645660113312399, 7.160020680191912845, -1.734723475976807094E-15 ) ) ;
#74071=CARTESIAN_POINT ( 'NONE',  ( -6.102578539926875933, 10.13377570664109051, 0.7216878364870267237 ) ) ;
#74072=CARTESIAN_POINT ( 'NONE',  ( 4.415115299905642665, 5.179997933758551554, -1.199719254218450271 ) ) ;
#74087=CARTESIAN_POINT ( 'NONE',  ( -5.798046968499580345, 6.793418213784815585, 1.199719254218452935 ) ) ;
#74088=CARTESIAN_POINT ( 'NONE',  ( -5.367048706163331850, 7.354919138647580290, -1.599625672291271394 ) ) ;
#74090=CARTESIAN_POINT ( 'NONE',  ( 5.844973620822835336, 7.912498205750389424, 1.443375672974064550 ) ) ;
#74101=CARTESIAN_POINT ( 'NONE',  ( -4.929275754869433257, 8.007250896656138650, 0.9949873637682864480 ) ) ;
#74102=CARTESIAN_POINT ( 'NONE',  ( -4.495112795249930571, 8.049017979306610115, -2.444655174081867166 ) ) ;
#74105=CARTESIAN_POINT ( 'NONE',  ( 4.502716413514295191, 6.346531463890372926, -1.443375672974068769 ) ) ;
#74110=CARTESIAN_POINT ( 'NONE',  ( -6.631873415740034083, 7.766215735565355160, 1.199719254218452047 ) ) ;
#74124=CARTESIAN_POINT ( 'NONE',  ( 4.746236293235721604, 7.694970221153795364, 1.199719254218451159 ) ) ;
#74135=B_SPLINE_CURVE_WITH_KNOTS ( 'NONE', 3,
 ( #22284, #89476, #117757, #101432, #135025, #155531, #55887, #23367, #186943, #2837 ),
 .UNSPECIFIED., .F., .F.,
 ( 4, 3, 3, 4 ),
 ( 9.585285410731671485E-17, 4.411882185274044424E-05, 8.611515704366408169E-05, 0.0001647628875604093836 ),
 .UNSPECIFIED. ) ;
#74136=CARTESIAN_POINT ( 'NONE',  ( -4.864214080903581205, 4.879786425613829692, -0.6392378712632117432 ) ) ;
#74163=CARTESIAN_POINT ( 'NONE',  ( 7.187230829020130329, 7.557726520044554697, 0.7216878364870267237 ) ) ;
#74167=DIRECTION ( 'NONE',  ( 1.000000000000000000, 0.000000000000000000, 0.000000000000000000 ) ) ;
#74168=CARTESIAN_POINT ( 'NONE',  ( 7.038091138825468107, 8.344099429118761790, -1.082531754730548412 ) ) ;
#74195=CARTESIAN_POINT ( 'NONE',  ( -4.842197138736131556, 5.678260079060780008, 1.199719254218452935 ) ) ;
#74197=CARTESIAN_POINT ( 'NONE',  ( 4.543390873910894356, 8.314723429622471684, 0.7216878364870317197 ) ) ;
#74203=CARTESIAN_POINT ( 'NONE',  ( -3.923105346307911745, 5.670318552149568703, -1.599625672291283607 ) ) ;
#74207=CARTESIAN_POINT ( 'NONE',  ( -6.699137298928187434, 8.909022496873262753, 1.443375672974064550 ) ) ;
#74210=CARTESIAN_POINT ( 'NONE',  ( -6.050681693448748177, 10.28115541899069463, 0.7998128361456291469 ) ) ;
#74214=CARTESIAN_POINT ( 'NONE',  ( -4.339491684825780737, 7.220434844675483355, -1.199719254218455378 ) ) ;
#74227=CARTESIAN_POINT ( 'NONE',  ( -5.695833931516914639, 6.778132687258748845, 1.082531754730549078 ) ) ;
#74229=CARTESIAN_POINT ( 'NONE',  ( -4.285785955251283141, 8.014184357852876417, 0.000000000000000000 ) ) ;
#74230=CARTESIAN_POINT ( 'NONE',  ( 6.170896192875352959, 7.228408975556602556, 1.199719254218453823 ) ) ;
#74232=CARTESIAN_POINT ( 'NONE',  ( -6.577640801285370209, 7.702944352034914566, -1.199719254218452047 ) ) ;
#74252=CARTESIAN_POINT ( 'NONE',  ( 7.038618024149998043, 8.240751112043669835, -1.199719254218452047 ) ) ;
#74258=CARTESIAN_POINT ( 'NONE',  ( -2.972099262745669712, 6.689475916503727859, 0.05200437644970179463 ) ) ;
#74287=CARTESIAN_POINT ( 'NONE',  ( 4.376249722160992839, 8.327651452488305850, 0.000000000000000000 ) ) ;
#74293=CARTESIAN_POINT ( 'NONE',  ( -5.112833325684904118, 8.979072956692109031, -0.7216878364870338292 ) ) ;
#74304=CARTESIAN_POINT ( 'NONE',  ( 5.643937085038755797, 9.806620042512378177, -0.7998128361456481317 ) ) ;
#74305=CARTESIAN_POINT ( 'NONE',  ( 6.215487077222150880, 6.216099443039444949, 0.000000000000000000 ) ) ;
#74317=CARTESIAN_POINT ( 'NONE',  ( 5.224688093219824303, 7.188831756880171397, -1.599625672291283607 ) ) ;
#74318=ORIENTED_EDGE ( 'NONE', *, *, #19773, .T. ) ;
#74328=CARTESIAN_POINT ( 'NONE',  ( 7.526184669361807522, 7.953172667109813077, 0.000000000000000000 ) ) ;
#74329=CARTESIAN_POINT ( 'NONE',  ( -5.478903473698268023, 5.564677938835638216, -0.7216878364870338292 ) ) ;
#74330=CARTESIAN_POINT ( 'NONE',  ( -7.422162748838431412, 7.623887726591770608, -0.7998128361456362523 ) ) ;
#74340=CARTESIAN_POINT ( 'NONE',  ( 5.345657705538078730, 9.458627433094950021, 0.7998128361456331437 ) ) ;
#74342=CARTESIAN_POINT ( 'NONE',  ( 6.717138760927786834, 6.801359740696030443, -0.7998128361456481317 ) ) ;
#74343=CARTESIAN_POINT ( 'NONE',  ( 6.688968683495743583, 8.897159112202094988, -1.599625672291283607 ) ) ;
#74346=CARTESIAN_POINT ( 'NONE',  ( 5.688527969385528849, 8.794310509995222347, -1.199719254218452047 ) ) ;
#74365=CARTESIAN_POINT ( 'NONE',  ( 5.923986774528332333, 5.876015756563318426, -0.7998128361456481317 ) ) ;
#74367=CARTESIAN_POINT ( 'NONE',  ( -3.923105346307911745, 5.670318552149568703, -1.599625672291283607 ) ) ;
#74370=CARTESIAN_POINT ( 'NONE',  ( 3.736153849017632922, 6.516540702899320081, -1.199719254218453823 ) ) ;
#74375=CARTESIAN_POINT ( 'NONE',  ( 8.018721507839716267, 8.319872945426633137, -0.7998128361456341429 ) ) ;
#74376=CARTESIAN_POINT ( 'NONE',  ( -5.608757509019071108, 5.629766575900002401, 7.500000000000000000 ) ) ;
#74379=CARTESIAN_POINT ( 'NONE',  ( 6.699137298928158124, 6.988284068270579574, 0.7216878364870328300 ) ) ;
#74382=CARTESIAN_POINT ( 'NONE',  ( -4.444040490229335560, 8.406740681901359480, 0.7998128361456352531 ) ) ;
#74384=CARTESIAN_POINT ( 'NONE',  ( 3.528865121306874464, 7.339036084825155015, -0.7998128361456362523 ) ) ;
#74391=CARTESIAN_POINT ( 'NONE',  ( -4.911143975938936812, 6.978132228647320190, -1.257868731225549208 ) ) ;
#74395=CARTESIAN_POINT ( 'NONE',  ( -4.228163802615396705, 6.026220084508304708, -1.599625672291271394 ) ) ;
#74400=ORIENTED_EDGE ( 'NONE', *, *, #81569, .T. ) ;
#74405=CARTESIAN_POINT ( 'NONE',  ( 0.3402877347799608265, 2.652045119545964891, -1.971798190796337336 ) ) ;
#74426=ORIENTED_EDGE ( 'NONE', *, *, #159272, .F. ) ;
#74430=CARTESIAN_POINT ( 'NONE',  ( 7.289443866002793371, 8.533381260871966134, 1.199719254218452047 ) ) ;
#74431=CARTESIAN_POINT ( 'NONE',  ( 5.207740400980577888, 5.248321020665011716, 0.000000000000000000 ) ) ;
#74442=CARTESIAN_POINT ( 'NONE',  ( -4.586401103172829785, 8.572828063668767484, 0.7998128361456281477 ) ) ;
#74444=CARTESIAN_POINT ( 'NONE',  ( 7.797347741190739256, 8.269529584243604958, 0.7216878364870267237 ) ) ;
#74453=CARTESIAN_POINT ( 'NONE',  ( -3.610214042988883598, 7.433943160120816351, 0.7998128361456352531 ) ) ;
#74460=ORIENTED_EDGE ( 'NONE', *, *, #50859, .T. ) ;
#74462=CARTESIAN_POINT ( 'NONE',  ( -4.659162064951642535, 5.464719159645540003, 1.199719254218452935 ) ) ;
#74485=CARTESIAN_POINT ( 'NONE',  ( -5.281783360975562225, 8.319775133516907673, 1.199719254218452935 ) ) ;
#74487=CARTESIAN_POINT ( 'NONE',  ( -2.993318053567081360, 6.714231172462041819, 0.000000000000000000 ) ) ;
#74512=CARTESIAN_POINT ( 'NONE',  ( -6.089547271193396227, 7.133501900260939443, -1.199719254218453823 ) ) ;
#74521=CARTESIAN_POINT ( 'NONE',  ( 7.146556367734764770, 9.431011410480991231, 1.443375672974063439 ) ) ;
#74529=CARTESIAN_POINT ( 'NONE',  ( -5.293380042321269130, 6.810232436340249329, 1.224475135354096800 ) ) ;
#74533=CARTESIAN_POINT ( 'NONE',  ( 5.747730777550676073, 5.670383760089384495, 0.000000000000000000 ) ) ;
#74541=CARTESIAN_POINT ( 'NONE',  ( 5.040599249230596435, 9.102725900736217568, 0.7998128361456341429 ) ) ;
#74543=CARTESIAN_POINT ( 'NONE',  ( 5.855142236255289845, 7.924361590421551860, -1.599625672291281386 ) ) ;
#74555=CARTESIAN_POINT ( 'NONE',  ( 6.479309170914094196, 6.755949689298615723, 0.1985876171829506487 ) ) ;
#74557=CARTESIAN_POINT ( 'NONE',  ( 5.777182853198898904, 6.873039762554409293, -1.082531754730548412 ) ) ;
#74566=CARTESIAN_POINT ( 'NONE',  ( -5.334207092333882017, 5.187939460669764635, 0.7998128361456281477 ) ) ;
#74574=CARTESIAN_POINT ( 'NONE',  ( -5.600926855776888758, 7.627776979863398310, -1.443375672974066548 ) ) ;
#74577=CARTESIAN_POINT ( 'NONE',  ( 5.820193082016415609, 10.01225203898631655, 0.000000000000000000 ) ) ;
#74578=EDGE_CURVE ( 'NONE', #199345, #7836, #31978, .T. ) ;
#74594=CARTESIAN_POINT ( 'NONE',  ( 5.936491157937257235, 8.019268665717216749, 1.599625672291268286 ) ) ;
#74611=CARTESIAN_POINT ( 'NONE',  ( -7.422162748838431412, 7.623887726591770608, -0.7998128361456362523 ) ) ;
#74632=CARTESIAN_POINT ( 'NONE',  ( 3.719872605471109761, 6.605953636083950364, -2.420000000000002149 ) ) ;
#74633=CARTESIAN_POINT ( 'NONE',  ( 4.570507181582611267, 8.346359121906111511, 0.000000000000000000 ) ) ;
#74645=CARTESIAN_POINT ( 'NONE',  ( -4.909461021924285795, 6.821066840368686712, 1.443375672974058777 ) ) ;
#74649=DIRECTION ( 'NONE',  ( -0.6507913734559641616, -0.7592566023653004592, 0.000000000000000000 ) ) ;
#74676=CARTESIAN_POINT ( 'NONE',  ( 4.686278372178935392, 5.496354851410763409, 1.199719254218452047 ) ) ;
#74689=CARTESIAN_POINT ( 'NONE',  ( -7.119440060951841787, 7.478637290631501067, 0.000000000000000000 ) ) ;
#74691=CARTESIAN_POINT ( 'NONE',  ( 7.095713291905693332, 9.371694488680407886, 1.599625672291268286 ) ) ;
#74711=CARTESIAN_POINT ( 'NONE',  ( 4.706088717274896638, 7.544168365912456764, 1.082531754730548412 ) ) ;
#74712=CARTESIAN_POINT ( 'NONE',  ( 3.913815762669449416, 7.330443837381343641, -0.8582294057540799104 ) ) ;
#74713=DIRECTION ( 'NONE',  ( 1.000000000000000000, 0.000000000000000000, 0.000000000000000000 ) ) ;
#74739=CARTESIAN_POINT ( 'NONE',  ( -5.433785704026946384, 9.561443431331920095, 0.000000000000000000 ) ) ;
#74741=( BOUNDED_SURFACE ( )  B_SPLINE_SURFACE ( 1, 2, ( 
 ( #85360, #52861, #151442, #150376, #3013, #53935, #86432, #100541, #1946, #70151, #83210, #84290, #49659, #200156, #117928, #82147, #136262, #69083, #118994, #199079, #120071, #201220, #184973, #36598, #149293, #33404, #186047, #102685, #168743, #20346, #116850, #17134, #202282, #115782, #103759, #37682, #165541, #181771, #16063, #148239, #214241, #65871, #198030, #874, #122227, #189262, #104833, #137334, #89652, #203351, #153572, #173031, #107006, #57132, #5142, #55003, #157849, #75514, #38752, #74453, #21398, #121154, #191377, #108083, #140557, #125411, #24613, #174112, #170878, #188187, #39822, #90722, #73365, #8370, #87508, #139470, #23543, #187119, #156784, #206571, #25684, #205499, #124356, #123299, #88581, #40901, #43043, #6220, #154639, #22470, #207635, #58198, #190314, #41972, #72289, #138397, #204415, #56071, #169808, #59253, #105930, #171954, #91793, #9443, #155706, #71217, #7287, #141625, #61399, #128624, #44100, #76572, #28905, #142684, #92856, #112352, #46235, #210835, #158902, #208694, #97125, #14762, #192445, #13700, #175168, #60321, #130737, #47308, #79774, #64596, #178365, #113422, #110220, #127562, #193530, #29973, #12631, #162111, #26755, #78702, #177291, #126481, #96058, #145886, #179428, #144828, #63534, #62462, #27830, #194591, #196730, #159967, #109156, #10499, #111285, #211897, #176227, #93926, #129689, #94990, #195672, #31049, #163177, #11572, #80852, #146943, #212958, #77642, #143764, #209758, #45173, #161036, #2757, #184716, #66680, #131774, #149037, #183668, #69887, #48370, #17944, #19020, #198831, #115535, #67747, #36340, #3816, #1693, #200955, #151185, #86173, #167428, #199904, #85100, #133897, #182591, #117674, #152243, #118732, #132827, #34214, #102418, #181530, #50476, #81905, #100287, #150120, #114483, #168486, #116597, #68826, #165288, #136000, #612, #134948, #166354, #197777, #15820, #84031, #147993, #32099, #51550, #35271, #101349, #98184, #214003, #20085, #180480, #49415, #52603, #164232, #65624, #33158, #99239, #16882, #82963, #139203, #140297, #137068, #5956, #154379 ),
 ( #121958, #72027, #24348, #74203, #186862, #156524, #203093, #105656, #55804, #202013, #187925, #138139, #54738, #204148, #107830, #120888, #38492, #39555, #171684, #21136, #104570, #23281, #206316, #90458, #91537, #89393, #119804, #57940, #155441, #103493, #4879, #87239, #7026, #169554, #73102, #25431, #123050, #170615, #22202, #205233, #56874, #53672, #173855, #153304, #189001, #88315, #40644, #106747, #172774, #8115, #124105, #190068, #41720, #157596, #9191, #75262, #185783, #37417, #70958, #44920, #144574, #42789, #10249, #45984, #111028, #177033, #94737, #160783, #174921, #12376, #192190, #175979, #29724, #26501, #63277, #76325, #142431, #77389, #109968, #195422, #194343, #13452, #28650, #126229, #128375, #30796, #210588, #208439, #62218, #141376, #92608, #158651, #145646, #60073, #143505, #209502, #78456, #43854, #108898, #61142, #27572, #125164, #112105, #178108, #95806, #191123, #93670, #129439, #47052, #159713, #161862, #207387, #11311, #162925, #79528, #211642, #96875, #113168, #179172, #127304, #193275, #14506, #59008, #198581, #136553, #212709, #53154, #148793, #180235, #86718, #152787, #87789, #119283, #37974, #185269, #213757, #36892, #105126, #131526, #171166, #196483, #82716, #102974, #80597, #146693, #4367, #363, #54226, #169032, #120364, #130496, #186339, #20629, #70437, #170093, #202574, #39041, #81654, #181282, #104047, #5432, #98986, #163992, #32908, #21679, #64350, #48125, #153863, #71511, #16632, #147741, #137623, #203640, #114237, #55291, #121441, #187410, #31859, #97934, #15567, #65380, #197529, #66436, #49174, #115291, #165039, #132578, #8660, #159181, #89943, #107301, #56356, #74739, #124644, #88873, #93144, #24903, #125703, #139765, #60613, #189546, #191662, #41194, #155994, #40112, #126772, #42259, #75802, #206856, #205791, #23836, #57421, #122519, #110506, #192730, #106223, #188482, #207922, #141910, #123583, #22755, #154927, #190601, #173325, #140844, #6512, #142976, #204706, #25973, #91009, #58488, #157071, #108372, #73666, #174395, #10782, #92079, #158136, #9727, #59543, #43326 ) ),
 .UNSPECIFIED., .F., .F., .F. ) 
 B_SPLINE_SURFACE_WITH_KNOTS ( ( 2, 2 ),
 ( 3, 2, 2, 2, 2, 2, 2, 2, 2, 2, 2, 2, 2, 2, 2, 2, 2, 2, 2, 2, 2, 2, 2, 2, 2, 2, 2, 2, 2, 2, 2, 2, 2, 2, 2, 2, 2, 2, 2, 2, 2, 2, 2, 2, 2, 2, 2, 2, 2, 2, 2, 2, 2, 2, 2, 2, 2, 2, 2, 2, 2, 2, 2, 2, 2, 2, 2, 2, 2, 2, 2, 2, 2, 2, 2, 2, 2, 2, 2, 2, 2, 2, 2, 2, 2, 2, 2, 2, 2, 2, 2, 2, 2, 2, 2, 2, 2, 2, 2, 2, 2, 2, 2, 2, 2, 2, 2, 2, 2, 2, 2, 2, 2, 2, 2, 2, 2, 2, 2, 2, 3 ),
 ( 0.000000000000000000, 1.000000000000000000 ),
 ( 0.000000000000000000, 0.008333333333333333218, 0.01666666666666666644, 0.02500000000000000139, 0.03333333333333333287, 0.04166666666666666435, 0.05000000000000000278, 0.05833333333333333426, 0.06666666666666666574, 0.07499999999999999722, 0.08333333333333332871, 0.09166666666666666019, 0.1000000000000000056, 0.1083333333333333370, 0.1166666666666666685, 0.1250000000000000000, 0.1333333333333333315, 0.1416666666666666630, 0.1499999999999999944, 0.1583333333333333259, 0.1666666666666666574, 0.1749999999999999889, 0.1833333333333333204, 0.1916666666666666796, 0.2000000000000000111, 0.2083333333333333426, 0.2166666666666666741, 0.2250000000000000056, 0.2333333333333333370, 0.2416666666666666685, 0.2500000000000000000, 0.2583333333333333592, 0.2666666666666666630, 0.2750000000000000222, 0.2833333333333333259, 0.2916666666666666852, 0.2999999999999999889, 0.3083333333333333481, 0.3166666666666666519, 0.3250000000000000111, 0.3333333333333333148, 0.3416666666666666741, 0.3499999999999999778, 0.3583333333333333370, 0.3666666666666666408, 0.3750000000000000000, 0.3833333333333333592, 0.3916666666666666630, 0.4000000000000000222, 0.4083333333333333259, 0.4166666666666666852, 0.4249999999999999889, 0.4333333333333333481, 0.4416666666666666519, 0.4500000000000000111, 0.4583333333333333148, 0.4666666666666666741, 0.4749999999999999778, 0.4833333333333333370, 0.4916666666666666408, 0.5000000000000000000, 0.5083333333333333037, 0.5166666666666667185, 0.5250000000000000222, 0.5333333333333333259, 0.5416666666666666297, 0.5500000000000000444, 0.5583333333333333481, 0.5666666666666666519, 0.5749999999999999556, 0.5833333333333333703, 0.5916666666666666741, 0.5999999999999999778, 0.6083333333333332815, 0.6166666666666666963, 0.6250000000000000000, 0.6333333333333333037, 0.6416666666666667185, 0.6500000000000000222, 0.6583333333333333259, 0.6666666666666666297, 0.6750000000000000444, 0.6833333333333333481, 0.6916666666666666519, 0.6999999999999999556, 0.7083333333333333703, 0.7166666666666666741, 0.7249999999999999778, 0.7333333333333332815, 0.7416666666666666963, 0.7500000000000000000, 0.7583333333333333037, 0.7666666666666667185, 0.7750000000000000222, 0.7833333333333333259, 0.7916666666666666297, 0.8000000000000000444, 0.8083333333333333481, 0.8166666666666666519, 0.8249999999999999556, 0.8333333333333333703, 0.8416666666666666741, 0.8499999999999999778, 0.8583333333333332815, 0.8666666666666666963, 0.8750000000000000000, 0.8833333333333333037, 0.8916666666666667185, 0.9000000000000000222, 0.9083333333333333259, 0.9166666666666666297, 0.9250000000000000444, 0.9333333333333333481, 0.9416666666666666519, 0.9499999999999999556, 0.9583333333333333703, 0.9666666666666666741, 0.9749999999999999778, 0.9833333333333332815, 0.9916666666666666963, 1.000000000000000000 ),
 .UNSPECIFIED. ) 
 GEOMETRIC_REPRESENTATION_ITEM ( )  RATIONAL_B_SPLINE_SURFACE ( (
 ( 1.000000000000000000, 0.8660254037844387076, 1.000000000000000000, 0.8660254037844387076, 1.000000000000000000, 0.8660254037844387076, 1.000000000000000000, 0.8660254037844387076, 1.000000000000000000, 0.8660254037844387076, 1.000000000000000000, 0.8660254037844387076, 1.000000000000000000, 0.8660254037844387076, 1.000000000000000000, 0.8660254037844387076, 1.000000000000000000, 0.8660254037844387076, 1.000000000000000000, 0.8660254037844387076, 1.000000000000000000, 0.8660254037844387076, 1.000000000000000000, 0.8660254037844387076, 1.000000000000000000, 0.8660254037844387076, 1.000000000000000000, 0.8660254037844387076, 1.000000000000000000, 0.8660254037844387076, 1.000000000000000000, 0.8660254037844387076, 1.000000000000000000, 0.8660254037844387076, 1.000000000000000000, 0.8660254037844387076, 1.000000000000000000, 0.8660254037844387076, 1.000000000000000000, 0.8660254037844387076, 1.000000000000000000, 0.8660254037844387076, 1.000000000000000000, 0.8660254037844387076, 1.000000000000000000, 0.8660254037844387076, 1.000000000000000000, 0.8660254037844387076, 1.000000000000000000, 0.8660254037844387076, 1.000000000000000000, 0.8660254037844387076, 1.000000000000000000, 0.8660254037844387076, 1.000000000000000000, 0.8660254037844387076, 1.000000000000000000, 0.8660254037844387076, 1.000000000000000000, 0.8660254037844387076, 1.000000000000000000, 0.8660254037844387076, 1.000000000000000000, 0.8660254037844387076, 1.000000000000000000, 0.8660254037844387076, 1.000000000000000000, 0.8660254037844387076, 1.000000000000000000, 0.8660254037844387076, 1.000000000000000000, 0.8660254037844387076, 1.000000000000000000, 0.8660254037844387076, 1.000000000000000000, 0.8660254037844387076, 1.000000000000000000, 0.8660254037844387076, 1.000000000000000000, 0.8660254037844387076, 1.000000000000000000, 0.8660254037844387076, 1.000000000000000000, 0.8660254037844387076, 1.000000000000000000, 0.8660254037844387076, 1.000000000000000000, 0.8660254037844387076, 1.000000000000000000, 0.8660254037844387076, 1.000000000000000000, 0.8660254037844387076, 1.000000000000000000, 0.8660254037844387076, 1.000000000000000000, 0.8660254037844387076, 1.000000000000000000, 0.8660254037844387076, 1.000000000000000000, 0.8660254037844387076, 1.000000000000000000, 0.8660254037844387076, 1.000000000000000000, 0.8660254037844387076, 1.000000000000000000, 0.8660254037844387076, 1.000000000000000000, 0.8660254037844387076, 1.000000000000000000, 0.8660254037844387076, 1.000000000000000000, 0.8660254037844387076, 1.000000000000000000, 0.8660254037844387076, 1.000000000000000000, 0.8660254037844387076, 1.000000000000000000, 0.8660254037844387076, 1.000000000000000000, 0.8660254037844387076, 1.000000000000000000, 0.8660254037844387076, 1.000000000000000000, 0.8660254037844387076, 1.000000000000000000, 0.8660254037844387076, 1.000000000000000000, 0.8660254037844387076, 1.000000000000000000, 0.8660254037844387076, 1.000000000000000000, 0.8660254037844387076, 1.000000000000000000, 0.8660254037844387076, 1.000000000000000000, 0.8660254037844387076, 1.000000000000000000, 0.8660254037844387076, 1.000000000000000000, 0.8660254037844387076, 1.000000000000000000, 0.8660254037844387076, 1.000000000000000000, 0.8660254037844387076, 1.000000000000000000, 0.8660254037844387076, 1.000000000000000000, 0.8660254037844387076, 1.000000000000000000, 0.8660254037844387076, 1.000000000000000000, 0.8660254037844387076, 1.000000000000000000, 0.8660254037844387076, 1.000000000000000000, 0.8660254037844387076, 1.000000000000000000, 0.8660254037844387076, 1.000000000000000000, 0.8660254037844387076, 1.000000000000000000, 0.8660254037844387076, 1.000000000000000000, 0.8660254037844387076, 1.000000000000000000, 0.8660254037844387076, 1.000000000000000000, 0.8660254037844387076, 1.000000000000000000, 0.8660254037844387076, 1.000000000000000000, 0.8660254037844387076, 1.000000000000000000, 0.8660254037844387076, 1.000000000000000000, 0.8660254037844387076, 1.000000000000000000, 0.8660254037844387076, 1.000000000000000000, 0.8660254037844387076, 1.000000000000000000, 0.8660254037844387076, 1.000000000000000000, 0.8660254037844387076, 1.000000000000000000, 0.8660254037844387076, 1.000000000000000000, 0.8660254037844387076, 1.000000000000000000, 0.8660254037844387076, 1.000000000000000000, 0.8660254037844387076, 1.000000000000000000, 0.8660254037844387076, 1.000000000000000000, 0.8660254037844387076, 1.000000000000000000, 0.8660254037844387076, 1.000000000000000000, 0.8660254037844387076, 1.000000000000000000, 0.8660254037844387076, 1.000000000000000000, 0.8660254037844387076, 1.000000000000000000, 0.8660254037844387076, 1.000000000000000000, 0.8660254037844387076, 1.000000000000000000, 0.8660254037844387076, 1.000000000000000000, 0.8660254037844387076, 1.000000000000000000, 0.8660254037844387076, 1.000000000000000000, 0.8660254037844387076, 1.000000000000000000, 0.8660254037844387076, 1.000000000000000000, 0.8660254037844387076, 1.000000000000000000, 0.8660254037844387076, 1.000000000000000000, 0.8660254037844387076, 1.000000000000000000, 0.8660254037844387076, 1.000000000000000000, 0.8660254037844387076, 1.000000000000000000, 0.8660254037844387076, 1.000000000000000000, 0.8660254037844387076, 1.000000000000000000, 0.8660254037844387076, 1.000000000000000000, 0.8660254037844387076, 1.000000000000000000, 0.8660254037844387076, 1.000000000000000000, 0.8660254037844387076, 1.000000000000000000),
 ( 1.000000000000000000, 0.8660254037844387076, 1.000000000000000000, 0.8660254037844387076, 1.000000000000000000, 0.8660254037844387076, 1.000000000000000000, 0.8660254037844387076, 1.000000000000000000, 0.8660254037844387076, 1.000000000000000000, 0.8660254037844387076, 1.000000000000000000, 0.8660254037844387076, 1.000000000000000000, 0.8660254037844387076, 1.000000000000000000, 0.8660254037844387076, 1.000000000000000000, 0.8660254037844387076, 1.000000000000000000, 0.8660254037844387076, 1.000000000000000000, 0.8660254037844387076, 1.000000000000000000, 0.8660254037844387076, 1.000000000000000000, 0.8660254037844387076, 1.000000000000000000, 0.8660254037844387076, 1.000000000000000000, 0.8660254037844387076, 1.000000000000000000, 0.8660254037844387076, 1.000000000000000000, 0.8660254037844387076, 1.000000000000000000, 0.8660254037844387076, 1.000000000000000000, 0.8660254037844387076, 1.000000000000000000, 0.8660254037844387076, 1.000000000000000000, 0.8660254037844387076, 1.000000000000000000, 0.8660254037844387076, 1.000000000000000000, 0.8660254037844387076, 1.000000000000000000, 0.8660254037844387076, 1.000000000000000000, 0.8660254037844387076, 1.000000000000000000, 0.8660254037844387076, 1.000000000000000000, 0.8660254037844387076, 1.000000000000000000, 0.8660254037844387076, 1.000000000000000000, 0.8660254037844387076, 1.000000000000000000, 0.8660254037844387076, 1.000000000000000000, 0.8660254037844387076, 1.000000000000000000, 0.8660254037844387076, 1.000000000000000000, 0.8660254037844387076, 1.000000000000000000, 0.8660254037844387076, 1.000000000000000000, 0.8660254037844387076, 1.000000000000000000, 0.8660254037844387076, 1.000000000000000000, 0.8660254037844387076, 1.000000000000000000, 0.8660254037844387076, 1.000000000000000000, 0.8660254037844387076, 1.000000000000000000, 0.8660254037844387076, 1.000000000000000000, 0.8660254037844387076, 1.000000000000000000, 0.8660254037844387076, 1.000000000000000000, 0.8660254037844387076, 1.000000000000000000, 0.8660254037844387076, 1.000000000000000000, 0.8660254037844387076, 1.000000000000000000, 0.8660254037844387076, 1.000000000000000000, 0.8660254037844387076, 1.000000000000000000, 0.8660254037844387076, 1.000000000000000000, 0.8660254037844387076, 1.000000000000000000, 0.8660254037844387076, 1.000000000000000000, 0.8660254037844387076, 1.000000000000000000, 0.8660254037844387076, 1.000000000000000000, 0.8660254037844387076, 1.000000000000000000, 0.8660254037844387076, 1.000000000000000000, 0.8660254037844387076, 1.000000000000000000, 0.8660254037844387076, 1.000000000000000000, 0.8660254037844387076, 1.000000000000000000, 0.8660254037844387076, 1.000000000000000000, 0.8660254037844387076, 1.000000000000000000, 0.8660254037844387076, 1.000000000000000000, 0.8660254037844387076, 1.000000000000000000, 0.8660254037844387076, 1.000000000000000000, 0.8660254037844387076, 1.000000000000000000, 0.8660254037844387076, 1.000000000000000000, 0.8660254037844387076, 1.000000000000000000, 0.8660254037844387076, 1.000000000000000000, 0.8660254037844387076, 1.000000000000000000, 0.8660254037844387076, 1.000000000000000000, 0.8660254037844387076, 1.000000000000000000, 0.8660254037844387076, 1.000000000000000000, 0.8660254037844387076, 1.000000000000000000, 0.8660254037844387076, 1.000000000000000000, 0.8660254037844387076, 1.000000000000000000, 0.8660254037844387076, 1.000000000000000000, 0.8660254037844387076, 1.000000000000000000, 0.8660254037844387076, 1.000000000000000000, 0.8660254037844387076, 1.000000000000000000, 0.8660254037844387076, 1.000000000000000000, 0.8660254037844387076, 1.000000000000000000, 0.8660254037844387076, 1.000000000000000000, 0.8660254037844387076, 1.000000000000000000, 0.8660254037844387076, 1.000000000000000000, 0.8660254037844387076, 1.000000000000000000, 0.8660254037844387076, 1.000000000000000000, 0.8660254037844387076, 1.000000000000000000, 0.8660254037844387076, 1.000000000000000000, 0.8660254037844387076, 1.000000000000000000, 0.8660254037844387076, 1.000000000000000000, 0.8660254037844387076, 1.000000000000000000, 0.8660254037844387076, 1.000000000000000000, 0.8660254037844387076, 1.000000000000000000, 0.8660254037844387076, 1.000000000000000000, 0.8660254037844387076, 1.000000000000000000, 0.8660254037844387076, 1.000000000000000000, 0.8660254037844387076, 1.000000000000000000, 0.8660254037844387076, 1.000000000000000000, 0.8660254037844387076, 1.000000000000000000, 0.8660254037844387076, 1.000000000000000000, 0.8660254037844387076, 1.000000000000000000, 0.8660254037844387076, 1.000000000000000000, 0.8660254037844387076, 1.000000000000000000, 0.8660254037844387076, 1.000000000000000000, 0.8660254037844387076, 1.000000000000000000, 0.8660254037844387076, 1.000000000000000000, 0.8660254037844387076, 1.000000000000000000, 0.8660254037844387076, 1.000000000000000000, 0.8660254037844387076, 1.000000000000000000, 0.8660254037844387076, 1.000000000000000000, 0.8660254037844387076, 1.000000000000000000, 0.8660254037844387076, 1.000000000000000000, 0.8660254037844387076, 1.000000000000000000, 0.8660254037844387076, 1.000000000000000000, 0.8660254037844387076, 1.000000000000000000, 0.8660254037844387076, 1.000000000000000000, 0.8660254037844387076, 1.000000000000000000, 0.8660254037844387076, 1.000000000000000000, 0.8660254037844387076, 1.000000000000000000, 0.8660254037844387076, 1.000000000000000000, 0.8660254037844387076, 1.000000000000000000) ) ) 
 REPRESENTATION_ITEM ( '' )  SURFACE ( )  );
#74743=CARTESIAN_POINT ( 'NONE',  ( -4.762657100150483380, 8.778460060142702304, 0.000000000000000000 ) ) ;
#74749=CARTESIAN_POINT ( 'NONE',  ( -5.275531169048895741, 9.168887107283438809, -0.7216878364870338292 ) ) ;
#74751=CARTESIAN_POINT ( 'NONE',  ( 6.495764994278795612, 9.632124022417032805, 1.082531754730549078 ) ) ;
#74753=CARTESIAN_POINT ( 'NONE',  ( -4.085803189671902480, 5.860132702740892263, -1.599625672291271394 ) ) ;
#74756=CARTESIAN_POINT ( 'NONE',  ( -2.979759899953417612, 6.698413326579433225, 0.7998128361456352531 ) ) ;
#74764=CARTESIAN_POINT ( 'NONE',  ( -7.065734331377342414, 8.272386803808890576, -1.199719254218452047 ) ) ;
#74766=CARTESIAN_POINT ( 'NONE',  ( 5.599868899865946936, 7.382462344760764239, -1.240035354157904779 ) ) ;
#74770=CARTESIAN_POINT ( 'NONE',  ( 3.736153849017632922, 6.516540702899320081, -1.199719254218453823 ) ) ;
#74786=CARTESIAN_POINT ( 'NONE',  ( 2.943528747942701695, 6.448217615992859919, 0.000000000000000000 ) ) ;
#74796=CARTESIAN_POINT ( 'NONE',  ( 6.668631453075247073, 8.873432343378178544, -1.599625672291281386 ) ) ;
#74807=CARTESIAN_POINT ( 'NONE',  ( 0.4396062811529514169, 3.163270344466244666, 1.951136887981155033 ) ) ;
#74811=CARTESIAN_POINT ( 'NONE',  ( 6.454463653088309272, 6.866155873091829953, 0.6733577401037347254 ) ) ;
#74812=CARTESIAN_POINT ( 'NONE',  ( -4.136646265500958819, 7.840188053144158786, -0.7216878364870458196 ) ) ;
#74835=CARTESIAN_POINT ( 'NONE',  ( -0.1380770317961217131, 2.619511416136325987, -2.074674745642052898 ) ) ;
#74841=CARTESIAN_POINT ( 'NONE',  ( 4.577813143269636065, 5.369812084349879555, -1.199719254218450271 ) ) ;
#74860=CARTESIAN_POINT ( 'NONE',  ( -7.144220599758281054, 7.299621885998258897, 0.7998128361456341429 ) ) ;
#74873=CARTESIAN_POINT ( 'NONE',  ( 5.032011289327418702, 5.899709921417326974, 1.199719254218452935 ) ) ;
#74884=CARTESIAN_POINT ( 'NONE',  ( 5.975194856099406593, 7.098212677808693805, 1.080521340106417982 ) ) ;
#74901=AXIS2_PLACEMENT_3D ( 'NONE', #90064, #7708, #73791 ) ;
#74904=CARTESIAN_POINT ( 'NONE',  ( -5.492988512192097161, 6.437516681426083132, 1.199719254218452935 ) ) ;
#74906=CARTESIAN_POINT ( 'NONE',  ( 3.562760505341037831, 7.378580699531681830, -1.734723475976807094E-15 ) ) ;
#74909=CARTESIAN_POINT ( 'NONE',  ( -4.925354943514475003, 8.968274210734028529, 0.000000000000000000 ) ) ;
#74911=CARTESIAN_POINT ( 'NONE',  ( 3.036575945257459885, 6.282152860354720758, -0.6783893874775955846 ) ) ;
#74917=CARTESIAN_POINT ( 'NONE',  ( -4.612885993627734216, 8.463679738117141582, -0.3448095128447264957 ) ) ;
#74924=CARTESIAN_POINT ( 'NONE',  ( -4.245111494410291897, 7.006361605903701495, 1.082531754730549967 ) ) ;
#74934=CARTESIAN_POINT ( 'NONE',  ( 5.153507786970260796, 7.105788066255672497, -1.443375672974078761 ) ) ;
#74938=CARTESIAN_POINT ( 'NONE',  ( -6.936931872047518155, 8.122117267924091166, 1.199719254218452047 ) ) ;
#74952=CARTESIAN_POINT ( 'NONE',  ( 5.571474780572990504, 5.464751763615448787, 0.7998128361456352531 ) ) ;
#74980=CARTESIAN_POINT ( 'NONE',  ( -5.126391479742927970, 8.994890803093138487, 0.7216878364870267237 ) ) ;
#74983=ORIENTED_EDGE ( 'NONE', *, *, #105361, .F. ) ;
#75006=CARTESIAN_POINT ( 'NONE',  ( -6.071018923869249129, 10.30488218781460574, 0.7998128361456291469 ) ) ;
#75011=CARTESIAN_POINT ( 'NONE',  ( -5.147255595043616516, 6.034161611419515125, 1.199719254218452935 ) ) ;
#75020=CARTESIAN_POINT ( 'NONE',  ( -5.354544322754380303, 5.211666229493680191, 0.7998128361456281477 ) ) ;
#75022=CARTESIAN_POINT ( 'NONE',  ( 6.567098404289990476, 6.791591158854626720, -0.3517435911668670423 ) ) ;
#75026=CARTESIAN_POINT ( 'NONE',  ( 4.390861645979372341, 6.216034235099629157, -1.599625672291269396 ) ) ;
#75030=CARTESIAN_POINT ( 'NONE',  ( -5.354544322754380303, 5.211666229493680191, 0.7998128361456281477 ) ) ;
#75032=VERTEX_POINT ( 'NONE', #199206 ) ;
#75034=CARTESIAN_POINT ( 'NONE',  ( -3.610214042988883598, 7.433943160120816351, 0.7998128361456352531 ) ) ;
#75039=CARTESIAN_POINT ( 'NONE',  ( 4.814553946184248368, 7.670711132973337065, -1.082531754730548412 ) ) ;
#75040=CARTESIAN_POINT ( 'NONE',  ( -5.329763783503577379, 6.351050847909847086, 1.082531754730549078 ) ) ;
#75044=CARTESIAN_POINT ( 'NONE',  ( -4.111865726694519552, 8.019203457777400956, 0.000000000000000000 ) ) ;
#75047=CARTESIAN_POINT ( 'NONE',  ( 5.415556014015861841, 5.282846535965431300, -0.7998128361456481317 ) ) ;
#75051=CARTESIAN_POINT ( 'NONE',  ( -4.489185348024023803, 8.251483745236578571, -0.001312355330887114441 ) ) ;
#75055=CIRCLE ( 'NONE', #74901, 0.07999999999999998779 ) ;
#75056=CARTESIAN_POINT ( 'NONE',  ( 5.876533236880477240, 5.820653295974182129, 0.7998128361456350310 ) ) ;
#75059=CARTESIAN_POINT ( 'NONE',  ( 5.084740326411086642, 7.951855545768795608, 1.193092838546747414 ) ) ;
#75068=CARTESIAN_POINT ( 'NONE',  ( 6.225128807330042591, 7.291680359087043151, -1.199719254218452047 ) ) ;
#75078=CARTESIAN_POINT ( 'NONE',  ( 4.855733865602142707, 8.067643820953190215, 0.9155131637919884380 ) ) ;
#75085=CARTESIAN_POINT ( 'NONE',  ( 6.099189001301251523, 8.209082816308541197, 1.599625672291268286 ) ) ;
#75086=AXIS2_PLACEMENT_3D ( 'NONE', #209757, #97123, #14761 ) ;
#75090=CARTESIAN_POINT ( 'NONE',  ( -4.719039639065737646, 8.241789607316443167, 0.6479098462880685805 ) ) ;
#75099=CARTESIAN_POINT ( 'NONE',  ( -7.944151662964566540, 8.232874793072271657, 0.000000000000000000 ) ) ;
#75112=CARTESIAN_POINT ( 'NONE',  ( 5.176180785367283654, 9.260904359562321275, -0.7998128361456481317 ) ) ;
#75116=CARTESIAN_POINT ( 'NONE',  ( -4.081922216054144847, 7.264673858714298937, 0.8994561575802516584 ) ) ;
#75117=VERTEX_POINT ( 'NONE', #119239 ) ;
#75120=CARTESIAN_POINT ( 'NONE',  ( -7.892254816486440561, 8.380254505421877553, 0.000000000000000000 ) ) ;
#75122=CARTESIAN_POINT ( 'NONE',  ( 4.848976215542928792, 5.686169002002086970, 1.199719254218452047 ) ) ;
#75125=CARTESIAN_POINT ( 'NONE',  ( 5.031484404002891431, 5.042689024191078673, 0.7216878364870328300 ) ) ;
#75140=CARTESIAN_POINT ( 'NONE',  ( -3.786470039966538970, 7.639575156594750283, 0.000000000000000000 ) ) ;
#75141=CARTESIAN_POINT ( 'NONE',  ( 2.878073747850912412, 6.579779482459851003, -0.7998128361456362523 ) ) ;
#75153=CARTESIAN_POINT ( 'NONE',  ( -6.635789839245807897, 6.706452665400368218, 0.7998128361456341429 ) ) ;
#75154=CARTESIAN_POINT ( 'NONE',  ( -5.632486471834530661, 5.535932070087196344, -0.7998128361456362523 ) ) ;
#75156=CARTESIAN_POINT ( 'NONE',  ( 7.634649897826744080, 9.040084647953621655, 1.082531754730549078 ) ) ;
#75162=CARTESIAN_POINT ( 'NONE',  ( -7.065207446497166366, 9.336104335703744539, 0.000000000000000000 ) ) ;
#75169=CARTESIAN_POINT ( 'NONE',  ( -5.872679487624441030, 7.188158700483015195, -1.149102218512105145 ) ) ;
#75173=CARTESIAN_POINT ( 'NONE',  ( 4.879147978569815969, 4.879180288469956217, -0.1512534140984626019 ) ) ;
#75174=CARTESIAN_POINT ( 'NONE',  ( 4.340018570150304456, 6.156717313299049366, -1.443375672974068769 ) ) ;
#75178=CARTESIAN_POINT ( 'NONE',  ( -6.469175572376043348, 7.576401584974034265, 1.199719254218452047 ) ) ;
#75191=CARTESIAN_POINT ( 'NONE',  ( 5.692444392891300886, 7.734547439830227411, -1.599625672291281386 ) ) ;
#75208=CARTESIAN_POINT ( 'NONE',  ( 2.970662972610667918, 6.571530881558488524, 0.4515752934304059218 ) ) ;
#75225=ADVANCED_FACE ( 'NONE', ( #105084 ), #26993, .F. ) ;
#75227=CARTESIAN_POINT ( 'NONE',  ( 7.051649292883499953, 7.399548061218447437, -0.7216878364870317197 ) ) ;
#75232=CARTESIAN_POINT ( 'NONE',  ( 5.682275777458829502, 9.643422483761748154, 0.7216878364870317197 ) ) ;
#75254=CARTESIAN_POINT ( 'NONE',  ( -3.817502770699643388, 6.611447778194983194, 1.199719254218452935 ) ) ;
#75256=CARTESIAN_POINT ( 'NONE',  ( 4.977251789548238214, 7.860525283564661514, -1.082531754730548412 ) ) ;
#75262=CARTESIAN_POINT ( 'NONE',  ( -5.679940009482361774, 5.591294530676332641, 0.7998128361456281477 ) ) ;
#75267=CARTESIAN_POINT ( 'NONE',  ( -3.284818356260900796, 7.054314858938165678, 0.7998128361456352531 ) ) ;
#75268=AXIS2_PLACEMENT_3D ( 'NONE', #76914, #192791, #206918 ) ;
#75275=CARTESIAN_POINT ( 'NONE',  ( -5.309953438407606363, 6.223975762010839574, 1.199719254218452935 ) ) ;
#75284=CARTESIAN_POINT ( 'NONE',  ( -4.065465959251405081, 5.836405933916976707, -1.599625672291271394 ) ) ;
#75287=CARTESIAN_POINT ( 'NONE',  ( -4.177320726786319049, 6.927272377009067839, -1.082531754730551743 ) ) ;
#75289=CARTESIAN_POINT ( 'NONE',  ( -4.611181641979265500, 8.393812659035525314, 0.000000000000000000 ) ) ;
#75290=CARTESIAN_POINT ( 'NONE',  ( 6.119526231721748033, 8.232809585132461194, 1.599625672291269396 ) ) ;
#75291=CARTESIAN_POINT ( 'NONE',  ( -5.956828388357799042, 8.042995434541133193, 1.599625672291263179 ) ) ;
#75311=CARTESIAN_POINT ( 'NONE',  ( 6.688968683495743583, 8.897159112202094988, -1.599625672291283607 ) ) ;
#75330=CARTESIAN_POINT ( 'NONE',  ( 5.088145468715395303, 7.830155539619080507, -1.136959649167136543 ) ) ;
#75335=FACE_OUTER_BOUND ( 'NONE', #156752, .T. ) ;
#75348=CARTESIAN_POINT ( 'NONE',  ( 6.873057527484919937, 6.983264968346048818, 0.7998128361456352531 ) ) ;
#75351=( BOUNDED_SURFACE ( )  B_SPLINE_SURFACE ( 1, 2, ( 
 ( #4575, #105340, #171378, #89087, #189755, #137833, #203854, #169246, #138902, #136760, #139980, #202788, #106437, #70649, #107517, #73887, #172460, #24047, #173546, #20834, #5640, #25120, #90150, #91224, #55499, #88002, #206002, #201719, #121653, #157284, #8873, #185481, #86933, #135694, #53361, #119495, #37107, #54438, #186557, #38186, #10995, #141063, #109663, #95501, #190814, #93360, #30477, #74952, #43540, #111787, #178866, #159396, #175665, #174612, #162609, #96562, #42474, #207070, #27252, #112851, #192950, #108584, #26188, #76016, #92303, #211331, #61903, #60830, #58700, #45670, #78141, #124849, #142119, #158347, #9941, #208133, #129125, #209190, #59761, #177793, #125921, #191880, #77071, #13135, #143200, #44602, #12073, #144272, #126991, #110717, #176717, #28330, #94426, #160466, #210265, #128064, #194020, #29410, #161548, #62956, #79212, #145330, #195102, #46738, #84534, #197215, #48855, #1128, #101855, #130178, #16312, #49911, #199331, #17379, #97618, #15258, #150624, #52045, #99723, #81345, #179920, #148487, #34710, #2185, #113924, #33649, #18457, #68261, #183099, #67190, #134393, #55, #132261, #116032, #65072, #200396, #114969, #180969, #133327, #14185, #196171, #82397, #182019, #50976, #83462, #163675, #147425, #118171, #184158, #165795, #213449, #31542, #66118, #100780, #35779, #131227, #149542, #80278, #146376, #166862, #117098, #198268, #212390, #64032, #47811, #164723, #32591, #98668, #168983, #172201, #20583, #171116, #185216, #73615, #188430, #22709, #6462, #155947, #135434, #186287, #89896, #72539, #7532, #87736, #136504, #154879, #19522, #37925, #105078, #54173, #3256, #201456, #153811, #55243, #85598, #121390, #122470, #103999, #5383, #170042, #151686, #202524, #40065, #69324, #21628, #123535, #167923, #120313, #204659, #57372, #71460, #137573, #53100, #41145, #189500, #119233, #36840, #203591, #205739, #187363, #102922, #86668, #152735, #4317, #139715, #138637, #38993, #70387, #56309, #88824, #106175, #23789, #157022, #62687, #174345, #161276, #26986, #74691, #209994, #173275, #140794 ),
 ( #25923, #61636, #193757, #95226, #24855, #142926, #144002, #206806, #42208, #92031, #90957, #77880, #125652, #194828, #12863, #192681, #158089, #207873, #9677, #8608, #108325, #109397, #107255, #75753, #58439, #124594, #141863, #127803, #45404, #78937, #190552, #208926, #111520, #59495, #191614, #43276, #176457, #177526, #60561, #175402, #93093, #159134, #10736, #29139, #76806, #126720, #44334, #110456, #28069, #145059, #94163, #160203, #11805, #211062, #128846, #96294, #147171, #166607, #130971, #129923, #149283, #134140, #179662, #50716, #148233, #115773, #63763, #98405, #32337, #195910, #214234, #65862, #97357, #67998, #178597, #48601, #146114, #47546, #34461, #49650, #132012, #113658, #13929, #46463, #114719, #198022, #196963, #164470, #213198, #81084, #181763, #163414, #18196, #33396, #80009, #14990, #162346, #31282, #165533, #16056, #212125, #133072, #112586, #64827, #1938, #66930, #180714, #99474, #82140, #864, #17126, #83201, #30207, #199070, #116842, #100533, #182843, #84281, #150368, #187108, #171943, #153562, #37672, #184963, #22460, #170870, #103748, #36589, #3005, #89642, #88572, #188178, #154630, #39812, #203340, #122216, #152489, #202273, #5133, #136254, #169799, #86423, #20336, #121145, #102676, #105918, #71208, #167668, #168735, #101600, #69074, #104824, #21388, #19269, #72279, #7277, #4071, #155695, #6210, #70141, #38742, #35523, #138388, #120061, #137324, #51801, #53924, #204406, #23534, #56059, #87497, #186036, #73354, #200147, #54993, #117919, #183913, #85351, #151432, #135194, #201211, #52850, #118984, #27820, #127550, #93917, #193521, #142672, #61391, #91781, #58188, #123290, #110209, #157838, #12620, #45162, #10489, #124346, #25674, #41961, #40893, #140547, #141616, #139457, #190304, #173022, #106997, #206560, #159958, #11562, #111276, #205489, #175159, #176218, #24603, #74444, #108073, #208683, #143754, #92848, #57123, #207626, #59244, #9435, #77632, #189253, #125402, #75505, #174101, #191367, #177279, #43034, #90712, #192434, #109146, #26745, #156774, #158892, #28895, #76562, #8360 ) ),
 .UNSPECIFIED., .F., .F., .T. ) 
 B_SPLINE_SURFACE_WITH_KNOTS ( ( 2, 2 ),
 ( 3, 2, 2, 2, 2, 2, 2, 2, 2, 2, 2, 2, 2, 2, 2, 2, 2, 2, 2, 2, 2, 2, 2, 2, 2, 2, 2, 2, 2, 2, 2, 2, 2, 2, 2, 2, 2, 2, 2, 2, 2, 2, 2, 2, 2, 2, 2, 2, 2, 2, 2, 2, 2, 2, 2, 2, 2, 2, 2, 2, 2, 2, 2, 2, 2, 2, 2, 2, 2, 2, 2, 2, 2, 2, 2, 2, 2, 2, 2, 2, 2, 2, 2, 2, 2, 2, 2, 2, 2, 2, 2, 2, 2, 2, 2, 2, 2, 2, 2, 2, 2, 2, 2, 2, 2, 2, 2, 2, 2, 2, 2, 2, 2, 2, 2, 2, 2, 2, 2, 2, 3 ),
 ( 0.000000000000000000, 1.000000000000000000 ),
 ( 0.000000000000000000, 0.008333333333333333218, 0.01666666666666666644, 0.02500000000000000139, 0.03333333333333333287, 0.04166666666666666435, 0.05000000000000000278, 0.05833333333333333426, 0.06666666666666666574, 0.07499999999999999722, 0.08333333333333332871, 0.09166666666666666019, 0.1000000000000000056, 0.1083333333333333370, 0.1166666666666666685, 0.1250000000000000000, 0.1333333333333333315, 0.1416666666666666630, 0.1499999999999999944, 0.1583333333333333259, 0.1666666666666666574, 0.1749999999999999889, 0.1833333333333333204, 0.1916666666666666796, 0.2000000000000000111, 0.2083333333333333426, 0.2166666666666666741, 0.2250000000000000056, 0.2333333333333333370, 0.2416666666666666685, 0.2500000000000000000, 0.2583333333333333592, 0.2666666666666666630, 0.2750000000000000222, 0.2833333333333333259, 0.2916666666666666852, 0.2999999999999999889, 0.3083333333333333481, 0.3166666666666666519, 0.3250000000000000111, 0.3333333333333333148, 0.3416666666666666741, 0.3499999999999999778, 0.3583333333333333370, 0.3666666666666666408, 0.3750000000000000000, 0.3833333333333333592, 0.3916666666666666630, 0.4000000000000000222, 0.4083333333333333259, 0.4166666666666666852, 0.4249999999999999889, 0.4333333333333333481, 0.4416666666666666519, 0.4500000000000000111, 0.4583333333333333148, 0.4666666666666666741, 0.4749999999999999778, 0.4833333333333333370, 0.4916666666666666408, 0.5000000000000000000, 0.5083333333333333037, 0.5166666666666667185, 0.5250000000000000222, 0.5333333333333333259, 0.5416666666666666297, 0.5500000000000000444, 0.5583333333333333481, 0.5666666666666666519, 0.5749999999999999556, 0.5833333333333333703, 0.5916666666666666741, 0.5999999999999999778, 0.6083333333333332815, 0.6166666666666666963, 0.6250000000000000000, 0.6333333333333333037, 0.6416666666666667185, 0.6500000000000000222, 0.6583333333333333259, 0.6666666666666666297, 0.6750000000000000444, 0.6833333333333333481, 0.6916666666666666519, 0.6999999999999999556, 0.7083333333333333703, 0.7166666666666666741, 0.7249999999999999778, 0.7333333333333332815, 0.7416666666666666963, 0.7500000000000000000, 0.7583333333333333037, 0.7666666666666667185, 0.7750000000000000222, 0.7833333333333333259, 0.7916666666666666297, 0.8000000000000000444, 0.8083333333333333481, 0.8166666666666666519, 0.8249999999999999556, 0.8333333333333333703, 0.8416666666666666741, 0.8499999999999999778, 0.8583333333333332815, 0.8666666666666666963, 0.8750000000000000000, 0.8833333333333333037, 0.8916666666666667185, 0.9000000000000000222, 0.9083333333333333259, 0.9166666666666666297, 0.9250000000000000444, 0.9333333333333333481, 0.9416666666666666519, 0.9499999999999999556, 0.9583333333333333703, 0.9666666666666666741, 0.9749999999999999778, 0.9833333333333332815, 0.9916666666666666963, 1.000000000000000000 ),
 .UNSPECIFIED. ) 
 GEOMETRIC_REPRESENTATION_ITEM ( )  RATIONAL_B_SPLINE_SURFACE ( (
 ( 1.000000000000000000, 0.8660254037844387076, 1.000000000000000000, 0.8660254037844387076, 1.000000000000000000, 0.8660254037844387076, 1.000000000000000000, 0.8660254037844387076, 1.000000000000000000, 0.8660254037844387076, 1.000000000000000000, 0.8660254037844387076, 1.000000000000000000, 0.8660254037844387076, 1.000000000000000000, 0.8660254037844387076, 1.000000000000000000, 0.8660254037844387076, 1.000000000000000000, 0.8660254037844387076, 1.000000000000000000, 0.8660254037844387076, 1.000000000000000000, 0.8660254037844387076, 1.000000000000000000, 0.8660254037844387076, 1.000000000000000000, 0.8660254037844387076, 1.000000000000000000, 0.8660254037844387076, 1.000000000000000000, 0.8660254037844387076, 1.000000000000000000, 0.8660254037844387076, 1.000000000000000000, 0.8660254037844387076, 1.000000000000000000, 0.8660254037844387076, 1.000000000000000000, 0.8660254037844387076, 1.000000000000000000, 0.8660254037844387076, 1.000000000000000000, 0.8660254037844387076, 1.000000000000000000, 0.8660254037844387076, 1.000000000000000000, 0.8660254037844387076, 1.000000000000000000, 0.8660254037844387076, 1.000000000000000000, 0.8660254037844387076, 1.000000000000000000, 0.8660254037844387076, 1.000000000000000000, 0.8660254037844387076, 1.000000000000000000, 0.8660254037844387076, 1.000000000000000000, 0.8660254037844387076, 1.000000000000000000, 0.8660254037844387076, 1.000000000000000000, 0.8660254037844387076, 1.000000000000000000, 0.8660254037844387076, 1.000000000000000000, 0.8660254037844387076, 1.000000000000000000, 0.8660254037844387076, 1.000000000000000000, 0.8660254037844387076, 1.000000000000000000, 0.8660254037844387076, 1.000000000000000000, 0.8660254037844387076, 1.000000000000000000, 0.8660254037844387076, 1.000000000000000000, 0.8660254037844387076, 1.000000000000000000, 0.8660254037844387076, 1.000000000000000000, 0.8660254037844387076, 1.000000000000000000, 0.8660254037844387076, 1.000000000000000000, 0.8660254037844387076, 1.000000000000000000, 0.8660254037844387076, 1.000000000000000000, 0.8660254037844387076, 1.000000000000000000, 0.8660254037844387076, 1.000000000000000000, 0.8660254037844387076, 1.000000000000000000, 0.8660254037844387076, 1.000000000000000000, 0.8660254037844387076, 1.000000000000000000, 0.8660254037844387076, 1.000000000000000000, 0.8660254037844387076, 1.000000000000000000, 0.8660254037844387076, 1.000000000000000000, 0.8660254037844387076, 1.000000000000000000, 0.8660254037844387076, 1.000000000000000000, 0.8660254037844387076, 1.000000000000000000, 0.8660254037844387076, 1.000000000000000000, 0.8660254037844387076, 1.000000000000000000, 0.8660254037844387076, 1.000000000000000000, 0.8660254037844387076, 1.000000000000000000, 0.8660254037844387076, 1.000000000000000000, 0.8660254037844387076, 1.000000000000000000, 0.8660254037844387076, 1.000000000000000000, 0.8660254037844387076, 1.000000000000000000, 0.8660254037844387076, 1.000000000000000000, 0.8660254037844387076, 1.000000000000000000, 0.8660254037844387076, 1.000000000000000000, 0.8660254037844387076, 1.000000000000000000, 0.8660254037844387076, 1.000000000000000000, 0.8660254037844387076, 1.000000000000000000, 0.8660254037844387076, 1.000000000000000000, 0.8660254037844387076, 1.000000000000000000, 0.8660254037844387076, 1.000000000000000000, 0.8660254037844387076, 1.000000000000000000, 0.8660254037844387076, 1.000000000000000000, 0.8660254037844387076, 1.000000000000000000, 0.8660254037844387076, 1.000000000000000000, 0.8660254037844387076, 1.000000000000000000, 0.8660254037844387076, 1.000000000000000000, 0.8660254037844387076, 1.000000000000000000, 0.8660254037844387076, 1.000000000000000000, 0.8660254037844387076, 1.000000000000000000, 0.8660254037844387076, 1.000000000000000000, 0.8660254037844387076, 1.000000000000000000, 0.8660254037844387076, 1.000000000000000000, 0.8660254037844387076, 1.000000000000000000, 0.8660254037844387076, 1.000000000000000000, 0.8660254037844387076, 1.000000000000000000, 0.8660254037844387076, 1.000000000000000000, 0.8660254037844387076, 1.000000000000000000, 0.8660254037844387076, 1.000000000000000000, 0.8660254037844387076, 1.000000000000000000, 0.8660254037844387076, 1.000000000000000000, 0.8660254037844387076, 1.000000000000000000, 0.8660254037844387076, 1.000000000000000000, 0.8660254037844387076, 1.000000000000000000, 0.8660254037844387076, 1.000000000000000000, 0.8660254037844387076, 1.000000000000000000, 0.8660254037844387076, 1.000000000000000000, 0.8660254037844387076, 1.000000000000000000, 0.8660254037844387076, 1.000000000000000000, 0.8660254037844387076, 1.000000000000000000, 0.8660254037844387076, 1.000000000000000000, 0.8660254037844387076, 1.000000000000000000, 0.8660254037844387076, 1.000000000000000000, 0.8660254037844387076, 1.000000000000000000, 0.8660254037844387076, 1.000000000000000000, 0.8660254037844387076, 1.000000000000000000, 0.8660254037844387076, 1.000000000000000000, 0.8660254037844387076, 1.000000000000000000, 0.8660254037844387076, 1.000000000000000000, 0.8660254037844387076, 1.000000000000000000, 0.8660254037844387076, 1.000000000000000000, 0.8660254037844387076, 1.000000000000000000, 0.8660254037844387076, 1.000000000000000000, 0.8660254037844387076, 1.000000000000000000, 0.8660254037844387076, 1.000000000000000000, 0.8660254037844387076, 1.000000000000000000, 0.8660254037844387076, 1.000000000000000000, 0.8660254037844387076, 1.000000000000000000),
 ( 1.000000000000000000, 0.8660254037844387076, 1.000000000000000000, 0.8660254037844387076, 1.000000000000000000, 0.8660254037844387076, 1.000000000000000000, 0.8660254037844387076, 1.000000000000000000, 0.8660254037844387076, 1.000000000000000000, 0.8660254037844387076, 1.000000000000000000, 0.8660254037844387076, 1.000000000000000000, 0.8660254037844387076, 1.000000000000000000, 0.8660254037844387076, 1.000000000000000000, 0.8660254037844387076, 1.000000000000000000, 0.8660254037844387076, 1.000000000000000000, 0.8660254037844387076, 1.000000000000000000, 0.8660254037844387076, 1.000000000000000000, 0.8660254037844387076, 1.000000000000000000, 0.8660254037844387076, 1.000000000000000000, 0.8660254037844387076, 1.000000000000000000, 0.8660254037844387076, 1.000000000000000000, 0.8660254037844387076, 1.000000000000000000, 0.8660254037844387076, 1.000000000000000000, 0.8660254037844387076, 1.000000000000000000, 0.8660254037844387076, 1.000000000000000000, 0.8660254037844387076, 1.000000000000000000, 0.8660254037844387076, 1.000000000000000000, 0.8660254037844387076, 1.000000000000000000, 0.8660254037844387076, 1.000000000000000000, 0.8660254037844387076, 1.000000000000000000, 0.8660254037844387076, 1.000000000000000000, 0.8660254037844387076, 1.000000000000000000, 0.8660254037844387076, 1.000000000000000000, 0.8660254037844387076, 1.000000000000000000, 0.8660254037844387076, 1.000000000000000000, 0.8660254037844387076, 1.000000000000000000, 0.8660254037844387076, 1.000000000000000000, 0.8660254037844387076, 1.000000000000000000, 0.8660254037844387076, 1.000000000000000000, 0.8660254037844387076, 1.000000000000000000, 0.8660254037844387076, 1.000000000000000000, 0.8660254037844387076, 1.000000000000000000, 0.8660254037844387076, 1.000000000000000000, 0.8660254037844387076, 1.000000000000000000, 0.8660254037844387076, 1.000000000000000000, 0.8660254037844387076, 1.000000000000000000, 0.8660254037844387076, 1.000000000000000000, 0.8660254037844387076, 1.000000000000000000, 0.8660254037844387076, 1.000000000000000000, 0.8660254037844387076, 1.000000000000000000, 0.8660254037844387076, 1.000000000000000000, 0.8660254037844387076, 1.000000000000000000, 0.8660254037844387076, 1.000000000000000000, 0.8660254037844387076, 1.000000000000000000, 0.8660254037844387076, 1.000000000000000000, 0.8660254037844387076, 1.000000000000000000, 0.8660254037844387076, 1.000000000000000000, 0.8660254037844387076, 1.000000000000000000, 0.8660254037844387076, 1.000000000000000000, 0.8660254037844387076, 1.000000000000000000, 0.8660254037844387076, 1.000000000000000000, 0.8660254037844387076, 1.000000000000000000, 0.8660254037844387076, 1.000000000000000000, 0.8660254037844387076, 1.000000000000000000, 0.8660254037844387076, 1.000000000000000000, 0.8660254037844387076, 1.000000000000000000, 0.8660254037844387076, 1.000000000000000000, 0.8660254037844387076, 1.000000000000000000, 0.8660254037844387076, 1.000000000000000000, 0.8660254037844387076, 1.000000000000000000, 0.8660254037844387076, 1.000000000000000000, 0.8660254037844387076, 1.000000000000000000, 0.8660254037844387076, 1.000000000000000000, 0.8660254037844387076, 1.000000000000000000, 0.8660254037844387076, 1.000000000000000000, 0.8660254037844387076, 1.000000000000000000, 0.8660254037844387076, 1.000000000000000000, 0.8660254037844387076, 1.000000000000000000, 0.8660254037844387076, 1.000000000000000000, 0.8660254037844387076, 1.000000000000000000, 0.8660254037844387076, 1.000000000000000000, 0.8660254037844387076, 1.000000000000000000, 0.8660254037844387076, 1.000000000000000000, 0.8660254037844387076, 1.000000000000000000, 0.8660254037844387076, 1.000000000000000000, 0.8660254037844387076, 1.000000000000000000, 0.8660254037844387076, 1.000000000000000000, 0.8660254037844387076, 1.000000000000000000, 0.8660254037844387076, 1.000000000000000000, 0.8660254037844387076, 1.000000000000000000, 0.8660254037844387076, 1.000000000000000000, 0.8660254037844387076, 1.000000000000000000, 0.8660254037844387076, 1.000000000000000000, 0.8660254037844387076, 1.000000000000000000, 0.8660254037844387076, 1.000000000000000000, 0.8660254037844387076, 1.000000000000000000, 0.8660254037844387076, 1.000000000000000000, 0.8660254037844387076, 1.000000000000000000, 0.8660254037844387076, 1.000000000000000000, 0.8660254037844387076, 1.000000000000000000, 0.8660254037844387076, 1.000000000000000000, 0.8660254037844387076, 1.000000000000000000, 0.8660254037844387076, 1.000000000000000000, 0.8660254037844387076, 1.000000000000000000, 0.8660254037844387076, 1.000000000000000000, 0.8660254037844387076, 1.000000000000000000, 0.8660254037844387076, 1.000000000000000000, 0.8660254037844387076, 1.000000000000000000, 0.8660254037844387076, 1.000000000000000000, 0.8660254037844387076, 1.000000000000000000, 0.8660254037844387076, 1.000000000000000000, 0.8660254037844387076, 1.000000000000000000, 0.8660254037844387076, 1.000000000000000000, 0.8660254037844387076, 1.000000000000000000, 0.8660254037844387076, 1.000000000000000000, 0.8660254037844387076, 1.000000000000000000, 0.8660254037844387076, 1.000000000000000000, 0.8660254037844387076, 1.000000000000000000, 0.8660254037844387076, 1.000000000000000000, 0.8660254037844387076, 1.000000000000000000, 0.8660254037844387076, 1.000000000000000000, 0.8660254037844387076, 1.000000000000000000, 0.8660254037844387076, 1.000000000000000000, 0.8660254037844387076, 1.000000000000000000) ) ) 
 REPRESENTATION_ITEM ( '' )  SURFACE ( )  );
#75352=CARTESIAN_POINT ( 'NONE',  ( -5.029148636026397945, 4.832037928311032182, 0.7998128361456281477 ) ) ;
#75355=CARTESIAN_POINT ( 'NONE',  ( -7.404161286394468355, 7.810812053647902431, 0.000000000000000000 ) ) ;
#75367=CARTESIAN_POINT ( 'NONE',  ( 5.259637247458703868, 5.100941308315409373, 0.000000000000000000 ) ) ;
#75368=CARTESIAN_POINT ( 'NONE',  ( 4.694866332082116678, 8.699370830729650450, 0.7998128361456341429 ) ) ;
#75374=CARTESIAN_POINT ( 'NONE',  ( 4.543917759235442944, 5.330267469643351852, 1.199719254218452935 ) ) ;
#75380=CARTESIAN_POINT ( 'NONE',  ( 6.008198349511364000, 7.038594824965278995, 1.199719254218453823 ) ) ;
#75381=ORIENTED_EDGE ( 'NONE', *, *, #172230, .T. ) ;
#75393=CARTESIAN_POINT ( 'NONE',  ( 7.838022202476093270, 8.316983122409855156, 0.7216878364870267237 ) ) ;
#75394=CARTESIAN_POINT ( 'NONE',  ( -4.584065335196305213, 6.441438539186039591, 1.443375672974058777 ) ) ;
#75395=CARTESIAN_POINT ( 'NONE',  ( -7.262327558775498737, 8.501745569106741840, 1.199719254218452047 ) ) ;
#75397=CARTESIAN_POINT ( 'NONE',  ( -5.820051620566758288, 5.754758076941462797, 0.6671413377488121244 ) ) ;
#75407=CARTESIAN_POINT ( 'NONE',  ( 6.540882763950133238, 6.595727744222092959, 0.000000000000000000 ) ) ;
#75408=CARTESIAN_POINT ( 'NONE',  ( 6.282224075085741433, 8.422623735723785643, 1.599625672291268286 ) ) ;
#75411=CARTESIAN_POINT ( 'NONE',  ( 3.241808126998965811, 6.796210224891872542, 0.7216878364870257245 ) ) ;
#75413=ORIENTED_EDGE ( 'NONE', *, *, #63569, .T. ) ;
#75426=TOROIDAL_SURFACE ( 'NONE', #172224, 0.8300000000000010703, 0.08000000000000000167 ) ;
#75429=CARTESIAN_POINT ( 'NONE',  ( 4.115782150200256950, 6.959440387612411349, 1.199719254218452047 ) ) ;
#75433=CARTESIAN_POINT ( 'NONE',  ( 5.574337433874081427, 6.532423756721743580, -1.199719254218452047 ) ) ;
#75437=CARTESIAN_POINT ( 'NONE',  ( 5.671053392266061977, 9.838255734277600695, 0.7998128361456331437 ) ) ;
#75442=CARTESIAN_POINT ( 'NONE',  ( 4.570507181582611267, 8.346359121906111511, 0.000000000000000000 ) ) ;
#75444=CARTESIAN_POINT ( 'NONE',  ( -4.294900800479008574, 8.232744377192641849, 0.000000000000000000 ) ) ;
#75445=CARTESIAN_POINT ( 'NONE',  ( 5.401997860402196316, 5.267028690082820930, 0.000000000000000000 ) ) ;
#75452=CARTESIAN_POINT ( 'NONE',  ( -5.980802423990385641, 6.150226714305422782, 9.481663569016276247E-06 ) ) ;
#75455=CARTESIAN_POINT ( 'NONE',  ( -3.959863383643135393, 6.777535159962392086, 1.199719254218452935 ) ) ;
#75459=ORIENTED_EDGE ( 'NONE', *, *, #157556, .F. ) ;
#75490=CARTESIAN_POINT ( 'NONE',  ( -5.317278910447152285, 7.722098771695092623, -1.369991256297370619 ) ) ;
#75491=CARTESIAN_POINT ( 'NONE',  ( 5.221298554594243413, 5.264138866547622975, -0.7216878364870458196 ) ) ;
#75503=CARTESIAN_POINT ( 'NONE',  ( -6.771371375382467583, 6.864631124226471037, -0.7998128361456362523 ) ) ;
#75505=CARTESIAN_POINT ( 'NONE',  ( 7.960045584554727327, 8.459343734834927631, 0.7216878364870267237 ) ) ;
#75514=CARTESIAN_POINT ( 'NONE',  ( -4.634908411025374875, 6.500755460986618495, 1.599625672291263179 ) ) ;
#75521=CARTESIAN_POINT ( 'NONE',  ( -4.556949027968976829, 5.449433633119473264, 1.082531754730549078 ) ) ;
#75526=CARTESIAN_POINT ( 'NONE',  ( -5.204350862799341115, 7.165104988056252289, -1.599625672291271394 ) ) ;
#75549=ORIENTED_EDGE ( 'NONE', *, *, #183283, .T. ) ;
#75550=CARTESIAN_POINT ( 'NONE',  ( -6.903036488013351679, 8.082572653217566128, -1.199719254218452047 ) ) ;
#75551=CARTESIAN_POINT ( 'NONE',  ( -5.143339171537843590, 7.093924681584509173, 1.599625672291263179 ) ) ;
#75577=CARTESIAN_POINT ( 'NONE',  ( -4.999100218102086046, 8.030536425943571643, -1.156731540297722738 ) ) ;
#75578=CARTESIAN_POINT ( 'NONE',  ( -5.281783360975562225, 8.319775133516907673, 1.199719254218452935 ) ) ;
#75605=CARTESIAN_POINT ( 'NONE',  ( 6.042093733545556233, 7.078139439671806699, -1.199719254218452047 ) ) ;
#75609=CARTESIAN_POINT ( 'NONE',  ( -2.750656850324853409, 2.940527718787148803, -2.453100388279096933 ) ) ;
#75620=CIRCLE ( 'NONE', #61701, 0.08000000000000052902 ) ;
#75621=CARTESIAN_POINT ( 'NONE',  ( 6.396603524444617328, 6.809554808131969672, -0.5206029305389828776 ) ) ;
#75623=CARTESIAN_POINT ( 'NONE',  ( 5.533136088152891929, 9.469426179571447832, -0.7216878364870458196 ) ) ;
#75631=CARTESIAN_POINT ( 'NONE',  ( -3.447516199624892419, 7.244129009529488350, 0.7998128361456352531 ) ) ;
#75640=CARTESIAN_POINT ( 'NONE',  ( -5.438229012412890917, 8.398332043573416783, -1.082531754730549967 ) ) ;
#75645=CARTESIAN_POINT ( 'NONE',  ( 5.066578194877104480, 4.909125722664362534, -0.2447466197543680111 ) ) ;
#75649=CARTESIAN_POINT ( 'NONE',  ( -4.228163802615396705, 6.026220084508304708, -1.599625672291271394 ) ) ;
#75658=CARTESIAN_POINT ( 'NONE',  ( 5.494797395288433250, 9.632623737803665875, 0.000000000000000000 ) ) ;
#75676=CARTESIAN_POINT ( 'NONE',  ( -6.505933609711270549, 8.683618192786854095, -1.599625672291271394 ) ) ;
#75679=CARTESIAN_POINT ( 'NONE',  ( 6.099189001301251523, 8.209082816308541197, 1.599625672291268286 ) ) ;
#75695=FACE_OUTER_BOUND ( 'NONE', #93870, .T. ) ;
#75696=CARTESIAN_POINT ( 'NONE',  ( 4.584065335196261692, 7.401807753487379848, 1.082531754730549078 ) ) ;
#75703=CARTESIAN_POINT ( 'NONE',  ( 5.854088466050551887, 10.05179665369283981, 0.7998128361456341429 ) ) ;
#75707=CARTESIAN_POINT ( 'NONE',  ( -4.177320726786315497, 7.887641591310407208, -0.7216878364870458196 ) ) ;
#75710=EDGE_LOOP ( 'NONE', ( #24572, #144958 ) ) ;
#75725=EDGE_CURVE ( 'NONE', #134523, #43808, #160859, .T. ) ;
#75729=CARTESIAN_POINT ( 'NONE',  ( -5.294420283343134415, 6.244149675475041406, 1.216503418957364246 ) ) ;
#75739=CARTESIAN_POINT ( 'NONE',  ( 5.065906673361608270, 5.939254536123854677, -1.199719254218450271 ) ) ;
#75748=( BOUNDED_CURVE ( )  B_SPLINE_CURVE ( 2, ( #164453, #100515, #135177, #166590, #134123, #200132, #51785 ),
 .UNSPECIFIED., .F., .T. ) 
 B_SPLINE_CURVE_WITH_KNOTS ( ( 3, 2, 2, 3 ),
 ( 0.4000000000000005773, 0.4083333333333336590, 0.4166666666666667407, 0.4249999999999998224 ),
 .UNSPECIFIED. ) 
 CURVE ( )  GEOMETRIC_REPRESENTATION_ITEM ( )  RATIONAL_B_SPLINE_CURVE ( ( 0.9999999999999911182, 0.8660254037844475894, 1.000000000000000000, 0.8660254037844387076, 1.000000000000000000, 0.8660254037844413721, 0.9999999999999973355 ) ) 
 REPRESENTATION_ITEM ( '' )  );
#75751=CARTESIAN_POINT ( 'NONE',  ( -6.455090533882206216, 7.663932056684933158, -1.082531754730549967 ) ) ;
#75753=CARTESIAN_POINT ( 'NONE',  ( 5.194182247366881278, 5.232503174782402233, 0.7216878364870328300 ) ) ;
#75772=CARTESIAN_POINT ( 'NONE',  ( -4.394251184604987870, 5.259619482528146150, 1.082531754730549078 ) ) ;
#75776=CARTESIAN_POINT ( 'NONE',  ( -6.427974226210522168, 6.671927150099951298, 0.000000000000000000 ) ) ;
#75788=ORIENTED_EDGE ( 'NONE', *, *, #156207, .F. ) ;
#75802=CARTESIAN_POINT ( 'NONE',  ( -6.688968683495758683, 8.897159112202094988, -1.599625672291271394 ) ) ;
#75805=CARTESIAN_POINT ( 'NONE',  ( -6.961185525973791144, 7.086080966583015339, 0.7998128361456341429 ) ) ;
#75810=CARTESIAN_POINT ( 'NONE',  ( -5.261973015435229328, 9.153069261400824885, 0.000000000000000000 ) ) ;
#75811=CARTESIAN_POINT ( 'NONE',  ( 8.136301581532414673, 8.664975731308866003, 0.000000000000000000 ) ) ;
#75817=CARTESIAN_POINT ( 'NONE',  ( -6.005335696210345020, 5.970922831858983315, 0.7998128361456281477 ) ) ;
#75828=CARTESIAN_POINT ( 'NONE',  ( 5.772745519453025054, 7.247817053759448847, -1.191736586928717978 ) ) ;
#75832=CARTESIAN_POINT ( 'NONE',  ( 4.980641328173811999, 6.904110530993182948, 1.599625672291269396 ) ) ;
#75853=CARTESIAN_POINT ( 'NONE',  ( 2.925527285498711549, 6.635141943048991742, 0.7998128361456281477 ) ) ;
#75862=DIRECTION ( 'NONE',  ( -1.000000000000000000, 0.000000000000000000, 0.000000000000000000 ) ) ;
#75869=CARTESIAN_POINT ( 'NONE',  ( 6.333059215844621725, 6.948315255594014417, 0.8781869475623119703 ) ) ;
#75870=CARTESIAN_POINT ( 'NONE',  ( -5.167065940139584868, 6.161236697318522637, 1.082531754730549078 ) ) ;
#75889=AXIS2_PLACEMENT_3D ( 'NONE', #178756, #209079, #30368 ) ;
#75900=CARTESIAN_POINT ( 'NONE',  ( 5.063044020060520900, 4.871582543017558109, 0.7998128361456352531 ) ) ;
#75908=CARTESIAN_POINT ( 'NONE',  ( -6.116136693540540570, 10.14959355252369910, 0.000000000000000000 ) ) ;
#75919=CARTESIAN_POINT ( 'NONE',  ( -4.932134020321308654, 8.976183133675331050, 0.7998128361456291469 ) ) ;
#75934=CARTESIAN_POINT ( 'NONE',  ( 4.115782150200256950, 6.959440387612411349, 1.199719254218452047 ) ) ;
#75943=CARTESIAN_POINT ( 'NONE',  ( 4.805106176720093103, 8.123399998552004675, 0.8388070820863163801 ) ) ;
#75944=DIRECTION ( 'NONE',  ( -0.7771862570881746812, 0.6292706268317899143, 0.000000000000000000 ) ) ;
#75945=CARTESIAN_POINT ( 'NONE',  ( 4.802738015080052492, 8.126035781178083894, 0.8349615142884360131 ) ) ;
#75966=CARTESIAN_POINT ( 'NONE',  ( -4.769436176957319695, 8.786368983084006601, 0.7998128361456281477 ) ) ;
#75968=CARTESIAN_POINT ( 'NONE',  ( 5.061990249855835344, 6.999017606288844284, -1.599625672291273171 ) ) ;
#75972=CARTESIAN_POINT ( 'NONE',  ( -6.445975688654487001, 6.485002823043819475, -0.7998128361456362523 ) ) ;
#75980=CARTESIAN_POINT ( 'NONE',  ( -4.603205931398525408, 8.475712490939976362, -0.2800714110085516517 ) ) ;
#75981=CARTESIAN_POINT ( 'NONE',  ( 4.858757509019057785, 5.629766575900002401, -2.420000000000000373 ) ) ;
#75997=CARTESIAN_POINT ( 'NONE',  ( 6.048345925472191631, 6.229027465905275562, 0.7216878364870328300 ) ) ;
#76001=CARTESIAN_POINT ( 'NONE',  ( -7.611976899429754084, 7.845337568948314022, 0.7998128361456341429 ) ) ;
#76016=CARTESIAN_POINT ( 'NONE',  ( 4.736594563127852098, 6.619389305106191834, -1.599625672291273171 ) ) ;
#76019=VECTOR ( 'NONE', #149125, 1000.000000000000000 ) ;
#76031=ORIENTED_EDGE ( 'NONE', *, *, #48405, .F. ) ;
#76063=CARTESIAN_POINT ( 'NONE',  ( 4.523580528814945545, 5.306540700819438960, 1.199719254218452047 ) ) ;
#76066=ORIENTED_EDGE ( 'NONE', *, *, #140054, .T. ) ;
#76067=CARTESIAN_POINT ( 'NONE',  ( -7.391130018105325661, 8.652015104991543026, -1.199719254218452047 ) ) ;
#76073=CARTESIAN_POINT ( 'NONE',  ( -5.418418667316934112, 6.350518529071726981, -1.199719254218453823 ) ) ;
#76081=CARTESIAN_POINT ( 'NONE',  ( -4.736594563127865420, 6.619389305106191834, -1.599625672291271394 ) ) ;
#76083=CARTESIAN_POINT ( 'NONE',  ( 5.894874513638865388, 7.262872338272549300, -1.253420816524719150 ) ) ;
#76087=CARTESIAN_POINT ( 'NONE',  ( 5.578253857379852576, 5.472660686556754861, -0.7998128361456481317 ) ) ;
#76093=CARTESIAN_POINT ( 'NONE',  ( -7.262327558775498737, 8.501745569106741840, 1.199719254218452047 ) ) ;
#76097=CARTESIAN_POINT ( 'NONE',  ( -5.795184315198522285, 5.725746220678519904, -0.7998128361456362523 ) ) ;
#76101=CARTESIAN_POINT ( 'NONE',  ( 5.844973620822844218, 5.991759777147701804, 0.7216878364870328300 ) ) ;
#76102=CARTESIAN_POINT ( 'NONE',  ( -6.170369307550858551, 8.292126506933035657, 1.443375672974058777 ) ) ;
#76110=CARTESIAN_POINT ( 'NONE',  ( 2.891631901464575272, 6.595597328342462262, 0.000000000000000000 ) ) ;
#76118=SURFACE_STYLE_USAGE ( .BOTH. , #11101 ) ;
#76141=CARTESIAN_POINT ( 'NONE',  ( 4.763071791759735163, 8.170823326046956936, 0.7639991172946744014 ) ) ;
#76148=CARTESIAN_POINT ( 'NONE',  ( 7.666209513884374438, 7.908608952478760834, 0.7998128361456281477 ) ) ;
#76153=CARTESIAN_POINT ( 'NONE',  ( -4.764376198328064582, 8.188698463893414825, 0.7498042881181687935 ) ) ;
#76159=CARTESIAN_POINT ( 'NONE',  ( -6.420668264523499147, 9.648474187656182366, 1.199719254218452935 ) ) ;
#76171=CARTESIAN_POINT ( 'NONE',  ( 6.200875153403774043, 8.327716660428123419, -1.599625672291283607 ) ) ;
#76180=CARTESIAN_POINT ( 'NONE',  ( 3.555981428534177091, 7.370671776590375757, 0.7998128361456271485 ) ) ;
#76183=CARTESIAN_POINT ( 'NONE',  ( 5.682275777458851707, 6.762314840857718501, 1.082531754730549078 ) ) ;
#76185=ORIENTED_EDGE ( 'NONE', *, *, #10253, .F. ) ;
#76197=CARTESIAN_POINT ( 'NONE',  ( -4.930325137224961907, 5.781076077297750970, -1.199719254218453823 ) ) ;
#76198=CARTESIAN_POINT ( 'NONE',  ( 7.838022202476093270, 8.316983122409855156, 0.7216878364870267237 ) ) ;
#76210=CARTESIAN_POINT ( 'NONE',  ( -4.749098946536820520, 8.762642214260091933, 0.7998128361456281477 ) ) ;
#76211=CARTESIAN_POINT ( 'NONE',  ( -3.786470039966538970, 7.639575156594750283, 0.000000000000000000 ) ) ;
#76213=CARTESIAN_POINT ( 'NONE',  ( 5.506019780481205217, 9.437790487287811558, 0.000000000000000000 ) ) ;
#76220=CARTESIAN_POINT ( 'NONE',  ( -5.000000000000013323, 11.39843543023555661, -0.7749999999999996891 ) ) ;
#76224=CARTESIAN_POINT ( 'NONE',  ( -6.237206930280429162, 6.931128591455327559, -0.8289643595828979361 ) ) ;
#76225=FACE_BOUND ( 'NONE', #124265, .T. ) ;
#76231=CARTESIAN_POINT ( 'NONE',  ( 4.746763178560261309, 5.670883475476017566, 1.082531754730549078 ) ) ;
#76236=CARTESIAN_POINT ( 'NONE',  ( 1.854512760316388897, 0.000000000000000000, 2.484105960264901825 ) ) ;
#76237=CARTESIAN_POINT ( 'NONE',  ( -5.956828388357799042, 8.042995434541133193, 1.599625672291263179 ) ) ;
#76251=CARTESIAN_POINT ( 'NONE',  ( 6.690022453700429139, 6.769724048930809701, 0.7998128361456331437 ) ) ;
#76267=CARTESIAN_POINT ( 'NONE',  ( 2.971635387262909767, 6.554378586761894887, 0.4847971991465233610 ) ) ;
#76286=CARTESIAN_POINT ( 'NONE',  ( 5.058600711674583472, 8.915801573680086634, 0.000000000000000000 ) ) ;
#76290=CARTESIAN_POINT ( 'NONE',  ( 7.065207446497155708, 9.336104335703744539, 0.000000000000000000 ) ) ;
#76316=B_SPLINE_CURVE_WITH_KNOTS ( 'NONE', 3,
 ( #210280, #192966, #112866, #129141, #111803, #211347 ),
 .UNSPECIFIED., .F., .F.,
 ( 4, 2, 4 ),
 ( 2.054988457695394556E-16, 0.002406600572792993650, 0.004813201145585781736 ),
 .UNSPECIFIED. ) ;
#76317=ORIENTED_EDGE ( 'NONE', *, *, #77886, .F. ) ;
#76318=CARTESIAN_POINT ( 'NONE',  ( -5.340986169140711226, 5.195848383611072485, 0.000000000000000000 ) ) ;
#76320=CARTESIAN_POINT ( 'NONE',  ( 4.529832720297257254, 8.298905583739861314, 0.000000000000000000 ) ) ;
#76325=CARTESIAN_POINT ( 'NONE',  ( -4.899292406491858820, 6.809203455697518947, -1.599625672291271394 ) ) ;
#76330=CARTESIAN_POINT ( 'NONE',  ( -4.984557751679625781, 5.844347460828191565, 1.199719254218452935 ) ) ;
#76337=CARTESIAN_POINT ( 'NONE',  ( -3.474632506852224356, 7.275764701294714420, -0.7998128361456481317 ) ) ;
#76345=CARTESIAN_POINT ( 'NONE',  ( -5.307090785106547415, 5.156303768904543894, -0.7998128361456362523 ) ) ;
#76349=CARTESIAN_POINT ( 'NONE',  ( -7.105881907338178038, 7.462819444748888920, -0.7216878364870338292 ) ) ;
#76350=CARTESIAN_POINT ( 'NONE',  ( -6.577113915960849155, 6.845923454808663600, -0.7216878364870338292 ) ) ;
#76351=CARTESIAN_POINT ( 'NONE',  ( 7.049313524462606395, 7.188896964819984525, 0.000000000000000000 ) ) ;
#76352=CARTESIAN_POINT ( 'NONE',  ( -6.957269102468015554, 8.145844036748005834, 1.199719254218452047 ) ) ;
#76360=ORIENTED_EDGE ( 'NONE', *, *, #150546, .T. ) ;
#76370=CARTESIAN_POINT ( 'NONE',  ( 7.537407054554579489, 7.758339416593960536, 0.000000000000000000 ) ) ;
#76385=VECTOR ( 'NONE', #18158, 1000.000000000000000 ) ;
#76390=CARTESIAN_POINT ( 'NONE',  ( 4.623177087595867540, 8.455029494522658950, -0.3425024339245314464 ) ) ;
#76402=CARTESIAN_POINT ( 'NONE',  ( 6.225128807330042591, 7.291680359087043151, -1.199719254218452047 ) ) ;
#76405=CARTESIAN_POINT ( 'NONE',  ( -4.411198876399886615, 6.239761003923544713, -1.599625672291271394 ) ) ;
#76408=CARTESIAN_POINT ( 'NONE',  ( -7.255021596644144921, 7.636815748939187465, 0.7216878364870317197 ) ) ;
#76419=CARTESIAN_POINT ( 'NONE',  ( 5.083381250481017410, 4.895309311841474553, 0.7998128361456352531 ) ) ;
#76420=CARTESIAN_POINT ( 'NONE',  ( 4.532168488718122390, 8.509556680138327778, 0.7998128361456271485 ) ) ;
#76438=CARTESIAN_POINT ( 'NONE',  ( 6.387826650694035990, 7.481494509678370264, -1.199719254218452047 ) ) ;
#76449=CARTESIAN_POINT ( 'NONE',  ( 6.455090533882185788, 8.624301270986276080, -1.443375672974078761 ) ) ;
#76450=CARTESIAN_POINT ( 'NONE',  ( -6.455090533882213322, 6.703562842383589349, -0.7216878364870338292 ) ) ;
#76451=CARTESIAN_POINT ( 'NONE',  ( -7.286581212701773502, 7.465709267765667789, 0.7998128361456341429 ) ) ;
#76462=CARTESIAN_POINT ( 'NONE',  ( 5.017399365509065845, 8.011327138806002779, -1.199719254218450271 ) ) ;
#76463=CARTESIAN_POINT ( 'NONE',  ( 5.875479466675786355, 7.948088359245467416, -1.599625672291283607 ) ) ;
#76466=CARTESIAN_POINT ( 'NONE',  ( 4.543390873910906791, 6.393985001019784953, 1.443375672974065660 ) ) ;
#76480=FACE_OUTER_BOUND ( 'NONE', #82538, .T. ) ;
#76483=CARTESIAN_POINT ( 'NONE',  ( 3.074666975249065626, 6.809138247757705820, 0.000000000000000000 ) ) ;
#76485=CIRCLE ( 'NONE', #201076, 0.07999999999999948819 ) ;
#76487=CARTESIAN_POINT ( 'NONE',  ( 4.227110032410640095, 8.153655147779589996, 0.7998128361456271485 ) ) ;
#76493=CARTESIAN_POINT ( 'NONE',  ( 5.495418255317095380, 6.026204583819558813, -0.7979391942483995415 ) ) ;
#76497=CARTESIAN_POINT ( 'NONE',  ( 7.851580356089786328, 8.332800968292465527, 0.000000000000000000 ) ) ;
#76500=CARTESIAN_POINT ( 'NONE',  ( -4.847922445338252118, 7.813604065273374921, -1.199719254218453823 ) ) ;
#76501=CARTESIAN_POINT ( 'NONE',  ( 4.472210567661338843, 6.310941310395290493, 1.599625672291261402 ) ) ;
#76508=CARTESIAN_POINT ( 'NONE',  ( -4.001066012398721838, 7.682011088333574378, -6.818990669119789124E-05 ) ) ;
#76511=CARTESIAN_POINT ( 'NONE',  ( -5.147255595043616516, 6.034161611419515125, 1.199719254218452935 ) ) ;
#76541=ORIENTED_EDGE ( 'NONE', *, *, #39803, .F. ) ;
#76545=CARTESIAN_POINT ( 'NONE',  ( -5.458264003855187951, 7.602368174425947700, -1.382272695577278387 ) ) ;
#76546=CARTESIAN_POINT ( 'NONE',  ( 7.095713291905693332, 9.371694488680407886, 1.599625672291268286 ) ) ;
#76558=CARTESIAN_POINT ( 'NONE',  ( -4.793689830883590020, 7.750332681742931662, 1.199719254218452935 ) ) ;
#76560=CARTESIAN_POINT ( 'NONE',  ( -5.611095471209320174, 7.639640364534566075, 1.599625672291263179 ) ) ;
#76562=CARTESIAN_POINT ( 'NONE',  ( 8.122743427918724279, 8.649157885426255632, 0.7216878364870267237 ) ) ;
#76572=CARTESIAN_POINT ( 'NONE',  ( -5.367048706163331850, 7.354919138647580290, -1.599625672291271394 ) ) ;
#76579=CARTESIAN_POINT ( 'NONE',  ( -5.316205630334276400, 5.374863788244313767, -0.7216878364870338292 ) ) ;
#76584=CARTESIAN_POINT ( 'NONE',  ( -4.878955176071358757, 6.785476686873604280, -1.599625672291271394 ) ) ;
#76604=CARTESIAN_POINT ( 'NONE',  ( -5.420227550413282636, 9.545625585449309725, 0.7998128361456291469 ) ) ;
#76606=CARTESIAN_POINT ( 'NONE',  ( -6.140917232347002042, 6.129101290685087911, -0.7998128361456362523 ) ) ;
#76632=CARTESIAN_POINT ( 'NONE',  ( -4.959250327548641479, 9.007818825440551791, -0.7998128361456362523 ) ) ;
#76635=EDGE_CURVE ( 'NONE', #107579, #25034, #83744, .T. ) ;
#76658=CARTESIAN_POINT ( 'NONE',  ( 5.854088466050551887, 10.05179665369283981, 0.7998128361456341429 ) ) ;
#76661=CARTESIAN_POINT ( 'NONE',  ( 6.749980374757213575, 8.968339418673846097, 1.599625672291268286 ) ) ;
#76674=CARTESIAN_POINT ( 'NONE',  ( 6.086061792568233209, 7.019478939793144967, 0.9900148145245997178 ) ) ;
#76677=CARTESIAN_POINT ( 'NONE',  ( 5.722950238744198614, 8.730506807626655430, 1.082531754730549967 ) ) ;
#76683=CARTESIAN_POINT ( 'NONE',  ( -5.795184315198522285, 5.725746220678519904, -0.7998128361456362523 ) ) ;
#76686=EDGE_CURVE ( 'NONE', #137303, #112565, #108407, .T. ) ;
#76690=CARTESIAN_POINT ( 'NONE',  ( -7.065207446052822249, 7.415365906582643163, -0.7216878364870338292 ) ) ;
#76693=CARTESIAN_POINT ( 'NONE',  ( 7.828907357248368726, 8.098423103070084395, 0.7998128361456281477 ) ) ;
#76694=CARTESIAN_POINT ( 'NONE',  ( -5.785778052227864343, 5.972700719662596747, -0.3272196074983695357 ) ) ;
#76698=EDGE_CURVE ( 'NONE', #79244, #138713, #27076, .T. ) ;
#76699=CARTESIAN_POINT ( 'NONE',  ( -2.810282979782591006, 6.500690253046801814, 0.000000000000000000 ) ) ;
#76708=CARTESIAN_POINT ( 'NONE',  ( 5.083381250481017410, 4.895309311841474553, 0.7998128361456352531 ) ) ;
#76721=AXIS2_PLACEMENT_3D ( 'NONE', #83624, #210, #116196 ) ;
#76726=CARTESIAN_POINT ( 'NONE',  ( -7.598418745816086783, 7.829519723065708092, 0.000000000000000000 ) ) ;
#76729=CARTESIAN_POINT ( 'NONE',  ( 5.155843554946782703, 9.237177590738404831, -0.7998128361456481317 ) ) ;
#76742=CARTESIAN_POINT ( 'NONE',  ( 3.106226591306694651, 6.638031766584184368, 0.000000000000000000 ) ) ;
#76747=CARTESIAN_POINT ( 'NONE',  ( 4.095971805104276164, 7.792734516014745871, 0.7216878364870257245 ) ) ;
#76757=CARTESIAN_POINT ( 'NONE',  ( -5.261973015879593873, 8.192700047617899273, 1.082531754730549967 ) ) ;
#76763=CARTESIAN_POINT ( 'NONE',  ( 2.972921499820865066, 6.538163294370741063, -0.5146418828672996160 ) ) ;
#76791=CARTESIAN_POINT ( 'NONE',  ( 4.065465959251388206, 5.836405933916976707, -1.599625672291269396 ) ) ;
#76803=CARTESIAN_POINT ( 'NONE',  ( -5.126391479742927970, 8.994890803093138487, 0.7216878364870267237 ) ) ;
#76806=CARTESIAN_POINT ( 'NONE',  ( 4.055297343818931033, 6.784911763547157193, 1.082531754730549078 ) ) ;
#76824=CARTESIAN_POINT ( 'NONE',  ( -2.862179826260718762, 6.353310540697199471, 0.000000000000000000 ) ) ;
#76827=CARTESIAN_POINT ( 'NONE',  ( 4.217995187182933314, 7.935095128439808576, 0.7216878364870397133 ) ) ;
#76851=CARTESIAN_POINT ( 'NONE',  ( 5.586448450635356444, 5.811331697797319507, -0.7399639515439475623 ) ) ;
#76860=CARTESIAN_POINT ( 'NONE',  ( -5.803772275101700906, 8.928762199997411386, -1.199719254218452047 ) ) ;
#76861=CARTESIAN_POINT ( 'NONE',  ( -4.948302019123040019, 8.085739352127342627, 1.088677458455259650 ) ) ;
#76862=CARTESIAN_POINT ( 'NONE',  ( -4.457598643843001973, 8.422558527783969851, 0.000000000000000000 ) ) ;
#76872=CARTESIAN_POINT ( 'NONE',  ( -4.034433228518296666, 6.864533312316751790, -1.199719254218450271 ) ) ;
#76886=CARTESIAN_POINT ( 'NONE',  ( 5.896870467300973750, 5.844380064798101237, 0.7998128361456352531 ) ) ;
#76906=CARTESIAN_POINT ( 'NONE',  ( 4.044074958626150185, 7.940114228364351767, 0.7998128361456271485 ) ) ;
#76907=CARTESIAN_POINT ( 'NONE',  ( 5.896870467300973750, 5.844380064798101237, 0.7998128361456352531 ) ) ;
#76909=CARTESIAN_POINT ( 'NONE',  ( 3.390420931869152721, 6.113185632892752075, -1.199719254218452047 ) ) ;
#76914=CARTESIAN_POINT ( 'NONE',  ( -3.719872605471121751, 6.605953636083950364, -2.419999999999998597 ) ) ;
#76920=CARTESIAN_POINT ( 'NONE',  ( 5.307274686206796765, 7.744096871513173497, 1.304404211447189876 ) ) ;
#76922=CARTESIAN_POINT ( 'NONE',  ( -3.621436428181653788, 7.239109909604962922, 0.7216878364870338292 ) ) ;
#76952=CARTESIAN_POINT ( 'NONE',  ( 4.523580528814945545, 5.306540700819438960, 1.199719254218452047 ) ) ;
#76960=DIRECTION ( 'NONE',  ( 0.6507913734559640506, -0.7592566023653003482, 0.000000000000000000 ) ) ;
#76971=CARTESIAN_POINT ( 'NONE',  ( -7.469616286486262524, 7.679250187180907794, 0.7998128361456341429 ) ) ;
#76988=CARTESIAN_POINT ( 'NONE',  ( 4.064412189046650248, 7.963840997188264659, 0.7998128361456271485 ) ) ;
#76997=CARTESIAN_POINT ( 'NONE',  ( 6.966220764712121927, 6.002124920821316323, 2.420000000000000373 ) ) ;
#76998=CARTESIAN_POINT ( 'NONE',  ( 5.067666882003905471, 7.850148838107081417, 1.122879199148843377 ) ) ;
#76999=CARTESIAN_POINT ( 'NONE',  ( 5.569000761389712117, 7.517326589397093528, 1.347931912527022158 ) ) ;
#77017=CARTESIAN_POINT ( 'NONE',  ( -5.281783360975562225, 8.319775133516907673, 1.199719254218452935 ) ) ;
#77019=CARTESIAN_POINT ( 'NONE',  ( 4.869313445963426190, 5.709895770826003414, 1.199719254218452935 ) ) ;
#77023=CARTESIAN_POINT ( 'NONE',  ( -6.074935347375019390, 9.245119117649618801, 1.199719254218452047 ) ) ;
#77026=CARTESIAN_POINT ( 'NONE',  ( 5.989670002187236442, 10.20997511251894529, -0.7998128361456481317 ) ) ;
#77027=DIRECTION ( 'NONE',  ( 0.7592566023653005702, 0.6507913734559639396, 0.000000000000000000 ) ) ;
#77033=CARTESIAN_POINT ( 'NONE',  ( -5.426384371074921553, 7.636973626576035734, -1.343385757368668498 ) ) ;
#77051=CARTESIAN_POINT ( 'NONE',  ( 6.211043768836185031, 6.418841616496599123, 0.7216878364870328300 ) ) ;
#77065=CARTESIAN_POINT ( 'NONE',  ( -3.933273961740340496, 5.682181936820735579, 1.443375672974065660 ) ) ;
#77071=CARTESIAN_POINT ( 'NONE',  ( 5.520104819419390907, 6.469152373191302985, 1.199719254218452935 ) ) ;
#77096=DIRECTION ( 'NONE',  ( 0.000000000000000000, -1.000000000000000000, 0.000000000000000000 ) ) ;
#77102=EDGE_CURVE ( 'NONE', #110637, #26075, #93182, .T. ) ;
#77111=CARTESIAN_POINT ( 'NONE',  ( -4.970620135051034616, 8.062850052469723749, -1.111334424012894617 ) ) ;
#77115=CARTESIAN_POINT ( 'NONE',  ( -5.666381855868691808, 5.575476684793721383, 0.000000000000000000 ) ) ;
#77120=CARTESIAN_POINT ( 'NONE',  ( 4.913904330310220558, 4.697586238308844919, 0.000000000000000000 ) ) ;
#77124=CARTESIAN_POINT ( 'NONE',  ( -5.289089322662584358, 5.343228095960675716, 0.000000000000000000 ) ) ;
#77133=CARTESIAN_POINT ( 'NONE',  ( -5.123001941117347080, 7.070197912760590064, 1.599625672291263179 ) ) ;
#77142=CARTESIAN_POINT ( 'NONE',  ( -5.655686355556086120, 6.627330832017406692, 1.199719254218452935 ) ) ;
#77144=CARTESIAN_POINT ( 'NONE',  ( 6.272253174914359519, 6.990222103910356921, -0.9563742486745248073 ) ) ;
#77149=CARTESIAN_POINT ( 'NONE',  ( 4.193214648376505593, 8.114110533073061404, 0.000000000000000000 ) ) ;
#77154=CARTESIAN_POINT ( 'NONE',  ( -5.752402313948099533, 9.933162809573264695, -0.7998128361456362523 ) ) ;
#77159=CARTESIAN_POINT ( 'NONE',  ( -4.274563570058511175, 8.209017608368725405, 0.000000000000000000 ) ) ;
#77163=CARTESIAN_POINT ( 'NONE',  ( 4.217995187182915551, 7.935095128439824563, 0.7216878364870257245 ) ) ;
#77164=CARTESIAN_POINT ( 'NONE',  ( -4.760321331729590710, 8.567808963744235839, 0.7216878364870267237 ) ) ;
#77168=CARTESIAN_POINT ( 'NONE',  ( -6.473091995881817162, 6.516638514809040217, 0.7998128361456282587 ) ) ;
#77171=CARTESIAN_POINT ( 'NONE',  ( 4.369470645354133431, 8.319742529546998000, 0.7998128361456271485 ) ) ;
#77191=CARTESIAN_POINT ( 'NONE',  ( -3.011287625495571607, 6.360174617139689346, -0.7852620323503290978 ) ) ;
#77200=CARTESIAN_POINT ( 'NONE',  ( 5.176795123377851304, 7.746134302493202561, 1.185296789734613387 ) ) ;
#77208=CARTESIAN_POINT ( 'NONE',  ( 6.668631453075247073, 8.873432343378178544, -1.599625672291281386 ) ) ;
#77213=CARTESIAN_POINT ( 'NONE',  ( -4.740694425254917910, 8.216228820413899570, 0.6995903363472668612 ) ) ;
#77219=CARTESIAN_POINT ( 'NONE',  ( -7.456058132872594335, 7.663432341298296535, 0.000000000000000000 ) ) ;
#77230=CARTESIAN_POINT ( 'NONE',  ( -6.074935347375019390, 9.245119117649618801, 1.199719254218452047 ) ) ;
#77232=CARTESIAN_POINT ( 'NONE',  ( 6.176621499477501054, 9.363752961769195693, -1.199719254218452047 ) ) ;
#77240=ORIENTED_EDGE ( 'NONE', *, *, #202906, .F. ) ;
#77242=CARTESIAN_POINT ( 'NONE',  ( 3.553118775233146120, 6.302999783484076524, -1.199719254218453823 ) ) ;
#77245=CARTESIAN_POINT ( 'NONE',  ( 6.170369307550831017, 6.371388078330353366, 0.7216878364870328300 ) ) ;
#77255=CARTESIAN_POINT ( 'NONE',  ( -5.865985541149716376, 7.193105608424513520, 1.152625159504708119 ) ) ;
#77256=EDGE_CURVE ( 'NONE', #160913, #149147, #191038, .T. ) ;
#77264=CARTESIAN_POINT ( 'NONE',  ( -2.986538976760251263, 6.706322249520737522, -0.7998128361456481317 ) ) ;
#77265=CARTESIAN_POINT ( 'NONE',  ( 6.780486220610169035, 9.003929572168926754, -1.443375672974078761 ) ) ;
#77277=ORIENTED_EDGE ( 'NONE', *, *, #24605, .T. ) ;
#77278=CARTESIAN_POINT ( 'NONE',  ( -7.598418745816086783, 7.829519723065708092, 0.000000000000000000 ) ) ;
#77279=CARTESIAN_POINT ( 'NONE',  ( -6.283277845290492714, 6.295188672452495915, -0.7998128361456362523 ) ) ;
#77281=CARTESIAN_POINT ( 'NONE',  ( 6.116136693096175136, 9.189224337703940648, -1.082531754730548412 ) ) ;
#77283=ORIENTED_EDGE ( 'NONE', *, *, #39803, .T. ) ;
#77290=DIRECTION ( 'NONE',  ( -0.8271092603132983445, -0.5620411653108593475, 3.452101583626667318E-12 ) ) ;
#77294=CARTESIAN_POINT ( 'NONE',  ( -6.348239482750515528, 6.857177101084271698, -0.6483580952693357435 ) ) ;
#77295=CARTESIAN_POINT ( 'NONE',  ( -3.188928480291426837, 8.980740528189164351, -2.451733079074508659 ) ) ;
#77299=CARTESIAN_POINT ( 'NONE',  ( 5.234856708652227297, 7.200695141551334721, 1.443375672974065660 ) ) ;
#77300=CARTESIAN_POINT ( 'NONE',  ( -2.428612866367529932E-14, 2.999999999999999112, 2.420000000000000373 ) ) ;
#77304=CARTESIAN_POINT ( 'NONE',  ( -6.149505192250180663, 9.332117270003974951, -1.199719254218452047 ) ) ;
#77319=CARTESIAN_POINT ( 'NONE',  ( 7.028976294042106332, 7.165170195996068969, 0.000000000000000000 ) ) ;
#77330=EDGE_CURVE ( 'NONE', #82462, #90832, #109124, .T. ) ;
#77345=ORIENTED_EDGE ( 'NONE', *, *, #70182, .T. ) ;
#77354=CARTESIAN_POINT ( 'NONE',  ( 3.230585741806197841, 6.991043475407723307, 0.7998128361456271485 ) ) ;
#77382=CARTESIAN_POINT ( 'NONE',  ( -3.980200614063634568, 6.801261928786307642, 1.199719254218452935 ) ) ;
#77384=CARTESIAN_POINT ( 'NONE',  ( 6.685579144870162693, 6.972466221869550118, -0.7216878364870458196 ) ) ;
#77389=CARTESIAN_POINT ( 'NONE',  ( -5.978219388983010418, 5.939287140093762574, -0.7998128361456362523 ) ) ;
#77395=CARTESIAN_POINT ( 'NONE',  ( -5.646044625448194410, 5.551749915969804938, 0.000000000000000000 ) ) ;
#77402=CARTESIAN_POINT ( 'NONE',  ( -5.478376588373717659, 8.549133898814758936, -1.199719254218452047 ) ) ;
#77412=CARTESIAN_POINT ( 'NONE',  ( -3.447516199624892419, 7.244129009529488350, 0.7998128361456352531 ) ) ;
#77417=CARTESIAN_POINT ( 'NONE',  ( -6.780486220610195680, 7.083191143566240910, -0.7216878364870338292 ) ) ;
#77418=CARTESIAN_POINT ( 'NONE',  ( -6.089020385868867180, 7.236850217336030511, -1.082531754730549967 ) ) ;
#77419=CARTESIAN_POINT ( 'NONE',  ( 7.225569521440261767, 7.394528961293920233, -0.7998128361456341429 ) ) ;
#77420=CARTESIAN_POINT ( 'NONE',  ( -6.903036488013351679, 8.082572653217566128, -1.199719254218452047 ) ) ;
#77444=CARTESIAN_POINT ( 'NONE',  ( -5.346851039111044201, 6.199209027673978412, 7.500000000000000000 ) ) ;
#77457=CARTESIAN_POINT ( 'NONE',  ( 4.648548116941726427, 8.423941524322412278, -0.4686463081053967583 ) ) ;
#77471=CARTESIAN_POINT ( 'NONE',  ( 5.525830126021535449, 8.604496359403894346, -1.199719254218452047 ) ) ;
#77478=CARTESIAN_POINT ( 'NONE',  ( -5.926322542504864899, 8.967774495347393682, -1.082531754730549967 ) ) ;
#77489=CARTESIAN_POINT ( 'NONE',  ( 3.923105346307896202, 5.670318552149568703, -1.599625672291269396 ) ) ;
#77490=CARTESIAN_POINT ( 'NONE',  ( 4.857564175446106525, 8.889184981320973122, 0.7998128361456331437 ) ) ;
#77504=CARTESIAN_POINT ( 'NONE',  ( 5.525830126021535449, 8.604496359403894346, -1.199719254218452047 ) ) ;
#77518=CARTESIAN_POINT ( 'NONE',  ( -4.177320726786319049, 6.927272377009067839, -1.082531754730551743 ) ) ;
#77519=CARTESIAN_POINT ( 'NONE',  ( -7.611976899429754084, 7.845337568948314022, 0.7998128361456341429 ) ) ;
#77525=EDGE_LOOP ( 'NONE', ( #45701, #119190, #167210, #64552 ) ) ;
#77529=VERTEX_POINT ( 'NONE', #16133 ) ;
#77530=CARTESIAN_POINT ( 'NONE',  ( -2.810282979782591006, 6.500690253046801814, 0.000000000000000000 ) ) ;
#77531=CARTESIAN_POINT ( 'NONE',  ( 7.212011367826596242, 7.378711115411311638, 0.000000000000000000 ) ) ;
#77534=CARTESIAN_POINT ( 'NONE',  ( 7.014364370223726830, 9.276787413384745662, -1.599625672291269396 ) ) ;
#77552=CARTESIAN_POINT ( 'NONE',  ( 3.400062661977048428, 7.188766548940353829, -1.734723475976807094E-15 ) ) ;
#77555=AXIS2_PLACEMENT_3D ( 'NONE', #40081, #88841, #159153 ) ;
#77558=CARTESIAN_POINT ( 'NONE',  ( 4.712340909201580885, 7.655425606447271214, -1.199719254218452047 ) ) ;
#77569=CARTESIAN_POINT ( 'NONE',  ( 6.916067756746836714, 8.201738816693689316, -1.082531754730548412 ) ) ;
#77571=CARTESIAN_POINT ( 'NONE',  ( -7.117104292530948229, 7.267986194233038155, -0.7998128361456362523 ) ) ;
#77572=CARTESIAN_POINT ( 'NONE',  ( 6.229045230835819069, 6.231917288922055320, -0.7998128361456481317 ) ) ;
#77582=CARTESIAN_POINT ( 'NONE',  ( -3.949167883330528372, 7.829389307186077396, 1.214306433183764966E-14 ) ) ;
#77616=CARTESIAN_POINT ( 'NONE',  ( 3.567203813726958828, 6.215469311773181182, 1.082531754730549078 ) ) ;
#77628=CARTESIAN_POINT ( 'NONE',  ( -3.806807270387036368, 7.663301925418665839, 0.000000000000000000 ) ) ;
#77630=CARTESIAN_POINT ( 'NONE',  ( -5.966470118465691641, 9.118576350588734059, -1.199719254218452047 ) ) ;
#77632=CARTESIAN_POINT ( 'NONE',  ( 6.495764994278795612, 9.632124022417032805, 1.082531754730549078 ) ) ;
#77642=CARTESIAN_POINT ( 'NONE',  ( -5.074494633264801990, 9.142270515442742607, 0.7998128361456291469 ) ) ;
#77649=CARTESIAN_POINT ( 'NONE',  ( -3.526529353330350336, 7.128384988945109413, -0.7216878364870458196 ) ) ;
#77653=CARTESIAN_POINT ( 'NONE',  ( -3.772911886352873445, 7.623757310712140800, 0.7998128361456352531 ) ) ;
#77662=CARTESIAN_POINT ( 'NONE',  ( -6.462464340777758665, 6.712165690604718016, -0.3031571887801186027 ) ) ;
#77674=CARTESIAN_POINT ( 'NONE',  ( -5.257529707049291900, 9.355811434857983500, 0.7998128361456291469 ) ) ;
#77675=DIRECTION ( 'NONE',  ( 1.000000000000000000, 0.000000000000000000, 0.000000000000000000 ) ) ;
#77676=CARTESIAN_POINT ( 'NONE',  ( -4.411198876399886615, 6.239761003923544713, -1.599625672291271394 ) ) ;
#77702=CARTESIAN_POINT ( 'NONE',  ( -6.282224075085783177, 8.422623735723785643, 1.599625672291269396 ) ) ;
#77730=CARTESIAN_POINT ( 'NONE',  ( 8.005163354226054295, 8.304055099544019214, 0.000000000000000000 ) ) ;
#77735=CIRCLE ( 'NONE', #209136, 0.4800000000000000933 ) ;
#77743=CARTESIAN_POINT ( 'NONE',  ( 5.417061852544872380, 7.532864896096530316, 1.248242807326222392 ) ) ;
#77745=CARTESIAN_POINT ( 'NONE',  ( 5.234856708652215751, 9.121433570154021453, 0.7216878364870317197 ) ) ;
#77752=CARTESIAN_POINT ( 'NONE',  ( -4.878955176071358757, 6.785476686873604280, -1.599625672291271394 ) ) ;
#77758=CARTESIAN_POINT ( 'NONE',  ( -7.390603132780803719, 7.794994207765291172, -0.7216878364870338292 ) ) ;
#77762=CARTESIAN_POINT ( 'NONE',  ( 5.072905659164107739, 4.910989440906482706, -0.2235617647182771561 ) ) ;
#77765=VECTOR ( 'NONE', #61582, 1000.000000000000114 ) ;
#77769=CARTESIAN_POINT ( 'NONE',  ( -4.767627293860968507, 5.591261926706423857, -1.199719254218453823 ) ) ;
#77779=CARTESIAN_POINT ( 'NONE',  ( 7.614839552730775729, 8.913009562054615031, 1.199719254218452047 ) ) ;
#77798=CARTESIAN_POINT ( 'NONE',  ( -6.912678218121246942, 9.158153569265168770, 1.599625672291269396 ) ) ;
#77800=CARTESIAN_POINT ( 'NONE',  ( 6.587282531393223728, 8.778525268082516320, 1.599625672291268286 ) ) ;
#77802=CARTESIAN_POINT ( 'NONE',  ( -5.425839481171796486, 7.540841100536294306, 1.248335065278019629 ) ) ;
#77808=CARTESIAN_POINT ( 'NONE',  ( 6.150558962454855561, 7.204682206732687000, 1.199719254218452047 ) ) ;
#77819=CARTESIAN_POINT ( 'NONE',  ( 4.529832720741620022, 7.338536369956936589, -1.082531754730548412 ) ) ;
#77830=CARTESIAN_POINT ( 'NONE',  ( -6.292392690518223475, 6.513748691792265788, -0.7216878364870338292 ) ) ;
#77863=CARTESIAN_POINT ( 'NONE',  ( 3.867818961648523235, 7.734482231890414283, 1.040834085586084257E-14 ) ) ;
#77877=CARTESIAN_POINT ( 'NONE',  ( -6.238160076063538284, 9.331584951165851294, 1.082531754730549967 ) ) ;
#77880=CARTESIAN_POINT ( 'NONE',  ( 5.031484404002891431, 5.042689024191078673, 0.7216878364870328300 ) ) ;
#77886=EDGE_CURVE ( 'NONE', #9659, #211508, #88339, .T. ) ;
#77897=CARTESIAN_POINT ( 'NONE',  ( -3.363831509966363598, 5.978201624052440266, -1.082531754730548412 ) ) ;
#77903=EDGE_CURVE ( 'NONE', #35911, #105939, #63189, .T. ) ;
#77935=CARTESIAN_POINT ( 'NONE',  ( -4.762965077474956566, 8.286028185285090331, 0.8196324637163689975 ) ) ;
#77936=CARTESIAN_POINT ( 'NONE',  ( -5.607897038807837298, 5.667647723685407257, 0.4330508580119977746 ) ) ;
#77937=CARTESIAN_POINT ( 'NONE',  ( -4.969177613625957335, 8.005234357488689056, 1.071350258858670967 ) ) ;
#77938=ORIENTED_EDGE ( 'NONE', *, *, #180702, .T. ) ;
#77940=DIRECTION ( 'NONE',  ( 0.9446243521954068578, 0.000000000000000000, 0.3281536732072456997 ) ) ;
#77943=CARTESIAN_POINT ( 'NONE',  ( -3.169574050544739841, 6.919863168935977527, -0.7998128361456481317 ) ) ;
#77946=CARTESIAN_POINT ( 'NONE',  ( -3.494969737272722643, 7.299491470118629088, -0.7998128361456481317 ) ) ;
#77959=CARTESIAN_POINT ( 'NONE',  ( 3.901714345682657292, 7.774026846596938434, 0.7998128361456271485 ) ) ;
#77964=DIRECTION ( 'NONE',  ( -0.000000000000000000, -1.000000000000000000, -0.000000000000000000 ) ) ;
#77981=EDGE_CURVE ( 'NONE', #89251, #22085, #101210, .T. ) ;
#77982=CARTESIAN_POINT ( 'NONE',  ( 5.285699784481295183, 7.260012063351913625, 1.599625672291268286 ) ) ;
#77983=CARTESIAN_POINT ( 'NONE',  ( 3.736153849017632922, 6.516540702899320081, -1.199719254218453823 ) ) ;
#77985=CARTESIAN_POINT ( 'NONE',  ( 5.401997860402196316, 5.267028690082820930, 0.000000000000000000 ) ) ;
#77997=CARTESIAN_POINT ( 'NONE',  ( -2.973958751752119767, 6.684155243576896943, 0.05118324351628460861 ) ) ;
#77998=CARTESIAN_POINT ( 'NONE',  ( 5.126881573038487794, 7.911131357477594328, 1.221340741751137493 ) ) ;
#77999=CARTESIAN_POINT ( 'NONE',  ( -5.614485009390564940, 5.722856397143323726, 0.000000000000000000 ) ) ;
#78006=DIRECTION ( 'NONE',  ( 0.6507913734559640506, -0.7592566023653003482, 0.000000000000000000 ) ) ;
#78019=CARTESIAN_POINT ( 'NONE',  ( -0.4000000000000243916, 3.000000000000566214, -2.023857702507757317 ) ) ;
#78026=CARTESIAN_POINT ( 'NONE',  ( 2.878073747850912412, 6.579779482459851003, -0.7998128361456362523 ) ) ;
#78046=CARTESIAN_POINT ( 'NONE',  ( -5.447343857640614573, 9.577261277214532242, -0.7998128361456362523 ) ) ;
#78063=CARTESIAN_POINT ( 'NONE',  ( 6.008198349511364000, 7.038594824965278995, 1.199719254218453823 ) ) ;
#78074=CARTESIAN_POINT ( 'NONE',  ( 4.702859892337409420, 8.240897811179339172, 0.6291740908887258898 ) ) ;
#78092=CARTESIAN_POINT ( 'NONE',  ( -6.306477729012051725, 7.386587434382707151, 1.199719254218452047 ) ) ;
#78094=CARTESIAN_POINT ( 'NONE',  ( 6.222266154028957885, 6.224008365980749247, 0.7998128361456352531 ) ) ;
#78098=CARTESIAN_POINT ( 'NONE',  ( -5.912237504011027767, 9.055304967058290799, 1.199719254218454489 ) ) ;
#78102=DIRECTION ( 'NONE',  ( -1.000000000000000000, 0.000000000000000000, 0.000000000000000000 ) ) ;
#78106=CARTESIAN_POINT ( 'NONE',  ( -5.058680321808019187, 7.974527835229765493, -1.188367278328520849 ) ) ;
#78122=CARTESIAN_POINT ( 'NONE',  ( 5.234856708652227297, 7.200695141551334721, 1.443375672974065660 ) ) ;
#78141=CARTESIAN_POINT ( 'NONE',  ( 5.357406976055401948, 6.279338222599979424, 1.199719254218452935 ) ) ;
#78147=LINE ( 'NONE', #62962, #135880 ) ;
#78171=ORIENTED_EDGE ( 'NONE', *, *, #157556, .T. ) ;
#78180=DIRECTION ( 'NONE',  ( -0.6292706268317891372, -0.7771862570881751253, 0.000000000000000000 ) ) ;
#78194=CARTESIAN_POINT ( 'NONE',  ( -5.600926855776901192, 5.707038551260711579, -0.7216878364870338292 ) ) ;
#78198=DIRECTION ( 'NONE',  ( 0.000000000000000000, 0.000000000000000000, -1.000000000000000000 ) ) ;
#78200=CARTESIAN_POINT ( 'NONE',  ( -3.949167883330528372, 7.829389307186077396, 1.214306433183764966E-14 ) ) ;
#78206=ORIENTED_EDGE ( 'NONE', *, *, #142525, .F. ) ;
#78210=CARTESIAN_POINT ( 'NONE',  ( -5.815521545619021460, 5.749472989502435460, -0.7998128361456362523 ) ) ;
#78212=CARTESIAN_POINT ( 'NONE',  ( 5.602183562003149042, 7.492195738860313092, 1.335281325244306982 ) ) ;
#78218=CARTESIAN_POINT ( 'NONE',  ( 5.448397627845284141, 7.449826213943242514, 1.599625672291268286 ) ) ;
#78225=CARTESIAN_POINT ( 'NONE',  ( -3.923105346307911745, 5.670318552149568703, -1.599625672291283607 ) ) ;
#78230=CARTESIAN_POINT ( 'NONE',  ( -6.473091995881817162, 6.516638514809040217, 0.7998128361456281477 ) ) ;
#78234=CARTESIAN_POINT ( 'NONE',  ( 5.194182247366861738, 9.073980031987776584, 0.7216878364870317197 ) ) ;
#78236=CARTESIAN_POINT ( 'NONE',  ( -6.766928066552171828, 7.067373297165212342, 0.7216878364870317197 ) ) ;
#78240=CARTESIAN_POINT ( 'NONE',  ( -4.437261413422502798, 8.398831758960053406, 0.000000000000000000 ) ) ;
#78243=CARTESIAN_POINT ( 'NONE',  ( 5.041653019435334393, 6.975290837464928728, -1.599625672291269396 ) ) ;
#78249=CARTESIAN_POINT ( 'NONE',  ( 6.527324610336439292, 6.579909898339485252, 0.7998128361456332547 ) ) ;
#78269=CARTESIAN_POINT ( 'NONE',  ( 4.625518323863472503, 8.335144253906971556, 0.3473850511846506839 ) ) ;
#78276=CARTESIAN_POINT ( 'NONE',  ( 7.126746022638799971, 8.343567110280638133, 1.199719254218452047 ) ) ;
#78281=CARTESIAN_POINT ( 'NONE',  ( -4.624779211906307808, 8.357533986720639518, 0.2900094174717957607 ) ) ;
#78287=CARTESIAN_POINT ( 'NONE',  ( -4.136646265500970365, 5.919449624541475607, -1.443375672974066548 ) ) ;
#78299=CARTESIAN_POINT ( 'NONE',  ( -4.248501033035892327, 6.049946853332221153, -1.599625672291271394 ) ) ;
#78301=CARTESIAN_POINT ( 'NONE',  ( 5.501576472095266901, 9.640532660744973725, -0.7998128361456481317 ) ) ;
#78304=( BOUNDED_CURVE ( )  B_SPLINE_CURVE ( 2, ( #160509, #192991, #77115, #80321, #96603 ),
 .UNSPECIFIED., .F., .T. ) 
 B_SPLINE_CURVE_WITH_KNOTS ( ( 3, 2, 3 ),
 ( 0.2225013972065820467, 0.2250000000000000056, 0.2278796248419688031 ),
 .UNSPECIFIED. ) 
 CURVE ( )  GEOMETRIC_REPRESENTATION_ITEM ( )  RATIONAL_B_SPLINE_CURVE ( ( 0.9437486473799283626, 0.9598300839578506327, 1.000000000000000000, 0.9537044109453918228, 0.9394041646864383921 ) ) 
 REPRESENTATION_ITEM ( '' )  );
#78308=ORIENTED_EDGE ( 'NONE', *, *, #28350, .T. ) ;
#78310=CARTESIAN_POINT ( 'NONE',  ( 6.150558962454855561, 7.204682206732687000, 1.199719254218452047 ) ) ;
#78313=CARTESIAN_POINT ( 'NONE',  ( 5.356880090730872013, 6.382686539675070492, 1.082531754730549078 ) ) ;
#78321=DIRECTION ( 'NONE',  ( 0.7592566023653005702, -0.6507913734559639396, 0.000000000000000000 ) ) ;
#78322=CARTESIAN_POINT ( 'NONE',  ( -6.501436840734760914, 6.757938919538193367, -0.04654198066046839888 ) ) ;
#78324=AXIS2_PLACEMENT_3D ( 'NONE', #198763, #183597, #118669 ) ;
#78331=CARTESIAN_POINT ( 'NONE',  ( -5.320648938720212051, 5.172121614787156929, 0.000000000000000000 ) ) ;
#78332=CARTESIAN_POINT ( 'NONE',  ( 5.885648082108177803, 9.880690172519326353, 0.7216878364870317197 ) ) ;
#78339=VERTEX_POINT ( 'NONE', #119058 ) ;
#78341=ORIENTED_EDGE ( 'NONE', *, *, #72882, .T. ) ;
#78342=CARTESIAN_POINT ( 'NONE',  ( -4.762657100150483380, 8.778460060142702304, 0.000000000000000000 ) ) ;
#78343=CARTESIAN_POINT ( 'NONE',  ( -4.827585214917754719, 7.789877296449459365, -1.199719254218453823 ) ) ;
#78345=CARTESIAN_POINT ( 'NONE',  ( 6.577113915960825175, 8.766661883411348555, -1.443375672974078761 ) ) ;
#78357=CARTESIAN_POINT ( 'NONE',  ( -6.444026653998019327, 6.794751805161505231, -0.4079633569072909638 ) ) ;
#78367=CARTESIAN_POINT ( 'NONE',  ( -7.781453819600577582, 8.043060642480948985, 0.000000000000000000 ) ) ;
#78384=CARTESIAN_POINT ( 'NONE',  ( 6.692885107001518286, 7.837396042037102717, -1.199719254218452047 ) ) ;
#78409=ORIENTED_EDGE ( 'NONE', *, *, #81748, .F. ) ;
#78414=DIRECTION ( 'NONE',  ( 0.000000000000000000, 1.000000000000000000, 0.000000000000000000 ) ) ;
#78418=CARTESIAN_POINT ( 'NONE',  ( 3.217027588192558074, 6.975225629525113824, -1.734723475976807094E-15 ) ) ;
#78449=CARTESIAN_POINT ( 'NONE',  ( -5.224688093219839402, 7.188831756880171397, -1.599625672291271394 ) ) ;
#78451=CARTESIAN_POINT ( 'NONE',  ( 7.322812364712459221, 7.715904978352238430, 0.000000000000000000 ) ) ;
#78456=CARTESIAN_POINT ( 'NONE',  ( -4.132202957115018727, 8.042930226601317401, 0.000000000000000000 ) ) ;
#78461=CARTESIAN_POINT ( 'NONE',  ( -4.442231607132987925, 5.211633625523774960, -1.199719254218453823 ) ) ;
#78467=CARTESIAN_POINT ( 'NONE',  ( -4.111865726694519552, 8.019203457777400956, 0.000000000000000000 ) ) ;
#78477=CARTESIAN_POINT ( 'NONE',  ( -3.474632506852224356, 7.275764701294714420, -0.7998128361456481317 ) ) ;
#78482=CARTESIAN_POINT ( 'NONE',  ( -6.631346530859867805, 6.909194838857525944, 0.000000000000000000 ) ) ;
#78483=CARTESIAN_POINT ( 'NONE',  ( -6.739811759324831897, 7.996106819701333634, -1.082531754730549967 ) ) ;
#78484=CARTESIAN_POINT ( 'NONE',  ( 7.212011367826596242, 7.378711115411311638, 0.000000000000000000 ) ) ;
#78485=CARTESIAN_POINT ( 'NONE',  ( -5.433785704026946384, 9.561443431331920095, 0.000000000000000000 ) ) ;
#78503=CARTESIAN_POINT ( 'NONE',  ( -1.853343808665687931, 2.488708180678084414, -2.484983702926222726 ) ) ;
#78522=CARTESIAN_POINT ( 'NONE',  ( 4.701115458738250652, 8.361069499448168685, -0.6471830670988186762 ) ) ;
#78536=CARTESIAN_POINT ( 'NONE',  ( 6.984385409695311964, 8.177479728513226576, 1.199719254218452935 ) ) ;
#78539=CARTESIAN_POINT ( 'NONE',  ( -4.305596300791617814, 7.180890229968955651, 1.199719254218452935 ) ) ;
#78543=CARTESIAN_POINT ( 'NONE',  ( -5.261973015435229328, 9.153069261400824885, 0.000000000000000000 ) ) ;
#78554=CARTESIAN_POINT ( 'NONE',  ( 3.061108821635398769, 6.793320401875094561, -0.7998128361456362523 ) ) ;
#78555=CARTESIAN_POINT ( 'NONE',  ( 5.071631979963703962, 8.074598522336444262, 1.199719254218451159 ) ) ;
#78569=CARTESIAN_POINT ( 'NONE',  ( 5.688527969385528849, 8.794310509995222347, -1.199719254218452047 ) ) ;
#78581=CARTESIAN_POINT ( 'NONE',  ( -4.285785955695645910, 7.053815144069948140, 1.082531754730549967 ) ) ;
#78582=CARTESIAN_POINT ( 'NONE',  ( -6.454563648557663846, 9.688018802362710957, -1.199719254218452047 ) ) ;
#78588=ORIENTED_EDGE ( 'NONE', *, *, #204577, .T. ) ;
#78596=CARTESIAN_POINT ( 'NONE',  ( 6.068156270568149324, 9.237210194708310951, 1.199719254218452047 ) ) ;
#78599=CARTESIAN_POINT ( 'NONE',  ( 6.502017186205484300, 9.743381262951846367, -1.199719254218452047 ) ) ;
#78614=CARTESIAN_POINT ( 'NONE',  ( 6.900173834712277632, 7.014900660111269559, -0.7998128361456341429 ) ) ;
#78616=CARTESIAN_POINT ( 'NONE',  ( -4.411198876399886615, 6.239761003923544713, -1.599625672291271394 ) ) ;
#78620=CARTESIAN_POINT ( 'NONE',  ( 5.737035277238070385, 6.722237907313067140, -1.199719254218452047 ) ) ;
#78629=CARTESIAN_POINT ( 'NONE',  ( 5.546694241766559230, 9.485244025454063532, 0.000000000000000000 ) ) ;
#78631=CARTESIAN_POINT ( 'NONE',  ( -7.795011973214244883, 8.058878488363559356, 0.7998128361456341429 ) ) ;
#78632=CARTESIAN_POINT ( 'NONE',  ( 3.555981428534177091, 7.370671776590375757, 0.7998128361456271485 ) ) ;
#78641=CARTESIAN_POINT ( 'NONE',  ( -4.716257332707368910, 6.595662536282280719, -1.599625672291271394 ) ) ;
#78659=ORIENTED_EDGE ( 'NONE', *, *, #210003, .F. ) ;
#78670=CARTESIAN_POINT ( 'NONE',  ( 3.607878275012302627, 7.223292064240769861, 0.7216878364870257245 ) ) ;
#78676=CARTESIAN_POINT ( 'NONE',  ( 4.380693030546913391, 7.164540064729805202, 1.082531754730549078 ) ) ;
#78689=CARTESIAN_POINT ( 'NONE',  ( -7.279802135894939852, 7.457800344824362604, -0.7998128361456362523 ) ) ;
#78691=CARTESIAN_POINT ( 'NONE',  ( -5.915100157312088491, 10.12297696016459092, -0.7998128361456362523 ) ) ;
#78702=CARTESIAN_POINT ( 'NONE',  ( -6.798487682609798632, 6.896266815991691779, 0.7998128361456341429 ) ) ;
#78708=CARTESIAN_POINT ( 'NONE',  ( -5.153507786970276783, 6.145418851954329575, -1.082531754730549967 ) ) ;
#78712=CARTESIAN_POINT ( 'NONE',  ( -5.255720823952942489, 6.160704378480398979, -1.199719254218453823 ) ) ;
#78733=CARTESIAN_POINT ( 'NONE',  ( -7.279802135894939852, 7.457800344824362604, -0.7998128361456362523 ) ) ;
#78736=CARTESIAN_POINT ( 'NONE',  ( -5.842637852846353397, 5.781108681267656202, 0.7998128361456281477 ) ) ;
#78745=CARTESIAN_POINT ( 'NONE',  ( 5.031484404002879884, 6.963427452793765404, 1.443375672974065660 ) ) ;
#78761=CARTESIAN_POINT ( 'NONE',  ( -5.108390017298964914, 9.181815130149269422, 0.000000000000000000 ) ) ;
#78787=CARTESIAN_POINT ( 'NONE',  ( 6.424584688029230328, 8.588711117491191871, 1.599625672291268286 ) ) ;
#78799=CARTESIAN_POINT ( 'NONE',  ( 5.916355900263067014, 7.140870225795406867, 1.119544393390920600 ) ) ;
#78801=CARTESIAN_POINT ( 'NONE',  ( 6.048345925472178308, 9.110135108809304327, 1.082531754730549967 ) ) ;
#78807=CARTESIAN_POINT ( 'NONE',  ( -4.125423880308188629, 8.035021303660014880, -0.7998128361456481317 ) ) ;
#78810=AXIS2_PLACEMENT_3D ( 'NONE', #207538, #26655, #143663 ) ;
#78814=CARTESIAN_POINT ( 'NONE',  ( -6.631346530415505036, 7.869564052640446228, 1.082531754730549078 ) ) ;
#78817=CARTESIAN_POINT ( 'NONE',  ( -4.000897611406796450, 7.681767652865702622, 0.01012816533798947816 ) ) ;
#78821=EDGE_CURVE ( 'NONE', #99737, #127411, #150332, .T. ) ;
#78823=CARTESIAN_POINT ( 'NONE',  ( -5.157951095356222204, 4.982307464195829816, 0.000000000000000000 ) ) ;
#78833=CARTESIAN_POINT ( 'NONE',  ( 6.373214726875630731, 9.593111727067046957, 1.199719254218452047 ) ) ;
#78837=EDGE_LOOP ( 'NONE', ( #28212, #4227, #60892, #64086 ) ) ;
#78850=VERTEX_POINT ( 'NONE', #96416 ) ;
#78855=CARTESIAN_POINT ( 'NONE',  ( 5.668190738965027897, 8.770583741171307679, -1.199719254218452047 ) ) ;
#78857=CARTESIAN_POINT ( 'NONE',  ( -5.488562097922137895, 7.488332829134150437, 1.250156803814896245 ) ) ;
#78864=CARTESIAN_POINT ( 'NONE',  ( 5.041653019435334393, 6.975290837464928728, -1.599625672291269396 ) ) ;
#78867=CARTESIAN_POINT ( 'NONE',  ( -5.584636475198561989, 5.818617271341436137, -0.4844363064898093429 ) ) ;
#78871=CARTESIAN_POINT ( 'NONE',  ( 4.095971805104288599, 5.871996087412059140, 1.443375672974058777 ) ) ;
#78875=CARTESIAN_POINT ( 'NONE',  ( 5.153507786970260796, 7.105788066255672497, -1.443375672974078761 ) ) ;
#78886=CARTESIAN_POINT ( 'NONE',  ( -5.478903473698255588, 7.485416367438324059, -1.443375672974066548 ) ) ;
#78898=AXIS2_PLACEMENT_3D ( 'NONE', #176678, #44563, #78102 ) ;
#78920=CARTESIAN_POINT ( 'NONE',  ( 4.505052181490820651, 8.477920988373101707, -0.7998128361456381397 ) ) ;
#78922=CARTESIAN_POINT ( 'NONE',  ( 5.956828388357757298, 8.042995434541133193, 1.599625672291269396 ) ) ;
#78934=CARTESIAN_POINT ( 'NONE',  ( -7.431277594066152403, 8.802816960232885179, -1.082531754730549967 ) ) ;
#78937=CARTESIAN_POINT ( 'NONE',  ( 3.377389663135653031, 6.954388683717978026, -0.7216878364870338292 ) ) ;
#78945=ADVANCED_FACE ( 'NONE', ( #130037 ), #111290, .T. ) ;
#78954=CARTESIAN_POINT ( 'NONE',  ( -4.489158259900630554, 8.251452046610447510, 0.000000000000000000 ) ) ;
#78956=CARTESIAN_POINT ( 'NONE',  ( -4.177320726786319049, 6.927272377009067839, -1.082531754730551743 ) ) ;
#78957=CARTESIAN_POINT ( 'NONE',  ( 4.234574664202256145, 7.152588777595761727, 1.178691574056603075 ) ) ;
#78959=CARTESIAN_POINT ( 'NONE',  ( 4.204437033569277560, 7.919277282557212416, 0.000000000000000000 ) ) ;
#78974=ORIENTED_EDGE ( 'NONE', *, *, #45594, .T. ) ;
#78996=CARTESIAN_POINT ( 'NONE',  ( -5.901542003698421190, 10.10715911428198055, 0.000000000000000000 ) ) ;
#78997=CARTESIAN_POINT ( 'NONE',  ( -4.618765760061220860, 8.456409177651165621, 0.3783674834792974950 ) ) ;
#79004=CARTESIAN_POINT ( 'NONE',  ( 6.966220764712143243, 6.002124920821316323, -2.500000000000000444 ) ) ;
#79008=CARTESIAN_POINT ( 'NONE',  ( -4.736594563127865420, 6.619389305106191834, -1.599625672291271394 ) ) ;
#79021=CARTESIAN_POINT ( 'NONE',  ( 3.549202351727371862, 7.362762853649070571, -0.7998128361456362523 ) ) ;
#79045=CARTESIAN_POINT ( 'NONE',  ( 4.179656494762836516, 8.098292687190454586, -0.7998128361456362523 ) ) ;
#79046=CARTESIAN_POINT ( 'NONE',  ( 3.576318658954677598, 7.394398545414291313, 0.7998128361456281477 ) ) ;
#79048=CARTESIAN_POINT ( 'NONE',  ( 4.309512724297349884, 6.121127159803966933, 1.599625672291261402 ) ) ;
#79059=CARTESIAN_POINT ( 'NONE',  ( 5.184698244283005408, 7.856242361780820360, 1.254847465626233616 ) ) ;
#79060=CARTESIAN_POINT ( 'NONE',  ( -5.519577934094894722, 7.532869904567736974, 1.443375672974058777 ) ) ;
#79061=CARTESIAN_POINT ( 'NONE',  ( -2.981281212289682792, 6.492261378021210838, -0.0003813922843012157449 ) ) ;
#79075=ORIENTED_EDGE ( 'NONE', *, *, #42883, .T. ) ;
#79082=CARTESIAN_POINT ( 'NONE',  ( -5.607971574822836480, 5.595440440058774278, -0.3944387069941719393 ) ) ;
#79089=CARTESIAN_POINT ( 'NONE',  ( 4.016958651398847557, 7.908478536599129249, -0.7998128361456362523 ) ) ;
#79091=CARTESIAN_POINT ( 'NONE',  ( 4.760848217054122422, 5.583353003765119560, -1.199719254218452047 ) ) ;
#79098=CYLINDRICAL_SURFACE ( 'NONE', #75889, 1.250000000000000000 ) ;
#79108=CARTESIAN_POINT ( 'NONE',  ( -7.957709816578236506, 8.248692638954882028, 0.7998128361456341429 ) ) ;
#79121=CARTESIAN_POINT ( 'NONE',  ( 4.206772801990143584, 8.129928378955675328, 0.7998128361456271485 ) ) ;
#79127=CARTESIAN_POINT ( 'NONE',  ( 4.525389411911321602, 8.501647757197021704, -0.7998128361456381397 ) ) ;
#79151=CARTESIAN_POINT ( 'NONE',  ( -6.316846275044603942, 6.877910198612338100, 0.7063612664817873199 ) ) ;
#79160=CARTESIAN_POINT ( 'NONE',  ( -4.457598643843001973, 8.422558527783969851, 0.000000000000000000 ) ) ;
#79162=CARTESIAN_POINT ( 'NONE',  ( 5.845500506147374153, 6.848780674373954547, 1.199719254218453823 ) ) ;
#79166=CARTESIAN_POINT ( 'NONE',  ( -6.505933609711270549, 8.683618192786854095, -1.599625672291271394 ) ) ;
#79170=CARTESIAN_POINT ( 'NONE',  ( 8.011942431032855083, 8.311964022485323511, 0.7998128361456291469 ) ) ;
#79175=CARTESIAN_POINT ( 'NONE',  ( -6.161504026110072196, 7.065710439381887475, -1.087211863304170523 ) ) ;
#79190=VERTEX_POINT ( 'NONE', #135851 ) ;
#79194=CARTESIAN_POINT ( 'NONE',  ( 6.265276383290871109, 7.442482214328385304, -1.082531754730548412 ) ) ;
#79208=CARTESIAN_POINT ( 'NONE',  ( -3.851925040058333582, 7.508013290127760087, -0.7216878364870458196 ) ) ;
#79212=CARTESIAN_POINT ( 'NONE',  ( 4.712340909201580885, 7.655425606447271214, -1.199719254218452047 ) ) ;
#79232=CARTESIAN_POINT ( 'NONE',  ( 6.007671464186823407, 9.062681570643055906, 1.082531754730549967 ) ) ;
#79244=VERTEX_POINT ( 'NONE', #52459 ) ;
#79259=CARTESIAN_POINT ( 'NONE',  ( 4.923019175537949543, 4.916146257648610352, 0.000000000000000000 ) ) ;
#79264=CARTESIAN_POINT ( 'NONE',  ( 3.390420931869152721, 6.113185632892752075, -1.199719254218452047 ) ) ;
#79268=CARTESIAN_POINT ( 'NONE',  ( -4.706088717274938382, 6.583799151611112954, 1.443375672974058777 ) ) ;
#79273=CARTESIAN_POINT ( 'NONE',  ( -4.125423880308188629, 8.035021303660014880, -0.7998128361456481317 ) ) ;
#79276=AXIS2_PLACEMENT_3D ( 'NONE', #156315, #73987, #123896 ) ;
#79282=CARTESIAN_POINT ( 'NONE',  ( -3.494969737272722643, 7.299491470118629088, -0.7998128361456481317 ) ) ;
#79284=CARTESIAN_POINT ( 'NONE',  ( 6.454463653088309272, 6.866155873091829953, 0.6733577401037347254 ) ) ;
#79289=CARTESIAN_POINT ( 'NONE',  ( 4.681308178468477799, 8.683552984847038303, 0.000000000000000000 ) ) ;
#79297=CARTESIAN_POINT ( 'NONE',  ( -7.075376061485238566, 9.347967719856493218, 1.599625672291269396 ) ) ;
#79303=CARTESIAN_POINT ( 'NONE',  ( -4.502189528189771472, 7.410248995266807803, -1.199719254218453823 ) ) ;
#79307=CARTESIAN_POINT ( 'NONE',  ( 5.356880090730850696, 9.263794182579101033, 0.7216878364870317197 ) ) ;
#79309=CARTESIAN_POINT ( 'NONE',  ( -7.078765599666485997, 7.431183752465250869, 0.000000000000000000 ) ) ;
#79316=CARTESIAN_POINT ( 'NONE',  ( 5.285699784481295183, 7.260012063351913625, 1.599625672291268286 ) ) ;
#79340=CARTESIAN_POINT ( 'NONE',  ( 3.809456170543987774, 8.470288933811271903, -2.500000000000000444 ) ) ;
#79345=CARTESIAN_POINT ( 'NONE',  ( 4.978641999450219124, 7.938775605734648799, 1.052364473307040305 ) ) ;
#79354=CARTESIAN_POINT ( 'NONE',  ( 5.345657705538078730, 9.458627433094950021, 0.7998128361456331437 ) ) ;
#79359=CARTESIAN_POINT ( 'NONE',  ( -5.295344997983027824, 7.654313019038245791, -1.225062028442117423 ) ) ;
#79365=CARTESIAN_POINT ( 'NONE',  ( -4.624739795592948788, 5.528522862014106920, -1.082531754730549967 ) ) ;
#79375=CARTESIAN_POINT ( 'NONE',  ( -5.191846479390389568, 5.021852078902356631, 0.7998128361456281477 ) ) ;
#79385=CARTESIAN_POINT ( 'NONE',  ( 4.206772801990143584, 8.129928378955675328, 0.7998128361456271485 ) ) ;
#79388=CARTESIAN_POINT ( 'NONE',  ( 5.519577934094852978, 7.532869904567736974, 1.443375672974064550 ) ) ;
#79389=CARTESIAN_POINT ( 'NONE',  ( -1.298432343300637860E-14, 2.519999999999999130, -2.000000000000000000 ) ) ;
#79397=DIRECTION ( 'NONE',  ( -0.000000000000000000, -1.000000000000000000, -0.000000000000000000 ) ) ;
#79403=CARTESIAN_POINT ( 'NONE',  ( -4.122561227007127016, 6.967349310553715647, 1.199719254218452935 ) ) ;
#79404=CARTESIAN_POINT ( 'NONE',  ( 3.054329744828568227, 6.785411478933790264, 0.000000000000000000 ) ) ;
#79413=ORIENTED_EDGE ( 'NONE', *, *, #143526, .T. ) ;
#79416=CARTESIAN_POINT ( 'NONE',  ( -5.413448473606448985, 9.537716662508005427, 0.000000000000000000 ) ) ;
#79417=CARTESIAN_POINT ( 'NONE',  ( 6.017840079619279692, 8.114175741012878973, -1.599625672291281386 ) ) ;
#79424=CARTESIAN_POINT ( 'NONE',  ( 3.607351389687783794, 6.366271167014519783, 1.199719254218451159 ) ) ;
#79430=CARTESIAN_POINT ( 'NONE',  ( -5.773448424614897156, 7.353550462951784716, 1.313087523158409153 ) ) ;
#79439=CARTESIAN_POINT ( 'NONE',  ( -4.516274566683622815, 5.401980094953223066, 1.082531754730549078 ) ) ;
#79455=CARTESIAN_POINT ( 'NONE',  ( 6.042093733545556233, 7.078139439671806699, -1.199719254218452047 ) ) ;
#79480=ORIENTED_EDGE ( 'NONE', *, *, #196460, .F. ) ;
#79488=CARTESIAN_POINT ( 'NONE',  ( 4.903208829997618423, 5.749440385532527564, -1.199719254218450271 ) ) ;
#79492=CARTESIAN_POINT ( 'NONE',  ( 4.882344714252594642, 4.868692719482363707, 0.000000000000000000 ) ) ;
#79521=CARTESIAN_POINT ( 'NONE',  ( -5.173318132066234476, 8.193232366456022930, -1.199719254218453823 ) ) ;
#79523=CARTESIAN_POINT ( 'NONE',  ( 6.089020385868848528, 8.197219431637373432, -1.443375672974078761 ) ) ;
#79528=CARTESIAN_POINT ( 'NONE',  ( -6.479871072688648148, 6.524547437750345402, 0.000000000000000000 ) ) ;
#79533=CARTESIAN_POINT ( 'NONE',  ( -5.307090785106547415, 5.156303768904543894, -0.7998128361456362523 ) ) ;
#79538=CARTESIAN_POINT ( 'NONE',  ( -6.286140498591554326, 7.362860665558790707, 1.199719254218452047 ) ) ;
#79548=CARTESIAN_POINT ( 'NONE',  ( -3.786470039966538970, 7.639575156594750283, 0.000000000000000000 ) ) ;
#79552=CARTESIAN_POINT ( 'NONE',  ( -6.956742217587851052, 7.288823140040177506, 0.000000000000000000 ) ) ;
#79553=CARTESIAN_POINT ( 'NONE',  ( -5.112833325684904118, 8.979072956692109031, -0.7216878364870338292 ) ) ;
#79554=CARTESIAN_POINT ( 'NONE',  ( 5.691390622686558487, 9.861982503101517139, 0.7998128361456341429 ) ) ;
#79555=CARTESIAN_POINT ( 'NONE',  ( -7.119966945832006289, 8.335658187339330283, 1.199719254218452047 ) ) ;
#79593=CARTESIAN_POINT ( 'NONE',  ( 4.605689926069578277, 8.476745573306274650, -0.2140288463435610078 ) ) ;
#79606=CARTESIAN_POINT ( 'NONE',  ( 5.363132282657546490, 8.414682208812571673, -1.199719254218452047 ) ) ;
#79609=CARTESIAN_POINT ( 'NONE',  ( -4.492547798081878874, 6.334668079219206049, 1.599625672291263179 ) ) ;
#79613=CARTESIAN_POINT ( 'NONE',  ( -7.566859129758459979, 8.000626204239226880, 0.000000000000000000 ) ) ;
#79623=CARTESIAN_POINT ( 'NONE',  ( 5.411639590510088027, 6.342609606130419131, -1.199719254218452047 ) ) ;
#79625=CARTESIAN_POINT ( 'NONE',  ( 5.559725510055676168, 8.644040974110419384, 1.199719254218451159 ) ) ;
#79640=CARTESIAN_POINT ( 'NONE',  ( 7.374709211190586089, 7.568525266002632534, 0.000000000000000000 ) ) ;
#79641=VERTEX_POINT ( 'NONE', #148382 ) ;
#79643=EDGE_CURVE ( 'NONE', #193413, #160443, #198168, .T. ) ;
#79651=FACE_OUTER_BOUND ( 'NONE', #121183, .T. ) ;
#79654=CARTESIAN_POINT ( 'NONE',  ( -5.980555157403903976, 6.149938236492225485, 0.000000000000000000 ) ) ;
#79655=CARTESIAN_POINT ( 'NONE',  ( 4.068855497876973537, 7.761098824249525130, -0.7216878364870338292 ) ) ;
#79667=CARTESIAN_POINT ( 'NONE',  ( -5.912764389335557702, 8.951956649983198844, 1.082531754730550855 ) ) ;
#79671=CARTESIAN_POINT ( 'NONE',  ( 3.553645660113312399, 7.160020680191912845, -1.734723475976807094E-15 ) ) ;
#79688=CARTESIAN_POINT ( 'NONE',  ( 6.073126464278658432, 6.050012061272033392, 0.000000000000000000 ) ) ;
#79690=CARTESIAN_POINT ( 'NONE',  ( -4.787964524281469458, 5.614988695530339413, -1.199719254218453823 ) ) ;
#79701=CARTESIAN_POINT ( 'NONE',  ( 5.383996398402570271, 9.295429874862735531, 0.000000000000000000 ) ) ;
#79703=CARTESIAN_POINT ( 'NONE',  ( -5.956828388357799042, 8.042995434541133193, 1.599625672291263179 ) ) ;
#79704=CARTESIAN_POINT ( 'NONE',  ( 6.540882763950133238, 6.595727744222092959, 0.000000000000000000 ) ) ;
#79705=ORIENTED_EDGE ( 'NONE', *, *, #63015, .T. ) ;
#79712=CARTESIAN_POINT ( 'NONE',  ( -6.296835998904160014, 6.311006518335105397, 0.000000000000000000 ) ) ;
#79739=CARTESIAN_POINT ( 'NONE',  ( 4.990809943606266508, 6.915973915664348937, -1.443375672974068769 ) ) ;
#79745=CARTESIAN_POINT ( 'NONE',  ( 5.519577934094864524, 5.612131475965050242, 0.7216878364870328300 ) ) ;
#79757=CARTESIAN_POINT ( 'NONE',  ( -5.173318132066234476, 8.193232366456022930, -1.199719254218453823 ) ) ;
#79759=CARTESIAN_POINT ( 'NONE',  ( -7.099629715411508890, 8.311931418515415615, 1.199719254218452047 ) ) ;
#79767=CARTESIAN_POINT ( 'NONE',  ( 3.051993976407674225, 6.574760382535328240, -0.7216878364870338292 ) ) ;
#79774=CARTESIAN_POINT ( 'NONE',  ( -6.123442655227560927, 7.173046514967467147, 1.199719254218452047 ) ) ;
#79780=CARTESIAN_POINT ( 'NONE',  ( -4.828112100242291760, 6.726159765073026264, -1.443375672974066548 ) ) ;
#79783=CARTESIAN_POINT ( 'NONE',  ( -4.098307573080856692, 8.003385611894792362, 0.7998128361456352531 ) ) ;
#79799=CARTESIAN_POINT ( 'NONE',  ( -6.569768201793956486, 6.780247303854220142, 0.5133454205821968985 ) ) ;
#79804=CARTESIAN_POINT ( 'NONE',  ( -3.757017964318317471, 6.436919154129725484, 1.082531754730549967 ) ) ;
#79805=CARTESIAN_POINT ( 'NONE',  ( 5.083381250481017410, 4.895309311841474553, 0.7998128361456352531 ) ) ;
#79806=CARTESIAN_POINT ( 'NONE',  ( -3.657667580636712934, 7.489305620709952649, -0.7998128361456481317 ) ) ;
#79833=CARTESIAN_POINT ( 'NONE',  ( -5.610041701004606196, 9.767075427805856691, -0.7998128361456362523 ) ) ;
#79857=CARTESIAN_POINT ( 'NONE',  ( 5.677832469072920496, 9.846164657218904992, 0.000000000000000000 ) ) ;
#79858=CARTESIAN_POINT ( 'NONE',  ( 5.345657705538078730, 9.458627433094950021, 0.7998128361456331437 ) ) ;
#79870=CARTESIAN_POINT ( 'NONE',  ( 4.943016831304842817, 7.975319854387232787, 1.017975537214605319 ) ) ;
#79872=CARTESIAN_POINT ( 'NONE',  ( 5.045042558060919724, 8.899983727797476263, -0.7216878364870458196 ) ) ;
#79877=CARTESIAN_POINT ( 'NONE',  ( -4.797606254389363833, 6.690569611577942943, 1.599625672291263179 ) ) ;
#79884=CARTESIAN_POINT ( 'NONE',  ( -7.444835747235459600, 8.818634805597074688, 1.082531754730549078 ) ) ;
#79892=CARTESIAN_POINT ( 'NONE',  ( -3.122120512896910505, 6.864500708346841229, 0.7998128361456352531 ) ) ;
#79903=CARTESIAN_POINT ( 'NONE',  ( 6.668631453075247073, 8.873432343378178544, -1.599625672291281386 ) ) ;
#79927=CARTESIAN_POINT ( 'NONE',  ( 7.126746022638799971, 8.343567110280638133, 1.199719254218452047 ) ) ;
#79929=CARTESIAN_POINT ( 'NONE',  ( -6.401963353335964335, 6.822014978843597532, 0.5293317295896986518 ) ) ;
#79936=CARTESIAN_POINT ( 'NONE',  ( 4.355912491740495440, 8.303924683664389406, 0.000000000000000000 ) ) ;
#79937=CARTESIAN_POINT ( 'NONE',  ( -6.966220764712148572, 6.002124920821316323, 2.500000000000000444 ) ) ;
#79944=CARTESIAN_POINT ( 'NONE',  ( 5.248414862265931902, 5.295774558831261913, 0.000000000000000000 ) ) ;
#79947=DIRECTION ( 'NONE',  ( 1.000000000000000000, 0.000000000000000000, 0.000000000000000000 ) ) ;
#79948=CARTESIAN_POINT ( 'NONE',  ( 5.207740401424913124, 9.089797878388800711, -0.7216878364870458196 ) ) ;
#79959=CARTESIAN_POINT ( 'NONE',  ( -4.665414256878293031, 7.496714828783040296, -1.082531754730549967 ) ) ;
#79977=CIRCLE ( 'NONE', #201022, 0.7500000000000011102 ) ;
#79984=CARTESIAN_POINT ( 'NONE',  ( 4.651856102820254968, 7.480896982382013505, -1.082531754730548412 ) ) ;
#79994=CARTESIAN_POINT ( 'NONE',  ( 4.355912491740495440, 8.303924683664389406, 0.000000000000000000 ) ) ;
#79996=CARTESIAN_POINT ( 'NONE',  ( 5.143339171537801846, 7.093924681584509173, 1.599625672291269396 ) ) ;
#80006=CARTESIAN_POINT ( 'NONE',  ( -6.455090533882193782, 9.584670485287619002, -1.082531754730549967 ) ) ;
#80009=CARTESIAN_POINT ( 'NONE',  ( 5.682275777458851707, 6.762314840857718501, 1.082531754730549078 ) ) ;
#80025=CARTESIAN_POINT ( 'NONE',  ( -5.587368702607575344, 8.572328348800551723, 1.082531754730550855 ) ) ;
#80027=CARTESIAN_POINT ( 'NONE',  ( -4.014622883422329203, 6.737458226417744278, -1.082531754730546636 ) ) ;
#80043=CARTESIAN_POINT ( 'NONE',  ( -5.144392941742557568, 4.966489618313220333, -0.7998128361456362523 ) ) ;
#80055=CARTESIAN_POINT ( 'NONE',  ( -3.169574050544739841, 6.919863168935977527, -0.7998128361456481317 ) ) ;
#80065=CARTESIAN_POINT ( 'NONE',  ( -5.413448473606448985, 9.537716662508005427, 0.000000000000000000 ) ) ;
#80066=CARTESIAN_POINT ( 'NONE',  ( -4.845071979149651042, 8.194897641035423064, 0.9605101338234197650 ) ) ;
#80073=CARTESIAN_POINT ( 'NONE',  ( -5.061990249855848667, 6.999017606288844284, -1.599625672291271394 ) ) ;
#80076=CARTESIAN_POINT ( 'NONE',  ( -5.492988512192097161, 6.437516681426083132, 1.199719254218452935 ) ) ;
#80086=CARTESIAN_POINT ( 'NONE',  ( 5.143339171537801846, 7.093924681584509173, 1.599625672291269396 ) ) ;
#80110=CARTESIAN_POINT ( 'NONE',  ( 5.716698046817569434, 6.698511138489155137, -1.199719254218452047 ) ) ;
#80111=CARTESIAN_POINT ( 'NONE',  ( 5.435893244436359240, 5.306573304789342416, -0.7998128361456481317 ) ) ;
#80116=CARTESIAN_POINT ( 'NONE',  ( -4.434925645001631445, 8.188180662561569179, 0.7216878364870504825 ) ) ;
#80125=CARTESIAN_POINT ( 'NONE',  ( 4.624709440338444111, 8.453137518702421360, 0.3515692964491355932 ) ) ;
#80126=CARTESIAN_POINT ( 'NONE',  ( -5.383996397958228819, 8.335060660042973524, 1.082531754730550855 ) ) ;
#80134=CIRCLE ( 'NONE', #177091, 0.08000000000000025147 ) ;
#80155=CARTESIAN_POINT ( 'NONE',  ( 6.039231080244466199, 6.010467446565510130, 0.7998128361456352531 ) ) ;
#80157=CARTESIAN_POINT ( 'NONE',  ( 4.598150373690133463, 5.393538853173795111, -1.199719254218452047 ) ) ;
#80177=CARTESIAN_POINT ( 'NONE',  ( -7.445362632559989535, 8.715286488521982733, 1.199719254218452047 ) ) ;
#80188=CARTESIAN_POINT ( 'NONE',  ( 4.369470645354133431, 8.319742529546998000, 0.7998128361456271485 ) ) ;
#80192=CARTESIAN_POINT ( 'NONE',  ( 6.384963997392946844, 6.413822516572072807, 0.7998128361456352531 ) ) ;
#80204=CARTESIAN_POINT ( 'NONE',  ( 4.651083699394226834, 8.303454393088664176, 0.4639335724816190942 ) ) ;
#80228=CARTESIAN_POINT ( 'NONE',  ( -6.642568916052639771, 6.714361588341672515, 0.000000000000000000 ) ) ;
#80230=CARTESIAN_POINT ( 'NONE',  ( 4.688087255275310561, 8.691461907788344377, -0.7998128361456381397 ) ) ;
#80231=CARTESIAN_POINT ( 'NONE',  ( -6.137101742630204804, 5.375560105519675780, 2.500000000000000888 ) ) ;
#80234=CARTESIAN_POINT ( 'NONE',  ( -8.086512275908061653, 8.398962174839683215, 0.000000000000000000 ) ) ;
#80244=CARTESIAN_POINT ( 'NONE',  ( 0.1009995753616283604, 2.612933547399907130, -1.997555607063249195 ) ) ;
#80260=CARTESIAN_POINT ( 'NONE',  ( 6.536439455564164724, 7.758839131980592718, 1.082531754730549967 ) ) ;
#80268=FACE_OUTER_BOUND ( 'NONE', #177770, .T. ) ;
#80275=CARTESIAN_POINT ( 'NONE',  ( -5.831415467653581430, 5.975941931783510519, 0.7216878364870257245 ) ) ;
#80278=CARTESIAN_POINT ( 'NONE',  ( 7.062871678076271920, 7.204714810702593120, -0.7998128361456341429 ) ) ;
#80320=CARTESIAN_POINT ( 'NONE',  ( 4.760321332173959696, 4.726332107057286791, 0.000000000000000000 ) ) ;
#80321=CARTESIAN_POINT ( 'NONE',  ( -5.670636218918978066, 5.580440108352386019, 0.2509703219331788637 ) ) ;
#80325=CARTESIAN_POINT ( 'NONE',  ( 3.984117037569365305, 5.741498858621315371, 1.599625672291261402 ) ) ;
#80327=CARTESIAN_POINT ( 'NONE',  ( -4.187547269546461948, 7.837270521969020187, 0.3263639828635342410 ) ) ;
#80329=EDGE_LOOP ( 'NONE', ( #151411, #45799, #61960, #152198, #110102, #187351 ) ) ;
#80330=CARTESIAN_POINT ( 'NONE',  ( -4.868786560638931782, 6.773613302202437403, 1.443375672974058777 ) ) ;
#80336=CARTESIAN_POINT ( 'NONE',  ( -6.283277845290492714, 6.295188672452495915, -0.7998128361456362523 ) ) ;
#80345=CARTESIAN_POINT ( 'NONE',  ( -5.666381855868691808, 5.575476684793721383, 0.000000000000000000 ) ) ;
#80348=CARTESIAN_POINT ( 'NONE',  ( 6.378761646814803399, 6.917158162233129737, 0.8102004381213165907 ) ) ;
#80354=CARTESIAN_POINT ( 'NONE',  ( 4.518610335104485287, 8.493738834255713854, 0.000000000000000000 ) ) ;
#80358=ADVANCED_FACE ( 'NONE', ( #83228 ), #25300, .T. ) ;
#80364=CARTESIAN_POINT ( 'NONE',  ( -4.573896719763875574, 6.429575154514868274, -1.599625672291271394 ) ) ;
#80369=CARTESIAN_POINT ( 'NONE',  ( -5.101610940492132151, 9.173906207207963348, -0.7998128361456362523 ) ) ;
#80373=CARTESIAN_POINT ( 'NONE',  ( 6.983858524370782916, 7.320458831286981827, 0.7216878364870328300 ) ) ;
#80375=CARTESIAN_POINT ( 'NONE',  ( -6.007671464186866928, 8.102312356341712984, 1.443375672974058777 ) ) ;
#80381=CARTESIAN_POINT ( 'NONE',  ( 3.854260808034858155, 7.718664386007802136, -0.7998128361456362523 ) ) ;
#80388=CARTESIAN_POINT ( 'NONE',  ( 5.558836782162522638, 7.518240855878357110, -1.384758111419039039 ) ) ;
#80424=CARTESIAN_POINT ( 'NONE',  ( -6.290641498436300161, 6.895329709839009169, -0.7498213622291228786 ) ) ;
#80427=VERTEX_POINT ( 'NONE', #71236 ) ;
#80432=CARTESIAN_POINT ( 'NONE',  ( -5.139949632912262700, 5.169231791251960750, 0.7216878364870257245 ) ) ;
#80443=CARTESIAN_POINT ( 'NONE',  ( -5.002032328799064231, 4.800402236545811441, -0.7998128361456362523 ) ) ;
#80445=CARTESIAN_POINT ( 'NONE',  ( 8.174640274396848483, 8.501778173076651512, 0.7998128361456291469 ) ) ;
#80453=ORIENTED_EDGE ( 'NONE', *, *, #106488, .F. ) ;
#80455=CARTESIAN_POINT ( 'NONE',  ( 5.825163275726873202, 6.825053905550038991, 1.199719254218452047 ) ) ;
#80458=CARTESIAN_POINT ( 'NONE',  ( 5.180624093753221970, 9.058162186105164437, 0.000000000000000000 ) ) ;
#80472=CARTESIAN_POINT ( 'NONE',  ( -5.098748287191073203, 8.106234214101666780, 1.199719254218452935 ) ) ;
#80473=CARTESIAN_POINT ( 'NONE',  ( 4.258142763143749399, 7.125527769379820242, 1.199719254218451159 ) ) ;
#80483=VERTEX_POINT ( 'NONE', #184992 ) ;
#80484=CARTESIAN_POINT ( 'NONE',  ( -5.427006627220116286, 9.553534508390610469, -0.7998128361456362523 ) ) ;
#80485=CARTESIAN_POINT ( 'NONE',  ( 5.668190738965027897, 8.770583741171307679, -1.199719254218452047 ) ) ;
#80487=DIRECTION ( 'NONE',  ( -0.000000000000000000, 1.000000000000000000, -0.000000000000000000 ) ) ;
#80492=CARTESIAN_POINT ( 'NONE',  ( 5.876533236880477240, 5.820653295974182129, 0.7998128361456352531 ) ) ;
#80495=CARTESIAN_POINT ( 'NONE',  ( -0.4820161904281213272, 2.981954314639482018, 1.941394296928433238 ) ) ;
#80499=CARTESIAN_POINT ( 'NONE',  ( -6.019435214058361794, 7.168094078216475040, 1.196694171119830008 ) ) ;
#80507=CARTESIAN_POINT ( 'NONE',  ( -6.312203035614172286, 9.521931420595302953, -1.199719254218452047 ) ) ;
#80557=CARTESIAN_POINT ( 'NONE',  ( 6.034787771858531435, 10.05468647722803865, 0.000000000000000000 ) ) ;
#80558=CARTESIAN_POINT ( 'NONE',  ( -3.472296738875691346, 6.104744391113324120, 1.082531754730549967 ) ) ;
#80561=CARTESIAN_POINT ( 'NONE',  ( 4.883600829025052548, 4.870158186716897042, -0.06686181454683927383 ) ) ;
#80590=CARTESIAN_POINT ( 'NONE',  ( -4.308458954092677651, 8.248562223075252220, -0.7998128361456362523 ) ) ;
#80592=CARTESIAN_POINT ( 'NONE',  ( 5.180624093753221970, 9.058162186105164437, 0.000000000000000000 ) ) ;
#80597=CARTESIAN_POINT ( 'NONE',  ( -4.769436176957319695, 8.786368983084006601, 0.7998128361456281477 ) ) ;
#80603=CARTESIAN_POINT ( 'NONE',  ( -4.176793841461789114, 7.030620694084159794, -1.199719254218455378 ) ) ;
#80610=CARTESIAN_POINT ( 'NONE',  ( -6.798487682609798632, 6.896266815991691779, 0.7998128361456341429 ) ) ;
#80624=CARTESIAN_POINT ( 'NONE',  ( -5.418418667316934112, 6.350518529071726981, -1.199719254218453823 ) ) ;
#80627=CARTESIAN_POINT ( 'NONE',  ( -6.292392690518223475, 6.513748691792265788, -0.7216878364870338292 ) ) ;
#80628=CARTESIAN_POINT ( 'NONE',  ( -7.241463443030476732, 7.620997903056574430, 0.000000000000000000 ) ) ;
#80629=CARTESIAN_POINT ( 'NONE',  ( 6.526270840131753737, 8.707344961610770540, -1.599625672291283607 ) ) ;
#80630=CARTESIAN_POINT ( 'NONE',  ( -6.770317605177755382, 8.992066187497757213, 1.599625672291269396 ) ) ;
#80652=VECTOR ( 'NONE', #86348, 1000.000000000000000 ) ;
#80669=CARTESIAN_POINT ( 'NONE',  ( 5.364009635805341958, 7.578432035813580825, -1.241402483855597039 ) ) ;
#80681=CARTESIAN_POINT ( 'NONE',  ( -4.596923820214036560, 8.483565078729160547, 0.2266403168418751335 ) ) ;
#80685=CARTESIAN_POINT ( 'NONE',  ( 7.700104897918568447, 7.948153567185284096, 0.000000000000000000 ) ) ;
#80688=CARTESIAN_POINT ( 'NONE',  ( -6.168033539574333979, 6.160736982450306876, 0.7998128361456281477 ) ) ;
#80692=CARTESIAN_POINT ( 'NONE',  ( -6.224601922005509991, 10.27613631906616476, 0.7216878364870267237 ) ) ;
#80703=CARTESIAN_POINT ( 'NONE',  ( 5.923986774528332333, 5.876015756563318426, -0.7998128361456481317 ) ) ;
#80705=CARTESIAN_POINT ( 'NONE',  ( 6.481679955784983349, 9.719654494127929922, -1.199719254218452047 ) ) ;
#80712=ORIENTED_EDGE ( 'NONE', *, *, #48284, .T. ) ;
#80713=CARTESIAN_POINT ( 'NONE',  ( 4.706615602599436343, 5.520081620234675412, 1.199719254218452935 ) ) ;
#80717=CARTESIAN_POINT ( 'NONE',  ( 4.525389411911321602, 8.501647757197021704, -0.7998128361456381397 ) ) ;
#80730=CARTESIAN_POINT ( 'NONE',  ( -4.177320726786315497, 7.887641591310407208, -0.7216878364870458196 ) ) ;
#80731=CARTESIAN_POINT ( 'NONE',  ( 6.224601922449876312, 6.434659462379210382, 0.000000000000000000 ) ) ;
#80739=EDGE_CURVE ( 'NONE', #96695, #44793, #103507, .T. ) ;
#80743=CARTESIAN_POINT ( 'NONE',  ( -3.471769853551161411, 6.208092708188416076, 1.199719254218452935 ) ) ;
#80744=CARTESIAN_POINT ( 'NONE',  ( -7.268579750702168774, 7.652633595340216921, -0.7216878364870338292 ) ) ;
#80745=CARTESIAN_POINT ( 'NONE',  ( 6.393551957296131683, 9.616838495890963401, 1.199719254218452047 ) ) ;
#80748=CARTESIAN_POINT ( 'NONE',  ( 6.360183458142179447, 6.592837920686898556, -0.7216878364870458196 ) ) ;
#80762=CARTESIAN_POINT ( 'NONE',  ( -5.842658511366215279, 6.642451456931087073, 0.9392888627727929984 ) ) ;
#80765=CARTESIAN_POINT ( 'NONE',  ( 6.412080304620304538, 6.445458208337293549, -0.7998128361456481317 ) ) ;
#80767=CARTESIAN_POINT ( 'NONE',  ( -5.178288325776719603, 5.006034233019745372, 0.000000000000000000 ) ) ;
#80781=CARTESIAN_POINT ( 'NONE',  ( 5.397554552016204710, 9.311247720745345902, 0.7216878364870317197 ) ) ;
#80783=CARTESIAN_POINT ( 'NONE',  ( -6.740338644649361832, 7.892758502626242567, -1.199719254218452047 ) ) ;
#80784=CARTESIAN_POINT ( 'NONE',  ( 6.364626766972446781, 6.390095747748157251, 0.7998128361456352531 ) ) ;
#80785=ORIENTED_EDGE ( 'NONE', *, *, #125818, .F. ) ;
#80792=CARTESIAN_POINT ( 'NONE',  ( -4.938913097128142304, 8.984092056616635347, -0.7998128361456362523 ) ) ;
#80819=CARTESIAN_POINT ( 'NONE',  ( 5.072158865288233009, 7.010880990960010273, 1.443375672974065660 ) ) ;
#80820=VERTEX_POINT ( 'NONE', #171972 ) ;
#80825=CARTESIAN_POINT ( 'NONE',  ( 4.028181036591620412, 7.713645286083276709, -0.7216878364870338292 ) ) ;
#80834=AXIS2_PLACEMENT_3D ( 'NONE', #163888, #80487, #31751 ) ;
#80838=CARTESIAN_POINT ( 'NONE',  ( -6.954406449166956605, 7.078172043641714595, -0.7998128361456362523 ) ) ;
#80840=CARTESIAN_POINT ( 'NONE',  ( -5.264308783856126439, 9.363720357799287797, -0.7998128361456362523 ) ) ;
#80847=CARTESIAN_POINT ( 'NONE',  ( 8.188198428010544205, 8.517596018959260107, 0.000000000000000000 ) ) ;
#80852=CARTESIAN_POINT ( 'NONE',  ( -6.611536185319534908, 7.742488966741438716, 1.199719254218452047 ) ) ;
#80859=CARTESIAN_POINT ( 'NONE',  ( -5.045042558060949034, 6.018876084893449274, 1.082531754730549078 ) ) ;
#80862=CARTESIAN_POINT ( 'NONE',  ( -4.599959256786493533, 8.588645909551377855, 0.000000000000000000 ) ) ;
#80882=CARTESIAN_POINT ( 'NONE',  ( -3.973948422136981407, 5.729635473950147606, -1.443375672974066548 ) ) ;
#80883=CARTESIAN_POINT ( 'NONE',  ( 4.411198876399872404, 6.239761003923544713, -1.599625672291273171 ) ) ;
#80884=CARTESIAN_POINT ( 'NONE',  ( -6.303615075710993665, 6.318915441276411471, -0.7998128361456362523 ) ) ;
#80909=CARTESIAN_POINT ( 'NONE',  ( -5.759181390754928742, 9.941071732514568993, 0.000000000000000000 ) ) ;
#80932=CARTESIAN_POINT ( 'NONE',  ( 6.156284269057003655, 9.340026192945279249, -1.199719254218452047 ) ) ;
#80933=DIRECTION ( 'NONE',  ( 0.000000000000000000, 0.000000000000000000, -1.000000000000000000 ) ) ;
#80944=CARTESIAN_POINT ( 'NONE',  ( 5.614387949662905442, 7.370906683214474953, 1.237392280610301931 ) ) ;
#80946=CARTESIAN_POINT ( 'NONE',  ( 3.067887898442204442, 6.801229324816399746, 0.7998128361456271485 ) ) ;
#80951=VERTEX_POINT ( 'NONE', #208714 ) ;
#80952=CARTESIAN_POINT ( 'NONE',  ( -5.936491157937300756, 8.019268665717216749, 1.599625672291263179 ) ) ;
#80957=CARTESIAN_POINT ( 'NONE',  ( -6.089020385868850305, 10.11795786024005572, -0.7216878364870338292 ) ) ;
#80960=CARTESIAN_POINT ( 'NONE',  ( -5.000214209863262482, 4.798281097787373994, 0.2926532548524369837 ) ) ;
#80967=CARTESIAN_POINT ( 'NONE',  ( -5.971440312176176768, 5.931378217152456500, 0.000000000000000000 ) ) ;
#80980=CARTESIAN_POINT ( 'NONE',  ( 3.736153849017632922, 6.516540702899320081, -1.199719254218453823 ) ) ;
#81000=CARTESIAN_POINT ( 'NONE',  ( -6.749980374757255319, 8.968339418673846097, 1.599625672291269396 ) ) ;
#81011=CARTESIAN_POINT ( 'NONE',  ( 6.527324610336440180, 6.579909898339485252, 0.7998128361456331437 ) ) ;
#81017=CARTESIAN_POINT ( 'NONE',  ( 4.258669648468281110, 6.061810238003387141, 1.443375672974058777 ) ) ;
#81020=CARTESIAN_POINT ( 'NONE',  ( -4.823892679392753458, 8.212814747032918916, -0.9657451781678332292 ) ) ;
#81021=CARTESIAN_POINT ( 'NONE',  ( 5.885648082108190238, 7.959951743916638733, 1.443375672974065660 ) ) ;
#81033=CARTESIAN_POINT ( 'NONE',  ( -5.316205630334251531, 9.216340645449683677, -0.7216878364870338292 ) ) ;
#81068=CARTESIAN_POINT ( 'NONE',  ( 4.342354338126830804, 8.288106837781779035, -0.7998128361456381397 ) ) ;
#81070=CARTESIAN_POINT ( 'NONE',  ( 4.715203562502613188, 8.723097599553565118, 0.7998128361456341429 ) ) ;
#81081=CARTESIAN_POINT ( 'NONE',  ( -4.496464221587651799, 5.274905009054215554, 1.199719254218452935 ) ) ;
#81084=CARTESIAN_POINT ( 'NONE',  ( 4.190878879955609371, 7.903459436674603822, -0.7216878364870338292 ) ) ;
#81096=CARTESIAN_POINT ( 'NONE',  ( -6.129694847154220305, 8.244672969803623630, -1.443375672974066548 ) ) ;
#81098=CARTESIAN_POINT ( 'NONE',  ( -5.533136088152923904, 6.588318536667425285, 1.082531754730549078 ) ) ;
#81116=CARTESIAN_POINT ( 'NONE',  ( -3.363304624641834106, 6.081549941127532222, -1.199719254218452047 ) ) ;
#81128=CARTESIAN_POINT ( 'NONE',  ( -3.494969737272722643, 7.299491470118629088, -0.7998128361456481317 ) ) ;
#81129=CARTESIAN_POINT ( 'NONE',  ( -5.608757509019104859, 5.636543682890225782, -0.3643211599073498674 ) ) ;
#81131=CARTESIAN_POINT ( 'NONE',  ( 7.065207446497155708, 9.336104335703744539, 0.000000000000000000 ) ) ;
#81135=CARTESIAN_POINT ( 'NONE',  ( 3.865483193227626124, 7.523831135491951372, -0.7216878364870337181 ) ) ;
#81139=CARTESIAN_POINT ( 'NONE',  ( -6.400331034103001748, 9.624747418832267698, 1.199719254218452935 ) ) ;
#81140=CARTESIAN_POINT ( 'NONE',  ( -5.638125304375204649, 7.460809226315815224, 1.342380602066863160 ) ) ;
#81145=DIRECTION ( 'NONE',  ( 0.3281536732072464768, -0.000000000000000000, -0.9446243521954066358 ) ) ;
#81157=AXIS2_PLACEMENT_3D ( 'NONE', #112503, #178514, #49565 ) ;
#81160=CARTESIAN_POINT ( 'NONE',  ( 6.574778147984297938, 6.635272358928617997, -0.7998128361456481317 ) ) ;
#81172=EDGE_CURVE ( 'NONE', #169017, #80483, #134615, .T. ) ;
#81185=CARTESIAN_POINT ( 'NONE',  ( 6.530187263637528439, 7.647581891445782709, -1.199719254218452047 ) ) ;
#81186=CARTESIAN_POINT ( 'NONE',  ( 3.901714345682657292, 7.774026846596938434, 0.7998128361456271485 ) ) ;
#81188=CARTESIAN_POINT ( 'NONE',  ( 5.564695703766185275, 5.456842840674144490, 0.000000000000000000 ) ) ;
#81200=CARTESIAN_POINT ( 'NONE',  ( 4.757636082118741783, 8.295611710538327799, 0.7840751985381082534 ) ) ;
#81201=CARTESIAN_POINT ( 'NONE',  ( -5.275531169048909952, 7.248148678680751189, -1.443375672974066548 ) ) ;
#81202=CARTESIAN_POINT ( 'NONE',  ( 3.716343503921665459, 6.389465617000312569, -1.082531754730549967 ) ) ;
#81226=CARTESIAN_POINT ( 'NONE',  ( 6.215487077222150880, 6.216099443039444949, 0.000000000000000000 ) ) ;
#81228=CARTESIAN_POINT ( 'NONE',  ( 4.004454267989866700, 5.765225627445230927, 1.599625672291262513 ) ) ;
#81244=B_SPLINE_CURVE_WITH_KNOTS ( 'NONE', 3,
 ( #181519, #166341, #211885, #82953 ),
 .UNSPECIFIED., .F., .F.,
 ( 4, 4 ),
 ( 0.000000000000000000, 0.0001938699898735654636 ),
 .UNSPECIFIED. ) ;
#81246=ADVANCED_FACE ( 'NONE', ( #166121 ), #107480, .T. ) ;
#81259=CARTESIAN_POINT ( 'NONE',  ( 5.773793314573267388, 7.829454515125894964, 1.599625672291268286 ) ) ;
#81263=CARTESIAN_POINT ( 'NONE',  ( 5.794130544993763898, 7.853181283949808744, 1.599625672291269396 ) ) ;
#81275=CARTESIAN_POINT ( 'NONE',  ( -1.843739406749240750, 8.920000000000001705, 0.7750000000000013545 ) ) ;
#81276=CARTESIAN_POINT ( 'NONE',  ( 4.735857411151594754, 8.202189375375613878, -0.7076125000919450958 ) ) ;
#81285=CARTESIAN_POINT ( 'NONE',  ( 4.924072945520472366, 4.709449622720799589, 0.000000000000000000 ) ) ;
#81300=CARTESIAN_POINT ( 'NONE',  ( -6.038177310039794854, 8.137902509836795417, -1.599625672291271394 ) ) ;
#81302=CARTESIAN_POINT ( 'NONE',  ( 4.864343252252968597, 8.897093904262280972, 0.000000000000000000 ) ) ;
#81306=CARTESIAN_POINT ( 'NONE',  ( -5.901542003698421190, 10.10715911428198055, 0.000000000000000000 ) ) ;
#81313=CARTESIAN_POINT ( 'NONE',  ( -6.434009798946909164, 6.877700593631734804, -0.7366733183416813713 ) ) ;
#81327=CARTESIAN_POINT ( 'NONE',  ( 6.427974226654860956, 7.632296364919712417, -1.082531754730548412 ) ) ;
#81330=CARTESIAN_POINT ( 'NONE',  ( -6.064239847062411926, 10.29697326487330500, 0.000000000000000000 ) ) ;
#81343=CARTESIAN_POINT ( 'NONE',  ( -5.966997003790240228, 6.134120390609613338, -0.7216878364870338292 ) ) ;
#81345=CARTESIAN_POINT ( 'NONE',  ( 6.547661840756936691, 6.603636667163397256, 0.7998128361456352531 ) ) ;
#81368=CARTESIAN_POINT ( 'NONE',  ( 5.755082894556171169, 5.678961229929130106, -0.4337107928850430505 ) ) ;
#81392=CARTESIAN_POINT ( 'NONE',  ( 3.379725431556547477, 7.165039780116438273, -1.734723475976807094E-15 ) ) ;
#81394=DIRECTION ( 'NONE',  ( 1.000000000000000000, 0.000000000000000000, 0.000000000000000000 ) ) ;
#81397=CARTESIAN_POINT ( 'NONE',  ( -5.438229012412911345, 5.517224400669388018, -0.7216878364870338292 ) ) ;
#81404=CARTESIAN_POINT ( 'NONE',  ( -5.041653019435350380, 6.975290837464928728, -1.599625672291271394 ) ) ;
#81412=DIRECTION ( 'NONE',  ( 0.7592566023653005702, -0.6507913734559639396, 0.000000000000000000 ) ) ;
#81413=CARTESIAN_POINT ( 'NONE',  ( -6.089547271193396227, 7.133501900260939443, -1.199719254218453823 ) ) ;
#81416=CARTESIAN_POINT ( 'NONE',  ( 6.044612043767858545, 7.151903759757407109, 1.166429756139725660 ) ) ;
#81421=CARTESIAN_POINT ( 'NONE',  ( 4.993145711582793744, 9.047363440147082159, -0.7998128361456481317 ) ) ;
#81429=CARTESIAN_POINT ( 'NONE',  ( -3.793249116773374396, 7.647484079536056356, 0.7998128361456352531 ) ) ;
#81436=CARTESIAN_POINT ( 'NONE',  ( -7.273023059088104425, 7.449891421883056530, 0.000000000000000000 ) ) ;
#81441=CARTESIAN_POINT ( 'NONE',  ( 6.007671464186823407, 9.062681570643055906, 1.082531754730549967 ) ) ;
#81443=CARTESIAN_POINT ( 'NONE',  ( -6.075462232255183892, 10.10214001435745246, 0.000000000000000000 ) ) ;
#81450=CARTESIAN_POINT ( 'NONE',  ( 4.518610335104485287, 8.493738834255713854, 0.000000000000000000 ) ) ;
#81474=CARTESIAN_POINT ( 'NONE',  ( 3.177206141917496840, 8.963489737286222336, -2.500000000000001332 ) ) ;
#81486=CARTESIAN_POINT ( 'NONE',  ( 7.343676480457483002, 8.596652644402405841, -1.199719254218452047 ) ) ;
#81491=CARTESIAN_POINT ( 'NONE',  ( -6.087706144486034532, 7.033779493390481363, -0.9955609822858858537 ) ) ;
#81494=EDGE_LOOP ( 'NONE', ( #164201, #34516, #98211, #113989 ) ) ;
#81509=CARTESIAN_POINT ( 'NONE',  ( -5.354544322754380303, 5.211666229493680191, 0.7998128361456281477 ) ) ;
#81511=CARTESIAN_POINT ( 'NONE',  ( 6.016786309414542622, 10.24161080428416426, 0.7998128361456341429 ) ) ;
#81521=CARTESIAN_POINT ( 'NONE',  ( 5.448397627845284141, 7.449826213943242514, 1.599625672291268286 ) ) ;
#81524=CARTESIAN_POINT ( 'NONE',  ( 5.017926250389229459, 8.868348035513836436, 0.000000000000000000 ) ) ;
#81531=CARTESIAN_POINT ( 'NONE',  ( 0.000000000000000000, 8.980740528189222971, 0.000000000000000000 ) ) ;
#81536=CARTESIAN_POINT ( 'NONE',  ( -5.123001941117347080, 7.070197912760590064, 1.599625672291263179 ) ) ;
#81537=CARTESIAN_POINT ( 'NONE',  ( 3.230585741806197841, 6.991043475407723307, 0.7998128361456271485 ) ) ;
#81546=CARTESIAN_POINT ( 'NONE',  ( -6.064239847062411926, 10.29697326487330500, 0.000000000000000000 ) ) ;
#81547=CARTESIAN_POINT ( 'NONE',  ( 4.830447868218803897, 8.857549289555754157, -0.7998128361456481317 ) ) ;
#81553=CARTESIAN_POINT ( 'NONE',  ( 3.770049233051776749, 6.556085317605844232, 1.199719254218451159 ) ) ;
#81559=CARTESIAN_POINT ( 'NONE',  ( -6.592485395868785680, 6.772832640907240354, 0.2792626473412176957 ) ) ;
#81568=CARTESIAN_POINT ( 'NONE',  ( -5.745623237141265882, 9.925253886631958622, 0.7998128361456291469 ) ) ;
#81569=EDGE_CURVE ( 'NONE', #49308, #145598, #18315, .T. ) ;
#81570=CARTESIAN_POINT ( 'NONE',  ( -4.380693030546956912, 6.204170850428461392, 1.443375672974065660 ) ) ;
#81577=CARTESIAN_POINT ( 'NONE',  ( 5.484430959185962351, 6.043327615839653610, 0.8208683321978844649 ) ) ;
#81618=CARTESIAN_POINT ( 'NONE',  ( 4.065465959251388206, 5.836405933916976707, -1.599625672291269396 ) ) ;
#81619=CARTESIAN_POINT ( 'NONE',  ( -5.004368097219957789, 5.011053332944274352, 0.000000000000000000 ) ) ;
#81620=CARTESIAN_POINT ( 'NONE',  ( -5.608633734226008194, 5.643391804966442216, 0.4859901473732997079 ) ) ;
#81647=CARTESIAN_POINT ( 'NONE',  ( -4.281342646865346602, 8.216926531310035031, 0.7998128361456352531 ) ) ;
#81649=CARTESIAN_POINT ( 'NONE',  ( 5.519577934094840543, 9.453608333170423705, 0.7216878364870317197 ) ) ;
#81654=CARTESIAN_POINT ( 'NONE',  ( -4.959250327548641479, 9.007818825440551791, -0.7998128361456362523 ) ) ;
#81663=CARTESIAN_POINT ( 'NONE',  ( -6.473091995881817162, 6.516638514809040217, 0.7998128361456281477 ) ) ;
#81675=CARTESIAN_POINT ( 'NONE',  ( -6.231907884136888676, 7.299589282028351001, -1.199719254218453823 ) ) ;
#81678=CARTESIAN_POINT ( 'NONE',  ( -7.322812365156824654, 8.676274193172000437, 1.082531754730549078 ) ) ;
#81681=CARTESIAN_POINT ( 'NONE',  ( -5.750066545527201534, 9.722511713174800008, 0.000000000000000000 ) ) ;
#81682=CARTESIAN_POINT ( 'NONE',  ( 7.686546744304875389, 7.932335721302671949, 0.7998128361456291469 ) ) ;
#81683=CARTESIAN_POINT ( 'NONE',  ( -3.160459205317013076, 6.701303149596211206, -0.7216878364870458196 ) ) ;
#81693=VERTEX_POINT ( 'NONE', #19886 ) ;
#81702=CARTESIAN_POINT ( 'NONE',  ( -0.3979845002021665801, 2.888372890405577209, 2.025450573642260554 ) ) ;
#81707=CARTESIAN_POINT ( 'NONE',  ( -1.837596251593757390, 2.507245085144842012, -2.496647680644803025 ) ) ;
#81708=CARTESIAN_POINT ( 'NONE',  ( 6.606300428615679898, 6.765996464729716386, -0.04887194053871009303 ) ) ;
#81726=CARTESIAN_POINT ( 'NONE',  ( 6.492781079782697695, 6.747302000852300807, 0.03582484399037785816 ) ) ;
#81741=CARTESIAN_POINT ( 'NONE',  ( 5.677832469072920496, 9.846164657218904992, 0.000000000000000000 ) ) ;
#81744=CARTESIAN_POINT ( 'NONE',  ( -3.969505113751027547, 7.853116076009993840, 1.214306433183764966E-14 ) ) ;
#81748=EDGE_CURVE ( 'NONE', #61771, #197229, #15629, .T. ) ;
#81758=CARTESIAN_POINT ( 'NONE',  ( 4.278479993564246797, 7.149254538203735798, 1.199719254218452047 ) ) ;
#81760=CARTESIAN_POINT ( 'NONE',  ( 7.343676480457483002, 8.596652644402405841, -1.199719254218452047 ) ) ;
#81767=CARTESIAN_POINT ( 'NONE',  ( -6.034787771414192648, 9.094317262408276648, 1.082531754730549967 ) ) ;
#81774=CARTESIAN_POINT ( 'NONE',  ( 5.664274315459256748, 9.830346811336296398, -0.7998128361456481317 ) ) ;
#81785=AXIS2_PLACEMENT_3D ( 'NONE', #127533, #94960, #93901 ) ;
#81787=CARTESIAN_POINT ( 'NONE',  ( -5.966997003790228682, 8.054858819212300958, -1.443375672974066548 ) ) ;
#81788=CARTESIAN_POINT ( 'NONE',  ( 5.899206235721897507, 6.055031161196562373, 0.000000000000000000 ) ) ;
#81797=VERTEX_POINT ( 'NONE', #1485 ) ;
#81798=CARTESIAN_POINT ( 'NONE',  ( -4.995253251992230581, 4.792493313604505367, 0.000000000000000000 ) ) ;
#81799=CARTESIAN_POINT ( 'NONE',  ( -5.628043163448566588, 9.580151100749725757, 0.000000000000000000 ) ) ;
#81804=CARTESIAN_POINT ( 'NONE',  ( 4.516274566683592617, 8.283087737857252719, -0.7216878364870357165 ) ) ;
#81806=ORIENTED_EDGE ( 'NONE', *, *, #85855, .T. ) ;
#81808=EDGE_CURVE ( 'NONE', #113990, #82462, #173350, .T. ) ;
#81817=DIRECTION ( 'NONE',  ( 1.000000000000000000, 0.000000000000000000, 0.000000000000000000 ) ) ;
#81822=CARTESIAN_POINT ( 'NONE',  ( -4.655245641445871385, 6.524482229810530498, 1.599625672291263179 ) ) ;
#81829=CARTESIAN_POINT ( 'NONE',  ( 4.647606103345025552, 8.407977806742819027, 0.6343139517084724899 ) ) ;
#81833=CARTESIAN_POINT ( 'NONE',  ( 4.634908411025333130, 6.500755460986618495, 1.599625672291268286 ) ) ;
#81835=CARTESIAN_POINT ( 'NONE',  ( -7.456058132872594335, 7.663432341298296535, 0.000000000000000000 ) ) ;
#81836=CARTESIAN_POINT ( 'NONE',  ( 5.773793314573267388, 7.829454515125894964, 1.599625672291268286 ) ) ;
#81845=CARTESIAN_POINT ( 'NONE',  ( -6.310394152517827315, 6.326824364217716656, 0.7998128361456281477 ) ) ;
#81872=CARTESIAN_POINT ( 'NONE',  ( 3.445180431648313224, 7.033477913649446300, 0.7216878364870257245 ) ) ;
#81878=CARTESIAN_POINT ( 'NONE',  ( 5.736508391913541338, 6.825586224388162648, -1.082531754730548412 ) ) ;
#81891=CARTESIAN_POINT ( 'NONE',  ( -6.631873415740034083, 7.766215735565355160, 1.199719254218452047 ) ) ;
#81893=CARTESIAN_POINT ( 'NONE',  ( -7.923814432544069142, 8.209148024248356990, 0.000000000000000000 ) ) ;
#81899=CARTESIAN_POINT ( 'NONE',  ( 6.339319342841494453, 9.553567112360518365, -1.199719254218452047 ) ) ;
#81905=CARTESIAN_POINT ( 'NONE',  ( -5.576146316970437944, 9.727530813099326323, 0.000000000000000000 ) ) ;
#81911=CARTESIAN_POINT ( 'NONE',  ( -6.455090533882213322, 6.703562842383589349, -0.7216878364870338292 ) ) ;
#81912=AXIS2_PLACEMENT_3D ( 'NONE', #127703, #60467, #175310 ) ;
#81915=CARTESIAN_POINT ( 'NONE',  ( -5.074494633264801990, 9.142270515442742607, 0.7998128361456291469 ) ) ;
#81931=CARTESIAN_POINT ( 'NONE',  ( -6.529133882450190107, 6.806989898173073428, 0.6212416517149940143 ) ) ;
#81934=CARTESIAN_POINT ( 'NONE',  ( -4.258669648468323743, 6.061810238003387141, 1.443375672974065660 ) ) ;
#81938=CARTESIAN_POINT ( 'NONE',  ( -6.257970421159510188, 9.458660037064859694, 1.199719254218452047 ) ) ;
#81939=CARTESIAN_POINT ( 'NONE',  ( 5.598591087800349086, 5.496387455380669529, -0.7998128361456481317 ) ) ;
#81940=CARTESIAN_POINT ( 'NONE',  ( -5.444481204339554736, 8.509589284108232121, 1.199719254218454489 ) ) ;
#81963=CARTESIAN_POINT ( 'NONE',  ( -5.447343857640614573, 9.577261277214532242, -0.7998128361456362523 ) ) ;
#81988=CARTESIAN_POINT ( 'NONE',  ( 5.422335090822693715, 5.290755458906732933, 0.000000000000000000 ) ) ;
#81994=CIRCLE ( 'NONE', #168578, 0.08000000000000025147 ) ;
#82002=CARTESIAN_POINT ( 'NONE',  ( 4.716601407767927689, 8.224641112169805979, 0.6639617910879731522 ) ) ;
#82004=CARTESIAN_POINT ( 'NONE',  ( 8.000720045840086669, 8.506797273001177828, 0.7216878364870267237 ) ) ;
#82009=CARTESIAN_POINT ( 'NONE',  ( -6.123442655227560927, 7.173046514967467147, 1.199719254218452047 ) ) ;
#82015=CARTESIAN_POINT ( 'NONE',  ( -7.227905289416804102, 8.565549271475310533, -1.082531754730549967 ) ) ;
#82024=CARTESIAN_POINT ( 'NONE',  ( -5.795184315198522285, 5.725746220678519904, -0.7998128361456362523 ) ) ;
#82034=CARTESIAN_POINT ( 'NONE',  ( 5.571474780572990504, 5.464751763615448787, 0.7998128361456352531 ) ) ;
#82051=CARTESIAN_POINT ( 'NONE',  ( 5.764883781430363285, 7.068005876895862016, -2.440105357730324886 ) ) ;
#82057=CARTESIAN_POINT ( 'NONE',  ( -6.064239847062411926, 10.29697326487330500, 0.000000000000000000 ) ) ;
#82066=CARTESIAN_POINT ( 'NONE',  ( 7.354371980770088690, 7.544798497178720531, 0.000000000000000000 ) ) ;
#82073=CARTESIAN_POINT ( 'NONE',  ( 5.153507786970260796, 7.105788066255672497, -1.443375672974078761 ) ) ;
#82076=CARTESIAN_POINT ( 'NONE',  ( 6.590672070018850803, 7.822110515511036866, -1.082531754730548412 ) ) ;
#82087=CARTESIAN_POINT ( 'NONE',  ( -7.444835747679825033, 7.858265591814152629, 0.000000000000000000 ) ) ;
#82112=CARTESIAN_POINT ( 'NONE',  ( -3.811250579217344558, 5.539821323877241355, 0.000000000000000000 ) ) ;
#82122=CARTESIAN_POINT ( 'NONE',  ( 4.960304097753311936, 6.880383762169266504, 1.599625672291268286 ) ) ;
#82124=CARTESIAN_POINT ( 'NONE',  ( 6.008198349511364000, 7.038594824965278995, 1.199719254218453823 ) ) ;
#82137=CARTESIAN_POINT ( 'NONE',  ( -2.972980823146582186, 6.690504403638126263, 0.000000000000000000 ) ) ;
#82140=CARTESIAN_POINT ( 'NONE',  ( 6.346625304528514810, 6.577020074804287297, 0.000000000000000000 ) ) ;
#82147=CARTESIAN_POINT ( 'NONE',  ( -4.065465959251405081, 5.836405933916976707, -1.599625672291271394 ) ) ;
#82153=CARTESIAN_POINT ( 'NONE',  ( -7.431277594066152403, 8.802816960232885179, -1.082531754730549967 ) ) ;
#82155=CARTESIAN_POINT ( 'NONE',  ( -3.499413046103020175, 7.096749297179887783, 0.7216878364870338292 ) ) ;
#82171=CARTESIAN_POINT ( 'NONE',  ( -3.688700311369816909, 6.461178242310183784, -1.199719254218450271 ) ) ;
#82183=CARTESIAN_POINT ( 'NONE',  ( -5.829079699232685208, 5.765290835385048496, 0.000000000000000000 ) ) ;
#82192=CARTESIAN_POINT ( 'NONE',  ( -6.050681693448748177, 10.28115541899069463, 0.7998128361456291469 ) ) ;
#82193=CARTESIAN_POINT ( 'NONE',  ( -4.818718062179155659, 8.223694781438435797, -0.9201054579500017594 ) ) ;
#82195=DIRECTION ( 'NONE',  ( 0.6507913734559641616, -0.7592566023653004592, 0.000000000000000000 ) ) ;
#82196=EDGE_LOOP ( 'NONE', ( #88741, #170770, #40429, #118480 ) ) ;
#82212=CARTESIAN_POINT ( 'NONE',  ( 5.580062740476173566, 8.667767742934335828, 1.199719254218451159 ) ) ;
#82236=CARTESIAN_POINT ( 'NONE',  ( 6.852720297064418986, 6.959538199522133262, 0.7998128361456331437 ) ) ;
#82237=CARTESIAN_POINT ( 'NONE',  ( 6.384963997392946844, 6.413822516572072807, 0.7998128361456352531 ) ) ;
#82239=CARTESIAN_POINT ( 'NONE',  ( 5.716698046817569434, 6.698511138489155137, -1.199719254218452047 ) ) ;
#82251=CARTESIAN_POINT ( 'NONE',  ( 4.669458948634179762, 8.398658883068243597, -0.5498995856093937817 ) ) ;
#82252=CARTESIAN_POINT ( 'NONE',  ( -6.590672069574513792, 6.861741300691274859, 0.000000000000000000 ) ) ;
#82253=CARTESIAN_POINT ( 'NONE',  ( 4.638297949650961982, 5.544340708415133712, -1.082531754730548412 ) ) ;
#82276=CARTESIAN_POINT ( 'NONE',  ( 4.366607992053101128, 7.252070536440704096, -1.199719254218448494 ) ) ;
#82278=CARTESIAN_POINT ( 'NONE',  ( 5.585032934186686226, 5.480569609498057382, 0.000000000000000000 ) ) ;
#82299=CARTESIAN_POINT ( 'NONE',  ( -6.077442586152565163, 6.376797013798398694, -0.4802106596381822134 ) ) ;
#82303=SPHERICAL_SURFACE ( 'NONE', #93115, 0.08000000000000000167 ) ;
#82308=CARTESIAN_POINT ( 'NONE',  ( 4.908934136599710563, 7.884784371745123366, 1.199719254218451159 ) ) ;
#82313=CARTESIAN_POINT ( 'NONE',  ( -6.265474751258844677, 6.912123529488261475, 0.7890932636151950508 ) ) ;
#82314=CARTESIAN_POINT ( 'NONE',  ( 4.766573523656222555, 7.718696989977711809, 1.199719254218452047 ) ) ;
#82326=CARTESIAN_POINT ( 'NONE',  ( 4.768187943840554333, 8.164982483533503199, -0.7738548252242994918 ) ) ;
#82334=CARTESIAN_POINT ( 'NONE',  ( 6.048345925472209395, 6.229027465905260463, 0.7216878364870190632 ) ) ;
#82341=CARTESIAN_POINT ( 'NONE',  ( -6.168302983024037900, 6.978022005381355974, 0.9131412519865607091 ) ) ;
#82348=CARTESIAN_POINT ( 'NONE',  ( -6.200875153403786477, 8.327716660428123419, -1.599625672291271394 ) ) ;
#82350=CARTESIAN_POINT ( 'NONE',  ( 5.468734858265785093, 7.473552982767158070, 1.599625672291269396 ) ) ;
#82351=CARTESIAN_POINT ( 'NONE',  ( 8.014278199453780616, 8.522615118883788199, 0.000000000000000000 ) ) ;
#82357=EDGE_LOOP ( 'NONE', ( #120079, #95798, #118310 ) ) ;
#82362=VECTOR ( 'NONE', #89818, 1000.000000000000000 ) ;
#82364=CARTESIAN_POINT ( 'NONE',  ( -6.258858270227934284, 6.997355405945988593, -0.9884160956115575214 ) ) ;
#82378=ORIENTED_EDGE ( 'NONE', *, *, #150147, .F. ) ;
#82381=CARTESIAN_POINT ( 'NONE',  ( 6.048345925472191631, 7.189396680206621149, 1.082531754730549967 ) ) ;
#82389=CARTESIAN_POINT ( 'NONE',  ( -0.4000000000000114575, 2.999999999999999112, 2.023857702507764422 ) ) ;
#82395=CARTESIAN_POINT ( 'NONE',  ( -5.533136088152923904, 6.588318536667425285, 1.082531754730549078 ) ) ;
#82397=CARTESIAN_POINT ( 'NONE',  ( 5.794130544993763898, 7.853181283949808744, 1.599625672291269396 ) ) ;
#82402=CARTESIAN_POINT ( 'NONE',  ( -3.169574050544739841, 6.919863168935977527, -0.7998128361456481317 ) ) ;
#82413=CARTESIAN_POINT ( 'NONE',  ( -1.298432343300637860E-14, 2.519999999999999130, -2.000000000000000000 ) ) ;
#82444=CARTESIAN_POINT ( 'NONE',  ( 5.551137550152489553, 5.441024994791534120, 0.7998128361456352531 ) ) ;
#82450=CARTESIAN_POINT ( 'NONE',  ( -5.926322542504877333, 7.047036066744706950, -1.082531754730549967 ) ) ;
#82458=CARTESIAN_POINT ( 'NONE',  ( -5.936491157937300756, 8.019268665717216749, 1.599625672291263179 ) ) ;
#82462=VERTEX_POINT ( 'NONE', #162724 ) ;
#82465=CYLINDRICAL_SURFACE ( 'NONE', #54817, 1.250000000000000000 ) ;
#82467=CARTESIAN_POINT ( 'NONE',  ( -6.306477729012051725, 7.386587434382707151, 1.199719254218452047 ) ) ;
#82469=CARTESIAN_POINT ( 'NONE',  ( 5.669760509565840323, 7.437725440679550992, 1.325564871123290356 ) ) ;
#82474=CARTESIAN_POINT ( 'NONE',  ( 6.210516883511641772, 9.403297576475722508, 1.199719254218452047 ) ) ;
#82481=CARTESIAN_POINT ( 'NONE',  ( -5.842637852846353397, 5.781108681267656202, 0.7998128361456281477 ) ) ;
#82487=CARTESIAN_POINT ( 'NONE',  ( -4.762657100150483380, 8.778460060142702304, 0.000000000000000000 ) ) ;
#82491=CARTESIAN_POINT ( 'NONE',  ( 7.499068361690118145, 7.921536974826172361, -0.7216878364870317197 ) ) ;
#82493=CARTESIAN_POINT ( 'NONE',  ( -5.926322542504864899, 8.967774495347393682, -1.082531754730549967 ) ) ;
#82499=CARTESIAN_POINT ( 'NONE',  ( 5.692444392891300886, 7.734547439830227411, -1.599625672291281386 ) ) ;
#82513=CARTESIAN_POINT ( 'NONE',  ( 6.246047416222394233, 7.008439898793222156, -0.9866338212708870570 ) ) ;
#82538=EDGE_LOOP ( 'NONE', ( #55416, #146322, #152733, #161467 ) ) ;
#82542=CARTESIAN_POINT ( 'NONE',  ( -4.981341760169012645, 7.953289812593539843, -1.047584607753747399 ) ) ;
#82562=CARTESIAN_POINT ( 'NONE',  ( -3.481411583659053566, 7.283673624236017830, 0.000000000000000000 ) ) ;
#82574=CARTESIAN_POINT ( 'NONE',  ( 5.017399365509065845, 8.011327138806002779, -1.199719254218450271 ) ) ;
#82577=CARTESIAN_POINT ( 'NONE',  ( 6.251718229232841928, 8.387033582228703210, -1.443375672974078761 ) ) ;
#82592=CARTESIAN_POINT ( 'NONE',  ( -5.285699784481336927, 7.260012063351913625, 1.599625672291263179 ) ) ;
#82594=CARTESIAN_POINT ( 'NONE',  ( 3.393283585170187688, 7.180857625999046867, 0.7998128361456271485 ) ) ;
#82603=CARTESIAN_POINT ( 'NONE',  ( -4.516801452008150086, 5.298631777878131111, 1.199719254218452935 ) ) ;
#82604=CARTESIAN_POINT ( 'NONE',  ( 6.475954649182838807, 7.584310507915338562, 1.199719254218452047 ) ) ;
#82611=CARTESIAN_POINT ( 'NONE',  ( 5.564695703766185275, 5.456842840674144490, 0.000000000000000000 ) ) ;
#82617=CARTESIAN_POINT ( 'NONE',  ( -6.569648045741773856, 6.787758985223060648, 0.3860807628459517749 ) ) ;
#82621=EDGE_CURVE ( 'NONE', #145598, #53161, #46752, .T. ) ;
#82626=CARTESIAN_POINT ( 'NONE',  ( -8.120407659942227241, 8.438506789546210030, 0.7998128361456341429 ) ) ;
#82632=CARTESIAN_POINT ( 'NONE',  ( -2.278321918429671467, 2.687264847271879198, 2.500000000000000444 ) ) ;
#82643=EDGE_CURVE ( 'NONE', #68330, #127411, #59777, .T. ) ;
#82658=CARTESIAN_POINT ( 'NONE',  ( 3.901714345682657292, 7.774026846596938434, 0.7998128361456271485 ) ) ;
#82678=CARTESIAN_POINT ( 'NONE',  ( 3.691562964670865199, 7.528850235416478576, -0.7998128361456362523 ) ) ;
#82679=CARTESIAN_POINT ( 'NONE',  ( -5.343321937561608337, 5.406499480009534508, 0.7216878364870257245 ) ) ;
#82682=( BOUNDED_CURVE ( )  B_SPLINE_CURVE ( 2, ( #108988, #143598, #27664 ),
 .UNSPECIFIED., .F., .T. ) 
 B_SPLINE_CURVE_WITH_KNOTS ( ( 3, 3 ),
 ( 0.000000000000000000, 0.004569332664469506929 ),
 .UNSPECIFIED. ) 
 CURVE ( )  GEOMETRIC_REPRESENTATION_ITEM ( )  RATIONAL_B_SPLINE_CURVE ( ( 1.000000000000000000, 0.9265390601563747719, 0.9336383135903749686 ) ) 
 REPRESENTATION_ITEM ( '' )  );
#82707=CARTESIAN_POINT ( 'NONE',  ( -6.154475385960665790, 6.144919136567696505, 0.000000000000000000 ) ) ;
#82710=CARTESIAN_POINT ( 'NONE',  ( 6.875393295461478260, 8.154285278527437342, -1.082531754730548412 ) ) ;
#82716=CARTESIAN_POINT ( 'NONE',  ( -5.794130544993808307, 7.853181283949808744, 1.599625672291263179 ) ) ;
#82725=CARTESIAN_POINT ( 'NONE',  ( -5.250750630242457362, 9.347902511916677426, 0.000000000000000000 ) ) ;
#82733=CARTESIAN_POINT ( 'NONE',  ( 3.040771591214902259, 6.769593633051179005, -0.7998128361456362523 ) ) ;
#82740=CARTESIAN_POINT ( 'NONE',  ( -6.608673532018475960, 6.674816973635147477, -0.7998128361456362523 ) ) ;
#82743=CARTESIAN_POINT ( 'NONE',  ( -6.292392690518202159, 9.394856334696294553, -1.082531754730549967 ) ) ;
#82745=CARTESIAN_POINT ( 'NONE',  ( -7.417719440008134768, 7.826629899530511025, 0.7216878364870317197 ) ) ;
#82746=CARTESIAN_POINT ( 'NONE',  ( 5.989670002187236442, 10.20997511251894529, -0.7998128361456481317 ) ) ;
#82747=CARTESIAN_POINT ( 'NONE',  ( -4.462041952228957165, 5.338708711422782471, -1.082531754730549967 ) ) ;
#82766=CARTESIAN_POINT ( 'NONE',  ( 6.231590709102786008, 7.018523052454695765, 1.002697108273574500 ) ) ;
#82772=CARTESIAN_POINT ( 'NONE',  ( 5.591026288145455325, 7.491806139540827303, -1.383104942081718969 ) ) ;
#82785=EDGE_CURVE ( 'NONE', #130236, #69840, #165906, .T. ) ;
#82787=CARTESIAN_POINT ( 'NONE',  ( 6.080034374691865473, 7.023743017405461586, -0.9950221519831742301 ) ) ;
#82799=CARTESIAN_POINT ( 'NONE',  ( 6.176621499477501054, 9.363752961769195693, -1.199719254218452047 ) ) ;
#82802=CARTESIAN_POINT ( 'NONE',  ( -4.034433228518296666, 6.864533312316751790, -1.199719254218450271 ) ) ;
#82816=CARTESIAN_POINT ( 'NONE',  ( 5.061990249855835344, 6.999017606288844284, -1.599625672291273171 ) ) ;
#82818=CARTESIAN_POINT ( 'NONE',  ( 6.505933609711257226, 8.683618192786854095, -1.599625672291281386 ) ) ;
#82824=CARTESIAN_POINT ( 'NONE',  ( -5.736508391913536897, 9.706693867292189637, 0.7216878364870267237 ) ) ;
#82830=CARTESIAN_POINT ( 'NONE',  ( 7.523848900940885542, 7.742521570711348389, 0.7998128361456291469 ) ) ;
#82843=CARTESIAN_POINT ( 'NONE',  ( -6.346625304972878467, 7.537389289624049304, 1.082531754730548412 ) ) ;
#82845=CARTESIAN_POINT ( 'NONE',  ( 3.906157654512984134, 7.571284673658201569, -0.7216878364870338292 ) ) ;
#82855=CARTESIAN_POINT ( 'NONE',  ( -4.309512724297390740, 6.121127159803966933, 1.599625672291270506 ) ) ;
#82856=CARTESIAN_POINT ( 'NONE',  ( -6.970300371201519241, 7.304640985922785212, 0.7216878364870317197 ) ) ;
#82857=CARTESIAN_POINT ( 'NONE',  ( 1.843539612419922813, 2.497715572767779335, -2.492262248206851272 ) ) ;
#82861=CARTESIAN_POINT ( 'NONE',  ( 5.709392084686216506, 5.833581318321598985, -0.7216878364870458196 ) ) ;
#82878=CARTESIAN_POINT ( 'NONE',  ( -5.842637852846353397, 5.781108681267656202, 0.7998128361456281477 ) ) ;
#82890=EDGE_CURVE ( 'NONE', #111999, #66325, #101969, .T. ) ;
#82891=CARTESIAN_POINT ( 'NONE',  ( 4.523580528814945545, 5.306540700819438960, 1.199719254218452047 ) ) ;
#82894=CARTESIAN_POINT ( 'NONE',  ( 4.532168488718122390, 8.509556680138327778, 0.7998128361456271485 ) ) ;
#82918=VERTEX_POINT ( 'NONE', #33763 ) ;
#82927=B_SPLINE_CURVE_WITH_KNOTS ( 'NONE', 3,
 ( #7959, #154235, #75116, #39411 ),
 .UNSPECIFIED., .F., .F.,
 ( 4, 4 ),
 ( 0.000000000000000000, 0.0003462261082409072736 ),
 .UNSPECIFIED. ) ;
#82929=CARTESIAN_POINT ( 'NONE',  ( 5.234856708652233515, 6.240325927249993576, 1.082531754730549078 ) ) ;
#82935=CARTESIAN_POINT ( 'NONE',  ( 4.787437638956922648, 6.678706226906775179, -1.443375672974068769 ) ) ;
#82948=CARTESIAN_POINT ( 'NONE',  ( -5.769876891067536206, 8.889217585290882795, 1.199719254218454489 ) ) ;
#82953=CARTESIAN_POINT ( 'NONE',  ( 4.542476715900265916, 4.951051008190067826, -0.8264431066547142102 ) ) ;
#82957=CARTESIAN_POINT ( 'NONE',  ( 6.176621499477501054, 9.363752961769195693, -1.199719254218452047 ) ) ;
#82962=CYLINDRICAL_SURFACE ( 'NONE', #75086, 0.08000000000000020983 ) ;
#82963=CARTESIAN_POINT ( 'NONE',  ( -8.100070429521727178, 8.414780020722290033, 0.7998128361456341429 ) ) ;
#82970=CARTESIAN_POINT ( 'NONE',  ( -5.966997003790228682, 8.054858819212300958, -1.443375672974066548 ) ) ;
#82973=CARTESIAN_POINT ( 'NONE',  ( -5.641074431737709283, 8.738948049406083385, -1.199719254218452047 ) ) ;
#82994=CARTESIAN_POINT ( 'NONE',  ( -4.678972410047611774, 5.591794245544547515, 1.082531754730549078 ) ) ;
#82995=CARTESIAN_POINT ( 'NONE',  ( 4.923546060418115822, 5.773167154356443120, -1.199719254218452047 ) ) ;
#82996=CARTESIAN_POINT ( 'NONE',  ( -4.457598643843001973, 8.422558527783969851, 0.000000000000000000 ) ) ;
#83016=CARTESIAN_POINT ( 'NONE',  ( 4.082413651490639062, 7.776916670132135501, 0.000000000000000000 ) ) ;
#83020=CARTESIAN_POINT ( 'NONE',  ( -6.420668264523499147, 9.648474187656182366, 1.199719254218452935 ) ) ;
#83048=CARTESIAN_POINT ( 'NONE',  ( 4.248501033035879004, 6.049946853332221153, -1.599625672291273171 ) ) ;
#83060=CARTESIAN_POINT ( 'NONE',  ( 4.615647837050825153, 8.347533190886938570, 0.2882115401751338402 ) ) ;
#83062=CARTESIAN_POINT ( 'NONE',  ( 5.063044020060520900, 4.871582543017558109, 0.7998128361456352531 ) ) ;
#83067=CARTESIAN_POINT ( 'NONE',  ( -4.274563570058511175, 8.209017608368725405, 0.000000000000000000 ) ) ;
#83080=CARTESIAN_POINT ( 'NONE',  ( 4.895902868310594513, 8.725987423088758632, 0.000000000000000000 ) ) ;
#83083=EDGE_CURVE ( 'NONE', #211313, #95167, #156899, .T. ) ;
#83084=CARTESIAN_POINT ( 'NONE',  ( -4.472210567661380587, 6.310941310395290493, 1.599625672291270506 ) ) ;
#83095=CARTESIAN_POINT ( 'NONE',  ( 3.067887898442204442, 6.801229324816399746, 0.7998128361456271485 ) ) ;
#83096=CARTESIAN_POINT ( 'NONE',  ( 4.386945222473598527, 7.275797305264619652, -1.199719254218452047 ) ) ;
#83108=ORIENTED_EDGE ( 'NONE', *, *, #100532, .F. ) ;
#83114=CARTESIAN_POINT ( 'NONE',  ( 3.188928480291414846, 8.980740528189164351, -2.451733079074511767 ) ) ;
#83119=CARTESIAN_POINT ( 'NONE',  ( 5.724925646405265134, 7.336609705370862322, 1.269948841093468506 ) ) ;
#83121=CARTESIAN_POINT ( 'NONE',  ( 5.820193082016415609, 10.01225203898631655, 0.000000000000000000 ) ) ;
#83128=CARTESIAN_POINT ( 'NONE',  ( 7.191674137406095291, 7.354984346587396082, 0.000000000000000000 ) ) ;
#83129=DIRECTION ( 'NONE',  ( 0.000000000000000000, 0.000000000000000000, -1.000000000000000000 ) ) ;
#83137=CARTESIAN_POINT ( 'NONE',  ( 3.770576118376296471, 7.413106214832098750, 0.7216878364870257245 ) ) ;
#83139=CARTESIAN_POINT ( 'NONE',  ( 4.858757509019037357, 5.629766575900002401, 2.499999999999999556 ) ) ;
#83140=CARTESIAN_POINT ( 'NONE',  ( 6.156811154381533591, 9.236677875870187293, -1.082531754730548412 ) ) ;
#83151=CARTESIAN_POINT ( 'NONE',  ( -6.455090533882206216, 7.663932056684933158, -1.082531754730549967 ) ) ;
#83168=ORIENTED_EDGE ( 'NONE', *, *, #180932, .F. ) ;
#83180=ORIENTED_EDGE ( 'NONE', *, *, #121643, .T. ) ;
#83184=CARTESIAN_POINT ( 'NONE',  ( 5.182959862174088883, 9.268813282503625572, 0.7998128361456331437 ) ) ;
#83186=CARTESIAN_POINT ( 'NONE',  ( 5.845500506147374153, 6.848780674373954547, 1.199719254218453823 ) ) ;
#83199=CARTESIAN_POINT ( 'NONE',  ( -5.307090785106547415, 5.156303768904543894, -0.7998128361456362523 ) ) ;
#83201=CARTESIAN_POINT ( 'NONE',  ( 5.438229012412886476, 7.437962829272074750, -1.443375672974078761 ) ) ;
#83202=EDGE_CURVE ( 'NONE', #162782, #6739, #2564, .T. ) ;
#83210=CARTESIAN_POINT ( 'NONE',  ( -3.471769853551161411, 6.208092708188416076, 1.199719254218452935 ) ) ;
#83217=CARTESIAN_POINT ( 'NONE',  ( -6.699137298928187434, 8.909022496873262753, 1.443375672974064550 ) ) ;
#83219=CARTESIAN_POINT ( 'NONE',  ( -4.828112100242291760, 6.726159765073026264, -1.443375672974066548 ) ) ;
#83226=CARTESIAN_POINT ( 'NONE',  ( 3.231779075379134003, 6.036511184309971689, 7.500000000000000000 ) ) ;
#83228=FACE_OUTER_BOUND ( 'NONE', #182151, .T. ) ;
#83233=CARTESIAN_POINT ( 'NONE',  ( -3.902768115887413014, 5.646591783325653147, -1.599625672291283607 ) ) ;
#83234=ORIENTED_EDGE ( 'NONE', *, *, #32740, .T. ) ;
#83244=CARTESIAN_POINT ( 'NONE',  ( -3.006876207180748217, 6.730049018344652190, -0.7998128361456481317 ) ) ;
#83247=CARTESIAN_POINT ( 'NONE',  ( 5.526144005543697446, 7.442112546579989996, -1.248357989223557452 ) ) ;
#83256=CARTESIAN_POINT ( 'NONE',  ( -5.645675577465527617, 7.454724071444114308, -1.341317915573495334 ) ) ;
#83271=CARTESIAN_POINT ( 'NONE',  ( 7.035755370848908896, 7.173079118937375931, 0.7998128361456352531 ) ) ;
#83296=EDGE_CURVE ( 'NONE', #105328, #172895, #167249, .T. ) ;
#83297=CARTESIAN_POINT ( 'NONE',  ( 5.885121196783658526, 9.023669275293071834, 1.199719254218452047 ) ) ;
#83298=CARTESIAN_POINT ( 'NONE',  ( 5.143339171537801846, 7.093924681584509173, 1.599625672291269396 ) ) ;
#83300=CARTESIAN_POINT ( 'NONE',  ( 5.499767588998890844, 6.445425604367387429, 1.199719254218451159 ) ) ;
#83310=CARTESIAN_POINT ( 'NONE',  ( 5.726091835933811325, 7.283405380927965744, -1.209259067671350163 ) ) ;
#83312=CARTESIAN_POINT ( 'NONE',  ( -4.597623488365601752, 8.377994813152914944, 0.7216878364870267237 ) ) ;
#83313=CARTESIAN_POINT ( 'NONE',  ( 5.261973015879598314, 5.311592404713873172, -0.7216878364870458196 ) ) ;
#83332=ORIENTED_EDGE ( 'NONE', *, *, #175741, .F. ) ;
#83339=CARTESIAN_POINT ( 'NONE',  ( 6.554440917563797875, 6.611545590104705994, -0.7998128361456481317 ) ) ;
#83340=CARTESIAN_POINT ( 'NONE',  ( 2.911969131885072670, 6.619324097166378706, 0.000000000000000000 ) ) ;
#83365=DIRECTION ( 'NONE',  ( 0.000000000000000000, 0.000000000000000000, 1.000000000000000000 ) ) ;
#83371=CARTESIAN_POINT ( 'NONE',  ( 7.693325821111733021, 7.940244644243982464, -0.7998128361456341429 ) ) ;
#83376=CARTESIAN_POINT ( 'NONE',  ( -6.160225556963538018, 6.983552031129079296, 0.9223575212774417498 ) ) ;
#83377=CARTESIAN_POINT ( 'NONE',  ( 7.686546744304875389, 7.932335721302671949, 0.7998128361456291469 ) ) ;
#83383=VERTEX_POINT ( 'NONE', #55744 ) ;
#83389=CARTESIAN_POINT ( 'NONE',  ( 1.833506991698445443, 2.501547993919093660, 2.496244204820597723 ) ) ;
#83396=CYLINDRICAL_SURFACE ( 'NONE', #18147, 1.250000000000000000 ) ;
#83407=FACE_OUTER_BOUND ( 'NONE', #210112, .T. ) ;
#83412=CARTESIAN_POINT ( 'NONE',  ( -6.957269102468015554, 8.145844036748005834, 1.199719254218452047 ) ) ;
#83414=CARTESIAN_POINT ( 'NONE',  ( 5.677832469072920496, 9.846164657218904992, 0.000000000000000000 ) ) ;
#83419=CARTESIAN_POINT ( 'NONE',  ( -3.174017359375036929, 6.717120995997236221, 0.7216878364870338292 ) ) ;
#83428=CARTESIAN_POINT ( 'NONE',  ( -6.600870636098118638, 6.767368133241304484, -0.2259646751960984468 ) ) ;
#83436=CARTESIAN_POINT ( 'NONE',  ( 5.806634928402749196, 9.996434193103704402, -0.7998128361456481317 ) ) ;
#83447=CARTESIAN_POINT ( 'NONE',  ( 6.373741612200162443, 8.529394195690610303, 1.443375672974065660 ) ) ;
#83449=CARTESIAN_POINT ( 'NONE',  ( 0.000000000000000000, 8.920000000000001705, 0.000000000000000000 ) ) ;
#83460=CARTESIAN_POINT ( 'NONE',  ( -4.177320726786319049, 6.927272377009067839, -1.082531754730551743 ) ) ;
#83462=CARTESIAN_POINT ( 'NONE',  ( 6.886615681098613884, 6.999082814228660077, 0.000000000000000000 ) ) ;
#83466=CIRCLE ( 'NONE', #45471, 0.08000000000000020983 ) ;
#83468=CARTESIAN_POINT ( 'NONE',  ( -3.980200614063634568, 6.801261928786307642, 1.199719254218452935 ) ) ;
#83476=VERTEX_POINT ( 'NONE', #140235 ) ;
#83506=CARTESIAN_POINT ( 'NONE',  ( 2.957086901556340575, 6.464035461875470290, 0.7216878364870257245 ) ) ;
#83511=CARTESIAN_POINT ( 'NONE',  ( 5.740951700743842423, 5.662474837148078421, -0.7998128361456481317 ) ) ;
#83517=CARTESIAN_POINT ( 'NONE',  ( -6.278834536460198734, 6.497930845391236332, 0.7216878364870257245 ) ) ;
#83524=CARTESIAN_POINT ( 'NONE',  ( -5.641074431737709283, 8.738948049406083385, -1.199719254218452047 ) ) ;
#83533=CARTESIAN_POINT ( 'NONE',  ( -7.144220599758281054, 7.299621885998258897, 0.7998128361456341429 ) ) ;
#83535=ORIENTED_EDGE ( 'NONE', *, *, #19728, .F. ) ;
#83536=CARTESIAN_POINT ( 'NONE',  ( 4.895464504754282409, 8.144056917144915531, 1.010406422583273178 ) ) ;
#83542=CARTESIAN_POINT ( 'NONE',  ( 5.182959862174088883, 9.268813282503625572, 0.7998128361456331437 ) ) ;
#83549=CARTESIAN_POINT ( 'NONE',  ( -4.468294144155606773, 7.370704380560280100, 1.199719254218452935 ) ) ;
#83553=CARTESIAN_POINT ( 'NONE',  ( -5.855142236255304944, 7.924361590421551860, -1.599625672291271394 ) ) ;
#83557=CARTESIAN_POINT ( 'NONE',  ( 7.634649897826744080, 9.040084647953621655, 1.082531754730549078 ) ) ;
#83559=CARTESIAN_POINT ( 'NONE',  ( -7.729556973122450714, 8.190440354830551328, 0.000000000000000000 ) ) ;
#83565=CARTESIAN_POINT ( 'NONE',  ( 7.015418140428412386, 7.149352350113456822, 0.7998128361456331437 ) ) ;
#83575=( NAMED_UNIT ( * ) SI_UNIT ( $, .STERADIAN. ) SOLID_ANGLE_UNIT ( ) );
#83577=DIRECTION ( 'NONE',  ( 1.000000000000000000, 0.000000000000000000, 0.000000000000000000 ) ) ;
#83582=CARTESIAN_POINT ( 'NONE',  ( 6.512538272292041519, 6.827515365185738538, -0.5364851146780359459 ) ) ;
#83595=EDGE_LOOP ( 'NONE', ( #79480, #42671, #67609, #76541 ) ) ;
#83597=CARTESIAN_POINT ( 'NONE',  ( -4.109529958273621553, 7.808552361378945150, 0.7216878364870283891 ) ) ;
#83605=CARTESIAN_POINT ( 'NONE',  ( 7.842465510862060896, 8.114240948952696542, 0.000000000000000000 ) ) ;
#83610=CARTESIAN_POINT ( 'NONE',  ( -4.945771867956824330, 7.989995641179508112, -1.012621479200847441 ) ) ;
#83624=CARTESIAN_POINT ( 'NONE',  ( 3.719872605471085336, 6.605953636083950364, 2.420000000000000373 ) ) ;
#83628=CARTESIAN_POINT ( 'NONE',  ( -5.330290668828105538, 6.247702530834755130, 1.199719254218452935 ) ) ;
#83630=CARTESIAN_POINT ( 'NONE',  ( 6.339319342841494453, 9.553567112360518365, -1.199719254218452047 ) ) ;
#83639=CARTESIAN_POINT ( 'NONE',  ( 6.692885107001518286, 7.837396042037102717, -1.199719254218452047 ) ) ;
#83642=CARTESIAN_POINT ( 'NONE',  ( 7.309254211098767051, 7.700087132469628948, 0.7216878364870267237 ) ) ;
#83656=CARTESIAN_POINT ( 'NONE',  ( -5.529746549527323474, 7.544733289238903851, -1.599625672291271394 ) ) ;
#83657=CARTESIAN_POINT ( 'NONE',  ( 5.252858170651868441, 5.093032385374103299, -0.7998128361456481317 ) ) ;
#83662=ORIENTED_EDGE ( 'NONE', *, *, #212227, .T. ) ;
#83665=CARTESIAN_POINT ( 'NONE',  ( -5.029148636026397945, 4.832037928311032182, 0.7998128361456281477 ) ) ;
#83666=CARTESIAN_POINT ( 'NONE',  ( 5.885121196783658526, 9.023669275293071834, 1.199719254218452047 ) ) ;
#83673=DIRECTION ( 'NONE',  ( 0.000000000000000000, -1.000000000000000000, 0.000000000000000000 ) ) ;
#83674=CARTESIAN_POINT ( 'NONE',  ( 5.228604516725597229, 6.129068686715179126, -1.199719254218450271 ) ) ;
#83681=VECTOR ( 'NONE', #187382, 1000.000000000000114 ) ;
#83682=CARTESIAN_POINT ( 'NONE',  ( -6.198085906554800850, 7.039857339855744023, 1.052733950999720003 ) ) ;
#83692=CARTESIAN_POINT ( 'NONE',  ( -5.772739544368596043, 9.956889578397179363, -0.7998128361456362523 ) ) ;
#83698=CARTESIAN_POINT ( 'NONE',  ( -3.620328817674902666, 3.489345133412038447, 2.447831560964403685 ) ) ;
#83712=CARTESIAN_POINT ( 'NONE',  ( -6.337068562759858636, 6.936200024879327408, -0.9492287992594623525 ) ) ;
#83724=CARTESIAN_POINT ( 'NONE',  ( 5.306037014901791693, 7.283738832175834510, 1.599625672291269396 ) ) ;
#83744=CIRCLE ( 'NONE', #18019, 1.250000000000000444 ) ;
#83745=CARTESIAN_POINT ( 'NONE',  ( 3.854260808034858155, 7.718664386007802136, -0.7998128361456362523 ) ) ;
#83772=CARTESIAN_POINT ( 'NONE',  ( -5.582925393777276035, 9.735439736040634173, 0.7998128361456291469 ) ) ;
#83786=CARTESIAN_POINT ( 'NONE',  ( -6.237633190739009237, 9.434933268240943249, 1.199719254218452047 ) ) ;
#83793=CARTESIAN_POINT ( 'NONE',  ( 2.891631901464575272, 6.595597328342462262, 0.000000000000000000 ) ) ;
#83796=EDGE_CURVE ( 'NONE', #129718, #95637, #90470, .T. ) ;
#83799=CARTESIAN_POINT ( 'NONE',  ( -4.098307573080856692, 8.003385611894792362, 0.7998128361456352531 ) ) ;
#83802=CARTESIAN_POINT ( 'NONE',  ( -6.943184063974178422, 8.233374508458908281, -1.082531754730549967 ) ) ;
#83805=CARTESIAN_POINT ( 'NONE',  ( 3.512971199272317602, 6.152197928242737923, -1.082531754730549967 ) ) ;
#83807=CARTESIAN_POINT ( 'NONE',  ( -4.678972410047611774, 5.591794245544547515, 1.082531754730549078 ) ) ;
#83825=CARTESIAN_POINT ( 'NONE',  ( 6.533654944624902150, 6.813559398729744032, -0.4760831665120857648 ) ) ;
#83847=CARTESIAN_POINT ( 'NONE',  ( 6.373787108001086388, 6.824503602047865769, -0.5760177672454840359 ) ) ;
#83861=CARTESIAN_POINT ( 'NONE',  ( 5.528692779322568640, 9.672168352510192690, 0.7998128361456341429 ) ) ;
#83864=CARTESIAN_POINT ( 'NONE',  ( -4.444040490229335560, 8.406740681901359480, 0.7998128361456352531 ) ) ;
#83877=CARTESIAN_POINT ( 'NONE',  ( 3.953084306836263995, 6.769626237021087789, 1.199719254218452047 ) ) ;
#83880=CARTESIAN_POINT ( 'NONE',  ( 5.345657705538078730, 9.458627433094950021, 0.7998128361456331437 ) ) ;
#83885=CARTESIAN_POINT ( 'NONE',  ( -7.404161286394468355, 7.810812053647902431, 0.000000000000000000 ) ) ;
#83890=CARTESIAN_POINT ( 'NONE',  ( 6.607619761813720238, 8.802252036906432764, 1.599625672291268286 ) ) ;
#83904=CARTESIAN_POINT ( 'NONE',  ( -5.099275172515603138, 8.002885897026576600, 1.082531754730549967 ) ) ;
#83905=CARTESIAN_POINT ( 'NONE',  ( 6.373741612200174878, 6.608655767087927124, 0.7216878364870328300 ) ) ;
#83915=CARTESIAN_POINT ( 'NONE',  ( -4.984557751679625781, 5.844347460828191565, 1.199719254218452935 ) ) ;
#83916=CARTESIAN_POINT ( 'NONE',  ( -7.621091744657483069, 8.063897588288083895, 0.7216878364870317197 ) ) ;
#83917=CARTESIAN_POINT ( 'NONE',  ( 6.016786309414542622, 10.24161080428416426, 0.7998128361456341429 ) ) ;
#83920=CARTESIAN_POINT ( 'NONE',  ( 3.702785349863636277, 7.334016984900627811, -0.7216878364870338292 ) ) ;
#83927=DIRECTION ( 'NONE',  ( 8.881784197001252323E-16, 0.000000000000000000, 1.000000000000000000 ) ) ;
#83933=CARTESIAN_POINT ( 'NONE',  ( -6.325812300595961446, 6.871976577178664058, 0.6903976412777796945 ) ) ;
#83938=CARTESIAN_POINT ( 'NONE',  ( 4.312902262922978736, 5.164712407232485702, -1.082531754730548412 ) ) ;
#83941=CARTESIAN_POINT ( 'NONE',  ( -5.764151584465413869, 6.753873599078290546, -1.199719254218453823 ) ) ;
#83953=CARTESIAN_POINT ( 'NONE',  ( 5.225741863424510747, 5.061396693608882558, 0.7998128361456352531 ) ) ;
#83993=CARTESIAN_POINT ( 'NONE',  ( 6.238160076063542725, 6.450477308261824305, -0.7216878364870458196 ) ) ;
#83998=CARTESIAN_POINT ( 'NONE',  ( 5.139949632912227173, 8.050339434155988627, -1.082531754730548412 ) ) ;
#84012=CARTESIAN_POINT ( 'NONE',  ( -6.363572996767778100, 8.517530811019446091, -1.599625672291271394 ) ) ;
#84024=CARTESIAN_POINT ( 'NONE',  ( 4.706088717274906408, 5.623429937309770921, 1.082531754730549078 ) ) ;
#84031=CARTESIAN_POINT ( 'NONE',  ( -6.291865805193673111, 9.498204651771386509, -1.199719254218452047 ) ) ;
#84037=CARTESIAN_POINT ( 'NONE',  ( -5.885648082108231982, 7.959951743916638733, 1.443375672974058777 ) ) ;
#84041=CARTESIAN_POINT ( 'NONE',  ( -4.613517410400161722, 8.604463755433990002, -0.7998128361456362523 ) ) ;
#84064=CARTESIAN_POINT ( 'NONE',  ( -6.312203035614172286, 9.521931420595302953, -1.199719254218452047 ) ) ;
#84065=CARTESIAN_POINT ( 'NONE',  ( 4.934241560730721510, 4.721313007132757811, 0.000000000000000000 ) ) ;
#84067=CARTESIAN_POINT ( 'NONE',  ( -4.411198876399886615, 6.239761003923544713, -1.599625672291271394 ) ) ;
#84068=CARTESIAN_POINT ( 'NONE',  ( -6.479871072688648148, 6.524547437750345402, 0.000000000000000000 ) ) ;
#84069=EDGE_LOOP ( 'NONE', ( #63742, #75788, #148613, #202992 ) ) ;
#84076=ORIENTED_EDGE ( 'NONE', *, *, #211296, .T. ) ;
#84091=CARTESIAN_POINT ( 'NONE',  ( 0.000000000000000000, 8.920000000000001705, 2.080000000000000071 ) ) ;
#84124=CARTESIAN_POINT ( 'NONE',  ( 3.898851692381625877, 6.706354853490643642, -1.199719254218452047 ) ) ;
#84137=CARTESIAN_POINT ( 'NONE',  ( 4.622017735560743468, 8.339529265130579461, 0.3277269337885590494 ) ) ;
#84139=CARTESIAN_POINT ( 'NONE',  ( 3.902768115887398803, 5.646591783325653147, -1.599625672291269396 ) ) ;
#84144=VERTEX_POINT ( 'NONE', #149814 ) ;
#84145=CARTESIAN_POINT ( 'NONE',  ( -6.798487682609798632, 6.896266815991691779, 0.7998128361456341429 ) ) ;
#84151=CARTESIAN_POINT ( 'NONE',  ( -6.902509602688818191, 9.146290184594002781, -1.443375672974066548 ) ) ;
#84159=CARTESIAN_POINT ( 'NONE',  ( 5.560252395380206991, 7.580323442733986283, 1.443375672974065660 ) ) ;
#84162=CARTESIAN_POINT ( 'NONE',  ( -4.610654757099099221, 7.536791762327691657, 1.199719254218452935 ) ) ;
#84173=CARTESIAN_POINT ( 'NONE',  ( 4.797606254389322089, 6.690569611577942943, 1.599625672291268286 ) ) ;
#84174=CARTESIAN_POINT ( 'NONE',  ( 5.747730777550676073, 5.670383760089384495, 0.000000000000000000 ) ) ;
#84197=CARTESIAN_POINT ( 'NONE',  ( 5.833751235630055376, 10.02806988486892514, 0.7998128361456331437 ) ) ;
#84207=CARTESIAN_POINT ( 'NONE',  ( 5.169401708560450004, 9.252995436621013425, 0.000000000000000000 ) ) ;
#84212=EDGE_CURVE ( 'NONE', #199345, #172448, #49227, .T. ) ;
#84213=CARTESIAN_POINT ( 'NONE',  ( 3.607878275012302627, 7.223292064240769861, 0.7216878364870257245 ) ) ;
#84216=CARTESIAN_POINT ( 'NONE',  ( 5.058600711674583472, 8.915801573680086634, 0.000000000000000000 ) ) ;
#84217=VERTEX_POINT ( 'NONE', #104261 ) ;
#84228=CARTESIAN_POINT ( 'NONE',  ( 6.170003545802125622, 6.961323287618347955, -0.9016653442153206299 ) ) ;
#84229=CARTESIAN_POINT ( 'NONE',  ( -7.607533591043815768, 8.048079742405473525, 0.000000000000000000 ) ) ;
#84261=EDGE_LOOP ( 'NONE', ( #56734, #76031, #175435, #191749, #84715, #119248, #88627, #16560, #209806, #44133, #136308, #158532, #212569, #118606, #139970, #126515, #160354, #59223, #187636 ) ) ;
#84265=CARTESIAN_POINT ( 'NONE',  ( 7.666209513884374438, 7.908608952478760834, 0.7998128361456281477 ) ) ;
#84267=CARTESIAN_POINT ( 'NONE',  ( 7.361151057576892143, 7.552707420120024828, 0.7998128361456291469 ) ) ;
#84279=CARTESIAN_POINT ( 'NONE',  ( -6.134138155540168391, 6.121192367743780949, 0.000000000000000000 ) ) ;
#84281=CARTESIAN_POINT ( 'NONE',  ( 5.519577934094852978, 7.532869904567736974, 1.443375672974064550 ) ) ;
#84290=CARTESIAN_POINT ( 'NONE',  ( -2.959422669532919326, 6.674686557755516780, 0.7998128361456352531 ) ) ;
#84296=CARTESIAN_POINT ( 'NONE',  ( -6.997416678428844072, 8.296645891989347987, 1.082531754730549078 ) ) ;
#84298=CARTESIAN_POINT ( 'NONE',  ( -4.936577329151611515, 7.813071746435248599, 1.082531754730549967 ) ) ;
#84323=CARTESIAN_POINT ( 'NONE',  ( -4.655245641445871385, 6.524482229810530498, 1.599625672291263179 ) ) ;
#84335=CARTESIAN_POINT ( 'NONE',  ( -4.992018142146231519, 8.041046192835899831, -1.132135330316372590 ) ) ;
#84353=CARTESIAN_POINT ( 'NONE',  ( 5.176180785367283654, 9.260904359562321275, -0.7998128361456481317 ) ) ;
#84368=EDGE_CURVE ( 'NONE', #180652, #142732, #3776, .T. ) ;
#84378=CARTESIAN_POINT ( 'NONE',  ( 6.505933609711257226, 8.683618192786854095, -1.599625672291281386 ) ) ;
#84379=CARTESIAN_POINT ( 'NONE',  ( 6.222266154028957885, 6.224008365980749247, 0.7998128361456352531 ) ) ;
#84381=CARTESIAN_POINT ( 'NONE',  ( 5.554000203453580475, 6.508696987897830688, -1.199719254218452047 ) ) ;
#84385=CARTESIAN_POINT ( 'NONE',  ( -6.966220764712169000, 6.002124920821316323, -2.500000000000000444 ) ) ;
#84394=CARTESIAN_POINT ( 'NONE',  ( 4.634937608369048334, 8.440560775401745985, -0.4060563726728562139 ) ) ;
#84395=CARTESIAN_POINT ( 'NONE',  ( -5.275531169048901958, 8.208517892982092334, -1.082531754730549967 ) ) ;
#84396=CARTESIAN_POINT ( 'NONE',  ( 4.177320726786311056, 5.966903162707725805, -1.443375672974068769 ) ) ;
#84415=CARTESIAN_POINT ( 'NONE',  ( -4.977251789548269301, 4.979417640660637190, 0.7216878364870257245 ) ) ;
#84421=CARTESIAN_POINT ( 'NONE',  ( 5.773793314573267388, 7.829454515125894964, 1.599625672291268286 ) ) ;
#84428=DIRECTION ( 'NONE',  ( -1.000000000000000000, 0.000000000000000000, 0.000000000000000000 ) ) ;
#84436=CARTESIAN_POINT ( 'NONE',  ( 5.594708818112484217, 5.774250729507365953, 0.6894988139244705438 ) ) ;
#84439=CARTESIAN_POINT ( 'NONE',  ( -4.558393992215756363, 7.582615019230624753, -1.001024991534285702 ) ) ;
#84448=CARTESIAN_POINT ( 'NONE',  ( 6.210516883511641772, 9.403297576475722508, 1.199719254218452047 ) ) ;
#84452=CARTESIAN_POINT ( 'NONE',  ( -5.157723666773176063, 7.780300641499326098, 1.171761296108381201 ) ) ;
#84453=CARTESIAN_POINT ( 'NONE',  ( 5.528692779322568640, 9.672168352510192690, 0.7998128361456341429 ) ) ;
#84460=CARTESIAN_POINT ( 'NONE',  ( -1.899821779672251632, 8.994870868756308369, 0.7750000000000013545 ) ) ;
#84476=EDGE_CURVE ( 'NONE', #56229, #138513, #95291, .T. ) ;
#84483=CARTESIAN_POINT ( 'NONE',  ( -6.607619761813764647, 8.802252036906432764, 1.599625672291269396 ) ) ;
#84485=CARTESIAN_POINT ( 'NONE',  ( 6.658989722967328717, 7.797851427330578566, 1.199719254218452935 ) ) ;
#84503=ADVANCED_FACE ( 'NONE', ( #61906 ), #212393, .F. ) ;
#84507=CARTESIAN_POINT ( 'NONE',  ( 6.047819040147648373, 9.213483425884394507, 1.199719254218452047 ) ) ;
#84519=CARTESIAN_POINT ( 'NONE',  ( 2.878073747850912412, 6.579779482459851003, -0.7998128361456362523 ) ) ;
#84532=CARTESIAN_POINT ( 'NONE',  ( -4.475600106286965918, 8.235634200727838916, 0.7216878364870338292 ) ) ;
#84534=CARTESIAN_POINT ( 'NONE',  ( 4.766573523656222555, 7.718696989977711809, 1.199719254218452047 ) ) ;
#84539=CARTESIAN_POINT ( 'NONE',  ( -4.034433228518296666, 6.864533312316751790, -1.199719254218450271 ) ) ;
#84547=AXIS2_PLACEMENT_3D ( 'NONE', #182979, #54057, #202403 ) ;
#84552=CARTESIAN_POINT ( 'NONE',  ( 3.777440027531570266, 7.356463756349603145, 0.3513329828547242517 ) ) ;
#84555=LINE ( 'NONE', #86689, #204728 ) ;
#84577=AXIS2_PLACEMENT_3D ( 'NONE', #176102, #61270, #194467 ) ;
#84583=CARTESIAN_POINT ( 'NONE',  ( 5.261973015879598314, 5.311592404713873172, -0.7216878364870458196 ) ) ;
#84588=CARTESIAN_POINT ( 'NONE',  ( 4.228163802615382494, 6.026220084508304708, -1.599625672291269396 ) ) ;
#84591=CARTESIAN_POINT ( 'NONE',  ( -4.285259070371116863, 7.157163461145040095, 1.199719254218452935 ) ) ;
#84594=CARTESIAN_POINT ( 'NONE',  ( -4.462041952228942954, 8.219816354326809460, -0.7216878364870338292 ) ) ;
#84600=CARTESIAN_POINT ( 'NONE',  ( -6.074935347375019390, 9.245119117649618801, 1.199719254218452047 ) ) ;
#84604=ORIENTED_EDGE ( 'NONE', *, *, #178698, .F. ) ;
#84605=CARTESIAN_POINT ( 'NONE',  ( 4.738043757352738083, 4.889522902105694513, -0.8057966945447234686 ) ) ;
#84607=CARTESIAN_POINT ( 'NONE',  ( -5.108390017298964914, 9.181815130149269422, 0.000000000000000000 ) ) ;
#84609=CARTESIAN_POINT ( 'NONE',  ( 4.684384365712907616, 8.380862967975740929, 0.5977175665230231028 ) ) ;
#84614=CARTESIAN_POINT ( 'NONE',  ( 6.318982112420993502, 9.529840343536603697, -1.199719254218452047 ) ) ;
#84620=CARTESIAN_POINT ( 'NONE',  ( -3.318713740295064163, 7.093859473644694269, 0.000000000000000000 ) ) ;
#84624=CARTESIAN_POINT ( 'NONE',  ( -4.586401103172829785, 8.572828063668767484, 0.7998128361456281477 ) ) ;
#84629=CARTESIAN_POINT ( 'NONE',  ( 7.987161891782087686, 8.490979426600148372, -0.7216878364870317197 ) ) ;
#84631=CARTESIAN_POINT ( 'NONE',  ( -5.750066545527201534, 9.722511713174800008, 0.000000000000000000 ) ) ;
#84637=CARTESIAN_POINT ( 'NONE',  ( 6.964048179274811012, 8.153752959689313684, 1.199719254218452047 ) ) ;
#84653=CARTESIAN_POINT ( 'NONE',  ( 5.561552386509557522, 7.525632394756676113, -1.337405013919689800 ) ) ;
#84667=EDGE_LOOP ( 'NONE', ( #152047, #127341 ) ) ;
#84684=CARTESIAN_POINT ( 'NONE',  ( -6.615421019548638704, 6.757903343899189785, 0.08170615477586136433 ) ) ;
#84687=ORIENTED_EDGE ( 'NONE', *, *, #209983, .T. ) ;
#84702=CARTESIAN_POINT ( 'NONE',  ( -4.294900800479008574, 8.232744377192641849, 0.000000000000000000 ) ) ;
#84704=CARTESIAN_POINT ( 'NONE',  ( -4.370663978927101567, 5.060324124126029943, -1.009771797811724214 ) ) ;
#84715=ORIENTED_EDGE ( 'NONE', *, *, #80739, .F. ) ;
#84716=CARTESIAN_POINT ( 'NONE',  ( 6.180537922983273091, 8.303989891604203422, -1.599625672291281386 ) ) ;
#84718=CARTESIAN_POINT ( 'NONE',  ( 7.146556367734776316, 7.510272981878305387, 0.7216878364870267237 ) ) ;
#84724=CARTESIAN_POINT ( 'NONE',  ( 4.828112100242276661, 6.726159765073026264, -1.443375672974068769 ) ) ;
#84732=CARTESIAN_POINT ( 'NONE',  ( -4.450819567036169211, 8.414649604842665553, -0.7998128361456362523 ) ) ;
#84733=VECTOR ( 'NONE', #164682, 1000.000000000000114 ) ;
#84734=CARTESIAN_POINT ( 'NONE',  ( 4.044074958626150185, 7.940114228364351767, 0.7998128361456271485 ) ) ;
#84743=CARTESIAN_POINT ( 'NONE',  ( -5.915100157312088491, 10.12297696016459092, -0.7998128361456362523 ) ) ;
#84744=CARTESIAN_POINT ( 'NONE',  ( 5.110497557708379546, 4.926945003606695295, -0.7998128361456481317 ) ) ;
#84753=CARTESIAN_POINT ( 'NONE',  ( 4.701645408888975197, 8.707279753670952971, 0.000000000000000000 ) ) ;
#84758=CARTESIAN_POINT ( 'NONE',  ( -4.745581203565001793, 8.305819929356548670, 0.7838639097331673300 ) ) ;
#84769=CARTESIAN_POINT ( 'NONE',  ( -4.950135482320939140, 4.947781948895412008, -0.7216878364870338292 ) ) ;
#84770=AXIS2_PLACEMENT_3D ( 'NONE', #74632, #140739, #158031 ) ;
#84778=CARTESIAN_POINT ( 'NONE',  ( 4.014622883422321209, 5.777089012116397804, -1.443375672974068769 ) ) ;
#84784=EDGE_CURVE ( 'NONE', #70814, #10691, #129129, .T. ) ;
#84798=CARTESIAN_POINT ( 'NONE',  ( 6.398522151006641678, 6.429640362454684954, 0.000000000000000000 ) ) ;
#84817=CARTESIAN_POINT ( 'NONE',  ( 0.2848239700905849103, 3.301821615535860399, 1.981129458308562352 ) ) ;
#84820=CARTESIAN_POINT ( 'NONE',  ( 5.554000203453580475, 6.508696987897830688, -1.199719254218452047 ) ) ;
#84821=CARTESIAN_POINT ( 'NONE',  ( -5.831415467653581430, 5.975941931783510519, 0.7216878364870257245 ) ) ;
#84840=( BOUNDED_CURVE ( )  B_SPLINE_CURVE ( 2, ( #79492, #80561, #29690 ),
 .UNSPECIFIED., .F., .T. ) 
 B_SPLINE_CURVE_WITH_KNOTS ( ( 3, 3 ),
 ( 0.000000000000000000, 0.0008788941494526597391 ),
 .UNSPECIFIED. ) 
 CURVE ( )  GEOMETRIC_REPRESENTATION_ITEM ( )  RATIONAL_B_SPLINE_CURVE ( ( 1.000000000000000000, 0.9858700613453033057, 0.9747206155903836988 ) ) 
 REPRESENTATION_ITEM ( '' )  );
#84846=CARTESIAN_POINT ( 'NONE',  ( -5.284646014276622950, 9.387447126623207794, -0.7998128361456362523 ) ) ;
#84852=FACE_OUTER_BOUND ( 'NONE', #105406, .T. ) ;
#84860=CARTESIAN_POINT ( 'NONE',  ( -7.937372586157736443, 8.224965870130965584, 0.7998128361456341429 ) ) ;
#84871=CARTESIAN_POINT ( 'NONE',  ( -4.599959256786493533, 8.588645909551377855, 0.000000000000000000 ) ) ;
#84874=CARTESIAN_POINT ( 'NONE',  ( -5.804299160426229953, 8.825413882922319431, -1.082531754730549967 ) ) ;
#84879=CARTESIAN_POINT ( 'NONE',  ( 5.207740400980577888, 5.248321020665011716, 0.000000000000000000 ) ) ;
#84881=CARTESIAN_POINT ( 'NONE',  ( -7.095713291905736853, 9.371694488680407886, 1.599625672291269396 ) ) ;
#84894=CARTESIAN_POINT ( 'NONE',  ( -0.3866901564497973731, 3.102326550341738098, 2.027579305719746205 ) ) ;
#84900=CARTESIAN_POINT ( 'NONE',  ( 6.493754380866193721, 6.839952184459461293, 0.5864284347954504817 ) ) ;
#84918=CARTESIAN_POINT ( 'NONE',  ( 6.477827756726281194, 6.756902019748111776, -0.2091553196570776485 ) ) ;
#84937=CARTESIAN_POINT ( 'NONE',  ( -6.818824913030298696, 6.919993584815607335, 0.7998128361456341429 ) ) ;
#84950=CARTESIAN_POINT ( 'NONE',  ( 4.850785098639300408, 8.881276058379668825, -0.7998128361456481317 ) ) ;
#84958=CARTESIAN_POINT ( 'NONE',  ( -5.275531169048895741, 9.168887107283438809, -0.7216878364870338292 ) ) ;
#84964=CARTESIAN_POINT ( 'NONE',  ( 6.444921918449731280, 8.612437886315108315, 1.599625672291268286 ) ) ;
#84973=B_SPLINE_CURVE_WITH_KNOTS ( 'NONE', 3,
 ( #106643, #21038, #120785, #87136, #170515, #186762, #119704, #39453, #89292, #22097, #152147, #88210, #3715, #155343 ),
 .UNSPECIFIED., .F., .F.,
 ( 4, 2, 2, 2, 2, 2, 4 ),
 ( 0.5000128224787536713, 0.5890577402443318844, 0.6781026580099100975, 0.7226251168926991486, 0.7671475757754881997, 0.8116700346582772507, 0.8561924935410664128 ),
 .UNSPECIFIED. ) ;
#84977=CARTESIAN_POINT ( 'NONE',  ( -6.455090533882206216, 7.663932056684933158, -1.082531754730549967 ) ) ;
#84978=CARTESIAN_POINT ( 'NONE',  ( 5.885648082108190238, 7.959951743916638733, 1.443375672974065660 ) ) ;
#84984=LINE ( 'NONE', #53555, #11206 ) ;
#84987=EDGE_LOOP ( 'NONE', ( #116136, #203685 ) ) ;
#84988=CARTESIAN_POINT ( 'NONE',  ( -3.688700311369816909, 6.461178242310183784, -1.199719254218450271 ) ) ;
#84989=CARTESIAN_POINT ( 'NONE',  ( -7.932929277771797238, 8.427708043588125975, 0.000000000000000000 ) ) ;
#84992=CARTESIAN_POINT ( 'NONE',  ( 4.380693030546905398, 8.124909279031149012, 0.7216878364870247253 ) ) ;
#85005=CARTESIAN_POINT ( 'NONE',  ( -5.000347810418038996, 7.933946187056884369, 1.064693650161437022 ) ) ;
#85009=CARTESIAN_POINT ( 'NONE',  ( -0.08174084574804243997, 3.472891232463431788, -1.998431917447621498 ) ) ;
#85014=CARTESIAN_POINT ( 'NONE',  ( -5.981082042284069367, 7.006959133200059142, 1.199719254218452935 ) ) ;
#85027=CARTESIAN_POINT ( 'NONE',  ( 3.770049233051776749, 6.556085317605844232, 1.199719254218451159 ) ) ;
#85054=ORIENTED_EDGE ( 'NONE', *, *, #50115, .T. ) ;
#85064=CARTESIAN_POINT ( 'NONE',  ( 6.373741612200174878, 6.608655767087927124, 0.7216878364870328300 ) ) ;
#85070=CARTESIAN_POINT ( 'NONE',  ( 5.302647476276220573, 8.240153584747313076, -1.082531754730548412 ) ) ;
#85071=CARTESIAN_POINT ( 'NONE',  ( -3.914023514147247251, 8.998170835453741745, 0.7749999999999996891 ) ) ;
#85084=CARTESIAN_POINT ( 'NONE',  ( -7.795011973214244883, 8.058878488363559356, 0.7998128361456341429 ) ) ;
#85095=CARTESIAN_POINT ( 'NONE',  ( 4.163762572728282763, 6.911454530608037494, -1.082531754730548412 ) ) ;
#85100=CARTESIAN_POINT ( 'NONE',  ( -5.427006627220116286, 9.553534508390610469, -0.7998128361456362523 ) ) ;
#85105=CARTESIAN_POINT ( 'NONE',  ( -6.509323148336870091, 7.727203440215372865, 1.082531754730549078 ) ) ;
#85108=CARTESIAN_POINT ( 'NONE',  ( -5.237192476628793614, 9.332084666034067055, 0.7998128361456291469 ) ) ;
#85129=CARTESIAN_POINT ( 'NONE',  ( -4.556949027968976829, 5.449433633119473264, 1.082531754730549078 ) ) ;
#85131=CARTESIAN_POINT ( 'NONE',  ( -5.939880696118548187, 6.102484698325975288, 0.000000000000000000 ) ) ;
#85133=CARTESIAN_POINT ( 'NONE',  ( 4.227110032410640095, 8.153655147779589996, 0.7998128361456271485 ) ) ;
#85134=CARTESIAN_POINT ( 'NONE',  ( -3.871735385154307263, 6.674719161725423788, -1.199719254218450271 ) ) ;
#85135=CARTESIAN_POINT ( 'NONE',  ( -7.117104292530948229, 7.267986194233038155, -0.7998128361456362523 ) ) ;
#85173=CARTESIAN_POINT ( 'NONE',  ( 3.553238514845298734, 7.337208092372121904, -0.2327671511505452484 ) ) ;
#85189=CARTESIAN_POINT ( 'NONE',  ( 3.250922972226694352, 7.014770244231638863, 0.7998128361456281477 ) ) ;
#85191=CARTESIAN_POINT ( 'NONE',  ( 5.361443639997856891, 4.701392137926264425, -2.440314829665658714 ) ) ;
#85200=B_SPLINE_CURVE_WITH_KNOTS ( 'NONE', 3,
 ( #196757, #100313, #65652, #129713, #81931, #148017, #194616, #79799, #17972, #195698, #131799, #180506, #163203 ),
 .UNSPECIFIED., .F., .F.,
 ( 4, 3, 3, 3, 4 ),
 ( 1.953129352420981408E-17, 6.251590020777592386E-05, 0.0001877400439070772351, 0.0002924247082610473628, 0.0003977189496704516282 ),
 .UNSPECIFIED. ) ;
#85203=CARTESIAN_POINT ( 'NONE',  ( 4.684024595049480766, 8.263433789595206136, 0.5754648794667740486 ) ) ;
#85206=CARTESIAN_POINT ( 'NONE',  ( 4.903208829997618423, 5.749440385532527564, -1.199719254218450271 ) ) ;
#85209=VERTEX_POINT ( 'NONE', #148491 ) ;
#85210=CARTESIAN_POINT ( 'NONE',  ( -4.261005416444848315, 8.193199762486115034, 0.7998128361456352531 ) ) ;
#85215=B_SPLINE_CURVE_WITH_KNOTS ( 'NONE', 3,
 ( #54191, #26749, #141619, #59246, #140550, #45166, #125404, #191369, #177283, #158896 ),
 .UNSPECIFIED., .F., .F.,
 ( 4, 3, 3, 4 ),
 ( 2.717543607569314096E-17, 3.125160614615090737E-05, 6.250328995029551141E-05, 0.0001021784628617198687 ),
 .UNSPECIFIED. ) ;
#85222=CARTESIAN_POINT ( 'NONE',  ( 6.888951449519509218, 7.209733910627123876, -0.7216878364870317197 ) ) ;
#85225=CARTESIAN_POINT ( 'NONE',  ( -4.938913097128142304, 8.984092056616635347, -0.7998128361456362523 ) ) ;
#85237=CARTESIAN_POINT ( 'NONE',  ( 3.770049233051776749, 6.556085317605844232, 1.199719254218451159 ) ) ;
#85238=CARTESIAN_POINT ( 'NONE',  ( 6.547661840756936691, 6.603636667163397256, 0.7998128361456352531 ) ) ;
#85239=ORIENTED_EDGE ( 'NONE', *, *, #193710, .F. ) ;
#85245=DIRECTION ( 'NONE',  ( 0.000000000000000000, 0.000000000000000000, -1.000000000000000000 ) ) ;
#85274=CARTESIAN_POINT ( 'NONE',  ( 5.668190738965027897, 8.770583741171307679, -1.199719254218452047 ) ) ;
#85280=CARTESIAN_POINT ( 'NONE',  ( 4.529832720741620022, 7.338536369956936589, -1.082531754730548412 ) ) ;
#85283=CARTESIAN_POINT ( 'NONE',  ( 2.905190055078214595, 6.611415174225076186, 0.7998128361456271485 ) ) ;
#85295=CARTESIAN_POINT ( 'NONE',  ( 6.321627859881460587, 6.858947107989728842, -0.6823232096292205506 ) ) ;
#85296=CARTESIAN_POINT ( 'NONE',  ( -7.268579750702168774, 7.652633595340216921, -0.7216878364870338292 ) ) ;
#85316=EDGE_CURVE ( 'NONE', #149695, #179985, #114447, .T. ) ;
#85332=CARTESIAN_POINT ( 'NONE',  ( 7.015418140428412386, 7.149352350113456822, 0.7998128361456331437 ) ) ;
#85335=CARTESIAN_POINT ( 'NONE',  ( 6.713222337422018349, 7.861122810861019161, -1.199719254218452047 ) ) ;
#85349=CARTESIAN_POINT ( 'NONE',  ( -5.581116510680924847, 6.540332679663050541, -1.199719254218453823 ) ) ;
#85351=CARTESIAN_POINT ( 'NONE',  ( 6.333067150914808430, 8.481940657524365434, 1.443375672974063439 ) ) ;
#85360=CARTESIAN_POINT ( 'NONE',  ( -2.810282979782591006, 6.500690253046801814, 0.000000000000000000 ) ) ;
#85367=CARTESIAN_POINT ( 'NONE',  ( -5.750066545971566079, 8.762142499391876171, 1.082531754730550855 ) ) ;
#85369=CARTESIAN_POINT ( 'NONE',  ( -4.990809943606269172, 8.836712344267034780, -0.7216878364870338292 ) ) ;
#85391=CARTESIAN_POINT ( 'NONE',  ( -5.991777542596674166, 5.955104985976372944, 0.000000000000000000 ) ) ;
#85400=CARTESIAN_POINT ( 'NONE',  ( 2.744865908132018362, 2.962146155648302415, -2.500000000000000888 ) ) ;
#85401=CARTESIAN_POINT ( 'NONE',  ( -5.577377183731011101, 7.510248947172004641, -1.348340355397449342 ) ) ;
#85419=CARTESIAN_POINT ( 'NONE',  ( 6.038177310039780643, 8.137902509836795417, -1.599625672291283607 ) ) ;
#85426=CARTESIAN_POINT ( 'NONE',  ( 1.843739406749228538, 8.920000000000001705, -0.7749999999999996891 ) ) ;
#85436=CARTESIAN_POINT ( 'NONE',  ( 3.867349521082877217, 7.341814853893565918, 0.5856213828667733434 ) ) ;
#85441=CARTESIAN_POINT ( 'NONE',  ( 5.006703865196457492, 9.063181286029688977, 0.000000000000000000 ) ) ;
#85442=CARTESIAN_POINT ( 'NONE',  ( 6.574778147984297938, 6.635272358928617997, -0.7998128361456481317 ) ) ;
#85444=CARTESIAN_POINT ( 'NONE',  ( 5.713835393516482952, 5.630839145382857680, 0.7998128361456352531 ) ) ;
#85448=FACE_OUTER_BOUND ( 'NONE', #134192, .T. ) ;
#85457=CARTESIAN_POINT ( 'NONE',  ( 4.915098833515745724, 8.004322973991836676, -0.9888141558981374812 ) ) ;
#85459=CARTESIAN_POINT ( 'NONE',  ( -6.631346530415505036, 7.869564052640446228, 1.082531754730549078 ) ) ;
#85460=CARTESIAN_POINT ( 'NONE',  ( 3.282482588284323821, 6.843663763058119187, 0.7216878364870257245 ) ) ;
#85481=CARTESIAN_POINT ( 'NONE',  ( -4.245111494410291897, 7.006361605903701495, 1.082531754730549967 ) ) ;
#85486=CARTESIAN_POINT ( 'NONE',  ( 7.191674137406095291, 7.354984346587396082, 0.000000000000000000 ) ) ;
#85513=CARTESIAN_POINT ( 'NONE',  ( 6.801350335910821165, 7.963938809097990124, 1.199719254218452047 ) ) ;
#85517=CARTESIAN_POINT ( 'NONE',  ( 5.040599249230596435, 9.102725900736217568, 0.7998128361456341429 ) ) ;
#85542=CARTESIAN_POINT ( 'NONE',  ( 3.431622278034673901, 7.017660067766835930, -1.734723475976807094E-15 ) ) ;
#85547=CARTESIAN_POINT ( 'NONE',  ( -5.257529707049291900, 9.355811434857983500, 0.7998128361456291469 ) ) ;
#85549=CARTESIAN_POINT ( 'NONE',  ( 6.068156270568149324, 9.237210194708310951, 1.199719254218452047 ) ) ;
#85552=CARTESIAN_POINT ( 'NONE',  ( -3.851925040058345573, 5.587274861525073355, -1.443375672974078761 ) ) ;
#85557=CARTESIAN_POINT ( 'NONE',  ( 2.449293598294706414E-16, 8.920000000000001705, 2.000000000000000000 ) ) ;
#85571=CARTESIAN_POINT ( 'NONE',  ( 5.657495238652423097, 9.822437888394988548, 0.000000000000000000 ) ) ;
#85581=CARTESIAN_POINT ( 'NONE',  ( 3.444653546323793947, 6.176457016423196222, 1.199719254218451159 ) ) ;
#85595=CARTESIAN_POINT ( 'NONE',  ( -6.631346530859867805, 6.909194838857525944, 0.000000000000000000 ) ) ;
#85598=CARTESIAN_POINT ( 'NONE',  ( 7.038618024149998043, 8.240751112043669835, -1.199719254218452047 ) ) ;
#85604=CARTESIAN_POINT ( 'NONE',  ( -8.086512275908061653, 8.398962174839683215, 0.000000000000000000 ) ) ;
#85621=DIRECTION ( 'NONE',  ( 0.000000000000000000, 1.000000000000000000, 0.000000000000000000 ) ) ;
#85653=CARTESIAN_POINT ( 'NONE',  ( -3.623772196602547346, 7.449761006003425834, 0.000000000000000000 ) ) ;
#85654=CARTESIAN_POINT ( 'NONE',  ( -5.492988512192097161, 6.437516681426083132, 1.199719254218452935 ) ) ;
#85657=CARTESIAN_POINT ( 'NONE',  ( -4.597623488365601752, 8.377994813152914944, 0.7216878364870267237 ) ) ;
#85660=CARTESIAN_POINT ( 'NONE',  ( 2.970157261343746136, 6.585292010301047938, 0.4235207732182846851 ) ) ;
#85664=CARTESIAN_POINT ( 'NONE',  ( -6.343235766347277149, 8.493804042195527870, -1.599625672291271394 ) ) ;
#85668=VERTEX_POINT ( 'NONE', #123840 ) ;
#85672=CARTESIAN_POINT ( 'NONE',  ( -5.444481204339554736, 8.509589284108232121, 1.199719254218454489 ) ) ;
#85674=CARTESIAN_POINT ( 'NONE',  ( 4.607021725950278146, 8.475092030744066918, 0.2235605714990263060 ) ) ;
#85679=CARTESIAN_POINT ( 'NONE',  ( 5.657495238652423097, 9.822437888394988548, 0.000000000000000000 ) ) ;
#85691=CARTESIAN_POINT ( 'NONE',  ( 4.913904330310220558, 4.697586238308844919, 0.000000000000000000 ) ) ;
#85694=CARTESIAN_POINT ( 'NONE',  ( -6.224601922005509991, 10.27613631906616476, 0.7216878364870267237 ) ) ;
#85700=CARTESIAN_POINT ( 'NONE',  ( 5.559725510055676168, 8.644040974110419384, 1.199719254218451159 ) ) ;
#85716=CARTESIAN_POINT ( 'NONE',  ( 5.943507298343291723, 7.226397084328657350, -1.228854570503196575 ) ) ;
#85720=AXIS2_PLACEMENT_3D ( 'NONE', #132225, #177751, #48817 ) ;
#85724=B_SPLINE_CURVE_WITH_KNOTS ( 'NONE', 3,
 ( #76545, #75490, #123275, #191351 ),
 .UNSPECIFIED., .F., .F.,
 ( 4, 4 ),
 ( 0.000000000000000000, 0.0005559729156925552647 ),
 .UNSPECIFIED. ) ;
#85750=CARTESIAN_POINT ( 'NONE',  ( -6.374142478797011790, 6.840173217398676897, -0.5947513654121737714 ) ) ;
#85768=CARTESIAN_POINT ( 'NONE',  ( -5.061990249855848667, 6.999017606288844284, -1.599625672291271394 ) ) ;
#85779=VERTEX_POINT ( 'NONE', #191918 ) ;
#85785=CARTESIAN_POINT ( 'NONE',  ( 5.006703865196457492, 9.063181286029688977, 0.000000000000000000 ) ) ;
#85786=CARTESIAN_POINT ( 'NONE',  ( -5.436182321379713578, 6.108390213082993903, 1.083092214668917919 ) ) ;
#85788=CARTESIAN_POINT ( 'NONE',  ( 6.495764994278795612, 9.632124022417032805, 1.082531754730549078 ) ) ;
#85798=CARTESIAN_POINT ( 'NONE',  ( 4.367134876933267407, 8.109091433148536865, 0.000000000000000000 ) ) ;
#85802=CARTESIAN_POINT ( 'NONE',  ( -6.720001414228860881, 7.869031733802326123, -1.199719254218452047 ) ) ;
#85803=CARTESIAN_POINT ( 'NONE',  ( 4.908934136599710563, 7.884784371745123366, 1.199719254218451159 ) ) ;
#85812=CARTESIAN_POINT ( 'NONE',  ( -3.654804927335652209, 6.421633627603656080, 1.199719254218452935 ) ) ;
#85813=CARTESIAN_POINT ( 'NONE',  ( 6.210516883511641772, 9.403297576475722508, 1.199719254218452047 ) ) ;
#85815=DIRECTION ( 'NONE',  ( 0.000000000000000000, 1.000000000000000000, 0.000000000000000000 ) ) ;
#85820=CARTESIAN_POINT ( 'NONE',  ( 7.523848900940885542, 7.742521570711348389, 0.7998128361456291469 ) ) ;
#85824=FACE_OUTER_BOUND ( 'NONE', #21693, .T. ) ;
#85826=CARTESIAN_POINT ( 'NONE',  ( -5.672142842012183550, 7.433492730264275927, 1.337035701138490351 ) ) ;
#85837=CARTESIAN_POINT ( 'NONE',  ( -7.553827861469316396, 8.841829255582865699, -1.199719254218452047 ) ) ;
#85847=CARTESIAN_POINT ( 'NONE',  ( 3.933273961740296087, 6.642551151122080277, 1.082531754730549078 ) ) ;
#85851=CARTESIAN_POINT ( 'NONE',  ( -4.586401103172829785, 8.572828063668767484, 0.7998128361456281477 ) ) ;
#85855=EDGE_CURVE ( 'NONE', #15686, #141689, #78304, .T. ) ;
#85868=CARTESIAN_POINT ( 'NONE',  ( 6.059568310664962709, 6.034194215389424798, 0.7998128361456350310 ) ) ;
#85891=CARTESIAN_POINT ( 'NONE',  ( 5.123001941117305336, 7.070197912760590064, 1.599625672291268286 ) ) ;
#85894=CARTESIAN_POINT ( 'NONE',  ( -5.994113311017573054, 6.165756082374834079, 0.7216878364870257245 ) ) ;
#85918=CARTESIAN_POINT ( 'NONE',  ( -7.632314129850253259, 7.869064337772231355, 0.7998128361456341429 ) ) ;
#85920=CARTESIAN_POINT ( 'NONE',  ( 6.170369307550816806, 9.252495721234380355, 1.082531754730549967 ) ) ;
#85934=CARTESIAN_POINT ( 'NONE',  ( -6.129167961829681488, 9.308390501180058507, -1.199719254218452047 ) ) ;
#85941=CARTESIAN_POINT ( 'NONE',  ( 5.388439706788500594, 5.251210844200210559, 0.7998128361456352531 ) ) ;
#85946=CARTESIAN_POINT ( 'NONE',  ( -6.720001414228860881, 7.869031733802326123, -1.199719254218452047 ) ) ;
#85949=CARTESIAN_POINT ( 'NONE',  ( -5.289089323106922258, 9.184704953684462936, 0.7216878364870267237 ) ) ;
#85953=CARTESIAN_POINT ( 'NONE',  ( 3.567203813726949058, 7.175838526074521440, 0.7216878364870257245 ) ) ;
#85954=CARTESIAN_POINT ( 'NONE',  ( -3.634994581795317536, 7.254927755487573293, 0.000000000000000000 ) ) ;
#85966=CARTESIAN_POINT ( 'NONE',  ( 0.4461838333975313153, 2.877219473291478646, 1.949594826320503849 ) ) ;
#85970=CARTESIAN_POINT ( 'NONE',  ( 1.886825320689233809, 2.480000000000016858, 2.459652456995882641 ) ) ;
#85971=CARTESIAN_POINT ( 'NONE',  ( 6.454497976780569246, 6.866128686250288382, -0.6735470152485992790 ) ) ;
#85992=CARTESIAN_POINT ( 'NONE',  ( 6.469672735924913987, 6.762149564967588233, 0.2594904213018677797 ) ) ;
#86010=CARTESIAN_POINT ( 'NONE',  ( -6.493429226302317225, 6.540365283632955773, 0.7998128361456341429 ) ) ;
#86022=CARTESIAN_POINT ( 'NONE',  ( 5.363132282657546490, 8.414682208812571673, -1.199719254218452047 ) ) ;
#86029=CARTESIAN_POINT ( 'NONE',  ( -7.065207446052813367, 8.375735120883982532, -1.082531754730549967 ) ) ;
#86033=CARTESIAN_POINT ( 'NONE',  ( 3.973948422136968084, 5.729635473950147606, -1.443375672974068769 ) ) ;
#86047=CARTESIAN_POINT ( 'NONE',  ( -5.804299160426229953, 8.825413882922319431, -1.082531754730549967 ) ) ;
#86048=CARTESIAN_POINT ( 'NONE',  ( 6.861835142292147083, 7.178098218861903135, 0.7216878364870328300 ) ) ;
#86059=CARTESIAN_POINT ( 'NONE',  ( -4.228163802615396705, 6.026220084508304708, -1.599625672291271394 ) ) ;
#86060=CARTESIAN_POINT ( 'NONE',  ( -6.102578539926875933, 10.13377570664109051, 0.7216878364870267237 ) ) ;
#86062=CARTESIAN_POINT ( 'NONE',  ( 5.356880090730857802, 8.303424968277756335, 1.082531754730548412 ) ) ;
#86075=CARTESIAN_POINT ( 'NONE',  ( -4.839221724899702259, 8.104102677821947154, -0.8803655321611182361 ) ) ;
#86080=CARTESIAN_POINT ( 'NONE',  ( 3.106226591306694651, 6.638031766584184368, 0.000000000000000000 ) ) ;
#86083=CARTESIAN_POINT ( 'NONE',  ( -5.119085517611572378, 8.129960982925583224, 1.199719254218452935 ) ) ;
#86084=CIRCLE ( 'NONE', #200322, 0.08000000000000020983 ) ;
#86097=CARTESIAN_POINT ( 'NONE',  ( 4.553559489343365740, 6.405848385690952718, -1.599625672291269396 ) ) ;
#86136=CARTESIAN_POINT ( 'NONE',  ( 5.397554552016212703, 8.350878506444006533, 1.082531754730547524 ) ) ;
#86140=CARTESIAN_POINT ( 'NONE',  ( 4.370663978927065152, 5.060324124126029943, 1.009771797811723326 ) ) ;
#86141=CARTESIAN_POINT ( 'NONE',  ( 4.529832720297257254, 8.298905583739861314, 0.000000000000000000 ) ) ;
#86155=CARTESIAN_POINT ( 'NONE',  ( -7.095713291905736853, 9.371694488680407886, 1.599625672291269396 ) ) ;
#86167=CARTESIAN_POINT ( 'NONE',  ( 5.248414861821569133, 6.256143772614186638, -1.082531754730548412 ) ) ;
#86173=CARTESIAN_POINT ( 'NONE',  ( -5.912237504011027767, 9.055304967058290799, 1.199719254218454489 ) ) ;
#86178=CARTESIAN_POINT ( 'NONE',  ( -7.783789588021474692, 8.253711738879413673, 0.7216878364870317197 ) ) ;
#86180=AXIS2_PLACEMENT_3D ( 'NONE', #46728, #62946, #61893 ) ;
#86182=CARTESIAN_POINT ( 'NONE',  ( -7.910256278930404505, 8.193330178365746619, -0.7998128361456362523 ) ) ;
#86201=CARTESIAN_POINT ( 'NONE',  ( -3.919715807682309094, 6.626733304721049933, 1.082531754730549967 ) ) ;
#86203=CARTESIAN_POINT ( 'NONE',  ( 5.248941747146098180, 6.152795455539095570, -1.199719254218452047 ) ) ;
#86204=CARTESIAN_POINT ( 'NONE',  ( -5.978219388983010418, 5.939287140093762574, -0.7998128361456362523 ) ) ;
#86205=CARTESIAN_POINT ( 'NONE',  ( -5.986807348886189040, 9.142303119412650503, -1.199719254218452047 ) ) ;
#86231=CARTESIAN_POINT ( 'NONE',  ( -7.553827861469316396, 8.841829255582865699, -1.199719254218452047 ) ) ;
#86260=CARTESIAN_POINT ( 'NONE',  ( 3.074666975249065626, 6.809138247757705820, 0.000000000000000000 ) ) ;
#86277=CARTESIAN_POINT ( 'NONE',  ( 4.203910148689107729, 7.062256385849379647, -1.199719254218448494 ) ) ;
#86284=CARTESIAN_POINT ( 'NONE',  ( -7.761116589180078407, 8.019333873657032541, 0.000000000000000000 ) ) ;
#86299=CARTESIAN_POINT ( 'NONE',  ( 5.939880696562888751, 7.062853913145737295, -1.082531754730548412 ) ) ;
#86302=CARTESIAN_POINT ( 'NONE',  ( -5.367048706163331850, 7.354919138647580290, -1.599625672291271394 ) ) ;
#86307=ORIENTED_EDGE ( 'NONE', *, *, #164010, .T. ) ;
#86311=CARTESIAN_POINT ( 'NONE',  ( 3.542423274920540432, 7.354853930707762721, -1.734723475976807094E-15 ) ) ;
#86312=CARTESIAN_POINT ( 'NONE',  ( 6.333594036239346359, 7.418223126147930557, 1.199719254218453823 ) ) ;
#86333=FACE_OUTER_BOUND ( 'NONE', #194049, .T. ) ;
#86341=CARTESIAN_POINT ( 'NONE',  ( 5.032011289327418702, 5.899709921417326974, 1.199719254218452935 ) ) ;
#86347=CARTESIAN_POINT ( 'NONE',  ( 6.879836604291781121, 6.991173891287354003, -0.7998128361456341429 ) ) ;
#86348=DIRECTION ( 'NONE',  ( 1.000000000000000000, -0.000000000000000000, -0.000000000000000000 ) ) ;
#86352=CARTESIAN_POINT ( 'NONE',  ( 5.234856708652227297, 7.200695141551334721, 1.443375672974065660 ) ) ;
#86355=CARTESIAN_POINT ( 'NONE',  ( 5.858531774880875176, 9.849054480754103835, -0.7216878364870458196 ) ) ;
#86356=VERTEX_POINT ( 'NONE', #180760 ) ;
#86364=CARTESIAN_POINT ( 'NONE',  ( 4.582993027900885252, 6.853944465854098667, -1.265546273303337133 ) ) ;
#86368=CARTESIAN_POINT ( 'NONE',  ( 6.457572779797339457, 6.769951385671206801, 0.3193968722623799494 ) ) ;
#86369=EDGE_CURVE ( 'NONE', #40348, #123271, #214128, .T. ) ;
#86370=CARTESIAN_POINT ( 'NONE',  ( -2.823841133396259639, 6.516508098929413961, -0.7998128361456481317 ) ) ;
#86405=CARTESIAN_POINT ( 'NONE',  ( 6.343235766347262938, 8.493804042195527870, -1.599625672291281386 ) ) ;
#86407=CARTESIAN_POINT ( 'NONE',  ( 6.821687566331318564, 7.987665577921906568, 1.199719254218452935 ) ) ;
#86420=CARTESIAN_POINT ( 'NONE',  ( -5.808742468812186033, 5.741564066561132940, 0.000000000000000000 ) ) ;
#86423=CARTESIAN_POINT ( 'NONE',  ( 5.844973620822835336, 7.912498205750389424, 1.443375672974064550 ) ) ;
#86432=CARTESIAN_POINT ( 'NONE',  ( -4.995253251992230581, 4.792493313604505367, 0.000000000000000000 ) ) ;
#86438=CARTESIAN_POINT ( 'NONE',  ( -5.966997003790217136, 9.975597247814986801, -0.7216878364870338292 ) ) ;
#86439=EDGE_LOOP ( 'NONE', ( #174598, #115994, #136300, #103385 ) ) ;
#86440=CARTESIAN_POINT ( 'NONE',  ( -5.424670859243583720, 8.382514198209223721, 1.082531754730550855 ) ) ;
#86448=CARTESIAN_POINT ( 'NONE',  ( -0.1437412632283050218, 3.385453691495572404, 2.075078668430507367 ) ) ;
#86464=CARTESIAN_POINT ( 'NONE',  ( -5.119085517611572378, 8.129960982925583224, 1.199719254218452935 ) ) ;
#86466=CARTESIAN_POINT ( 'NONE',  ( -5.354544322754380303, 5.211666229493680191, 0.7998128361456281477 ) ) ;
#86474=CARTESIAN_POINT ( 'NONE',  ( -5.233950224509621663, 7.808013953112580730, -1.290304472045332496 ) ) ;
#86488=CARTESIAN_POINT ( 'NONE',  ( 6.178787966740411086, 5.309377612921773348, 2.438151698554704261 ) ) ;
#86494=ADVANCED_FACE ( 'NONE', ( #199116 ), #3048, .F. ) ;
#86496=CARTESIAN_POINT ( 'NONE',  ( 1.930226670627054109, 8.999999999999998224, -0.7749999999999996891 ) ) ;
#86504=CARTESIAN_POINT ( 'NONE',  ( 5.357406976055401948, 6.279338222599979424, 1.199719254218452935 ) ) ;
#86512=CARTESIAN_POINT ( 'NONE',  ( 6.547661840756936691, 6.603636667163397256, 0.7998128361456352531 ) ) ;
#86514=CARTESIAN_POINT ( 'NONE',  ( 3.881377115262159894, 7.750300077773022878, 0.7998128361456271485 ) ) ;
#86518=CARTESIAN_POINT ( 'NONE',  ( -7.013428937081431336, 5.939655416065873439, -2.436399677959149024 ) ) ;
#86527=CARTESIAN_POINT ( 'NONE',  ( 5.441225816562971218, 7.512442699629209741, -1.249814574298679926 ) ) ;
#86529=CARTESIAN_POINT ( 'NONE',  ( -6.604230223188181093, 6.877559146573883453, 0.7216878364870317197 ) ) ;
#86530=CARTESIAN_POINT ( 'NONE',  ( 6.048345925472191631, 7.189396680206621149, 1.082531754730549967 ) ) ;
#86545=AXIS2_PLACEMENT_3D ( 'NONE', #179962, #31586, #97660 ) ;
#86551=CARTESIAN_POINT ( 'NONE',  ( -4.123088111887291518, 7.824370207261548416, 0.000000000000000000 ) ) ;
#86556=CARTESIAN_POINT ( 'NONE',  ( 5.611095471209277541, 7.639640364534566075, 1.599625672291268286 ) ) ;
#86576=CARTESIAN_POINT ( 'NONE',  ( -5.317937133690677776, 6.974616996837226246, -1.245902666257096669 ) ) ;
#86584=CARTESIAN_POINT ( 'NONE',  ( 7.367930134383754215, 7.560616343061329125, -0.7998128361456341429 ) ) ;
#86596=CARTESIAN_POINT ( 'NONE',  ( -2.996969800987126842, 6.406095355250562839, -0.7225173797624391270 ) ) ;
#86610=CARTESIAN_POINT ( 'NONE',  ( 0.4917504562595223505, 10.46609003534429760, -2.500000000000000444 ) ) ;
#86613=CARTESIAN_POINT ( 'NONE',  ( 3.933273961740296087, 6.642551151122080277, 1.082531754730549078 ) ) ;
#86618=CARTESIAN_POINT ( 'NONE',  ( -6.071018923869249129, 10.30488218781460574, 0.7998128361456291469 ) ) ;
#86620=CARTESIAN_POINT ( 'NONE',  ( 5.905458427204159477, 9.047396044116986502, 1.199719254218452047 ) ) ;
#86622=LINE ( 'NONE', #53051, #192309 ) ;
#86624=ADVANCED_FACE ( 'NONE', ( #136296 ), #108749, .T. ) ;
#86625=CARTESIAN_POINT ( 'NONE',  ( -3.526529353330355221, 6.168015774643768268, -1.082531754730546636 ) ) ;
#86629=DIRECTION ( 'NONE',  ( -0.000000000000000000, -0.000000000000000000, 1.000000000000000000 ) ) ;
#86643=CARTESIAN_POINT ( 'NONE',  ( 7.614839552730775729, 8.913009562054615031, 1.199719254218452047 ) ) ;
#86652=CARTESIAN_POINT ( 'NONE',  ( 6.034787771858531435, 10.05468647722803865, 0.000000000000000000 ) ) ;
#86656=ORIENTED_EDGE ( 'NONE', *, *, #187873, .T. ) ;
#86665=CARTESIAN_POINT ( 'NONE',  ( -4.963693636378939011, 8.805076652501815815, 0.7216878364870267237 ) ) ;
#86668=CARTESIAN_POINT ( 'NONE',  ( 5.826972158823246595, 10.02016096192762085, -0.7998128361456481317 ) ) ;
#86674=CARTESIAN_POINT ( 'NONE',  ( -4.516801452008150086, 5.298631777878131111, 1.199719254218452935 ) ) ;
#86689=CARTESIAN_POINT ( 'NONE',  ( -8.014278199453791274, 8.522615118883788199, 1.530808498934192557E-16 ) ) ;
#86703=ORIENTED_EDGE ( 'NONE', *, *, #114761, .T. ) ;
#86714=CARTESIAN_POINT ( 'NONE',  ( 5.234856708652235291, 5.279956712948652431, 0.7216878364870338292 ) ) ;
#86718=CARTESIAN_POINT ( 'NONE',  ( -5.631432701629818460, 7.663367133358481631, 1.599625672291263179 ) ) ;
#86722=CARTESIAN_POINT ( 'NONE',  ( -4.610654757099099221, 7.536791762327691657, 1.199719254218452935 ) ) ;
#86726=CARTESIAN_POINT ( 'NONE',  ( -6.604230223188181093, 6.877559146573883453, 0.7216878364870317197 ) ) ;
#86732=CARTESIAN_POINT ( 'NONE',  ( -6.882699257592852504, 8.058845884393651460, -1.199719254218452047 ) ) ;
#86741=CARTESIAN_POINT ( 'NONE',  ( -6.903036488013351679, 8.082572653217566128, -1.199719254218452047 ) ) ;
#86743=CARTESIAN_POINT ( 'NONE',  ( 4.617922728991994852, 8.461530327540957686, 0.3091873533234041904 ) ) ;
#86748=CARTESIAN_POINT ( 'NONE',  ( 5.820193082016415609, 10.01225203898631655, 0.000000000000000000 ) ) ;
#86761=CARTESIAN_POINT ( 'NONE',  ( -6.074935347375019390, 9.245119117649618801, 1.199719254218452047 ) ) ;
#86764=DIRECTION ( 'NONE',  ( 0.000000000000000000, 1.000000000000000000, 0.000000000000000000 ) ) ;
#86774=CARTESIAN_POINT ( 'NONE',  ( 6.367489420273535039, 7.457767740854454708, -1.199719254218452047 ) ) ;
#86787=CARTESIAN_POINT ( 'NONE',  ( -0.1476870296772063995, 2.615815853600972130, 2.075651118116234706 ) ) ;
#86788=CARTESIAN_POINT ( 'NONE',  ( 5.646014316602349759, 7.456765758048159221, -1.329534273556526758 ) ) ;
#86797=CARTESIAN_POINT ( 'NONE',  ( -5.346851039111044201, 6.199209027673978412, 7.500000000000000000 ) ) ;
#86817=CARTESIAN_POINT ( 'NONE',  ( -6.569648045741773856, 6.787758985223060648, 0.3860807628459517749 ) ) ;
#86836=CARTESIAN_POINT ( 'NONE',  ( -4.308458954092677651, 8.248562223075252220, -0.7998128361456362523 ) ) ;
#86849=B_SPLINE_CURVE_WITH_KNOTS ( 'NONE', 3,
 ( #157540, #156470, #109914, #8058 ),
 .UNSPECIFIED., .F., .F.,
 ( 4, 4 ),
 ( 7.552443772458755810E-16, 0.0003455271673302856279 ),
 .UNSPECIFIED. ) ;
#86854=CARTESIAN_POINT ( 'NONE',  ( 4.598150373690133463, 5.393538853173795111, -1.199719254218452047 ) ) ;
#86856=CARTESIAN_POINT ( 'NONE',  ( 7.309254211098760834, 8.660456346770972758, 1.082531754730549967 ) ) ;
#86869=CARTESIAN_POINT ( 'NONE',  ( -4.762657100150483380, 8.778460060142702304, 0.000000000000000000 ) ) ;
#86871=CARTESIAN_POINT ( 'NONE',  ( 5.692444392891300886, 7.734547439830227411, -1.599625672291281386 ) ) ;
#86881=CARTESIAN_POINT ( 'NONE',  ( -3.657667580636712934, 7.489305620709952649, -0.7998128361456481317 ) ) ;
#86882=CARTESIAN_POINT ( 'NONE',  ( 3.074666975249065626, 6.809138247757705820, 0.000000000000000000 ) ) ;
#86884=CARTESIAN_POINT ( 'NONE',  ( -6.615342224808818727, 6.750480251133849308, 0.3470571717737805373 ) ) ;
#86890=CARTESIAN_POINT ( 'NONE',  ( 6.387826650694035990, 7.481494509678370264, -1.199719254218452047 ) ) ;
#86895=CARTESIAN_POINT ( 'NONE',  ( -4.599258460307840579, 8.480642220064158465, 0.2485357878534207865 ) ) ;
#86901=VECTOR ( 'NONE', #103354, 1000.000000000000114 ) ;
#86906=CARTESIAN_POINT ( 'NONE',  ( -4.299344108864949554, 8.030002203735486788, -0.7216878364870338292 ) ) ;
#86915=CARTESIAN_POINT ( 'NONE',  ( 3.418064124421011041, 7.001842221884225559, -0.7216878364870338292 ) ) ;
#86919=CARTESIAN_POINT ( 'NONE',  ( -5.315678745009726924, 8.359319748223434487, -1.199719254218453823 ) ) ;
#86933=CARTESIAN_POINT ( 'NONE',  ( 3.790386463472274148, 6.579812086429759788, 1.199719254218452047 ) ) ;
#86937=CARTESIAN_POINT ( 'NONE',  ( 6.412080304620305427, 6.445458208337293549, -0.7998128361456481317 ) ) ;
#86956=ADVANCED_FACE ( 'NONE', ( #188844 ), #209319, .T. ) ;
#86957=CARTESIAN_POINT ( 'NONE',  ( -0.2916131387015714060, 3.292968587997009422, 2.053236966640526351 ) ) ;
#86959=CARTESIAN_POINT ( 'NONE',  ( -5.153507786970275006, 7.105788066255672497, -1.443375672974066548 ) ) ;
#86981=CARTESIAN_POINT ( 'NONE',  ( -5.121948170912633991, 9.197632976031879792, -0.7998128361456362523 ) ) ;
#86986=CARTESIAN_POINT ( 'NONE',  ( -3.471769853551161411, 6.208092708188416076, 1.199719254218452935 ) ) ;
#86993=CARTESIAN_POINT ( 'NONE',  ( -7.262327558775498737, 8.501745569106741840, 1.199719254218452047 ) ) ;
#87000=CARTESIAN_POINT ( 'NONE',  ( 4.577813143269636065, 5.369812084349879555, -1.199719254218450271 ) ) ;
#87005=CARTESIAN_POINT ( 'NONE',  ( -5.101610940492132151, 9.173906207207963348, -0.7998128361456362523 ) ) ;
#87009=CARTESIAN_POINT ( 'NONE',  ( -2.823841133396259639, 6.516508098929413961, -0.7998128361456481317 ) ) ;
#87013=CARTESIAN_POINT ( 'NONE',  ( 4.136646265500957043, 5.919449624541475607, -1.443375672974068769 ) ) ;
#87014=CARTESIAN_POINT ( 'NONE',  ( -6.427974226210522168, 6.671927150099951298, 0.000000000000000000 ) ) ;
#87020=CARTESIAN_POINT ( 'NONE',  ( -3.962726036944197450, 7.845207153068689543, -0.7998128361456481317 ) ) ;
#87024=ORIENTED_EDGE ( 'NONE', *, *, #62930, .F. ) ;
#87034=CARTESIAN_POINT ( 'NONE',  ( 5.753927575595171540, 7.371122731025397279, 1.306365966420112601 ) ) ;
#87044=CARTESIAN_POINT ( 'NONE',  ( 7.388267364804250725, 7.584343111885245570, -0.7998128361456341429 ) ) ;
#87055=CARTESIAN_POINT ( 'NONE',  ( 6.479309170914094196, 6.755949689298615723, 0.1985876171829506487 ) ) ;
#87073=CARTESIAN_POINT ( 'NONE',  ( -6.466312919074983512, 6.508729591867735031, -0.7998128361456362523 ) ) ;
#87086=CARTESIAN_POINT ( 'NONE',  ( 6.547661840756936691, 6.603636667163397256, 0.7998128361456352531 ) ) ;
#87088=CARTESIAN_POINT ( 'NONE',  ( 7.075376061485196821, 9.347967719856493218, 1.599625672291268286 ) ) ;
#87098=CARTESIAN_POINT ( 'NONE',  ( 4.868786560638889149, 6.773613302202437403, 1.443375672974065660 ) ) ;
#87112=CARTESIAN_POINT ( 'NONE',  ( -7.756673280794142755, 8.222076047114187602, -0.7216878364870338292 ) ) ;
#87113=CARTESIAN_POINT ( 'NONE',  ( 5.234856708652215751, 9.121433570154021453, 0.7216878364870317197 ) ) ;
#87124=CARTESIAN_POINT ( 'NONE',  ( -3.474632506852224356, 7.275764701294714420, -0.7998128361456481317 ) ) ;
#87125=CARTESIAN_POINT ( 'NONE',  ( -6.943184063974175757, 9.193743722760251202, -1.443375672974066548 ) ) ;
#87128=CARTESIAN_POINT ( 'NONE',  ( 4.868786560638878491, 8.694351730805124134, 0.7216878364870317197 ) ) ;
#87130=ORIENTED_EDGE ( 'NONE', *, *, #50115, .F. ) ;
#87133=CARTESIAN_POINT ( 'NONE',  ( -5.623259694695312838, 5.814328530587530075, 0.3973859538428151650 ) ) ;
#87136=CARTESIAN_POINT ( 'NONE',  ( -4.918597572616692837, 8.113217865663214567, 1.086842401077245279 ) ) ;
#87140=CARTESIAN_POINT ( 'NONE',  ( -4.693116838625758014, 8.272874032808440248, 0.5769273507626712094 ) ) ;
#87147=CARTESIAN_POINT ( 'NONE',  ( -5.306037014901836990, 7.283738832175834510, 1.599625672291263179 ) ) ;
#87159=CARTESIAN_POINT ( 'NONE',  ( 5.890091390494168522, 5.836471141856793388, 0.000000000000000000 ) ) ;
#87200=CARTESIAN_POINT ( 'NONE',  ( 5.885648082108190238, 7.959951743916638733, 1.443375672974065660 ) ) ;
#87205=CARTESIAN_POINT ( 'NONE',  ( 5.438229012412886476, 7.437962829272074750, -1.443375672974078761 ) ) ;
#87221=CARTESIAN_POINT ( 'NONE',  ( -6.851666526859749418, 9.086973262793417661, -1.599625672291271394 ) ) ;
#87231=CARTESIAN_POINT ( 'NONE',  ( -2.979759899953417612, 6.698413326579433225, 0.7998128361456352531 ) ) ;
#87233=CARTESIAN_POINT ( 'NONE',  ( 4.136646265500957043, 5.919449624541475607, -1.443375672974068769 ) ) ;
#87239=CARTESIAN_POINT ( 'NONE',  ( -5.354544322754380303, 5.211666229493680191, 0.7998128361456281477 ) ) ;
#87244=CARTESIAN_POINT ( 'NONE',  ( -7.268579750702168774, 7.652633595340216921, -0.7216878364870338292 ) ) ;
#87248=CARTESIAN_POINT ( 'NONE',  ( -7.598418745816086783, 7.829519723065708092, 0.000000000000000000 ) ) ;
#87268=CARTESIAN_POINT ( 'NONE',  ( -5.980555157403903976, 6.149938236492225485, 0.000000000000000000 ) ) ;
#87270=CARTESIAN_POINT ( 'NONE',  ( -4.570507181138272479, 7.385989907086349504, 1.082531754730549967 ) ) ;
#87271=CARTESIAN_POINT ( 'NONE',  ( 3.901714345682657292, 7.774026846596938434, 0.7998128361456271485 ) ) ;
#87272=CARTESIAN_POINT ( 'NONE',  ( -5.764151584465413869, 6.753873599078290546, -1.199719254218453823 ) ) ;
#87273=CARTESIAN_POINT ( 'NONE',  ( -5.607179047703544583, 8.699403434699558346, 1.199719254218454489 ) ) ;
#87331=CARTESIAN_POINT ( 'NONE',  ( 5.387385936583818591, 7.378645907471495846, -1.599625672291283607 ) ) ;
#87332=CARTESIAN_POINT ( 'NONE',  ( 5.939880696562888751, 7.062853913145737295, -1.082531754730548412 ) ) ;
#87350=CARTESIAN_POINT ( 'NONE',  ( 4.692003678781083487, 7.631698837623355658, -1.199719254218450271 ) ) ;
#87356=CARTESIAN_POINT ( 'NONE',  ( -7.286581212701773502, 7.465709267765667789, 0.7998128361456341429 ) ) ;
#87360=CARTESIAN_POINT ( 'NONE',  ( 4.037295881819344956, 7.932205305423046582, -0.7998128361456362523 ) ) ;
#87361=ORIENTED_EDGE ( 'NONE', *, *, #181468, .T. ) ;
#87366=CARTESIAN_POINT ( 'NONE',  ( -6.305925513666572613, 6.529536985466737775, -1.006778644550405474E-06 ) ) ;
#87370=CARTESIAN_POINT ( 'NONE',  ( -5.606595252507366567, 5.572856915785063592, -0.3451608010808376870 ) ) ;
#87371=CARTESIAN_POINT ( 'NONE',  ( 5.966997003790217136, 8.054858819212300958, -1.443375672974078761 ) ) ;
#87373=CARTESIAN_POINT ( 'NONE',  ( -5.045042558060949034, 6.018876084893449274, 1.082531754730549078 ) ) ;
#87374=CARTESIAN_POINT ( 'NONE',  ( -4.613517410400161722, 8.604463755433990002, -0.7998128361456362523 ) ) ;
#87387=CARTESIAN_POINT ( 'NONE',  ( 3.718679271898170491, 7.560485927181699317, 0.7998128361456271485 ) ) ;
#87388=CARTESIAN_POINT ( 'NONE',  ( 6.387826650694035990, 7.481494509678370264, -1.199719254218452047 ) ) ;
#87394=ORIENTED_EDGE ( 'NONE', *, *, #191290, .F. ) ;
#87403=VECTOR ( 'NONE', #184214, 1000.000000000000000 ) ;
#87409=CARTESIAN_POINT ( 'NONE',  ( 5.586791213849657822, 7.504901977030062454, -1.335864709735144817 ) ) ;
#87418=CARTESIAN_POINT ( 'NONE',  ( 4.706615602599436343, 5.520081620234675412, 1.199719254218452935 ) ) ;
#87422=CARTESIAN_POINT ( 'NONE',  ( 8.005163354226054295, 8.304055099544019214, 0.000000000000000000 ) ) ;
#87427=CARTESIAN_POINT ( 'NONE',  ( 6.536439455564164724, 7.758839131980592718, 1.082531754730549967 ) ) ;
#87430=CARTESIAN_POINT ( 'NONE',  ( 6.699137298928145690, 8.909022496873262753, 1.443375672974065660 ) ) ;
#87441=CARTESIAN_POINT ( 'NONE',  ( 6.469672735924913987, 6.762149564967588233, 0.2594904213018677797 ) ) ;
#87442=CARTESIAN_POINT ( 'NONE',  ( -3.284818356260900796, 7.054314858938165678, 0.7998128361456352531 ) ) ;
#87447=B_SPLINE_CURVE_WITH_KNOTS ( 'NONE', 3,
 ( #126016, #75051, #6819, #24144, #190915, #90246, #72898, #174712, #22849, #103067, #119376, #118309, #3400, #4456, #90031, #53246, #70526, #170185, #136643, #202668 ),
 .UNSPECIFIED., .F., .F.,
 ( 4, 2, 1, 1, 1, 1, 2, 2, 2, 2, 2, 4 ),
 ( 0.9387693520046538342, 0.9388889431140197139, 0.9390085342233857046, 0.9392477164421174640, 0.9397260808795810938, 0.9406828097545083534, 0.9425962675043629835, 0.9464231830040721327, 0.9540770140034904312, 0.9693846760023269171, 0.9846923380011635141, 1.000000000000000000 ),
 .UNSPECIFIED. ) ;
#87453=CARTESIAN_POINT ( 'NONE',  ( 0.3581693041846744086, 3.206512658508270164, -2.035393093115380747 ) ) ;
#87478=CARTESIAN_POINT ( 'NONE',  ( 6.852720297064418986, 6.959538199522133262, 0.7998128361456331437 ) ) ;
#87480=CARTESIAN_POINT ( 'NONE',  ( 5.013482942003290255, 9.071090208970993274, -0.7998128361456481317 ) ) ;
#87482=DIRECTION ( 'NONE',  ( -1.000000000000000000, 0.000000000000000000, 0.000000000000000000 ) ) ;
#87495=CARTESIAN_POINT ( 'NONE',  ( -5.472651281771599763, 6.413789912602166687, 1.199719254218452935 ) ) ;
#87497=CARTESIAN_POINT ( 'NONE',  ( 6.712695452097489301, 7.964471127936110229, -1.082531754730548412 ) ) ;
#87503=AXIS2_PLACEMENT_3D ( 'NONE', #143172, #58674, #124823 ) ;
#87508=CARTESIAN_POINT ( 'NONE',  ( -4.339491684825780737, 7.220434844675483355, -1.199719254218455378 ) ) ;
#87514=CARTESIAN_POINT ( 'NONE',  ( -3.634467696915153034, 6.397906858779740524, 1.199719254218452935 ) ) ;
#87516=CARTESIAN_POINT ( 'NONE',  ( -5.316205630334263965, 7.295602216847000498, -1.443375672974066548 ) ) ;
#87537=CARTESIAN_POINT ( 'NONE',  ( -5.712781623311813384, 7.758274208654143855, -1.599625672291271394 ) ) ;
#87538=CARTESIAN_POINT ( 'NONE',  ( -5.029148636026397945, 4.832037928311032182, 0.7998128361456281477 ) ) ;
#87546=CARTESIAN_POINT ( 'NONE',  ( 1.823500102806385970, 2.449814546280965732, -2.460149141570041831 ) ) ;
#87547=CARTESIAN_POINT ( 'NONE',  ( -6.453559683527718249, 6.864596255245277057, -0.6992757447422948136 ) ) ;
#87578=CARTESIAN_POINT ( 'NONE',  ( 3.413620815590684199, 7.204584394822967752, 0.7998128361456281477 ) ) ;
#87586=CARTESIAN_POINT ( 'NONE',  ( 7.523848900940885542, 7.742521570711348389, 0.7998128361456291469 ) ) ;
#87588=CARTESIAN_POINT ( 'NONE',  ( 5.071631979963703962, 8.074598522336444262, 1.199719254218451159 ) ) ;
#87601=DIRECTION ( 'NONE',  ( 0.000000000000000000, -1.000000000000000000, 0.000000000000000000 ) ) ;
#87602=CARTESIAN_POINT ( 'NONE',  ( 6.492506472431533560, 6.747478052702773788, -0.04572756507489894595 ) ) ;
#87605=CARTESIAN_POINT ( 'NONE',  ( 4.746763178560250651, 7.591621904078704297, 1.082531754730549078 ) ) ;
#87611=CARTESIAN_POINT ( 'NONE',  ( -4.981695098378565945, 4.776675467721892332, -0.7998128361456362523 ) ) ;
#87614=ORIENTED_EDGE ( 'NONE', *, *, #40364, .F. ) ;
#87622=CARTESIAN_POINT ( 'NONE',  ( -6.427974226210522168, 6.671927150099951298, 0.000000000000000000 ) ) ;
#87626=CARTESIAN_POINT ( 'NONE',  ( 4.505052181490820651, 8.477920988373101707, -0.7998128361456381397 ) ) ;
#87644=CARTESIAN_POINT ( 'NONE',  ( -5.361566827843197380, 4.701484413405883522, -2.440314516401218992 ) ) ;
#87679=CARTESIAN_POINT ( 'NONE',  ( 5.072158865288243668, 6.050511776658669127, 1.082531754730549078 ) ) ;
#87685=CARTESIAN_POINT ( 'NONE',  ( 6.200875153403774043, 8.327716660428123419, -1.599625672291283607 ) ) ;
#87689=CARTESIAN_POINT ( 'NONE',  ( -3.824808732831001201, 7.476377598362539345, 0.7216878364870338292 ) ) ;
#87704=AXIS2_PLACEMENT_3D ( 'NONE', #139016, #203962, #39360 ) ;
#87721=CARTESIAN_POINT ( 'NONE',  ( 7.512626515748113576, 7.937354821227203594, 0.7216878364870267237 ) ) ;
#87734=CARTESIAN_POINT ( 'NONE',  ( -5.641601317062247212, 7.675230518029648508, -1.443375672974066548 ) ) ;
#87736=CARTESIAN_POINT ( 'NONE',  ( 6.363572996767764778, 8.517530811019446091, -1.599625672291283607 ) ) ;
#87741=CARTESIAN_POINT ( 'NONE',  ( -6.317173229324657413, 6.334733287159020954, 0.000000000000000000 ) ) ;
#87743=CARTESIAN_POINT ( 'NONE',  ( 3.947215336577725164, 7.320702380770685025, -0.8969922371624715618 ) ) ;
#87785=CARTESIAN_POINT ( 'NONE',  ( 3.431622278034673901, 7.017660067766835930, -1.734723475976807094E-15 ) ) ;
#87789=CARTESIAN_POINT ( 'NONE',  ( -4.606738333593328072, 8.596554832492683929, 0.7998128361456281477 ) ) ;
#87793=CARTESIAN_POINT ( 'NONE',  ( -5.743814354044916470, 6.730146830254374990, -1.199719254218453823 ) ) ;
#87794=CARTESIAN_POINT ( 'NONE',  ( -4.522526758610270647, 7.433975764090723359, -1.199719254218453823 ) ) ;
#87798=CARTESIAN_POINT ( 'NONE',  ( -5.438229012412888252, 9.358701257874761481, -0.7216878364870338292 ) ) ;
#87806=CARTESIAN_POINT ( 'NONE',  ( -5.887983850084758330, 10.09134126839936840, 0.7998128361456291469 ) ) ;
#87814=CARTESIAN_POINT ( 'NONE',  ( -7.095713291905736853, 9.371694488680407886, 1.599625672291269396 ) ) ;
#87815=ORIENTED_EDGE ( 'NONE', *, *, #40298, .T. ) ;
#87816=CARTESIAN_POINT ( 'NONE',  ( 4.596911992430688265, 8.487755744900498556, -0.08351877912710949092 ) ) ;
#87821=CARTESIAN_POINT ( 'NONE',  ( 4.706615602599436343, 5.520081620234675412, 1.199719254218452935 ) ) ;
#87833=CARTESIAN_POINT ( 'NONE',  ( -8.086512275908061653, 8.398962174839683215, 0.000000000000000000 ) ) ;
#87845=CARTESIAN_POINT ( 'NONE',  ( 6.373214726875630731, 9.593111727067046957, 1.199719254218452047 ) ) ;
#87858=CARTESIAN_POINT ( 'NONE',  ( -0.4000000000000114575, 2.999999999999999112, 2.023857702507764422 ) ) ;
#87859=CARTESIAN_POINT ( 'NONE',  ( 6.378761646814803399, 6.917158162233129737, 0.8102004381213165907 ) ) ;
#87885=CARTESIAN_POINT ( 'NONE',  ( -5.987767821832088444, 7.191367801968548079, 1.216456708157914512 ) ) ;
#87904=CARTESIAN_POINT ( 'NONE',  ( -5.550083779947821760, 7.568460058062819407, -1.599625672291271394 ) ) ;
#87919=CARTESIAN_POINT ( 'NONE',  ( 3.923105346307896202, 5.670318552149568703, -1.599625672291269396 ) ) ;
#87921=CARTESIAN_POINT ( 'NONE',  ( 5.844973620822823790, 9.833236634353070826, 0.7216878364870317197 ) ) ;
#87938=CARTESIAN_POINT ( 'NONE',  ( 4.854701522145073334, 7.821512988214679218, -1.199719254218450271 ) ) ;
#87948=CARTESIAN_POINT ( 'NONE',  ( -3.793249116773374396, 7.647484079536056356, 0.7998128361456352531 ) ) ;
#87949=CARTESIAN_POINT ( 'NONE',  ( 5.643937085038755797, 9.806620042512378177, -0.7998128361456481317 ) ) ;
#87953=CARTESIAN_POINT ( 'NONE',  ( -5.478376588373717659, 8.549133898814758936, -1.199719254218452047 ) ) ;
#87956=CARTESIAN_POINT ( 'NONE',  ( 5.875479466675786355, 7.948088359245467416, -1.599625672291283607 ) ) ;
#87961=CARTESIAN_POINT ( 'NONE',  ( -4.584844773125573703, 8.498748274393685520, 0.004977730536110530624 ) ) ;
#87972=CARTESIAN_POINT ( 'NONE',  ( -5.763624699140883934, 6.857221916153382502, -1.082531754730549967 ) ) ;
#87982=CARTESIAN_POINT ( 'NONE',  ( 5.411112705629925301, 5.485588709422586362, 0.000000000000000000 ) ) ;
#87985=CARTESIAN_POINT ( 'NONE',  ( -5.424143973919053785, 8.485862515284315677, 1.199719254218454489 ) ) ;
#88002=CARTESIAN_POINT ( 'NONE',  ( 5.273195401072370281, 5.116759154198018855, -0.7998128361456481317 ) ) ;
#88026=CARTESIAN_POINT ( 'NONE',  ( -5.695833931516914639, 6.778132687258748845, 1.082531754730549078 ) ) ;
#88039=EDGE_CURVE ( 'NONE', #196836, #88097, #125428, .T. ) ;
#88052=CARTESIAN_POINT ( 'NONE',  ( -7.119966945832006289, 8.335658187339330283, 1.199719254218452047 ) ) ;
#88058=CARTESIAN_POINT ( 'NONE',  ( -3.772911886352873445, 7.623757310712140800, 0.7998128361456352531 ) ) ;
#88067=CARTESIAN_POINT ( 'NONE',  ( -4.950662367645459305, 5.804802846121667415, -1.199719254218453823 ) ) ;
#88069=CARTESIAN_POINT ( 'NONE',  ( 4.936581118797800372, 8.100871430792054184, -1.059671831818540966 ) ) ;
#88073=CARTESIAN_POINT ( 'NONE',  ( 4.044074958626150185, 7.940114228364351767, 0.7998128361456271485 ) ) ;
#88078=CARTESIAN_POINT ( 'NONE',  ( -6.774234028683526532, 7.932303117332766718, 1.199719254218452047 ) ) ;
#88083=CARTESIAN_POINT ( 'NONE',  ( -3.122120512896910505, 6.864500708346841229, 0.7998128361456352531 ) ) ;
#88087=CARTESIAN_POINT ( 'NONE',  ( -7.065207446052809814, 9.336104335185325453, -1.443375672974066548 ) ) ;
#88088=CARTESIAN_POINT ( 'NONE',  ( 5.356880090730874677, 5.422317325373725794, 0.7216878364870328300 ) ) ;
#88089=CARTESIAN_POINT ( 'NONE',  ( -4.123088111887291518, 7.824370207261548416, 0.000000000000000000 ) ) ;
#88093=CARTESIAN_POINT ( 'NONE',  ( -5.418418667316934112, 6.350518529071726981, -1.199719254218453823 ) ) ;
#88096=CARTESIAN_POINT ( 'NONE',  ( 3.555981428534177091, 7.370671776590375757, 0.7998128361456271485 ) ) ;
#88097=VERTEX_POINT ( 'NONE', #13057 ) ;
#88100=CIRCLE ( 'NONE', #160768, 0.08000000000000025147 ) ;
#88108=CARTESIAN_POINT ( 'NONE',  ( 1.854512760316388897, 2.488359591189891251, 2.484105960264901825 ) ) ;
#88109=CARTESIAN_POINT ( 'NONE',  ( 5.820234798683411981, 7.319712794923219690, 1.284739950006764220 ) ) ;
#88115=CARTESIAN_POINT ( 'NONE',  ( 6.076298462418691315, 7.128931413452940014, -1.143247356662546732 ) ) ;
#88119=CARTESIAN_POINT ( 'NONE',  ( 6.900173834712277632, 7.014900660111269559, -0.7998128361456341429 ) ) ;
#88129=CARTESIAN_POINT ( 'NONE',  ( 6.385878362533466301, 6.816559200039058020, 0.5486352003098924346 ) ) ;
#88141=CARTESIAN_POINT ( 'NONE',  ( 4.879147978569815969, 4.879180288469956217, -0.1512534140984626019 ) ) ;
#88147=CARTESIAN_POINT ( 'NONE',  ( -6.414942957921379474, 7.513130201443591005, -1.199719254218452047 ) ) ;
#88160=CARTESIAN_POINT ( 'NONE',  ( 4.213551878797002992, 8.137837301896977849, 0.000000000000000000 ) ) ;
#88168=ORIENTED_EDGE ( 'NONE', *, *, #30238, .T. ) ;
#88171=CARTESIAN_POINT ( 'NONE',  ( 4.299344108864946890, 6.109263775132799168, -1.443375672974068769 ) ) ;
#88187=CARTESIAN_POINT ( 'NONE',  ( -7.770231434407805615, 8.237893892996801526, 0.000000000000000000 ) ) ;
#88188=CARTESIAN_POINT ( 'NONE',  ( 4.909461021924231616, 8.741805268971372556, 0.7216878364870317197 ) ) ;
#88197=CARTESIAN_POINT ( 'NONE',  ( -6.296835998904160014, 6.311006518335105397, 0.000000000000000000 ) ) ;
#88198=CARTESIAN_POINT ( 'NONE',  ( -4.984557751679625781, 5.844347460828191565, 1.199719254218452935 ) ) ;
#88201=CARTESIAN_POINT ( 'NONE',  ( 6.522881301506172846, 6.782652071278222117, -0.7216878364870458196 ) ) ;
#88203=EDGE_LOOP ( 'NONE', ( #96806, #141257 ) ) ;
#88206=EDGE_CURVE ( 'NONE', #96770, #184855, #212880, .T. ) ;
#88210=CARTESIAN_POINT ( 'NONE',  ( -6.177748251148500458, 7.053635085330046905, 1.079103885897433779 ) ) ;
#88214=CARTESIAN_POINT ( 'NONE',  ( -4.612386318492403880, 8.373339136000554461, 0.1892495524792922046 ) ) ;
#88218=CARTESIAN_POINT ( 'NONE',  ( 4.421367491832268293, 7.211993602896056288, 1.082531754730549078 ) ) ;
#88222=CARTESIAN_POINT ( 'NONE',  ( -4.522526758610270647, 7.433975764090723359, -1.199719254218453823 ) ) ;
#88235=CARTESIAN_POINT ( 'NONE',  ( 4.193214648376505593, 8.114110533073061404, 0.000000000000000000 ) ) ;
#88237=EDGE_CURVE ( 'NONE', #183165, #123242, #3622, .T. ) ;
#88252=DIRECTION ( 'NONE',  ( -0.7592566023653003482, 0.6507913734559641616, 0.000000000000000000 ) ) ;
#88273=CARTESIAN_POINT ( 'NONE',  ( 6.224601922449876312, 6.434659462379210382, 0.000000000000000000 ) ) ;
#88280=CARTESIAN_POINT ( 'NONE',  ( 6.224601922005513543, 7.395028676162137771, -1.082531754730548412 ) ) ;
#88298=CARTESIAN_POINT ( 'NONE',  ( -8.106849506328558164, 8.422688943663599659, 0.000000000000000000 ) ) ;
#88309=CARTESIAN_POINT ( 'NONE',  ( 3.716343503477301802, 7.349834830783237294, -1.734723475976807094E-15 ) ) ;
#88315=CARTESIAN_POINT ( 'NONE',  ( -4.492547798081878874, 6.334668079219206049, 1.599625672291263179 ) ) ;
#88320=CARTESIAN_POINT ( 'NONE',  ( -6.455090533882193782, 9.584670485287619002, -1.082531754730549967 ) ) ;
#88323=CARTESIAN_POINT ( 'NONE',  ( -5.738844160334429567, 9.917344963690652548, 0.000000000000000000 ) ) ;
#88328=CARTESIAN_POINT ( 'NONE',  ( -3.962726036944197894, 7.845207153068690431, -0.7998128361456481317 ) ) ;
#88339=B_SPLINE_CURVE_WITH_KNOTS ( 'NONE', 3,
 ( #168807, #71282, #137395, #152558, #4145, #199148, #70216, #203414, #187187, #175239 ),
 .UNSPECIFIED., .F., .F.,
 ( 4, 3, 3, 4 ),
 ( 2.070599078951341269E-17, 6.251588761609448285E-05, 0.0001877407159084782664, 0.0003399624922859439112 ),
 .UNSPECIFIED. ) ;
#88342=CARTESIAN_POINT ( 'NONE',  ( -3.838366886444665393, 7.492195444245147939, 0.000000000000000000 ) ) ;
#88344=CARTESIAN_POINT ( 'NONE',  ( -4.136646265500964148, 6.879818838842817641, -1.082531754730551743 ) ) ;
#88346=CARTESIAN_POINT ( 'NONE',  ( 4.376249722160992839, 8.327651452488305850, 0.000000000000000000 ) ) ;
#88347=CARTESIAN_POINT ( 'NONE',  ( -5.631432701629818460, 7.663367133358481631, 1.599625672291263179 ) ) ;
#88348=CARTESIAN_POINT ( 'NONE',  ( -5.610041701004606196, 9.767075427805856691, -0.7998128361456362523 ) ) ;
#88351=FACE_BOUND ( 'NONE', #195313, .T. ) ;
#88389=( BOUNDED_SURFACE ( )  B_SPLINE_SURFACE ( 1, 2, ( 
 ( #169680, #55940, #206443, #205370, #190192, #122093, #121026, #23414, #38624, #171821, #170751, #41851, #22337, #203228, #57005, #9320, #156652, #123177, #155579, #71088, #189136, #107961, #173989, #89526, #40775, #54873, #185914, #141506, #137206, #154510, #186993, #37548, #106880, #21268, #188057, #58070, #172907, #25561, #39686, #104700, #7163, #88451, #73233, #6092, #91672, #72160, #138269, #204283, #157725, #103628, #139340, #24481, #90593, #74329, #8245, #124233, #87373, #75394, #207515, #59133, #153443, #5015, #77518, #110095, #93801, #211772, #193405, #142557, #208564, #60198, #78581, #63410, #159841, #95935, #29855, #12510, #210714, #178238, #176106, #45049, #62342, #61273, #129561, #161991, #13581, #209633, #194470, #47185, #145771, #127435, #79654, #11442, #195548, #113299, #179306, #192318, #175045, #80730, #43976, #126359, #30927, #111161, #10373, #97003, #128502, #163056, #94861, #46112, #27706, #14636, #146820, #143639, #177161, #212840, #125293, #191251, #112230, #42916, #109026, #28779, #160916, #158777, #144703, #26630, #92732, #76450, #35146, #196610, #64477, #98062, #83904, #101223, #132703, #65508, #50354, #147870, #131654, #198709, #167306, #184598, #166230, #493, #19963, #52481, #15701, #130617, #165165, #116476, #182466, #118609, #18893, #66561, #82843, #48249, #16760, #114364, #149994, #148920, #133772, #81787, #84977, #213885, #151069, #180358, #34095, #2631, #68704, #134826, #100166, #99116, #197657, #49303, #200830, #181411, #17821, #183540, #199780, #1565, #36215, #102294, #67627, #168368, #86047, #152123, #31984, #164118, #51426, #115419, #117546, #33038, #72981, #6904, #204029, #5834, #22075, #41594, #135876, #187804, #169430, #140164, #103368, #69770, #185666, #171559, #172650, #170491, #136949, #201895, #188877, #139084, #107705, #206187, #7982, #21014, #23156, #56754, #53548, #39432, #120763, #205111, #119679, #87112, #88187, #57815, #71905, #123977, #153182, #4756, #90327, #25308, #189944, #173731, #70831, #105525, #202974, #156396, #154259, #91410, #54615, #74071, #3693 ),
 ( #106620, #37295, #89271, #138014, #155320, #186741, #40518, #122919, #24225, #38363, #104442, #55677, #121833, #77264, #160657, #174797, #157470, #113045, #42663, #126103, #26373, #59947, #12254, #143377, #45861, #210456, #142306, #141249, #192063, #158525, #78331, #145520, #159586, #109841, #208317, #43726, #29598, #11184, #92486, #10122, #76197, #110902, #95684, #175855, #128253, #62094, #44797, #28523, #194216, #27444, #209376, #94613, #93542, #161738, #111982, #177983, #61020, #144453, #79403, #13329, #127179, #211519, #193147, #63155, #129320, #195296, #176908, #207258, #179051, #46927, #30670, #9065, #75140, #108772, #58886, #125042, #190997, #66319, #33844, #213636, #51174, #117297, #65263, #147618, #183294, #52238, #34899, #165986, #100972, #2384, #114119, #49050, #130370, #81536, #181165, #212589, #184354, #67384, #14380, #96753, #196361, #116230, #133524, #164917, #97808, #82592, #180111, #163871, #16510, #199531, #68462, #198465, #32789, #182221, #134590, #167061, #99925, #132463, #48001, #17572, #18653, #84732, #148679, #83656, #31735, #162803, #118365, #15447, #131409, #197409, #80472, #149746, #146571, #98865, #150821, #1323, #200590, #247, #115170, #50109, #64228, #24778, #20773, #43200, #86869, #53302, #103123, #175325, #168122, #35976, #208847, #135632, #4512, #119434, #102056, #190473, #19723, #123460, #207791, #58361, #109314, #189423, #185421, #90879, #169181, #156941, #152935, #26908, #70584, #37039, #139636, #93014, #85802, #205659, #42133, #173198, #141785, #91950, #57295, #151882, #41064, #107171, #174268, #159057, #8532, #74611, #140717, #206731, #125575, #124514, #108245, #25843, #158012, #9599, #191536, #75676, #59419, #10653, #76726, #142842, #60478, #126636, #3456, #69525, #201652, #130885, #97272, #31196, #62605, #47459, #114637, #213111, #128767, #81000, #12779, #64743, #147088, #196879, #45320, #27987, #148149, #111439, #61551, #48516, #194743, #77798, #180629, #195819, #163326, #162260, #129838, #95141, #32252, #98322, #161191, #29058, #164387, #214150, #15971, #113574, #82057 ) ),
 .UNSPECIFIED., .F., .F., .T. ) 
 B_SPLINE_SURFACE_WITH_KNOTS ( ( 2, 2 ),
 ( 3, 2, 2, 2, 2, 2, 2, 2, 2, 2, 2, 2, 2, 2, 2, 2, 2, 2, 2, 2, 2, 2, 2, 2, 2, 2, 2, 2, 2, 2, 2, 2, 2, 2, 2, 2, 2, 2, 2, 2, 2, 2, 2, 2, 2, 2, 2, 2, 2, 2, 2, 2, 2, 2, 2, 2, 2, 2, 2, 2, 2, 2, 2, 2, 2, 2, 2, 2, 2, 2, 2, 2, 2, 2, 2, 2, 2, 2, 2, 2, 2, 2, 2, 2, 2, 2, 2, 2, 2, 2, 2, 2, 2, 2, 2, 2, 2, 2, 2, 2, 2, 2, 2, 2, 2, 2, 2, 2, 2, 2, 2, 2, 2, 2, 2, 2, 2, 2, 2, 2, 3 ),
 ( 0.000000000000000000, 1.000000000000000000 ),
 ( 0.000000000000000000, 0.008333333333333333218, 0.01666666666666666644, 0.02500000000000000139, 0.03333333333333333287, 0.04166666666666666435, 0.05000000000000000278, 0.05833333333333333426, 0.06666666666666666574, 0.07499999999999999722, 0.08333333333333332871, 0.09166666666666666019, 0.1000000000000000056, 0.1083333333333333370, 0.1166666666666666685, 0.1250000000000000000, 0.1333333333333333315, 0.1416666666666666630, 0.1499999999999999944, 0.1583333333333333259, 0.1666666666666666574, 0.1749999999999999889, 0.1833333333333333204, 0.1916666666666666796, 0.2000000000000000111, 0.2083333333333333426, 0.2166666666666666741, 0.2250000000000000056, 0.2333333333333333370, 0.2416666666666666685, 0.2500000000000000000, 0.2583333333333333592, 0.2666666666666666630, 0.2750000000000000222, 0.2833333333333333259, 0.2916666666666666852, 0.2999999999999999889, 0.3083333333333333481, 0.3166666666666666519, 0.3250000000000000111, 0.3333333333333333148, 0.3416666666666666741, 0.3499999999999999778, 0.3583333333333333370, 0.3666666666666666408, 0.3750000000000000000, 0.3833333333333333592, 0.3916666666666666630, 0.4000000000000000222, 0.4083333333333333259, 0.4166666666666666852, 0.4249999999999999889, 0.4333333333333333481, 0.4416666666666666519, 0.4500000000000000111, 0.4583333333333333148, 0.4666666666666666741, 0.4749999999999999778, 0.4833333333333333370, 0.4916666666666666408, 0.5000000000000000000, 0.5083333333333333037, 0.5166666666666667185, 0.5250000000000000222, 0.5333333333333333259, 0.5416666666666666297, 0.5500000000000000444, 0.5583333333333333481, 0.5666666666666666519, 0.5749999999999999556, 0.5833333333333333703, 0.5916666666666666741, 0.5999999999999999778, 0.6083333333333332815, 0.6166666666666666963, 0.6250000000000000000, 0.6333333333333333037, 0.6416666666666667185, 0.6500000000000000222, 0.6583333333333333259, 0.6666666666666666297, 0.6750000000000000444, 0.6833333333333333481, 0.6916666666666666519, 0.6999999999999999556, 0.7083333333333333703, 0.7166666666666666741, 0.7249999999999999778, 0.7333333333333332815, 0.7416666666666666963, 0.7500000000000000000, 0.7583333333333333037, 0.7666666666666667185, 0.7750000000000000222, 0.7833333333333333259, 0.7916666666666666297, 0.8000000000000000444, 0.8083333333333333481, 0.8166666666666666519, 0.8249999999999999556, 0.8333333333333333703, 0.8416666666666666741, 0.8499999999999999778, 0.8583333333333332815, 0.8666666666666666963, 0.8750000000000000000, 0.8833333333333333037, 0.8916666666666667185, 0.9000000000000000222, 0.9083333333333333259, 0.9166666666666666297, 0.9250000000000000444, 0.9333333333333333481, 0.9416666666666666519, 0.9499999999999999556, 0.9583333333333333703, 0.9666666666666666741, 0.9749999999999999778, 0.9833333333333332815, 0.9916666666666666963, 1.000000000000000000 ),
 .UNSPECIFIED. ) 
 GEOMETRIC_REPRESENTATION_ITEM ( )  RATIONAL_B_SPLINE_SURFACE ( (
 ( 1.000000000000000000, 0.8660254037844387076, 1.000000000000000000, 0.8660254037844387076, 1.000000000000000000, 0.8660254037844387076, 1.000000000000000000, 0.8660254037844387076, 1.000000000000000000, 0.8660254037844387076, 1.000000000000000000, 0.8660254037844387076, 1.000000000000000000, 0.8660254037844387076, 1.000000000000000000, 0.8660254037844387076, 1.000000000000000000, 0.8660254037844387076, 1.000000000000000000, 0.8660254037844387076, 1.000000000000000000, 0.8660254037844387076, 1.000000000000000000, 0.8660254037844387076, 1.000000000000000000, 0.8660254037844387076, 1.000000000000000000, 0.8660254037844387076, 1.000000000000000000, 0.8660254037844387076, 1.000000000000000000, 0.8660254037844387076, 1.000000000000000000, 0.8660254037844387076, 1.000000000000000000, 0.8660254037844387076, 1.000000000000000000, 0.8660254037844387076, 1.000000000000000000, 0.8660254037844387076, 1.000000000000000000, 0.8660254037844387076, 1.000000000000000000, 0.8660254037844387076, 1.000000000000000000, 0.8660254037844387076, 1.000000000000000000, 0.8660254037844387076, 1.000000000000000000, 0.8660254037844387076, 1.000000000000000000, 0.8660254037844387076, 1.000000000000000000, 0.8660254037844387076, 1.000000000000000000, 0.8660254037844387076, 1.000000000000000000, 0.8660254037844387076, 1.000000000000000000, 0.8660254037844387076, 1.000000000000000000, 0.8660254037844387076, 1.000000000000000000, 0.8660254037844387076, 1.000000000000000000, 0.8660254037844387076, 1.000000000000000000, 0.8660254037844387076, 1.000000000000000000, 0.8660254037844387076, 1.000000000000000000, 0.8660254037844387076, 1.000000000000000000, 0.8660254037844387076, 1.000000000000000000, 0.8660254037844387076, 1.000000000000000000, 0.8660254037844387076, 1.000000000000000000, 0.8660254037844387076, 1.000000000000000000, 0.8660254037844387076, 1.000000000000000000, 0.8660254037844387076, 1.000000000000000000, 0.8660254037844387076, 1.000000000000000000, 0.8660254037844387076, 1.000000000000000000, 0.8660254037844387076, 1.000000000000000000, 0.8660254037844387076, 1.000000000000000000, 0.8660254037844387076, 1.000000000000000000, 0.8660254037844387076, 1.000000000000000000, 0.8660254037844387076, 1.000000000000000000, 0.8660254037844387076, 1.000000000000000000, 0.8660254037844387076, 1.000000000000000000, 0.8660254037844387076, 1.000000000000000000, 0.8660254037844387076, 1.000000000000000000, 0.8660254037844387076, 1.000000000000000000, 0.8660254037844387076, 1.000000000000000000, 0.8660254037844387076, 1.000000000000000000, 0.8660254037844387076, 1.000000000000000000, 0.8660254037844387076, 1.000000000000000000, 0.8660254037844387076, 1.000000000000000000, 0.8660254037844387076, 1.000000000000000000, 0.8660254037844387076, 1.000000000000000000, 0.8660254037844387076, 1.000000000000000000, 0.8660254037844387076, 1.000000000000000000, 0.8660254037844387076, 1.000000000000000000, 0.8660254037844387076, 1.000000000000000000, 0.8660254037844387076, 1.000000000000000000, 0.8660254037844387076, 1.000000000000000000, 0.8660254037844387076, 1.000000000000000000, 0.8660254037844387076, 1.000000000000000000, 0.8660254037844387076, 1.000000000000000000, 0.8660254037844387076, 1.000000000000000000, 0.8660254037844387076, 1.000000000000000000, 0.8660254037844387076, 1.000000000000000000, 0.8660254037844387076, 1.000000000000000000, 0.8660254037844387076, 1.000000000000000000, 0.8660254037844387076, 1.000000000000000000, 0.8660254037844387076, 1.000000000000000000, 0.8660254037844387076, 1.000000000000000000, 0.8660254037844387076, 1.000000000000000000, 0.8660254037844387076, 1.000000000000000000, 0.8660254037844387076, 1.000000000000000000, 0.8660254037844387076, 1.000000000000000000, 0.8660254037844387076, 1.000000000000000000, 0.8660254037844387076, 1.000000000000000000, 0.8660254037844387076, 1.000000000000000000, 0.8660254037844387076, 1.000000000000000000, 0.8660254037844387076, 1.000000000000000000, 0.8660254037844387076, 1.000000000000000000, 0.8660254037844387076, 1.000000000000000000, 0.8660254037844387076, 1.000000000000000000, 0.8660254037844387076, 1.000000000000000000, 0.8660254037844387076, 1.000000000000000000, 0.8660254037844387076, 1.000000000000000000, 0.8660254037844387076, 1.000000000000000000, 0.8660254037844387076, 1.000000000000000000, 0.8660254037844387076, 1.000000000000000000, 0.8660254037844387076, 1.000000000000000000, 0.8660254037844387076, 1.000000000000000000, 0.8660254037844387076, 1.000000000000000000, 0.8660254037844387076, 1.000000000000000000, 0.8660254037844387076, 1.000000000000000000, 0.8660254037844387076, 1.000000000000000000, 0.8660254037844387076, 1.000000000000000000, 0.8660254037844387076, 1.000000000000000000, 0.8660254037844387076, 1.000000000000000000, 0.8660254037844387076, 1.000000000000000000, 0.8660254037844387076, 1.000000000000000000, 0.8660254037844387076, 1.000000000000000000, 0.8660254037844387076, 1.000000000000000000, 0.8660254037844387076, 1.000000000000000000, 0.8660254037844387076, 1.000000000000000000, 0.8660254037844387076, 1.000000000000000000, 0.8660254037844387076, 1.000000000000000000, 0.8660254037844387076, 1.000000000000000000, 0.8660254037844387076, 1.000000000000000000, 0.8660254037844387076, 1.000000000000000000, 0.8660254037844387076, 1.000000000000000000, 0.8660254037844387076, 1.000000000000000000, 0.8660254037844387076, 1.000000000000000000, 0.8660254037844387076, 1.000000000000000000),
 ( 1.000000000000000000, 0.8660254037844387076, 1.000000000000000000, 0.8660254037844387076, 1.000000000000000000, 0.8660254037844387076, 1.000000000000000000, 0.8660254037844387076, 1.000000000000000000, 0.8660254037844387076, 1.000000000000000000, 0.8660254037844387076, 1.000000000000000000, 0.8660254037844387076, 1.000000000000000000, 0.8660254037844387076, 1.000000000000000000, 0.8660254037844387076, 1.000000000000000000, 0.8660254037844387076, 1.000000000000000000, 0.8660254037844387076, 1.000000000000000000, 0.8660254037844387076, 1.000000000000000000, 0.8660254037844387076, 1.000000000000000000, 0.8660254037844387076, 1.000000000000000000, 0.8660254037844387076, 1.000000000000000000, 0.8660254037844387076, 1.000000000000000000, 0.8660254037844387076, 1.000000000000000000, 0.8660254037844387076, 1.000000000000000000, 0.8660254037844387076, 1.000000000000000000, 0.8660254037844387076, 1.000000000000000000, 0.8660254037844387076, 1.000000000000000000, 0.8660254037844387076, 1.000000000000000000, 0.8660254037844387076, 1.000000000000000000, 0.8660254037844387076, 1.000000000000000000, 0.8660254037844387076, 1.000000000000000000, 0.8660254037844387076, 1.000000000000000000, 0.8660254037844387076, 1.000000000000000000, 0.8660254037844387076, 1.000000000000000000, 0.8660254037844387076, 1.000000000000000000, 0.8660254037844387076, 1.000000000000000000, 0.8660254037844387076, 1.000000000000000000, 0.8660254037844387076, 1.000000000000000000, 0.8660254037844387076, 1.000000000000000000, 0.8660254037844387076, 1.000000000000000000, 0.8660254037844387076, 1.000000000000000000, 0.8660254037844387076, 1.000000000000000000, 0.8660254037844387076, 1.000000000000000000, 0.8660254037844387076, 1.000000000000000000, 0.8660254037844387076, 1.000000000000000000, 0.8660254037844387076, 1.000000000000000000, 0.8660254037844387076, 1.000000000000000000, 0.8660254037844387076, 1.000000000000000000, 0.8660254037844387076, 1.000000000000000000, 0.8660254037844387076, 1.000000000000000000, 0.8660254037844387076, 1.000000000000000000, 0.8660254037844387076, 1.000000000000000000, 0.8660254037844387076, 1.000000000000000000, 0.8660254037844387076, 1.000000000000000000, 0.8660254037844387076, 1.000000000000000000, 0.8660254037844387076, 1.000000000000000000, 0.8660254037844387076, 1.000000000000000000, 0.8660254037844387076, 1.000000000000000000, 0.8660254037844387076, 1.000000000000000000, 0.8660254037844387076, 1.000000000000000000, 0.8660254037844387076, 1.000000000000000000, 0.8660254037844387076, 1.000000000000000000, 0.8660254037844387076, 1.000000000000000000, 0.8660254037844387076, 1.000000000000000000, 0.8660254037844387076, 1.000000000000000000, 0.8660254037844387076, 1.000000000000000000, 0.8660254037844387076, 1.000000000000000000, 0.8660254037844387076, 1.000000000000000000, 0.8660254037844387076, 1.000000000000000000, 0.8660254037844387076, 1.000000000000000000, 0.8660254037844387076, 1.000000000000000000, 0.8660254037844387076, 1.000000000000000000, 0.8660254037844387076, 1.000000000000000000, 0.8660254037844387076, 1.000000000000000000, 0.8660254037844387076, 1.000000000000000000, 0.8660254037844387076, 1.000000000000000000, 0.8660254037844387076, 1.000000000000000000, 0.8660254037844387076, 1.000000000000000000, 0.8660254037844387076, 1.000000000000000000, 0.8660254037844387076, 1.000000000000000000, 0.8660254037844387076, 1.000000000000000000, 0.8660254037844387076, 1.000000000000000000, 0.8660254037844387076, 1.000000000000000000, 0.8660254037844387076, 1.000000000000000000, 0.8660254037844387076, 1.000000000000000000, 0.8660254037844387076, 1.000000000000000000, 0.8660254037844387076, 1.000000000000000000, 0.8660254037844387076, 1.000000000000000000, 0.8660254037844387076, 1.000000000000000000, 0.8660254037844387076, 1.000000000000000000, 0.8660254037844387076, 1.000000000000000000, 0.8660254037844387076, 1.000000000000000000, 0.8660254037844387076, 1.000000000000000000, 0.8660254037844387076, 1.000000000000000000, 0.8660254037844387076, 1.000000000000000000, 0.8660254037844387076, 1.000000000000000000, 0.8660254037844387076, 1.000000000000000000, 0.8660254037844387076, 1.000000000000000000, 0.8660254037844387076, 1.000000000000000000, 0.8660254037844387076, 1.000000000000000000, 0.8660254037844387076, 1.000000000000000000, 0.8660254037844387076, 1.000000000000000000, 0.8660254037844387076, 1.000000000000000000, 0.8660254037844387076, 1.000000000000000000, 0.8660254037844387076, 1.000000000000000000, 0.8660254037844387076, 1.000000000000000000, 0.8660254037844387076, 1.000000000000000000, 0.8660254037844387076, 1.000000000000000000, 0.8660254037844387076, 1.000000000000000000, 0.8660254037844387076, 1.000000000000000000, 0.8660254037844387076, 1.000000000000000000, 0.8660254037844387076, 1.000000000000000000, 0.8660254037844387076, 1.000000000000000000, 0.8660254037844387076, 1.000000000000000000, 0.8660254037844387076, 1.000000000000000000, 0.8660254037844387076, 1.000000000000000000, 0.8660254037844387076, 1.000000000000000000, 0.8660254037844387076, 1.000000000000000000, 0.8660254037844387076, 1.000000000000000000, 0.8660254037844387076, 1.000000000000000000, 0.8660254037844387076, 1.000000000000000000, 0.8660254037844387076, 1.000000000000000000, 0.8660254037844387076, 1.000000000000000000, 0.8660254037844387076, 1.000000000000000000, 0.8660254037844387076, 1.000000000000000000, 0.8660254037844387076, 1.000000000000000000) ) ) 
 REPRESENTATION_ITEM ( '' )  SURFACE ( )  );
#88394=CARTESIAN_POINT ( 'NONE',  ( 5.052321652499934146, 4.905166280363509657, 0.2868986031296373862 ) ) ;
#88397=CARTESIAN_POINT ( 'NONE',  ( -4.981227357108504172, 4.889801201946265330, -0.2148083726750001365 ) ) ;
#88405=CARTESIAN_POINT ( 'NONE',  ( 6.073126464278658432, 6.050012061272033392, 0.000000000000000000 ) ) ;
#88424=CARTESIAN_POINT ( 'NONE',  ( 4.472210567661338843, 6.310941310395290493, 1.599625672291261402 ) ) ;
#88431=CARTESIAN_POINT ( 'NONE',  ( -6.237633190739009237, 9.434933268240943249, 1.199719254218452047 ) ) ;
#88436=CARTESIAN_POINT ( 'NONE',  ( 5.574337433874081427, 6.532423756721743580, -1.199719254218452047 ) ) ;
#88450=CARTESIAN_POINT ( 'NONE',  ( 5.709392085130549077, 9.675058176045386205, 0.000000000000000000 ) ) ;
#88451=CARTESIAN_POINT ( 'NONE',  ( -5.316205630334276400, 5.374863788244313767, -0.7216878364870338292 ) ) ;
#88452=CARTESIAN_POINT ( 'NONE',  ( -4.437261413422502798, 8.398831758960053406, 0.000000000000000000 ) ) ;
#88464=CARTESIAN_POINT ( 'NONE',  ( 5.041653019435334393, 6.975290837464928728, -1.599625672291269396 ) ) ;
#88465=CARTESIAN_POINT ( 'NONE',  ( 6.249382461256315580, 6.255644057745969988, -0.7998128361456481317 ) ) ;
#88483=CARTESIAN_POINT ( 'NONE',  ( 5.646014316602349759, 7.456765758048159221, -1.329534273556526758 ) ) ;
#88484=DIRECTION ( 'NONE',  ( -0.6095094443613831015, -1.732612801327082678E-12, 0.7927788072560203458 ) ) ;
#88485=ORIENTED_EDGE ( 'NONE', *, *, #181214, .F. ) ;
#88492=CARTESIAN_POINT ( 'NONE',  ( 3.562760505341037831, 7.378580699531681830, -1.734723475976807094E-15 ) ) ;
#88496=CARTESIAN_POINT ( 'NONE',  ( 5.806634928402749196, 9.996434193103704402, -0.7998128361456481317 ) ) ;
#88501=CARTESIAN_POINT ( 'NONE',  ( 6.861835142292147083, 7.178098218861903135, 0.7216878364870328300 ) ) ;
#88504=CARTESIAN_POINT ( 'NONE',  ( -6.330731382938325602, 6.350551133041632212, 0.7998128361456281477 ) ) ;
#88506=CARTESIAN_POINT ( 'NONE',  ( 7.851580356089786328, 8.332800968292465527, 0.000000000000000000 ) ) ;
#88514=CARTESIAN_POINT ( 'NONE',  ( -5.055603177353559019, 6.862042912877393874, -1.261393572340614666 ) ) ;
#88517=CARTESIAN_POINT ( 'NONE',  ( 6.229241538080760421, 6.920885192246182704, -0.8282608007674150397 ) ) ;
#88518=CARTESIAN_POINT ( 'NONE',  ( -6.861835142292179057, 9.098836647464588978, 1.443375672974064550 ) ) ;
#88534=CARTESIAN_POINT ( 'NONE',  ( 0.3999999999999758193, 2.999999999999999112, 7.500000000000000000 ) ) ;
#88552=CARTESIAN_POINT ( 'NONE',  ( 5.820193082016415609, 10.01225203898631655, 0.000000000000000000 ) ) ;
#88554=CARTESIAN_POINT ( 'NONE',  ( 5.580062740476173566, 8.667767742934335828, 1.199719254218451159 ) ) ;
#88570=CARTESIAN_POINT ( 'NONE',  ( -3.610214042988883598, 7.433943160120816351, 0.7998128361456352531 ) ) ;
#88572=CARTESIAN_POINT ( 'NONE',  ( 6.170369307550823912, 7.331757292631694511, 1.082531754730549967 ) ) ;
#88581=CARTESIAN_POINT ( 'NONE',  ( -3.949167883330528372, 7.829389307186077396, 1.214306433183764966E-14 ) ) ;
#88584=CARTESIAN_POINT ( 'NONE',  ( -4.502716413514313842, 5.386162249589033557, -1.082531754730549967 ) ) ;
#88588=CARTESIAN_POINT ( 'NONE',  ( -4.995253251992230581, 4.792493313604505367, 0.000000000000000000 ) ) ;
#88612=VECTOR ( 'NONE', #152947, 1000.000000000000000 ) ;
#88613=CARTESIAN_POINT ( 'NONE',  ( -4.630991987519598396, 7.560518531151607213, 1.199719254218452935 ) ) ;
#88624=CARTESIAN_POINT ( 'NONE',  ( -6.392190997713585787, 6.905894197498253284, -0.8087526810517248199 ) ) ;
#88627=ORIENTED_EDGE ( 'NONE', *, *, #92114, .F. ) ;
#88634=CARTESIAN_POINT ( 'NONE',  ( -1.854512760316423536, 9.001999999999998892, 2.484105960264900936 ) ) ;
#88637=CARTESIAN_POINT ( 'NONE',  ( -6.414942957921379474, 7.513130201443591005, -1.199719254218452047 ) ) ;
#88638=CARTESIAN_POINT ( 'NONE',  ( 5.293864907607461312, 4.747529046662108954, 2.500000000000000444 ) ) ;
#88645=CARTESIAN_POINT ( 'NONE',  ( 6.333067150914805765, 9.442309871825708356, 1.082531754730549967 ) ) ;
#88656=CARTESIAN_POINT ( 'NONE',  ( 3.725458348705031231, 7.568394850123006279, -1.734723475976807094E-15 ) ) ;
#88664=CARTESIAN_POINT ( 'NONE',  ( 6.282224075085741433, 8.422623735723785643, 1.599625672291268286 ) ) ;
#88666=CARTESIAN_POINT ( 'NONE',  ( 5.448397627845284141, 7.449826213943242514, 1.599625672291268286 ) ) ;
#88673=B_SPLINE_CURVE_WITH_KNOTS ( 'NONE', 3,
 ( #184346, #4505, #70576, #173471 ),
 .UNSPECIFIED., .F., .F.,
 ( 4, 4 ),
 ( 0.0006426233018256924130, 0.0009180112871920716004 ),
 .UNSPECIFIED. ) ;
#88680=CARTESIAN_POINT ( 'NONE',  ( 6.385878362533466301, 6.816559200039058020, 0.5486352003098924346 ) ) ;
#88682=CARTESIAN_POINT ( 'NONE',  ( 4.245111494854632461, 7.966730820723463502, 0.000000000000000000 ) ) ;
#88689=CARTESIAN_POINT ( 'NONE',  ( -2.810282979782591006, 6.500690253046801814, 0.000000000000000000 ) ) ;
#88695=CARTESIAN_POINT ( 'NONE',  ( 0.000000000000000000, 3.480000000000000426, -2.000000000000000000 ) ) ;
#88700=CARTESIAN_POINT ( 'NONE',  ( -4.787437638956927977, 7.639075441208117212, -1.082531754730549967 ) ) ;
#88706=CARTESIAN_POINT ( 'NONE',  ( 5.830888582329017744, 8.960397891762626799, -1.199719254218452047 ) ) ;
#88712=EDGE_CURVE ( 'NONE', #61752, #44, #47888, .T. ) ;
#88741=ORIENTED_EDGE ( 'NONE', *, *, #4565, .F. ) ;
#88755=CARTESIAN_POINT ( 'NONE',  ( 5.398914348987510436, 6.259949555863199677, -2.500000000000000444 ) ) ;
#88764=ORIENTED_EDGE ( 'NONE', *, *, #165266, .F. ) ;
#88765=CARTESIAN_POINT ( 'NONE',  ( 3.770576118376296471, 7.413106214832098750, 0.7216878364870257245 ) ) ;
#88775=CARTESIAN_POINT ( 'NONE',  ( -4.258669648468323743, 6.061810238003387141, 1.443375672974065660 ) ) ;
#88785=CARTESIAN_POINT ( 'NONE',  ( 6.183927461164522299, 6.387205924212962849, 0.000000000000000000 ) ) ;
#88805=CARTESIAN_POINT ( 'NONE',  ( 7.024532985656128936, 9.288650798055913427, 1.443375672974065660 ) ) ;
#88807=EDGE_CURVE ( 'NONE', #206426, #113379, #178435, .T. ) ;
#88819=CARTESIAN_POINT ( 'NONE',  ( -6.455090533882213322, 6.703562842383589349, -0.7216878364870338292 ) ) ;
#88824=CARTESIAN_POINT ( 'NONE',  ( 8.039058738260216330, 8.343599714250547805, -0.7998128361456341429 ) ) ;
#88829=CARTESIAN_POINT ( 'NONE',  ( -3.820365424000704557, 7.679119771301277098, -0.7998128361456481317 ) ) ;
#88841=DIRECTION ( 'NONE',  ( 0.000000000000000000, 0.000000000000000000, -1.000000000000000000 ) ) ;
#88854=EDGE_CURVE ( 'NONE', #81797, #68330, #107380, .T. ) ;
#88869=CARTESIAN_POINT ( 'NONE',  ( 4.800995793014950941, 5.734154859006458160, -1.082531754730548412 ) ) ;
#88873=CARTESIAN_POINT ( 'NONE',  ( -5.986807348886189040, 9.142303119412650503, -1.199719254218452047 ) ) ;
#88877=CARTESIAN_POINT ( 'NONE',  ( -6.947627372360122955, 7.070263120700404968, 0.000000000000000000 ) ) ;
#88882=CARTESIAN_POINT ( 'NONE',  ( -6.360183458142173230, 9.473945563590925545, 1.082531754730549967 ) ) ;
#88883=CARTESIAN_POINT ( 'NONE',  ( 7.960045584554727327, 8.459343734834927631, 0.7216878364870267237 ) ) ;
#88889=CARTESIAN_POINT ( 'NONE',  ( -5.340986169140711226, 5.195848383611072485, 0.000000000000000000 ) ) ;
#88894=CARTESIAN_POINT ( 'NONE',  ( -1.877679919396925134, 2.480539018720154143, 2.466641060286964837 ) ) ;
#88896=CARTESIAN_POINT ( 'NONE',  ( -6.526270840131767059, 8.707344961610770540, -1.599625672291271394 ) ) ;
#88898=CARTESIAN_POINT ( 'NONE',  ( 4.669458948634179762, 8.398658883068243597, -0.5498995856093937817 ) ) ;
#88901=FACE_OUTER_BOUND ( 'NONE', #92384, .T. ) ;
#88903=CARTESIAN_POINT ( 'NONE',  ( 5.246079093845007257, 5.085123462432798114, 0.7998128361456352531 ) ) ;
#88913=CARTESIAN_POINT ( 'NONE',  ( -7.774674742793745708, 8.035151719539642912, 0.7998128361456341429 ) ) ;
#88916=CARTESIAN_POINT ( 'NONE',  ( 2.947061413272269004, 6.452339058877361921, 0.1880404715405617766 ) ) ;
#88926=CARTESIAN_POINT ( 'NONE',  ( 4.085803189671889157, 5.860132702740892263, -1.599625672291273171 ) ) ;
#88941=CARTESIAN_POINT ( 'NONE',  ( 6.104935607482663507, 7.108274908414393245, 1.121150977946131722 ) ) ;
#88947=CARTESIAN_POINT ( 'NONE',  ( -5.600330155773479035, 5.743136491903856999, -0.2604917703057018641 ) ) ;
#88953=ORIENTED_EDGE ( 'NONE', *, *, #201515, .T. ) ;
#88968=CARTESIAN_POINT ( 'NONE',  ( -6.596192096975760144, 6.770415987340496322, 0.2575442448356154990 ) ) ;
#88988=CARTESIAN_POINT ( 'NONE',  ( -6.642568916052639771, 6.714361588341672515, 0.000000000000000000 ) ) ;
#89005=CARTESIAN_POINT ( 'NONE',  ( 4.869313445963426190, 5.709895770826003414, 1.199719254218452935 ) ) ;
#89017=CARTESIAN_POINT ( 'NONE',  ( -6.329400247113886380, 6.896658009377570231, 0.7645970852754442326 ) ) ;
#89024=CARTESIAN_POINT ( 'NONE',  ( 5.855142236255289845, 7.924361590421551860, -1.599625672291281386 ) ) ;
#89032=ORIENTED_EDGE ( 'NONE', *, *, #155084, .T. ) ;
#89034=CARTESIAN_POINT ( 'NONE',  ( -3.806807270387036368, 7.663301925418665839, 0.000000000000000000 ) ) ;
#89036=CARTESIAN_POINT ( 'NONE',  ( 4.278479993564246797, 7.149254538203735798, 1.199719254218452047 ) ) ;
#89039=CARTESIAN_POINT ( 'NONE',  ( -4.423703259808839938, 8.383013913077441259, 0.7998128361456352531 ) ) ;
#89042=CARTESIAN_POINT ( 'NONE',  ( 5.352436782344940802, 9.466536356036257871, 0.000000000000000000 ) ) ;
#89048=CARTESIAN_POINT ( 'NONE',  ( -5.468737822882341781, 7.600800700804905219, 1.347914668206271038 ) ) ;
#89058=CARTESIAN_POINT ( 'NONE',  ( -5.275531169048911728, 6.287779464379406491, -1.082531754730549967 ) ) ;
#89067=CARTESIAN_POINT ( 'NONE',  ( 4.909461021924256485, 4.900328411765999981, 0.7216878364870338292 ) ) ;
#89072=CARTESIAN_POINT ( 'NONE',  ( -6.424584688029276514, 8.588711117491191871, 1.599625672291269396 ) ) ;
#89087=CARTESIAN_POINT ( 'NONE',  ( 3.923105346307896202, 5.670318552149568703, -1.599625672291269396 ) ) ;
#89113=CARTESIAN_POINT ( 'NONE',  ( -5.655159470675923394, 5.770309935309573923, 0.000000000000000000 ) ) ;
#89137=ORIENTED_EDGE ( 'NONE', *, *, #56512, .F. ) ;
#89138=CARTESIAN_POINT ( 'NONE',  ( -6.257970421159510188, 9.458660037064859694, 1.199719254218452047 ) ) ;
#89144=CARTESIAN_POINT ( 'NONE',  ( -5.307090785106547415, 5.156303768904543894, -0.7998128361456362523 ) ) ;
#89153=CARTESIAN_POINT ( 'NONE',  ( -5.887983850084758330, 10.09134126839936840, 0.7998128361456291469 ) ) ;
#89155=CARTESIAN_POINT ( 'NONE',  ( 6.505076094845553492, 6.832456077006010098, -0.5564590407885674495 ) ) ;
#89159=CARTESIAN_POINT ( 'NONE',  ( 5.740951700743842423, 5.662474837148078421, -0.7998128361456481317 ) ) ;
#89164=CARTESIAN_POINT ( 'NONE',  ( -6.505933609711270549, 8.683618192786854095, -1.599625672291271394 ) ) ;
#89167=B_SPLINE_CURVE_WITH_KNOTS ( 'NONE', 3,
 ( #116096, #166935, #69397, #119303, #134463, #18528, #164792, #84605, #117169, #99795 ),
 .UNSPECIFIED., .F., .F.,
 ( 4, 3, 3, 4 ),
 ( 3.757351081995909416E-18, 3.125177024600283269E-05, 5.801553290628923905E-05, 8.478882652531181735E-05 ),
 .UNSPECIFIED. ) ;
#89169=CARTESIAN_POINT ( 'NONE',  ( -5.157951095356222204, 4.982307464195829816, 0.000000000000000000 ) ) ;
#89173=CARTESIAN_POINT ( 'NONE',  ( 4.245111494854632461, 7.966730820723463502, 0.000000000000000000 ) ) ;
#89174=CARTESIAN_POINT ( 'NONE',  ( 5.058600711230250013, 5.074324715956299414, -0.7216878364870458196 ) ) ;
#89175=CARTESIAN_POINT ( 'NONE',  ( -4.272227801637618505, 7.998366511970260717, 0.7216878364870338292 ) ) ;
#89182=CARTESIAN_POINT ( 'NONE',  ( 4.716257332707354699, 6.595662536282280719, -1.599625672291269396 ) ) ;
#89183=ORIENTED_EDGE ( 'NONE', *, *, #52019, .T. ) ;
#89194=CARTESIAN_POINT ( 'NONE',  ( 4.817101577040221905, 8.228953320636518853, 0.8951067572735508238 ) ) ;
#89202=CARTESIAN_POINT ( 'NONE',  ( 4.850785098639300408, 8.881276058379668825, -0.7998128361456481317 ) ) ;
#89213=CARTESIAN_POINT ( 'NONE',  ( 5.614387949662905442, 7.370906683214474953, 1.237392280610301931 ) ) ;
#89231=CARTESIAN_POINT ( 'NONE',  ( -8.120407659942227241, 8.438506789546210030, 0.7998128361456341429 ) ) ;
#89244=CARTESIAN_POINT ( 'NONE',  ( 5.200434439293556643, 8.224868058221247225, -1.199719254218452047 ) ) ;
#89251=VERTEX_POINT ( 'NONE', #95145 ) ;
#89252=CARTESIAN_POINT ( 'NONE',  ( 3.528865121306874464, 7.339036084825155015, -0.7998128361456362523 ) ) ;
#89256=CARTESIAN_POINT ( 'NONE',  ( 5.546694241322223107, 5.643767167730274537, -0.7216878364870458196 ) ) ;
#89271=CARTESIAN_POINT ( 'NONE',  ( -3.363304624641834106, 6.081549941127532222, -1.199719254218452047 ) ) ;
#89272=CARTESIAN_POINT ( 'NONE',  ( 7.187230829020130329, 7.557726520044554697, 0.7216878364870267237 ) ) ;
#89283=CARTESIAN_POINT ( 'NONE',  ( -4.586401103172829785, 8.572828063668767484, 0.7998128361456281477 ) ) ;
#89284=CARTESIAN_POINT ( 'NONE',  ( -3.447516199624892419, 7.244129009529488350, 0.7998128361456352531 ) ) ;
#89286=CARTESIAN_POINT ( 'NONE',  ( 4.678972410047582464, 8.472901888448573615, -0.7216878364870357165 ) ) ;
#89292=CARTESIAN_POINT ( 'NONE',  ( -5.721691974912406664, 7.393287073457107894, 1.332251608056257641 ) ) ;
#89296=CARTESIAN_POINT ( 'NONE',  ( -4.940673843451318881, 7.995311821131723562, 1.007273293859496155 ) ) ;
#89300=CARTESIAN_POINT ( 'NONE',  ( 5.234856708652233515, 6.240325927249993576, 1.082531754730549078 ) ) ;
#89304=CARTESIAN_POINT ( 'NONE',  ( -6.363572996767778100, 8.517530811019446091, -1.599625672291271394 ) ) ;
#89318=CARTESIAN_POINT ( 'NONE',  ( 5.879395890181562834, 6.888325289080478697, -1.199719254218452047 ) ) ;
#89354=CARTESIAN_POINT ( 'NONE',  ( 5.560252395380206103, 8.540692657035327429, 1.082531754730547524 ) ) ;
#89360=CARTESIAN_POINT ( 'NONE',  ( 7.065207446052794715, 9.336104335185329006, -1.443375672974064550 ) ) ;
#89384=CARTESIAN_POINT ( 'NONE',  ( -4.787964524281469458, 5.614988695530339413, -1.199719254218453823 ) ) ;
#89386=CARTESIAN_POINT ( 'NONE',  ( 4.190878879955609371, 7.903459436674603822, -0.7216878364870338292 ) ) ;
#89393=CARTESIAN_POINT ( 'NONE',  ( -3.169574050544739841, 6.919863168935977527, -0.7998128361456481317 ) ) ;
#89397=FACE_OUTER_BOUND ( 'NONE', #91138, .T. ) ;
#89398=CARTESIAN_POINT ( 'NONE',  ( -5.465345320084574965, 9.390336950158399532, 0.000000000000000000 ) ) ;
#89401=CARTESIAN_POINT ( 'NONE',  ( -6.064239847062411926, 10.29697326487330500, 0.000000000000000000 ) ) ;
#89406=CARTESIAN_POINT ( 'NONE',  ( -4.716257332707368910, 6.595662536282280719, -1.599625672291271394 ) ) ;
#89409=CIRCLE ( 'NONE', #20251, 0.8300000000000008482 ) ;
#89415=DIRECTION ( 'NONE',  ( 0.000000000000000000, 0.000000000000000000, 1.000000000000000000 ) ) ;
#89420=CARTESIAN_POINT ( 'NONE',  ( -5.153507786970275006, 7.105788066255672497, -1.443375672974066548 ) ) ;
#89422=CARTESIAN_POINT ( 'NONE',  ( -3.784134271545645412, 7.428924060196286483, 0.7216878364870338292 ) ) ;
#89423=CARTESIAN_POINT ( 'NONE',  ( 5.468734858265785093, 7.473552982767158070, 1.599625672291269396 ) ) ;
#89424=CARTESIAN_POINT ( 'NONE',  ( -5.281783360975562225, 8.319775133516907673, 1.199719254218452935 ) ) ;
#89425=CARTESIAN_POINT ( 'NONE',  ( -6.688968683495758683, 8.897159112202094988, -1.599625672291271394 ) ) ;
#89437=ORIENTED_EDGE ( 'NONE', *, *, #58668, .T. ) ;
#89444=CARTESIAN_POINT ( 'NONE',  ( 5.664274315459256748, 9.830346811336296398, -0.7998128361456481317 ) ) ;
#89476=CARTESIAN_POINT ( 'NONE',  ( 3.002403234314147351, 6.387006324390887002, -0.4858955912513076569 ) ) ;
#89485=CARTESIAN_POINT ( 'NONE',  ( 5.357406976055401948, 6.279338222599979424, 1.199719254218452935 ) ) ;
#89488=CARTESIAN_POINT ( 'NONE',  ( -4.842197138736131556, 5.678260079060780008, 1.199719254218452935 ) ) ;
#89502=CARTESIAN_POINT ( 'NONE',  ( 5.727393547130178675, 5.646656991265468939, 0.000000000000000000 ) ) ;
#89509=CARTESIAN_POINT ( 'NONE',  ( -6.587282531393266360, 8.778525268082516320, 1.599625672291269396 ) ) ;
#89514=CARTESIAN_POINT ( 'NONE',  ( 6.412080304620304538, 6.445458208337293549, -0.7998128361456481317 ) ) ;
#89524=CARTESIAN_POINT ( 'NONE',  ( 6.753369913382843315, 8.011924666102361314, -1.082531754730548412 ) ) ;
#89526=CARTESIAN_POINT ( 'NONE',  ( -3.174017359375036929, 6.717120995997236221, 0.7216878364870338292 ) ) ;
#89527=CARTESIAN_POINT ( 'NONE',  ( -6.286140498591554326, 7.362860665558790707, 1.199719254218452047 ) ) ;
#89534=ORIENTED_EDGE ( 'NONE', *, *, #67920, .T. ) ;
#89539=CARTESIAN_POINT ( 'NONE',  ( 6.204791576909545192, 7.267953590263130259, -1.199719254218452047 ) ) ;
#89540=CARTESIAN_POINT ( 'NONE',  ( 5.387385936583818591, 7.378645907471495846, -1.599625672291283607 ) ) ;
#89543=CARTESIAN_POINT ( 'NONE',  ( 6.875920180786008196, 8.050936961452347163, -1.199719254218452047 ) ) ;
#89546=ORIENTED_EDGE ( 'NONE', *, *, #34251, .F. ) ;
#89551=DIRECTION ( 'NONE',  ( 1.000000000000000000, 0.000000000000000000, 0.000000000000000000 ) ) ;
#89558=CARTESIAN_POINT ( 'NONE',  ( 5.207906507908255378, 7.834591108650524660, -1.266300940072472736 ) ) ;
#89559=ORIENTED_EDGE ( 'NONE', *, *, #102451, .T. ) ;
#89562=CARTESIAN_POINT ( 'NONE',  ( 0.3944177863135505113, 2.931182615571563677, 2.025436609040003333 ) ) ;
#89563=CARTESIAN_POINT ( 'NONE',  ( 4.736594563127852098, 6.619389305106191834, -1.599625672291273171 ) ) ;
#89568=CARTESIAN_POINT ( 'NONE',  ( 3.549202351727371862, 7.362762853649070571, -0.7998128361456362523 ) ) ;
#89573=CARTESIAN_POINT ( 'NONE',  ( 6.749980374757213575, 8.968339418673846097, 1.599625672291268286 ) ) ;
#89577=CARTESIAN_POINT ( 'NONE',  ( 5.234856708652222856, 8.161064355852680308, 1.082531754730549078 ) ) ;
#89579=CARTESIAN_POINT ( 'NONE',  ( -5.119085517611572378, 8.129960982925583224, 1.199719254218452935 ) ) ;
#89581=CARTESIAN_POINT ( 'NONE',  ( 7.675324359112103423, 8.127168971818530707, 0.7216878364870267237 ) ) ;
#89588=CARTESIAN_POINT ( 'NONE',  ( -5.794181935090157332, 6.277560012370397402, -0.7153197263606870804 ) ) ;
#89592=CARTESIAN_POINT ( 'NONE',  ( -4.065465959251405081, 5.836405933916976707, -1.599625672291271394 ) ) ;
#89601=CARTESIAN_POINT ( 'NONE',  ( 0.2395129731749547353, 2.570475252693285029, -1.989112730403746587 ) ) ;
#89611=ORIENTED_EDGE ( 'NONE', *, *, #107594, .T. ) ;
#89621=CARTESIAN_POINT ( 'NONE',  ( 4.095971805104288599, 5.871996087412059140, 1.443375672974058777 ) ) ;
#89626=CARTESIAN_POINT ( 'NONE',  ( 6.318982112420993502, 9.529840343536603697, -1.199719254218452047 ) ) ;
#89628=CARTESIAN_POINT ( 'NONE',  ( 8.188198428010544205, 8.517596018959260107, 0.000000000000000000 ) ) ;
#89630=CARTESIAN_POINT ( 'NONE',  ( 3.719872605471109761, 6.605953636083950364, -2.500000000000002220 ) ) ;
#89640=CARTESIAN_POINT ( 'NONE',  ( -4.423703259808839938, 8.383013913077441259, 0.7998128361456352531 ) ) ;
#89642=CARTESIAN_POINT ( 'NONE',  ( 5.682275777458846377, 7.722684055159064975, 1.443375672974064550 ) ) ;
#89652=CARTESIAN_POINT ( 'NONE',  ( -3.461074353238556167, 7.259946855412102273, 0.000000000000000000 ) ) ;
#89655=CARTESIAN_POINT ( 'NONE',  ( 0.000000000000000000, 8.980740528189222971, 0.000000000000000000 ) ) ;
#89660=CARTESIAN_POINT ( 'NONE',  ( -4.981695098378565945, 4.776675467721892332, -0.7998128361456362523 ) ) ;
#89687=CARTESIAN_POINT ( 'NONE',  ( -4.899292406491858820, 6.809203455697518947, -1.599625672291271394 ) ) ;
#89688=CARTESIAN_POINT ( 'NONE',  ( -3.169574050544739841, 6.919863168935977527, -0.7998128361456481317 ) ) ;
#89700=CARTESIAN_POINT ( 'NONE',  ( -4.207966135563093957, 7.175396087857926375, -0.9899555337401829691 ) ) ;
#89714=CARTESIAN_POINT ( 'NONE',  ( -5.764151584465413869, 6.753873599078290546, -1.199719254218453823 ) ) ;
#89720=B_SPLINE_CURVE_WITH_KNOTS ( 'NONE', 3,
 ( #170814, #86364, #2947, #53870 ),
 .UNSPECIFIED., .F., .F.,
 ( 4, 4 ),
 ( 2.718386964177322303E-17, 0.0008010247897357521693 ),
 .UNSPECIFIED. ) ;
#89722=CARTESIAN_POINT ( 'NONE',  ( 8.122743427918724279, 8.649157885426255632, 0.7216878364870267237 ) ) ;
#89731=CARTESIAN_POINT ( 'NONE',  ( -5.960701852718076843, 6.182757358283963889, 0.3440389873682374589 ) ) ;
#89735=CARTESIAN_POINT ( 'NONE',  ( 3.901714345682657292, 7.774026846596938434, 0.7998128361456271485 ) ) ;
#89743=CARTESIAN_POINT ( 'NONE',  ( 5.501576472095266901, 9.640532660744973725, -0.7998128361456481317 ) ) ;
#89745=CARTESIAN_POINT ( 'NONE',  ( 6.530187263637528439, 7.647581891445782709, -1.199719254218452047 ) ) ;
#89759=CARTESIAN_POINT ( 'NONE',  ( 5.925280661667059690, 7.134359284303951831, -1.114000666120490868 ) ) ;
#89761=CARTESIAN_POINT ( 'NONE',  ( 5.234856708652222856, 8.161064355852680308, 1.082531754730549078 ) ) ;
#89780=CARTESIAN_POINT ( 'NONE',  ( -4.407809337774280856, 7.196175756495025055, 1.082531754730549967 ) ) ;
#89786=ADVANCED_FACE ( 'NONE', ( #194747 ), #105790, .T. ) ;
#89803=CARTESIAN_POINT ( 'NONE',  ( 4.667750024854814050, 8.667735138964429709, -0.7998128361456381397 ) ) ;
#89807=ORIENTED_EDGE ( 'NONE', *, *, #128175, .T. ) ;
#89813=CARTESIAN_POINT ( 'NONE',  ( 5.695833931072550094, 5.817763472438987726, 0.000000000000000000 ) ) ;
#89818=DIRECTION ( 'NONE',  ( -1.000000000000000000, 0.000000000000000000, 0.000000000000000000 ) ) ;
#89839=CARTESIAN_POINT ( 'NONE',  ( 4.909461021924244051, 6.821066840368686712, 1.443375672974065660 ) ) ;
#89840=ORIENTED_EDGE ( 'NONE', *, *, #117200, .T. ) ;
#89849=CARTESIAN_POINT ( 'NONE',  ( -4.177320726786328819, 5.966903162707725805, -1.443375672974066548 ) ) ;
#89854=DIRECTION ( 'NONE',  ( 0.7592566023653005702, -0.6507913734559639396, 0.000000000000000000 ) ) ;
#89880=CARTESIAN_POINT ( 'NONE',  ( 5.727393547130178675, 5.646656991265468939, 0.000000000000000000 ) ) ;
#89893=CARTESIAN_POINT ( 'NONE',  ( -5.139949633356594383, 9.010708648975750634, 0.000000000000000000 ) ) ;
#89896=CARTESIAN_POINT ( 'NONE',  ( 7.374709211190586089, 7.568525266002632534, 0.000000000000000000 ) ) ;
#89912=CARTESIAN_POINT ( 'NONE',  ( -5.017926250833627755, 5.026871178826882947, 0.7216878364870257245 ) ) ;
#89915=CARTESIAN_POINT ( 'NONE',  ( -4.370663978927107785, 5.060324124126027279, -2.420000000000000373 ) ) ;
#89943=CARTESIAN_POINT ( 'NONE',  ( -6.444921918449773024, 8.612437886315108315, 1.599625672291269396 ) ) ;
#89947=CARTESIAN_POINT ( 'NONE',  ( -5.261446130555064826, 8.296048364692991228, 1.199719254218452935 ) ) ;
#89952=CARTESIAN_POINT ( 'NONE',  ( -6.658462837642833421, 8.861568958707010779, 1.443375672974064550 ) ) ;
#89958=CARTESIAN_POINT ( 'NONE',  ( -3.817502770699643388, 6.611447778194983194, 1.199719254218452935 ) ) ;
#89965=CARTESIAN_POINT ( 'NONE',  ( -7.445362632559989535, 8.715286488521982733, 1.199719254218452047 ) ) ;
#89967=CARTESIAN_POINT ( 'NONE',  ( 5.213898493288036562, 7.712005038449616379, -1.200564631081424416 ) ) ;
#89970=CARTESIAN_POINT ( 'NONE',  ( 7.015401035077338143, 6.062865449010540253, 2.437084766375293476 ) ) ;
#89972=CARTESIAN_POINT ( 'NONE',  ( 4.004454267989866700, 5.765225627445230927, 1.599625672291262513 ) ) ;
#89981=CARTESIAN_POINT ( 'NONE',  ( -4.001066012398721838, 7.682011088333574378, -6.818990669119789124E-05 ) ) ;
#89994=CARTESIAN_POINT ( 'NONE',  ( 5.657495238652423097, 9.822437888394988548, 0.000000000000000000 ) ) ;
#90008=CARTESIAN_POINT ( 'NONE',  ( 5.770588788983777917, 7.358121641400980018, 1.301467365913897112 ) ) ;
#90009=CARTESIAN_POINT ( 'NONE',  ( -5.329763783503577379, 6.351050847909847086, 1.082531754730549078 ) ) ;
#90031=CARTESIAN_POINT ( 'NONE',  ( -5.019256313770280364, 7.854014895727056356, -1.116509978709074202 ) ) ;
#90035=CARTESIAN_POINT ( 'NONE',  ( 5.225741863424510747, 5.061396693608882558, 0.7998128361456352531 ) ) ;
#90055=CARTESIAN_POINT ( 'NONE',  ( -7.117104292530948229, 7.267986194233038155, -0.7998128361456362523 ) ) ;
#90062=CARTESIAN_POINT ( 'NONE',  ( 5.727393547130178675, 5.646656991265468939, 0.000000000000000000 ) ) ;
#90064=CARTESIAN_POINT ( 'NONE',  ( -3.147653791585729444, 8.920000000000001705, 2.419999999999999485 ) ) ;
#90070=CARTESIAN_POINT ( 'NONE',  ( 4.411198876399872404, 6.239761003923544713, -1.599625672291273171 ) ) ;
#90072=CARTESIAN_POINT ( 'NONE',  ( 7.065207446052794715, 9.336104335185329006, -1.443375672974064550 ) ) ;
#90079=CARTESIAN_POINT ( 'NONE',  ( 4.674980212565337467, 8.274328803998008297, 0.5478015097085631169 ) ) ;
#90082=CARTESIAN_POINT ( 'NONE',  ( 6.233692552841108458, 6.917895963632635592, 0.8214459722771473293 ) ) ;
#90084=CARTESIAN_POINT ( 'NONE',  ( -3.668686106071647579, 7.354262979464277095, -0.2566626154702719154 ) ) ;
#90099=CARTESIAN_POINT ( 'NONE',  ( -3.969505113751027547, 7.853116076009993840, 1.214306433183764966E-14 ) ) ;
#90101=CARTESIAN_POINT ( 'NONE',  ( 4.050854035433010480, 7.948023151305657841, 0.000000000000000000 ) ) ;
#90104=CARTESIAN_POINT ( 'NONE',  ( -6.459533842268148973, 6.500820668926428958, 0.000000000000000000 ) ) ;
#90108=CARTESIAN_POINT ( 'NONE',  ( 7.225569521440261767, 7.394528961293920233, -0.7998128361456341429 ) ) ;
#90113=CARTESIAN_POINT ( 'NONE',  ( -4.609429383499759503, 8.467968972964683871, -0.3232828671759068739 ) ) ;
#90122=CARTESIAN_POINT ( 'NONE',  ( -5.600926855776901192, 5.707038551260711579, -0.7216878364870338292 ) ) ;
#90132=CARTESIAN_POINT ( 'NONE',  ( 5.777182853198898904, 6.873039762554409293, -1.082531754730548412 ) ) ;
#90136=CARTESIAN_POINT ( 'NONE',  ( -6.587282531393266360, 8.778525268082516320, 1.599625672291269396 ) ) ;
#90150=CARTESIAN_POINT ( 'NONE',  ( 4.706615602599436343, 5.520081620234675412, 1.199719254218452935 ) ) ;
#90176=EDGE_CURVE ( 'NONE', #211530, #53040, #92263, .T. ) ;
#90179=CARTESIAN_POINT ( 'NONE',  ( 0.4917504562594980921, 10.46609003534429050, 2.500000000000000444 ) ) ;
#90181=CARTESIAN_POINT ( 'NONE',  ( -4.936577329151611515, 7.813071746435248599, 1.082531754730549967 ) ) ;
#90203=CARTESIAN_POINT ( 'NONE',  ( -5.112833325684928987, 5.137596099486740897, -0.7216878364870338292 ) ) ;
#90208=CARTESIAN_POINT ( 'NONE',  ( -3.637330350216213759, 7.465578851886037093, -0.7998128361456481317 ) ) ;
#90216=CARTESIAN_POINT ( 'NONE',  ( -7.587723245503481095, 8.881373870289390737, 1.199719254218452047 ) ) ;
#90218=CARTESIAN_POINT ( 'NONE',  ( 6.007156502879952953, 7.179297369210805080, -1.191424252104013037 ) ) ;
#90222=CARTESIAN_POINT ( 'NONE',  ( 6.229045230835819069, 6.231917288922055320, -0.7998128361456481317 ) ) ;
#90227=CARTESIAN_POINT ( 'NONE',  ( -7.435720902452096936, 7.639705572474380091, 0.000000000000000000 ) ) ;
#90230=CARTESIAN_POINT ( 'NONE',  ( -4.228163802615396705, 6.026220084508304708, -1.599625672291271394 ) ) ;
#90235=CARTESIAN_POINT ( 'NONE',  ( 4.692530563661249765, 8.488719734331187539, 0.000000000000000000 ) ) ;
#90236=CARTESIAN_POINT ( 'NONE',  ( -6.278834536460198734, 6.497930845391236332, 0.7216878364870257245 ) ) ;
#90242=CARTESIAN_POINT ( 'NONE',  ( 3.390420931869152721, 6.113185632892752075, -1.199719254218452047 ) ) ;
#90246=CARTESIAN_POINT ( 'NONE',  ( -4.490256990713600516, 8.252036901523048584, -0.03636953492806980354 ) ) ;
#90249=CARTESIAN_POINT ( 'NONE',  ( -1.854512760316423536, 2.488359591189891251, 2.484105960264900936 ) ) ;
#90253=CARTESIAN_POINT ( 'NONE',  ( 5.644368669187761256, 7.458116220610145675, 1.329639117314229235 ) ) ;
#90262=CARTESIAN_POINT ( 'NONE',  ( 6.873057527484919937, 6.983264968346048818, 0.7998128361456352531 ) ) ;
#90272=CARTESIAN_POINT ( 'NONE',  ( 6.457572779797339457, 6.769951385671206801, 0.3193968722623799494 ) ) ;
#90289=CARTESIAN_POINT ( 'NONE',  ( -6.957269102468015554, 8.145844036748005834, 1.199719254218452047 ) ) ;
#90294=CARTESIAN_POINT ( 'NONE',  ( -4.624346020613643304, 4.914118431181374369, -0.7231984802981470395 ) ) ;
#90301=CARTESIAN_POINT ( 'NONE',  ( 5.677832469072920496, 9.846164657218904992, 0.000000000000000000 ) ) ;
#90308=CARTESIAN_POINT ( 'NONE',  ( -7.444835747235459600, 8.818634805597074688, 1.082531754730549078 ) ) ;
#90310=CARTESIAN_POINT ( 'NONE',  ( 3.444653546323793947, 6.176457016423196222, 1.199719254218451159 ) ) ;
#90312=CARTESIAN_POINT ( 'NONE',  ( 5.383996397958233260, 5.453953017138946535, -0.7216878364870458196 ) ) ;
#90313=CARTESIAN_POINT ( 'NONE',  ( 5.608569151319391821, 5.681340981270094126, 0.4042273303749412960 ) ) ;
#90327=CARTESIAN_POINT ( 'NONE',  ( -5.953438850176548947, 9.959779401932374654, 0.000000000000000000 ) ) ;
#90328=CARTESIAN_POINT ( 'NONE',  ( 5.076602173674213070, 4.887400388900169368, 0.000000000000000000 ) ) ;
#90338=VERTEX_POINT ( 'NONE', #184885 ) ;
#90339=CARTESIAN_POINT ( 'NONE',  ( -6.123442655227560927, 7.173046514967467147, 1.199719254218452047 ) ) ;
#90340=CARTESIAN_POINT ( 'NONE',  ( -3.637330350216213759, 7.465578851886037093, -0.7998128361456481317 ) ) ;
#90342=CARTESIAN_POINT ( 'NONE',  ( 4.841670253411575864, 8.662716039039905169, -0.7216878364870458196 ) ) ;
#90356=CARTESIAN_POINT ( 'NONE',  ( -4.695470500997839025, 8.269974592382618894, -0.5850018098894956831 ) ) ;
#90358=CARTESIAN_POINT ( 'NONE',  ( -3.853570894305263561, 8.531289074211878543, -2.447542183238071711 ) ) ;
#90361=CARTESIAN_POINT ( 'NONE',  ( 4.892487020634524342, 4.880525410245029505, -1.277330582746047388E-09 ) ) ;
#90362=CARTESIAN_POINT ( 'NONE',  ( 3.743459811148990291, 7.381470523066878009, -0.7216878364870338292 ) ) ;
#90367=CARTESIAN_POINT ( 'NONE',  ( -4.959250327548641479, 9.007818825440551791, -0.7998128361456362523 ) ) ;
#90380=CARTESIAN_POINT ( 'NONE',  ( 4.692003678781083487, 7.631698837623355658, -1.199719254218450271 ) ) ;
#90407=ORIENTED_EDGE ( 'NONE', *, *, #84784, .F. ) ;
#90417=CARTESIAN_POINT ( 'NONE',  ( 7.377044979611483200, 7.779176362401098999, -0.7216878364870317197 ) ) ;
#90422=CARTESIAN_POINT ( 'NONE',  ( 7.309254211098760834, 8.660456346770972758, 1.082531754730549967 ) ) ;
#90450=CARTESIAN_POINT ( 'NONE',  ( -3.871735385154307263, 6.674719161725423788, -1.199719254218450271 ) ) ;
#90452=CARTESIAN_POINT ( 'NONE',  ( 5.899206235277530297, 7.015400374979486209, -1.082531754730548412 ) ) ;
#90458=CARTESIAN_POINT ( 'NONE',  ( -3.142457743317409680, 6.888227477170756785, 0.7998128361456352531 ) ) ;
#90462=CARTESIAN_POINT ( 'NONE',  ( -7.105881907338169157, 8.423188659050232729, -1.082531754730549967 ) ) ;
#90470=B_SPLINE_CURVE_WITH_KNOTS ( 'NONE', 3,
 ( #191067, #91477, #9133, #75208, #141319, #10193, #42731, #76267, #142376, #186803 ),
 .UNSPECIFIED., .F., .F.,
 ( 4, 3, 3, 4 ),
 ( 1.654962790341811419E-18, 3.125188815118514071E-05, 5.930006937714327664E-05, 8.735821697256892582E-05 ),
 .UNSPECIFIED. ) ;
#90471=CARTESIAN_POINT ( 'NONE',  ( -4.285259070371116863, 7.157163461145040095, 1.199719254218452935 ) ) ;
#90485=CARTESIAN_POINT ( 'NONE',  ( -5.316205630334268406, 6.335233002545657577, -1.082531754730549967 ) ) ;
#90487=CARTESIAN_POINT ( 'NONE',  ( -6.251718229232867685, 6.466295153626015590, -0.7216878364870338292 ) ) ;
#90489=CARTESIAN_POINT ( 'NONE',  ( 5.712781623311797397, 7.758274208654143855, -1.599625672291283607 ) ) ;
#90490=CARTESIAN_POINT ( 'NONE',  ( -4.932134020321308654, 8.976183133675331050, 0.7998128361456291469 ) ) ;
#90509=CARTESIAN_POINT ( 'NONE',  ( 7.862802741282558294, 8.137967717776607657, 0.000000000000000000 ) ) ;
#90511=PRODUCT_DEFINITION ( 'UNKNOWN', '', #97314, #35704 ) ;
#90548=CARTESIAN_POINT ( 'NONE',  ( 4.552505719138623341, 8.533283448962240669, 0.7998128361456341429 ) ) ;
#90555=CARTESIAN_POINT ( 'NONE',  ( -6.468648687051513413, 7.679749902049126220, 1.082531754730549078 ) ) ;
#90561=ADVANCED_FACE ( 'NONE', ( #24523 ), #156693, .T. ) ;
#90566=CARTESIAN_POINT ( 'NONE',  ( 3.810548893104213963, 8.469546410357091659, 2.499999999999999556 ) ) ;
#90569=CARTESIAN_POINT ( 'NONE',  ( 3.074666975249065626, 6.809138247757705820, 0.000000000000000000 ) ) ;
#90570=CARTESIAN_POINT ( 'NONE',  ( 4.016958651398847557, 7.908478536599129249, -0.7998128361456362523 ) ) ;
#90573=DIRECTION ( 'NONE',  ( -1.000000000000000000, 0.000000000000000000, 0.000000000000000000 ) ) ;
#90577=CARTESIAN_POINT ( 'NONE',  ( -6.994027139803241866, 9.253060644560830994, -1.599625672291271394 ) ) ;
#90581=ORIENTED_EDGE ( 'NONE', *, *, #210167, .F. ) ;
#90582=CARTESIAN_POINT ( 'NONE',  ( 5.520104819419390907, 6.469152373191302985, 1.199719254218452935 ) ) ;
#90592=CARTESIAN_POINT ( 'NONE',  ( 5.546694241766559230, 9.485244025454063532, 0.000000000000000000 ) ) ;
#90593=CARTESIAN_POINT ( 'NONE',  ( -4.990809943606286048, 5.955604701363006015, -1.082531754730549967 ) ) ;
#90594=CARTESIAN_POINT ( 'NONE',  ( -5.576146316970437944, 9.727530813099326323, 0.000000000000000000 ) ) ;
#90605=CARTESIAN_POINT ( 'NONE',  ( 6.261886844665240481, 8.398896966899865646, 1.599625672291268286 ) ) ;
#90606=ORIENTED_EDGE ( 'NONE', *, *, #112074, .F. ) ;
#90607=CARTESIAN_POINT ( 'NONE',  ( 6.215487077222150880, 6.216099443039444949, 0.000000000000000000 ) ) ;
#90608=CARTESIAN_POINT ( 'NONE',  ( 7.700104897918568447, 7.948153567185284096, 0.000000000000000000 ) ) ;
#90611=CARTESIAN_POINT ( 'NONE',  ( 6.851666526859736983, 9.086973262793417661, -1.599625672291269396 ) ) ;
#90630=ADVANCED_FACE ( 'NONE', ( #158817 ), #72610, .T. ) ;
#90631=CARTESIAN_POINT ( 'NONE',  ( 5.747730777550676073, 5.670383760089384495, 0.000000000000000000 ) ) ;
#90635=CARTESIAN_POINT ( 'NONE',  ( 5.571474780572990504, 5.464751763615448787, 0.7998128361456352531 ) ) ;
#90640=CARTESIAN_POINT ( 'NONE',  ( 4.085803189671889157, 5.860132702740892263, -1.599625672291273171 ) ) ;
#90644=CARTESIAN_POINT ( 'NONE',  ( 6.048345925472191631, 7.189396680206621149, 1.082531754730549967 ) ) ;
#90646=CARTESIAN_POINT ( 'NONE',  ( -6.818824913030298696, 6.919993584815607335, 0.7998128361456341429 ) ) ;
#90648=CARTESIAN_POINT ( 'NONE',  ( 3.393283585170187688, 7.180857625999046867, 0.7998128361456271485 ) ) ;
#90657=CARTESIAN_POINT ( 'NONE',  ( -5.939880696562884310, 9.943961556049767836, 0.7216878364870267237 ) ) ;
#90694=CARTESIAN_POINT ( 'NONE',  ( 0.4461838333974484927, 2.877219473291486640, 1.949594826320268481 ) ) ;
#90696=CARTESIAN_POINT ( 'NONE',  ( 3.729901657090948230, 6.405283462364505631, 1.082531754730549078 ) ) ;
#90698=DIRECTION ( 'NONE',  ( 0.2636569930688775210, -0.9646164989289152114, 0.000000000000000000 ) ) ;
#90710=CARTESIAN_POINT ( 'NONE',  ( -4.827585214917754719, 7.789877296449459365, -1.199719254218453823 ) ) ;
#90712=CARTESIAN_POINT ( 'NONE',  ( 6.604230223188150894, 9.758666789477915771, -1.082531754730548412 ) ) ;
#90722=CARTESIAN_POINT ( 'NONE',  ( -3.772911886352873445, 7.623757310712140800, 0.7998128361456352531 ) ) ;
#90726=CARTESIAN_POINT ( 'NONE',  ( -5.017926250833627755, 5.026871178826882947, 0.7216878364870257245 ) ) ;
#90730=CARTESIAN_POINT ( 'NONE',  ( -3.122120512896910505, 6.864500708346841229, 0.7998128361456352531 ) ) ;
#90738=CARTESIAN_POINT ( 'NONE',  ( -6.468692700515624949, 6.719432036793461904, 1.751973777778555601E-06 ) ) ;
#90753=CARTESIAN_POINT ( 'NONE',  ( -6.095272577795516789, 9.268845886473535245, 1.199719254218452047 ) ) ;
#90759=ORIENTED_EDGE ( 'NONE', *, *, #64317, .T. ) ;
#90775=DIRECTION ( 'NONE',  ( -0.6507913734559658270, 0.7592566023652989049, 0.000000000000000000 ) ) ;
#90778=CARTESIAN_POINT ( 'NONE',  ( -5.875479466675803231, 7.948088359245467416, -1.599625672291271394 ) ) ;
#90792=CARTESIAN_POINT ( 'NONE',  ( -4.943116297174857898, 7.129802832403653312, 1.247573795494796078 ) ) ;
#90796=CARTESIAN_POINT ( 'NONE',  ( 3.576318658954677598, 7.394398545414291313, 0.7998128361456281477 ) ) ;
#90803=CARTESIAN_POINT ( 'NONE',  ( 6.038177310039780643, 8.137902509836795417, -1.599625672291283607 ) ) ;
#90805=CARTESIAN_POINT ( 'NONE',  ( 7.042534447655770080, 7.180988041878682004, -0.7998128361456341429 ) ) ;
#90819=CARTESIAN_POINT ( 'NONE',  ( 6.053075614097062740, 7.042710966267798689, -1.019147762646470001 ) ) ;
#90821=CARTESIAN_POINT ( 'NONE',  ( 4.570507181582611267, 8.346359121906111511, 0.000000000000000000 ) ) ;
#90829=CARTESIAN_POINT ( 'NONE',  ( -5.008811405605897882, 4.808311159487113073, 0.7998128361456281477 ) ) ;
#90832=VERTEX_POINT ( 'NONE', #27425 ) ;
#90839=CARTESIAN_POINT ( 'NONE',  ( -5.763624699140883934, 6.857221916153382502, -1.082531754730549967 ) ) ;
#90843=CARTESIAN_POINT ( 'NONE',  ( 6.210516883511641772, 9.403297576475722508, 1.199719254218452047 ) ) ;
#90860=CARTESIAN_POINT ( 'NONE',  ( 6.530187263637528439, 7.647581891445782709, -1.199719254218452047 ) ) ;
#90878=ORIENTED_EDGE ( 'NONE', *, *, #201515, .F. ) ;
#90879=CARTESIAN_POINT ( 'NONE',  ( -7.123883369337781879, 7.275895117174344229, 0.7998128361456341429 ) ) ;
#90901=CARTESIAN_POINT ( 'NONE',  ( 4.855228407469603269, 7.718164671139588151, -1.082531754730548412 ) ) ;
#90905=CARTESIAN_POINT ( 'NONE',  ( -7.957709816578236506, 8.248692638954882028, 0.7998128361456341429 ) ) ;
#90910=CARTESIAN_POINT ( 'NONE',  ( -4.123088112331656951, 6.864000993478624579, 1.082531754730549967 ) ) ;
#90915=CARTESIAN_POINT ( 'NONE',  ( 5.573523442662557059, 5.863030555295438262, 0.6332236521834158083 ) ) ;
#90942=CARTESIAN_POINT ( 'NONE',  ( 5.401997860402196316, 5.267028690082820930, 0.000000000000000000 ) ) ;
#90945=CARTESIAN_POINT ( 'NONE',  ( 4.837112831242089683, 4.711959172683063635, 0.000000000000000000 ) ) ;
#90955=CARTESIAN_POINT ( 'NONE',  ( -7.593975437430151132, 8.032261896522864930, -0.7216878364870338292 ) ) ;
#90957=CARTESIAN_POINT ( 'NONE',  ( 4.543390873910913896, 5.433615786718446472, 1.082531754730549078 ) ) ;
#90965=( BOUNDED_SURFACE ( )  B_SPLINE_SURFACE ( 1, 2, ( 
 ( #93562, #44817, #113065, #160677, #27464, #26394, #92507, #158544, #159608, #96773, #110922, #128274, #178003, #176927, #28544, #161758, #29618, #94634, #95704, #13349, #79424, #145541, #63173, #15468, #32808, #133543, #97827, #197427, #199551, #162825, #116250, #100991, #81553, #132481, #65280, #163892, #31756, #16528, #149764, #48022, #182238, #130389, #18672, #147636, #33863, #213654, #183312, #99942, #82611, #131427, #196380, #98883, #180130, #114137, #166006, #17590, #49069, #14400, #146590, #66335, #115188, #67403, #83674, #51194, #181183, #164936, #117316, #1341, #34918, #148695, #167081, #80492, #212608, #64247, #265, #198483, #50128, #207972, #192782, #127906, #63866, #209027, #11909, #130021, #141960, #62791, #31379, #126825, #12969, #176559, #60662, #76906, #45507, #162448, #27093, #128953, #109496, #163510, #80110, #196012, #59599, #79045, #161385, #47648, #110558, #77982, #97455, #145161, #143032, #211166, #125757, #93200, #159231, #146215, #29244, #144105, #194932, #44440, #112688, #191718, #46569, #178699, #15096, #210099, #193858, #61739, #10832, #43375, #175503, #28169, #212233, #111623, #30313, #96398, #177636, #95336, #14024, #94265, #113759, #160305, #179763, #184001, #105733, #82236, #51889, #150465, #19361, #3095, #201299, #35616, #135285, #122037, #69165, #50812, #166701, #181859, #18292, #98504, #81185, #149382, #165632, #148327, #85441, #214327, #133166, #65959, #118012, #147263, #2026, #167764, #101694, #115874, #199166, #964, #151526, #39628, #188002, #132108, #197059, #164566, #114811, #116938, #198116, #55879, #182938, #171762, #34554, #213295, #83297, #67029, #64921, #32436, #100625, #131071, #48697, #84378, #68095, #134230, #180810, #200239, #16151, #49747, #33495, #99568, #17220, #128473, #28750, #190171, #92704, #74304, #62314, #208537, #26603, #158750, #127402, #60173, #194441, #11414, #175016, #192289, #111129, #43949, #12480, #42890, #142529, #27675, #193374, #108999, #126330, #159810, #112202, #110065, #59106, #210685, #25536, #140400, #93770, #156630, #144672, #176077, #160885 ),
 ( #207487, #10345, #46083, #77489, #91644, #143608, #24455, #41825, #124208, #94834, #209601, #76419, #61245, #157697, #45019, #8219, #177132, #78554, #90569, #206419, #58043, #107938, #173963, #9294, #75367, #125266, #141479, #191227, #49271, #197627, #180330, #65478, #148892, #96975, #31952, #51399, #29825, #66534, #199754, #179275, #465, #33009, #116445, #100137, #83877, #132676, #17790, #1538, #166200, #147840, #115393, #64446, #181386, #195517, #178209, #98037, #48222, #30898, #182439, #163023, #15671, #14605, #198682, #95908, #99088, #50327, #34066, #212809, #81758, #164090, #149969, #133746, #67600, #80703, #79623, #47154, #211742, #213858, #146793, #161961, #131628, #114335, #16731, #130591, #13551, #145742, #165140, #82816, #63381, #129536, #113270, #196580, #2608, #183512, #151039, #3666, #121809, #20989, #202946, #136919, #119653, #4731, #88160, #36190, #185638, #205085, #35121, #5800, #139058, #118582, #154228, #186710, #55653, #39408, #23127, #71877, #171534, #155295, #105502, #87086, #54590, #69743, #120737, #134800, #117519, #37270, #201871, #184570, #187776, #102266, #169403, #168341, #137987, #101192, #38339, #204004, #89244, #152095, #153156, #103340, #6878, #72956, #167281, #19936, #18866, #200806, #68677, #70806, #86022, #84950, #104415, #52457, #170464, #135848, #53519, #22049, #60994, #7955, #125013, #106595, #94584, #26346, #58857, #190970, #159558, #92459, #160627, #43699, #207233, #10097, #143351, #76171, #44768, #75112, #174771, #59919, #11155, #141224, #158498, #192036, #144426, #142276, #91384, #28493, #57791, #172622, #126075, #188854, #176881, #208287, #193120, #110876, #209346, #12228, #122895, #109816, #175826, #78301, #25282, #42636, #56727, #27418, #123951, #93516, #40490, #74047, #156371, #127147, #77232, #24198, #90301, #140137, #206163, #108745, #189920, #41565, #107678, #173707, #157444, #9038, #83630, #114093, #30644, #182189, #211491, #111953, #213608, #128225, #116202, #147590, #132434, #198435, #148650, #50081, #62070, #81511, #15421, #33817, #179026, #80445, #99896 ) ),
 .UNSPECIFIED., .F., .F., .T. ) 
 B_SPLINE_SURFACE_WITH_KNOTS ( ( 2, 2 ),
 ( 3, 2, 2, 2, 2, 2, 2, 2, 2, 2, 2, 2, 2, 2, 2, 2, 2, 2, 2, 2, 2, 2, 2, 2, 2, 2, 2, 2, 2, 2, 2, 2, 2, 2, 2, 2, 2, 2, 2, 2, 2, 2, 2, 2, 2, 2, 2, 2, 2, 2, 2, 2, 2, 2, 2, 2, 2, 2, 2, 2, 2, 2, 2, 2, 2, 2, 2, 2, 2, 2, 2, 2, 2, 2, 2, 2, 2, 2, 2, 2, 2, 2, 2, 2, 2, 2, 2, 2, 2, 2, 2, 2, 2, 2, 2, 2, 2, 2, 2, 2, 2, 2, 2, 2, 2, 2, 2, 2, 2, 2, 2, 2, 2, 2, 2, 2, 2, 2, 2, 2, 3 ),
 ( 0.000000000000000000, 1.000000000000000000 ),
 ( 0.000000000000000000, 0.008333333333333333218, 0.01666666666666666644, 0.02500000000000000139, 0.03333333333333333287, 0.04166666666666666435, 0.05000000000000000278, 0.05833333333333333426, 0.06666666666666666574, 0.07499999999999999722, 0.08333333333333332871, 0.09166666666666666019, 0.1000000000000000056, 0.1083333333333333370, 0.1166666666666666685, 0.1250000000000000000, 0.1333333333333333315, 0.1416666666666666630, 0.1499999999999999944, 0.1583333333333333259, 0.1666666666666666574, 0.1749999999999999889, 0.1833333333333333204, 0.1916666666666666796, 0.2000000000000000111, 0.2083333333333333426, 0.2166666666666666741, 0.2250000000000000056, 0.2333333333333333370, 0.2416666666666666685, 0.2500000000000000000, 0.2583333333333333592, 0.2666666666666666630, 0.2750000000000000222, 0.2833333333333333259, 0.2916666666666666852, 0.2999999999999999889, 0.3083333333333333481, 0.3166666666666666519, 0.3250000000000000111, 0.3333333333333333148, 0.3416666666666666741, 0.3499999999999999778, 0.3583333333333333370, 0.3666666666666666408, 0.3750000000000000000, 0.3833333333333333592, 0.3916666666666666630, 0.4000000000000000222, 0.4083333333333333259, 0.4166666666666666852, 0.4249999999999999889, 0.4333333333333333481, 0.4416666666666666519, 0.4500000000000000111, 0.4583333333333333148, 0.4666666666666666741, 0.4749999999999999778, 0.4833333333333333370, 0.4916666666666666408, 0.5000000000000000000, 0.5083333333333333037, 0.5166666666666667185, 0.5250000000000000222, 0.5333333333333333259, 0.5416666666666666297, 0.5500000000000000444, 0.5583333333333333481, 0.5666666666666666519, 0.5749999999999999556, 0.5833333333333333703, 0.5916666666666666741, 0.5999999999999999778, 0.6083333333333332815, 0.6166666666666666963, 0.6250000000000000000, 0.6333333333333333037, 0.6416666666666667185, 0.6500000000000000222, 0.6583333333333333259, 0.6666666666666666297, 0.6750000000000000444, 0.6833333333333333481, 0.6916666666666666519, 0.6999999999999999556, 0.7083333333333333703, 0.7166666666666666741, 0.7249999999999999778, 0.7333333333333332815, 0.7416666666666666963, 0.7500000000000000000, 0.7583333333333333037, 0.7666666666666667185, 0.7750000000000000222, 0.7833333333333333259, 0.7916666666666666297, 0.8000000000000000444, 0.8083333333333333481, 0.8166666666666666519, 0.8249999999999999556, 0.8333333333333333703, 0.8416666666666666741, 0.8499999999999999778, 0.8583333333333332815, 0.8666666666666666963, 0.8750000000000000000, 0.8833333333333333037, 0.8916666666666667185, 0.9000000000000000222, 0.9083333333333333259, 0.9166666666666666297, 0.9250000000000000444, 0.9333333333333333481, 0.9416666666666666519, 0.9499999999999999556, 0.9583333333333333703, 0.9666666666666666741, 0.9749999999999999778, 0.9833333333333332815, 0.9916666666666666963, 1.000000000000000000 ),
 .UNSPECIFIED. ) 
 GEOMETRIC_REPRESENTATION_ITEM ( )  RATIONAL_B_SPLINE_SURFACE ( (
 ( 1.000000000000000000, 0.8660254037844387076, 1.000000000000000000, 0.8660254037844387076, 1.000000000000000000, 0.8660254037844387076, 1.000000000000000000, 0.8660254037844387076, 1.000000000000000000, 0.8660254037844387076, 1.000000000000000000, 0.8660254037844387076, 1.000000000000000000, 0.8660254037844387076, 1.000000000000000000, 0.8660254037844387076, 1.000000000000000000, 0.8660254037844387076, 1.000000000000000000, 0.8660254037844387076, 1.000000000000000000, 0.8660254037844387076, 1.000000000000000000, 0.8660254037844387076, 1.000000000000000000, 0.8660254037844387076, 1.000000000000000000, 0.8660254037844387076, 1.000000000000000000, 0.8660254037844387076, 1.000000000000000000, 0.8660254037844387076, 1.000000000000000000, 0.8660254037844387076, 1.000000000000000000, 0.8660254037844387076, 1.000000000000000000, 0.8660254037844387076, 1.000000000000000000, 0.8660254037844387076, 1.000000000000000000, 0.8660254037844387076, 1.000000000000000000, 0.8660254037844387076, 1.000000000000000000, 0.8660254037844387076, 1.000000000000000000, 0.8660254037844387076, 1.000000000000000000, 0.8660254037844387076, 1.000000000000000000, 0.8660254037844387076, 1.000000000000000000, 0.8660254037844387076, 1.000000000000000000, 0.8660254037844387076, 1.000000000000000000, 0.8660254037844387076, 1.000000000000000000, 0.8660254037844387076, 1.000000000000000000, 0.8660254037844387076, 1.000000000000000000, 0.8660254037844387076, 1.000000000000000000, 0.8660254037844387076, 1.000000000000000000, 0.8660254037844387076, 1.000000000000000000, 0.8660254037844387076, 1.000000000000000000, 0.8660254037844387076, 1.000000000000000000, 0.8660254037844387076, 1.000000000000000000, 0.8660254037844387076, 1.000000000000000000, 0.8660254037844387076, 1.000000000000000000, 0.8660254037844387076, 1.000000000000000000, 0.8660254037844387076, 1.000000000000000000, 0.8660254037844387076, 1.000000000000000000, 0.8660254037844387076, 1.000000000000000000, 0.8660254037844387076, 1.000000000000000000, 0.8660254037844387076, 1.000000000000000000, 0.8660254037844387076, 1.000000000000000000, 0.8660254037844387076, 1.000000000000000000, 0.8660254037844387076, 1.000000000000000000, 0.8660254037844387076, 1.000000000000000000, 0.8660254037844387076, 1.000000000000000000, 0.8660254037844387076, 1.000000000000000000, 0.8660254037844387076, 1.000000000000000000, 0.8660254037844387076, 1.000000000000000000, 0.8660254037844387076, 1.000000000000000000, 0.8660254037844387076, 1.000000000000000000, 0.8660254037844387076, 1.000000000000000000, 0.8660254037844387076, 1.000000000000000000, 0.8660254037844387076, 1.000000000000000000, 0.8660254037844387076, 1.000000000000000000, 0.8660254037844387076, 1.000000000000000000, 0.8660254037844387076, 1.000000000000000000, 0.8660254037844387076, 1.000000000000000000, 0.8660254037844387076, 1.000000000000000000, 0.8660254037844387076, 1.000000000000000000, 0.8660254037844387076, 1.000000000000000000, 0.8660254037844387076, 1.000000000000000000, 0.8660254037844387076, 1.000000000000000000, 0.8660254037844387076, 1.000000000000000000, 0.8660254037844387076, 1.000000000000000000, 0.8660254037844387076, 1.000000000000000000, 0.8660254037844387076, 1.000000000000000000, 0.8660254037844387076, 1.000000000000000000, 0.8660254037844387076, 1.000000000000000000, 0.8660254037844387076, 1.000000000000000000, 0.8660254037844387076, 1.000000000000000000, 0.8660254037844387076, 1.000000000000000000, 0.8660254037844387076, 1.000000000000000000, 0.8660254037844387076, 1.000000000000000000, 0.8660254037844387076, 1.000000000000000000, 0.8660254037844387076, 1.000000000000000000, 0.8660254037844387076, 1.000000000000000000, 0.8660254037844387076, 1.000000000000000000, 0.8660254037844387076, 1.000000000000000000, 0.8660254037844387076, 1.000000000000000000, 0.8660254037844387076, 1.000000000000000000, 0.8660254037844387076, 1.000000000000000000, 0.8660254037844387076, 1.000000000000000000, 0.8660254037844387076, 1.000000000000000000, 0.8660254037844387076, 1.000000000000000000, 0.8660254037844387076, 1.000000000000000000, 0.8660254037844387076, 1.000000000000000000, 0.8660254037844387076, 1.000000000000000000, 0.8660254037844387076, 1.000000000000000000, 0.8660254037844387076, 1.000000000000000000, 0.8660254037844387076, 1.000000000000000000, 0.8660254037844387076, 1.000000000000000000, 0.8660254037844387076, 1.000000000000000000, 0.8660254037844387076, 1.000000000000000000, 0.8660254037844387076, 1.000000000000000000, 0.8660254037844387076, 1.000000000000000000, 0.8660254037844387076, 1.000000000000000000, 0.8660254037844387076, 1.000000000000000000, 0.8660254037844387076, 1.000000000000000000, 0.8660254037844387076, 1.000000000000000000, 0.8660254037844387076, 1.000000000000000000, 0.8660254037844387076, 1.000000000000000000, 0.8660254037844387076, 1.000000000000000000, 0.8660254037844387076, 1.000000000000000000, 0.8660254037844387076, 1.000000000000000000, 0.8660254037844387076, 1.000000000000000000, 0.8660254037844387076, 1.000000000000000000, 0.8660254037844387076, 1.000000000000000000, 0.8660254037844387076, 1.000000000000000000, 0.8660254037844387076, 1.000000000000000000, 0.8660254037844387076, 1.000000000000000000, 0.8660254037844387076, 1.000000000000000000, 0.8660254037844387076, 1.000000000000000000, 0.8660254037844387076, 1.000000000000000000, 0.8660254037844387076, 1.000000000000000000, 0.8660254037844387076, 1.000000000000000000),
 ( 1.000000000000000000, 0.8660254037844387076, 1.000000000000000000, 0.8660254037844387076, 1.000000000000000000, 0.8660254037844387076, 1.000000000000000000, 0.8660254037844387076, 1.000000000000000000, 0.8660254037844387076, 1.000000000000000000, 0.8660254037844387076, 1.000000000000000000, 0.8660254037844387076, 1.000000000000000000, 0.8660254037844387076, 1.000000000000000000, 0.8660254037844387076, 1.000000000000000000, 0.8660254037844387076, 1.000000000000000000, 0.8660254037844387076, 1.000000000000000000, 0.8660254037844387076, 1.000000000000000000, 0.8660254037844387076, 1.000000000000000000, 0.8660254037844387076, 1.000000000000000000, 0.8660254037844387076, 1.000000000000000000, 0.8660254037844387076, 1.000000000000000000, 0.8660254037844387076, 1.000000000000000000, 0.8660254037844387076, 1.000000000000000000, 0.8660254037844387076, 1.000000000000000000, 0.8660254037844387076, 1.000000000000000000, 0.8660254037844387076, 1.000000000000000000, 0.8660254037844387076, 1.000000000000000000, 0.8660254037844387076, 1.000000000000000000, 0.8660254037844387076, 1.000000000000000000, 0.8660254037844387076, 1.000000000000000000, 0.8660254037844387076, 1.000000000000000000, 0.8660254037844387076, 1.000000000000000000, 0.8660254037844387076, 1.000000000000000000, 0.8660254037844387076, 1.000000000000000000, 0.8660254037844387076, 1.000000000000000000, 0.8660254037844387076, 1.000000000000000000, 0.8660254037844387076, 1.000000000000000000, 0.8660254037844387076, 1.000000000000000000, 0.8660254037844387076, 1.000000000000000000, 0.8660254037844387076, 1.000000000000000000, 0.8660254037844387076, 1.000000000000000000, 0.8660254037844387076, 1.000000000000000000, 0.8660254037844387076, 1.000000000000000000, 0.8660254037844387076, 1.000000000000000000, 0.8660254037844387076, 1.000000000000000000, 0.8660254037844387076, 1.000000000000000000, 0.8660254037844387076, 1.000000000000000000, 0.8660254037844387076, 1.000000000000000000, 0.8660254037844387076, 1.000000000000000000, 0.8660254037844387076, 1.000000000000000000, 0.8660254037844387076, 1.000000000000000000, 0.8660254037844387076, 1.000000000000000000, 0.8660254037844387076, 1.000000000000000000, 0.8660254037844387076, 1.000000000000000000, 0.8660254037844387076, 1.000000000000000000, 0.8660254037844387076, 1.000000000000000000, 0.8660254037844387076, 1.000000000000000000, 0.8660254037844387076, 1.000000000000000000, 0.8660254037844387076, 1.000000000000000000, 0.8660254037844387076, 1.000000000000000000, 0.8660254037844387076, 1.000000000000000000, 0.8660254037844387076, 1.000000000000000000, 0.8660254037844387076, 1.000000000000000000, 0.8660254037844387076, 1.000000000000000000, 0.8660254037844387076, 1.000000000000000000, 0.8660254037844387076, 1.000000000000000000, 0.8660254037844387076, 1.000000000000000000, 0.8660254037844387076, 1.000000000000000000, 0.8660254037844387076, 1.000000000000000000, 0.8660254037844387076, 1.000000000000000000, 0.8660254037844387076, 1.000000000000000000, 0.8660254037844387076, 1.000000000000000000, 0.8660254037844387076, 1.000000000000000000, 0.8660254037844387076, 1.000000000000000000, 0.8660254037844387076, 1.000000000000000000, 0.8660254037844387076, 1.000000000000000000, 0.8660254037844387076, 1.000000000000000000, 0.8660254037844387076, 1.000000000000000000, 0.8660254037844387076, 1.000000000000000000, 0.8660254037844387076, 1.000000000000000000, 0.8660254037844387076, 1.000000000000000000, 0.8660254037844387076, 1.000000000000000000, 0.8660254037844387076, 1.000000000000000000, 0.8660254037844387076, 1.000000000000000000, 0.8660254037844387076, 1.000000000000000000, 0.8660254037844387076, 1.000000000000000000, 0.8660254037844387076, 1.000000000000000000, 0.8660254037844387076, 1.000000000000000000, 0.8660254037844387076, 1.000000000000000000, 0.8660254037844387076, 1.000000000000000000, 0.8660254037844387076, 1.000000000000000000, 0.8660254037844387076, 1.000000000000000000, 0.8660254037844387076, 1.000000000000000000, 0.8660254037844387076, 1.000000000000000000, 0.8660254037844387076, 1.000000000000000000, 0.8660254037844387076, 1.000000000000000000, 0.8660254037844387076, 1.000000000000000000, 0.8660254037844387076, 1.000000000000000000, 0.8660254037844387076, 1.000000000000000000, 0.8660254037844387076, 1.000000000000000000, 0.8660254037844387076, 1.000000000000000000, 0.8660254037844387076, 1.000000000000000000, 0.8660254037844387076, 1.000000000000000000, 0.8660254037844387076, 1.000000000000000000, 0.8660254037844387076, 1.000000000000000000, 0.8660254037844387076, 1.000000000000000000, 0.8660254037844387076, 1.000000000000000000, 0.8660254037844387076, 1.000000000000000000, 0.8660254037844387076, 1.000000000000000000, 0.8660254037844387076, 1.000000000000000000, 0.8660254037844387076, 1.000000000000000000, 0.8660254037844387076, 1.000000000000000000, 0.8660254037844387076, 1.000000000000000000, 0.8660254037844387076, 1.000000000000000000, 0.8660254037844387076, 1.000000000000000000, 0.8660254037844387076, 1.000000000000000000, 0.8660254037844387076, 1.000000000000000000, 0.8660254037844387076, 1.000000000000000000, 0.8660254037844387076, 1.000000000000000000, 0.8660254037844387076, 1.000000000000000000, 0.8660254037844387076, 1.000000000000000000, 0.8660254037844387076, 1.000000000000000000, 0.8660254037844387076, 1.000000000000000000, 0.8660254037844387076, 1.000000000000000000, 0.8660254037844387076, 1.000000000000000000) ) ) 
 REPRESENTATION_ITEM ( '' )  SURFACE ( )  );
#90977=CARTESIAN_POINT ( 'NONE',  ( -3.174017359375036929, 6.717120995997236221, 0.7216878364870338292 ) ) ;
#91009=CARTESIAN_POINT ( 'NONE',  ( -5.935437387732586778, 10.14670372898850381, -0.7998128361456362523 ) ) ;
#91012=CARTESIAN_POINT ( 'NONE',  ( -4.925354943514475003, 8.968274210734028529, 0.000000000000000000 ) ) ;
#91017=CARTESIAN_POINT ( 'NONE',  ( -7.404161286394468355, 7.810812053647902431, 0.000000000000000000 ) ) ;
#91023=CARTESIAN_POINT ( 'NONE',  ( -4.004454267989906668, 5.765225627445230927, 1.599625672291270506 ) ) ;
#91032=( BOUNDED_CURVE ( )  B_SPLINE_CURVE ( 2, ( #209642, #61283, #193415, #45058, #168374, #34102, #201903 ),
 .UNSPECIFIED., .F., .T. ) 
 B_SPLINE_CURVE_WITH_KNOTS ( ( 3, 2, 2, 3 ),
 ( 0.3999999999999997446, 0.4083333333333331039, 0.4166666666666665741, 0.4249999999999999334 ),
 .UNSPECIFIED. ) 
 CURVE ( )  GEOMETRIC_REPRESENTATION_ITEM ( )  RATIONAL_B_SPLINE_CURVE ( ( 1.000000000000004441, 0.8660254037844342667, 1.000000000000000000, 0.8660254037844387076, 1.000000000000000000, 0.8660254037844395958, 0.9999999999999991118 ) ) 
 REPRESENTATION_ITEM ( '' )  );
#91033=CARTESIAN_POINT ( 'NONE',  ( -6.851666526859749418, 9.086973262793417661, -1.599625672291271394 ) ) ;
#91035=CARTESIAN_POINT ( 'NONE',  ( 5.142555292688428814, 7.778213139218437711, -1.168464917166486039 ) ) ;
#91039=CARTESIAN_POINT ( 'NONE',  ( 8.154303043976348420, 8.478051404252736845, 0.7998128361456281477 ) ) ;
#91052=DIRECTION ( 'NONE',  ( -1.000000000000000000, 0.000000000000000000, 0.000000000000000000 ) ) ;
#91062=CARTESIAN_POINT ( 'NONE',  ( 5.481239241674765950, 9.616805891921051952, -0.7998128361456481317 ) ) ;
#91078=CARTESIAN_POINT ( 'NONE',  ( 6.536750166778501736, 6.811520125210166476, 0.4662371894542677864 ) ) ;
#91079=CARTESIAN_POINT ( 'NONE',  ( -4.868786560638931782, 6.773613302202437403, 1.443375672974058777 ) ) ;
#91107=CARTESIAN_POINT ( 'NONE',  ( 3.902768115887398803, 5.646591783325653147, -1.599625672291269396 ) ) ;
#91123=CARTESIAN_POINT ( 'NONE',  ( -5.956828388357799042, 8.042995434541133193, 1.599625672291263179 ) ) ;
#91128=EDGE_CURVE ( 'NONE', #128658, #80820, #143518, .T. ) ;
#91138=EDGE_LOOP ( 'NONE', ( #103274, #40046, #171802, #90759, #185544, #102981, #195169, #114957, #24236, #18417, #106699, #210794, #64303 ) ) ;
#91141=CARTESIAN_POINT ( 'NONE',  ( 4.923546060418115822, 5.773167154356443120, -1.199719254218452047 ) ) ;
#91152=CARTESIAN_POINT ( 'NONE',  ( 4.764469552112262640, 8.169203124620777245, 0.7669358090897534508 ) ) ;
#91155=CARTESIAN_POINT ( 'NONE',  ( 4.990887655837901171, 7.926359819171765686, 1.063311220390166234 ) ) ;
#91173=CARTESIAN_POINT ( 'NONE',  ( -6.140917232347002042, 6.129101290685087911, -0.7998128361456362523 ) ) ;
#91175=CARTESIAN_POINT ( 'NONE',  ( 5.194709132691408549, 6.089524072008651423, 1.199719254218452935 ) ) ;
#91178=CARTESIAN_POINT ( 'NONE',  ( -4.613517410400161722, 8.604463755433990002, -0.7998128361456362523 ) ) ;
#91184=CARTESIAN_POINT ( 'NONE',  ( -4.595593225409446703, 8.485229224138180371, -0.2149309537713070539 ) ) ;
#91192=CARTESIAN_POINT ( 'NONE',  ( -5.194182247366913252, 7.153241603385088965, 1.443375672974058777 ) ) ;
#91203=CARTESIAN_POINT ( 'NONE',  ( 6.224601922449876312, 6.434659462379210382, 0.000000000000000000 ) ) ;
#91207=CARTESIAN_POINT ( 'NONE',  ( -7.449279056065764237, 7.655523418356991350, 0.7998128361456341429 ) ) ;
#91218=CARTESIAN_POINT ( 'NONE',  ( -4.502716413514313842, 5.386162249589033557, -1.082531754730549967 ) ) ;
#91224=CARTESIAN_POINT ( 'NONE',  ( 5.246079093845007257, 5.085123462432798114, 0.7998128361456352531 ) ) ;
#91239=CARTESIAN_POINT ( 'NONE',  ( 3.570880328030153539, 7.341005539872356600, 0.2896471194287209006 ) ) ;
#91249=CARTESIAN_POINT ( 'NONE',  ( -5.858531774880906262, 6.967946837850073294, 1.082531754730549078 ) ) ;
#91277=CARTESIAN_POINT ( 'NONE',  ( -4.977251789548269301, 4.979417640660637190, 0.7216878364870257245 ) ) ;
#91278=CARTESIAN_POINT ( 'NONE',  ( -4.516801452008150086, 5.298631777878131111, 1.199719254218452935 ) ) ;
#91283=CARTESIAN_POINT ( 'NONE',  ( -5.309953438407606363, 6.223975762010839574, 1.199719254218452935 ) ) ;
#91286=FACE_OUTER_BOUND ( 'NONE', #176695, .T. ) ;
#91293=CARTESIAN_POINT ( 'NONE',  ( -5.327428015527048366, 5.180030537728460338, -0.7998128361456362523 ) ) ;
#91295=CARTESIAN_POINT ( 'NONE',  ( 5.959663945170571075, 7.214374732172471383, -1.219933935757764099 ) ) ;
#91299=CARTESIAN_POINT ( 'NONE',  ( 5.713835393516482952, 5.630839145382857680, 0.7998128361456352531 ) ) ;
#91303=CARTESIAN_POINT ( 'NONE',  ( -5.340986169140711226, 5.195848383611072485, 0.000000000000000000 ) ) ;
#91308=CARTESIAN_POINT ( 'NONE',  ( -4.634908411025374875, 6.500755460986618495, 1.599625672291263179 ) ) ;
#91314=CARTESIAN_POINT ( 'NONE',  ( 6.007671464186837618, 6.181573927739029806, 0.7216878364870328300 ) ) ;
#91315=CARTESIAN_POINT ( 'NONE',  ( -5.438229012412899799, 7.437962829272074750, -1.443375672974066548 ) ) ;
#91318=CARTESIAN_POINT ( 'NONE',  ( -6.120580001926503755, 6.105374521861167025, -0.7998128361456361413 ) ) ;
#91321=CARTESIAN_POINT ( 'NONE',  ( 5.076602173674213070, 4.887400388900169368, 0.000000000000000000 ) ) ;
#91329=CARTESIAN_POINT ( 'NONE',  ( 4.881097632946307385, 6.623252254984194565, 1.537733183400882053 ) ) ;
#91332=CARTESIAN_POINT ( 'NONE',  ( 4.710809438828709617, 8.349644928513606956, 0.6747337923850562635 ) ) ;
#91341=CARTESIAN_POINT ( 'NONE',  ( 5.176180785367283654, 9.260904359562321275, -0.7998128361456481317 ) ) ;
#91350=CARTESIAN_POINT ( 'NONE',  ( 5.264264421420239870, 7.666326994050936428, 1.218248458220503094 ) ) ;
#91358=CARTESIAN_POINT ( 'NONE',  ( 7.517069824134078537, 7.734612647770044092, 0.000000000000000000 ) ) ;
#91363=CARTESIAN_POINT ( 'NONE',  ( -4.617805310829839804, 8.366410568267871994, -0.2388493967704352627 ) ) ;
#91370=EDGE_CURVE ( 'NONE', #78339, #149147, #189382, .T. ) ;
#91371=CARTESIAN_POINT ( 'NONE',  ( -6.282224075085783177, 8.422623735723785643, 1.599625672291269396 ) ) ;
#91384=CARTESIAN_POINT ( 'NONE',  ( 6.875920180786008196, 8.050936961452347163, -1.199719254218452047 ) ) ;
#91390=CARTESIAN_POINT ( 'NONE',  ( -7.065207446052809814, 9.336104335185325453, -1.443375672974066548 ) ) ;
#91392=CARTESIAN_POINT ( 'NONE',  ( 5.713835393516482952, 5.630839145382857680, 0.7998128361456352531 ) ) ;
#91395=CARTESIAN_POINT ( 'NONE',  ( 3.892599500454941630, 6.595097612955829192, 1.082531754730549078 ) ) ;
#91396=LINE ( 'NONE', #155308, #86901 ) ;
#91410=CARTESIAN_POINT ( 'NONE',  ( -7.024532985656169792, 9.288650798055913427, 1.443375672974064550 ) ) ;
#91411=CARTESIAN_POINT ( 'NONE',  ( 3.390420931869152721, 6.113185632892752075, -1.199719254218452047 ) ) ;
#91423=CARTESIAN_POINT ( 'NONE',  ( -6.608673532018475960, 6.674816973635147477, -0.7998128361456362523 ) ) ;
#91424=CARTESIAN_POINT ( 'NONE',  ( -5.204350862799341115, 7.165104988056252289, -1.599625672291271394 ) ) ;
#91426=CARTESIAN_POINT ( 'NONE',  ( 7.146556367734764770, 9.431011410480991231, 1.443375672974063439 ) ) ;
#91437=CARTESIAN_POINT ( 'NONE',  ( -5.178050853460543834, 7.761234873892349562, -1.181743852105126669 ) ) ;
#91441=CARTESIAN_POINT ( 'NONE',  ( 5.885648082108200896, 6.039213315313952002, 0.7216878364870328300 ) ) ;
#91445=CARTESIAN_POINT ( 'NONE',  ( -6.794571259104023930, 7.956029886156682274, 1.199719254218452047 ) ) ;
#91459=CARTESIAN_POINT ( 'NONE',  ( 3.867818961648523235, 7.734482231890414283, 1.040834085586084257E-14 ) ) ;
#91475=DIRECTION ( 'NONE',  ( 0.6292706268317891372, -0.7771862570881751253, 0.000000000000000000 ) ) ;
#91477=CARTESIAN_POINT ( 'NONE',  ( 2.970281070238892873, 6.580799555089337893, 0.4329187822878322600 ) ) ;
#91496=AXIS2_PLACEMENT_3D ( 'NONE', #143407, #176935, #208346 ) ;
#91497=CARTESIAN_POINT ( 'NONE',  ( 5.695833931516881776, 9.659240330162777610, -0.7216878364870458196 ) ) ;
#91501=DIRECTION ( 'NONE',  ( 0.000000000000000000, -1.000000000000000000, 0.000000000000000000 ) ) ;
#91502=CARTESIAN_POINT ( 'NONE',  ( 7.336370518326124746, 7.731722824234849689, -0.7216878364870317197 ) ) ;
#91530=CARTESIAN_POINT ( 'NONE',  ( -5.842637852846353397, 5.781108681267656202, 0.7998128361456281477 ) ) ;
#91532=CARTESIAN_POINT ( 'NONE',  ( 6.522881301506172846, 6.782652071278222117, -0.7216878364870458196 ) ) ;
#91537=CARTESIAN_POINT ( 'NONE',  ( -3.156015896931072540, 6.904045323053366268, 0.000000000000000000 ) ) ;
#91542=CARTESIAN_POINT ( 'NONE',  ( -4.553559489343377287, 6.405848385690952718, -1.599625672291271394 ) ) ;
#91550=CARTESIAN_POINT ( 'NONE',  ( -4.610654757099099221, 7.536791762327691657, 1.199719254218452935 ) ) ;
#91560=CARTESIAN_POINT ( 'NONE',  ( -3.471769853551161411, 6.208092708188416076, 1.199719254218452935 ) ) ;
#91566=CARTESIAN_POINT ( 'NONE',  ( -4.828112100242291760, 6.726159765073026264, -1.443375672974066548 ) ) ;
#91567=CARTESIAN_POINT ( 'NONE',  ( -4.895902867866254837, 7.765618208269001066, 1.082531754730549967 ) ) ;
#91568=CARTESIAN_POINT ( 'NONE',  ( 6.225128807330042591, 7.291680359087043151, -1.199719254218452047 ) ) ;
#91570=CARTESIAN_POINT ( 'NONE',  ( -6.642568916052639771, 6.714361588341672515, 0.000000000000000000 ) ) ;
#91574=DIRECTION ( 'NONE',  ( 0.000000000000000000, 0.000000000000000000, -1.000000000000000000 ) ) ;
#91590=CARTESIAN_POINT ( 'NONE',  ( 8.011942431032855083, 8.311964022485323511, 0.7998128361456291469 ) ) ;
#91613=AXIS2_PLACEMENT_3D ( 'NONE', #83139, #178532, #79947 ) ;
#91619=CARTESIAN_POINT ( 'NONE',  ( 5.055755612212820438, 4.906101081808937892, 0.2771076874560872705 ) ) ;
#91620=CARTESIAN_POINT ( 'NONE',  ( -1.843739406749240750, 8.920000000000001705, -0.7749999999999996891 ) ) ;
#91627=CARTESIAN_POINT ( 'NONE',  ( 5.143339171537801846, 7.093924681584509173, 1.599625672291269396 ) ) ;
#91633=CARTESIAN_POINT ( 'NONE',  ( -6.170369307550858551, 8.292126506933035657, 1.443375672974058777 ) ) ;
#91644=CARTESIAN_POINT ( 'NONE',  ( 3.410758162289653672, 6.136912401716668519, -1.199719254218453823 ) ) ;
#91645=CARTESIAN_POINT ( 'NONE',  ( 7.015418140428412386, 7.149352350113456822, 0.7998128361456331437 ) ) ;
#91656=ORIENTED_EDGE ( 'NONE', *, *, #163618, .T. ) ;
#91657=CARTESIAN_POINT ( 'NONE',  ( 3.725458348705031231, 7.568394850123006279, -1.734723475976807094E-15 ) ) ;
#91670=ORIENTED_EDGE ( 'NONE', *, *, #136398, .T. ) ;
#91671=CARTESIAN_POINT ( 'NONE',  ( 6.916067756746836714, 8.201738816693689316, -1.082531754730548412 ) ) ;
#91672=CARTESIAN_POINT ( 'NONE',  ( -4.882344714696960075, 5.829061934302122161, 1.082531754730549078 ) ) ;
#91673=CARTESIAN_POINT ( 'NONE',  ( -5.237192476628793614, 9.332084666034067055, 0.7998128361456291469 ) ) ;
#91684=CARTESIAN_POINT ( 'NONE',  ( 6.703580607314123085, 6.785541894813420072, 0.000000000000000000 ) ) ;
#91685=CARTESIAN_POINT ( 'NONE',  ( 5.027041095616958444, 9.086908054853605421, 0.000000000000000000 ) ) ;
#91688=CARTESIAN_POINT ( 'NONE',  ( 3.390947816749319443, 6.970206529600588397, -1.734723475976807094E-15 ) ) ;
#91707=CARTESIAN_POINT ( 'NONE',  ( 4.278479993564246797, 7.149254538203735798, 1.199719254218452047 ) ) ;
#91709=CARTESIAN_POINT ( 'NONE',  ( -5.015590482412729756, 4.816220082428420923, 0.000000000000000000 ) ) ;
#91712=CARTESIAN_POINT ( 'NONE',  ( 5.061990249855835344, 6.999017606288844284, -1.599625672291273171 ) ) ;
#91717=CARTESIAN_POINT ( 'NONE',  ( 7.126746022638799971, 8.343567110280638133, 1.199719254218452047 ) ) ;
#91722=CARTESIAN_POINT ( 'NONE',  ( 6.888951449519509218, 7.209733910627123876, -0.7216878364870317197 ) ) ;
#91724=CARTESIAN_POINT ( 'NONE',  ( -5.010620288702242853, 8.003418215864698482, -1.199719254218453823 ) ) ;
#91725=CARTESIAN_POINT ( 'NONE',  ( 5.065906673361608270, 5.939254536123854677, -1.199719254218450271 ) ) ;
#91735=CARTESIAN_POINT ( 'NONE',  ( -4.472210567661380587, 6.310941310395290493, 1.599625672291270506 ) ) ;
#91762=CARTESIAN_POINT ( 'NONE',  ( 3.268924434670684498, 6.827845917175511481, -1.734723475976807094E-15 ) ) ;
#91767=CARTESIAN_POINT ( 'NONE',  ( 5.969332771766739931, 10.18624834369502885, -0.7998128361456481317 ) ) ;
#91768=CARTESIAN_POINT ( 'NONE',  ( 3.512971199272317602, 6.152197928242737923, -1.082531754730549967 ) ) ;
#91779=CARTESIAN_POINT ( 'NONE',  ( -6.394605727500880299, 7.489403432619674561, -1.199719254218452047 ) ) ;
#91781=CARTESIAN_POINT ( 'NONE',  ( 6.495764994278797388, 8.671754808115688107, 1.443375672974063439 ) ) ;
#91782=B_SPLINE_CURVE_WITH_KNOTS ( 'NONE', 3,
 ( #39840, #18223, #19295, #86448, #55020, #168760, #20363, #138413, #105947, #120089 ),
 .UNSPECIFIED., .F., .F.,
 ( 4, 2, 2, 2, 4 ),
 ( 0.0001032556302127828247, 0.0003933207648079593225, 0.0006833858994031357390, 0.0009734510339983121555, 0.001263516168593488680 ),
 .UNSPECIFIED. ) ;
#91793=CARTESIAN_POINT ( 'NONE',  ( -6.296835998904160014, 6.311006518335105397, 0.000000000000000000 ) ) ;
#91803=CARTESIAN_POINT ( 'NONE',  ( -4.984557751679625781, 5.844347460828191565, 1.199719254218452935 ) ) ;
#91826=CARTESIAN_POINT ( 'NONE',  ( -5.271087860662956537, 9.371629280740593870, 0.000000000000000000 ) ) ;
#91828=CARTESIAN_POINT ( 'NONE',  ( -6.168033539574333979, 6.160736982450306876, 0.7998128361456281477 ) ) ;
#91837=CARTESIAN_POINT ( 'NONE',  ( -6.161504026110072196, 7.065710439381887475, -1.087211863304170523 ) ) ;
#91854=CARTESIAN_POINT ( 'NONE',  ( -6.805266759416629618, 6.904175738932996964, 0.000000000000000000 ) ) ;
#91884=CARTESIAN_POINT ( 'NONE',  ( 5.529746549527311039, 7.544733289238903851, -1.599625672291281386 ) ) ;
#91893=CARTESIAN_POINT ( 'NONE',  ( 6.512744780709700088, 6.750401516064612473, 0.09762648057792142064 ) ) ;
#91897=CARTESIAN_POINT ( 'NONE',  ( 6.276967689384127524, 6.888745287521969907, 0.7578909454171089966 ) ) ;
#91899=CARTESIAN_POINT ( 'NONE',  ( 5.885648082108188461, 8.920320958217979879, 1.082531754730549967 ) ) ;
#91906=CARTESIAN_POINT ( 'NONE',  ( -4.664887371553763096, 7.600063145858131364, -1.199719254218453823 ) ) ;
#91914=CARTESIAN_POINT ( 'NONE',  ( -4.760321331729590710, 8.567808963744235839, 0.7216878364870267237 ) ) ;
#91918=CARTESIAN_POINT ( 'NONE',  ( 5.481239241674765950, 9.616805891921051952, -0.7998128361456481317 ) ) ;
#91919=CARTESIAN_POINT ( 'NONE',  ( -5.817856928050925802, 5.960123635580414359, -1.359047942450207100E-08 ) ) ;
#91933=CARTESIAN_POINT ( 'NONE',  ( 4.543917759235442944, 5.330267469643351852, 1.199719254218452935 ) ) ;
#91950=CARTESIAN_POINT ( 'NONE',  ( -6.261886844665283114, 8.398896966899865646, 1.599625672291269396 ) ) ;
#91955=CARTESIAN_POINT ( 'NONE',  ( -6.435690514315323796, 6.800136771869164320, 0.4354173353855045336 ) ) ;
#91957=CIRCLE ( 'NONE', #130060, 0.8300000000000008482 ) ;
#91974=CARTESIAN_POINT ( 'NONE',  ( 6.265276383290871109, 7.442482214328385304, -1.082531754730548412 ) ) ;
#91985=CARTESIAN_POINT ( 'NONE',  ( -3.689227196694341515, 7.318199139536432973, -0.7216878364870458196 ) ) ;
#91995=DIRECTION ( 'NONE',  ( -0.7592566023652995710, 0.6507913734559650498, 0.000000000000000000 ) ) ;
#92017=CARTESIAN_POINT ( 'NONE',  ( 3.878514461961128479, 6.682628084666728085, -1.199719254218448494 ) ) ;
#92019=CARTESIAN_POINT ( 'NONE',  ( -1.833030277982346634, 2.531131934864056632, -2.499999999999998668 ) ) ;
#92029=CARTESIAN_POINT ( 'NONE',  ( -5.465345320084574965, 9.390336950158399532, 0.000000000000000000 ) ) ;
#92031=CARTESIAN_POINT ( 'NONE',  ( 4.055297343818933697, 5.824542549245813383, 1.443375672974058777 ) ) ;
#92049=CARTESIAN_POINT ( 'NONE',  ( -5.180624094197616714, 5.216685329418210948, 0.7216878364870257245 ) ) ;
#92079=CARTESIAN_POINT ( 'NONE',  ( -7.608060475923978494, 8.905100639113307182, 1.199719254218452047 ) ) ;
#92082=CARTESIAN_POINT ( 'NONE',  ( -5.855142236255304944, 7.924361590421551860, -1.599625672291271394 ) ) ;
#92083=CARTESIAN_POINT ( 'NONE',  ( -5.602815672633493449, 5.724646472043899870, 0.3052438699321499693 ) ) ;
#92085=CARTESIAN_POINT ( 'NONE',  ( -4.642607672489913462, 8.343425853053251018, 0.4124909477912245825 ) ) ;
#92086=VERTEX_POINT ( 'NONE', #134014 ) ;
#92088=CARTESIAN_POINT ( 'NONE',  ( -5.411112705185557203, 9.327065566109540740, 0.7216878364870267237 ) ) ;
#92089=B_SPLINE_CURVE_WITH_KNOTS ( 'NONE', 3,
 ( #15008, #147188, #78957, #160221, #145079, #211082, #48618, #13945, #212144, #63780 ),
 .UNSPECIFIED., .F., .F.,
 ( 4, 3, 3, 4 ),
 ( 0.000000000000000000, 6.251591618973194396E-05, 0.0001688574560067633145, 0.0002758324972496365921 ),
 .UNSPECIFIED. ) ;
#92090=CARTESIAN_POINT ( 'NONE',  ( 6.658462837642789012, 9.821938173008357253, 1.082531754730549078 ) ) ;
#92092=CARTESIAN_POINT ( 'NONE',  ( -5.002032328799064231, 4.800402236545811441, -0.7998128361456362523 ) ) ;
#92096=CARTESIAN_POINT ( 'NONE',  ( -5.191846479390389568, 5.021852078902356631, 0.7998128361456281477 ) ) ;
#92105=ORIENTED_EDGE ( 'NONE', *, *, #123715, .F. ) ;
#92106=CARTESIAN_POINT ( 'NONE',  ( 5.647444738788365726, 7.344714329438926548, -1.230740020431456028 ) ) ;
#92110=CARTESIAN_POINT ( 'NONE',  ( 4.923546060418115822, 5.773167154356443120, -1.199719254218452047 ) ) ;
#92114=EDGE_CURVE ( 'NONE', #188684, #150164, #29428, .T. ) ;
#92117=AXIS2_PLACEMENT_3D ( 'NONE', #149684, #38067, #198407 ) ;
#92134=CARTESIAN_POINT ( 'NONE',  ( 8.154303043976348420, 8.478051404252736845, 0.7998128361456281477 ) ) ;
#92151=DIRECTION ( 'NONE',  ( -0.000000000000000000, -1.000000000000000000, -0.000000000000000000 ) ) ;
#92152=CARTESIAN_POINT ( 'NONE',  ( 6.592372495380235620, 6.775069446727209233, 0.2122460957004346782 ) ) ;
#92153=CARTESIAN_POINT ( 'NONE',  ( -3.946832114909637479, 7.618738210787614484, 0.7216878364870338292 ) ) ;
#92160=CARTESIAN_POINT ( 'NONE',  ( 4.549612403093820312, 8.500000000000243361, -0.2314049244472246580 ) ) ;
#92167=ORIENTED_EDGE ( 'NONE', *, *, #145312, .T. ) ;
#92183=CARTESIAN_POINT ( 'NONE',  ( 4.472210567661338843, 6.310941310395290493, 1.599625672291261402 ) ) ;
#92205=CARTESIAN_POINT ( 'NONE',  ( -4.457598643843001973, 8.422558527783969851, 0.000000000000000000 ) ) ;
#92218=CARTESIAN_POINT ( 'NONE',  ( 3.888156192069020634, 7.758209000714329839, 1.040834085586084257E-14 ) ) ;
#92226=CARTESIAN_POINT ( 'NONE',  ( 4.688369027973070757, 8.258219454933637849, 0.5882785783308928096 ) ) ;
#92228=CARTESIAN_POINT ( 'NONE',  ( 4.909045613421183063, 8.010784895652180992, 0.9812996480243344477 ) ) ;
#92249=VECTOR ( 'NONE', #194192, 1000.000000000000000 ) ;
#92252=CARTESIAN_POINT ( 'NONE',  ( -4.294900800479008574, 8.232744377192641849, 0.000000000000000000 ) ) ;
#92254=CARTESIAN_POINT ( 'NONE',  ( 5.086243903782109221, 5.962981304947771122, -1.199719254218452047 ) ) ;
#92258=CARTESIAN_POINT ( 'NONE',  ( -4.599959256786493533, 8.588645909551377855, 0.000000000000000000 ) ) ;
#92261=CARTESIAN_POINT ( 'NONE',  ( 8.174640274396848483, 8.501778173076651512, 0.7998128361456291469 ) ) ;
#92263=( BOUNDED_CURVE ( )  B_SPLINE_CURVE ( 2, ( #169719, #5052, #71128, #54912, #187029, #38663, #135112 ),
 .UNSPECIFIED., .F., .T. ) 
 B_SPLINE_CURVE_WITH_KNOTS ( ( 3, 2, 2, 3 ),
 ( 0.4250000000000004885, 0.4333333333333335147, 0.4416666666666664853, 0.4499999999999995115 ),
 .UNSPECIFIED. ) 
 CURVE ( )  GEOMETRIC_REPRESENTATION_ITEM ( )  RATIONAL_B_SPLINE_CURVE ( ( 0.9999999999999920064, 0.8660254037844467012, 1.000000000000000000, 0.8660254037844387076, 1.000000000000000000, 0.8660254037844467012, 0.9999999999999920064 ) ) 
 REPRESENTATION_ITEM ( '' )  );
#92267=CARTESIAN_POINT ( 'NONE',  ( -5.780704523637806069, 7.347994962087573079, -1.310296981949153006 ) ) ;
#92268=FACE_OUTER_BOUND ( 'NONE', #84069, .T. ) ;
#92285=CARTESIAN_POINT ( 'NONE',  ( 4.407809338218622308, 8.156544971314787063, 0.000000000000000000 ) ) ;
#92286=DIRECTION ( 'NONE',  ( 0.6507913734559658270, 0.7592566023652989049, 0.000000000000000000 ) ) ;
#92289=CARTESIAN_POINT ( 'NONE',  ( -5.101610940492132151, 9.173906207207963348, -0.7998128361456362523 ) ) ;
#92291=ORIENTED_EDGE ( 'NONE', *, *, #213238, .T. ) ;
#92298=CARTESIAN_POINT ( 'NONE',  ( -3.363831509966363598, 5.978201624052440266, -1.082531754730548412 ) ) ;
#92303=CARTESIAN_POINT ( 'NONE',  ( 4.224247379109608680, 7.085983154673295203, -1.199719254218452047 ) ) ;
#92307=CARTESIAN_POINT ( 'NONE',  ( -4.902626719552124257, 4.881029176893854959, -0.5815614086314065956 ) ) ;
#92354=CARTESIAN_POINT ( 'NONE',  ( -3.757017964318317471, 6.436919154129725484, 1.082531754730549967 ) ) ;
#92361=CARTESIAN_POINT ( 'NONE',  ( -5.795184315198522285, 5.725746220678519904, -0.7998128361456362523 ) ) ;
#92364=CARTESIAN_POINT ( 'NONE',  ( 5.397554552016217144, 7.390509292142662723, 1.443375672974065660 ) ) ;
#92369=CARTESIAN_POINT ( 'NONE',  ( -4.248501033035892327, 6.049946853332221153, -1.599625672291271394 ) ) ;
#92370=CARTESIAN_POINT ( 'NONE',  ( 6.606300428615679898, 6.765996464729716386, -0.04887194053871009303 ) ) ;
#92374=CARTESIAN_POINT ( 'NONE',  ( 5.551137550152489553, 5.441024994791534120, 0.7998128361456352531 ) ) ;
#92382=CARTESIAN_POINT ( 'NONE',  ( -2.830620210203090181, 6.524417021870718258, 0.000000000000000000 ) ) ;
#92384=EDGE_LOOP ( 'NONE', ( #125709, #147228, #174692, #133791 ) ) ;
#92386=CARTESIAN_POINT ( 'NONE',  ( -4.125423880308188629, 8.035021303660014880, -0.7998128361456481317 ) ) ;
#92390=CARTESIAN_POINT ( 'NONE',  ( 4.055297343818923039, 7.745280977848496562, 0.7216878364870257245 ) ) ;
#92391=CARTESIAN_POINT ( 'NONE',  ( -6.902509602688830626, 7.225551755991315162, -0.7216878364870338292 ) ) ;
#92397=CARTESIAN_POINT ( 'NONE',  ( 5.551137550152489553, 5.441024994791534120, 0.7998128361456352531 ) ) ;
#92405=CARTESIAN_POINT ( 'NONE',  ( 5.879395890181562834, 6.888325289080478697, -1.199719254218452047 ) ) ;
#92425=CARTESIAN_POINT ( 'NONE',  ( 4.600487305768355739, 8.366733224642864286, -0.1591645125929436189 ) ) ;
#92432=CARTESIAN_POINT ( 'NONE',  ( 5.494797395288433250, 9.632623737803665875, 0.000000000000000000 ) ) ;
#92438=CARTESIAN_POINT ( 'NONE',  ( -4.879429750001362365, 8.060225557361109239, -0.9362273787268098335 ) ) ;
#92443=ADVANCED_FACE ( 'NONE', ( #23406 ), #92724, .F. ) ;
#92447=CARTESIAN_POINT ( 'NONE',  ( -7.306918443122272677, 7.489436036589583345, 0.7998128361456341429 ) ) ;
#92453=CARTESIAN_POINT ( 'NONE',  ( -4.499752021454321849, 4.967787669261691796, -0.8784368744512593974 ) ) ;
#92459=CARTESIAN_POINT ( 'NONE',  ( 6.119526231721748033, 8.232809585132461194, 1.599625672291269396 ) ) ;
#92469=CARTESIAN_POINT ( 'NONE',  ( 3.217027588192558074, 6.975225629525113824, -1.734723475976807094E-15 ) ) ;
#92472=CARTESIAN_POINT ( 'NONE',  ( 4.529832720297257254, 8.298905583739861314, 0.000000000000000000 ) ) ;
#92486=CARTESIAN_POINT ( 'NONE',  ( -3.851398154733808088, 6.650992392901508232, -1.199719254218450271 ) ) ;
#92487=CARTESIAN_POINT ( 'NONE',  ( 7.688882512725796481, 8.142986817701137525, 0.000000000000000000 ) ) ;
#92496=ORIENTED_EDGE ( 'NONE', *, *, #14937, .F. ) ;
#92498=EDGE_LOOP ( 'NONE', ( #44515, #13204, #173750 ) ) ;
#92499=CARTESIAN_POINT ( 'NONE',  ( -6.286140498591554326, 7.362860665558790707, 1.199719254218452047 ) ) ;
#92500=CARTESIAN_POINT ( 'NONE',  ( -5.646044625448194410, 5.551749915969804938, 0.000000000000000000 ) ) ;
#92502=CARTESIAN_POINT ( 'NONE',  ( 7.824464048418096951, 8.301165276008827476, -0.7216878364870317197 ) ) ;
#92504=ORIENTED_EDGE ( 'NONE', *, *, #101474, .T. ) ;
#92507=CARTESIAN_POINT ( 'NONE',  ( 2.891631901464575272, 6.595597328342462262, 0.000000000000000000 ) ) ;
#92514=CARTESIAN_POINT ( 'NONE',  ( -5.355672060655169098, 7.601107163255693244, -1.239215230201977436 ) ) ;
#92519=CARTESIAN_POINT ( 'NONE',  ( 4.963693636378940788, 5.923969009597785274, -1.082531754730548412 ) ) ;
#92524=CARTESIAN_POINT ( 'NONE',  ( -5.875479466675803231, 7.948088359245467416, -1.599625672291271394 ) ) ;
#92538=CARTESIAN_POINT ( 'NONE',  ( 4.681308178468477799, 8.683552984847038303, 0.000000000000000000 ) ) ;
#92572=CARTESIAN_POINT ( 'NONE',  ( 7.363486825997814123, 7.763358516518489516, 0.000000000000000000 ) ) ;
#92579=CARTESIAN_POINT ( 'NONE',  ( 5.844973620822823790, 9.833236634353070826, 0.7216878364870317197 ) ) ;
#92601=CARTESIAN_POINT ( 'NONE',  ( -3.644109427023046521, 7.473487774827342278, 0.000000000000000000 ) ) ;
#92603=CARTESIAN_POINT ( 'NONE',  ( 5.275531169048895741, 7.248148678680751189, -1.443375672974078761 ) ) ;
#92608=CARTESIAN_POINT ( 'NONE',  ( -6.154475385960665790, 6.144919136567696505, 0.000000000000000000 ) ) ;
#92614=CARTESIAN_POINT ( 'NONE',  ( -3.363304624641834106, 6.081549941127532222, -1.199719254218452047 ) ) ;
#92622=CARTESIAN_POINT ( 'NONE',  ( -3.461074353238556167, 7.259946855412102273, 0.000000000000000000 ) ) ;
#92632=CARTESIAN_POINT ( 'NONE',  ( -5.320648938720212051, 5.172121614787156929, 0.000000000000000000 ) ) ;
#92635=CARTESIAN_POINT ( 'NONE',  ( -6.943184063974186415, 7.273005294157565359, -0.7216878364870338292 ) ) ;
#92636=CARTESIAN_POINT ( 'NONE',  ( -4.597623488365601752, 8.377994813152914944, 0.7216878364870267237 ) ) ;
#92637=CARTESIAN_POINT ( 'NONE',  ( 4.538947565524982686, 8.517465603079630299, 0.000000000000000000 ) ) ;
#92638=CARTESIAN_POINT ( 'NONE',  ( -5.818384198920079520, 6.817144982608731141, 1.199719254218452935 ) ) ;
#92656=CARTESIAN_POINT ( 'NONE',  ( 5.352436782344940802, 9.466536356036257871, 0.000000000000000000 ) ) ;
#92674=CARTESIAN_POINT ( 'NONE',  ( 4.598366155629488361, 8.485928551783258555, 0.1149073004905968448 ) ) ;
#92687=CARTESIAN_POINT ( 'NONE',  ( 5.040599249230596435, 9.102725900736217568, 0.7998128361456341429 ) ) ;
#92690=CARTESIAN_POINT ( 'NONE',  ( -3.871735385154307263, 6.674719161725423788, -1.199719254218450271 ) ) ;
#92693=CARTESIAN_POINT ( 'NONE',  ( -6.983858524370814003, 9.241197259889665006, 1.443375672974064550 ) ) ;
#92704=CARTESIAN_POINT ( 'NONE',  ( 6.156284269057003655, 9.340026192945279249, -1.199719254218452047 ) ) ;
#92705=CARTESIAN_POINT ( 'NONE',  ( 5.529746549527311039, 7.544733289238903851, -1.599625672291281386 ) ) ;
#92713=ORIENTED_EDGE ( 'NONE', *, *, #44262, .T. ) ;
#92714=CARTESIAN_POINT ( 'NONE',  ( 2.898410978271408922, 6.603506251283770112, -0.7998128361456362523 ) ) ;
#92720=CARTESIAN_POINT ( 'NONE',  ( 6.170896192875352959, 7.228408975556602556, 1.199719254218453823 ) ) ;
#92724=PLANE ( 'NONE',  #112453 ) ;
#92731=CARTESIAN_POINT ( 'NONE',  ( 6.048345925472166762, 10.07050432311064903, 0.7216878364870317197 ) ) ;
#92732=CARTESIAN_POINT ( 'NONE',  ( -5.966997003790232235, 7.094489604910957148, -1.082531754730549967 ) ) ;
#92733=CARTESIAN_POINT ( 'NONE',  ( -7.923814432544069142, 8.209148024248356990, 0.000000000000000000 ) ) ;
#92746=CARTESIAN_POINT ( 'NONE',  ( 4.193214648376505593, 8.114110533073061404, 0.000000000000000000 ) ) ;
#92747=CARTESIAN_POINT ( 'NONE',  ( 7.049313524462606395, 7.188896964819984525, 0.000000000000000000 ) ) ;
#92750=CARTESIAN_POINT ( 'NONE',  ( 3.838366886000300404, 6.531826229425389485, -1.082531754730548412 ) ) ;
#92754=DIRECTION ( 'NONE',  ( 0.7592566023653005702, -0.6507913734559639396, 0.000000000000000000 ) ) ;
#92757=CARTESIAN_POINT ( 'NONE',  ( -3.231779075379147770, 6.036511184309971689, 2.420000000000000373 ) ) ;
#92767=AXIS2_PLACEMENT_3D ( 'NONE', #44000, #93825, #89551 ) ;
#92770=CARTESIAN_POINT ( 'NONE',  ( 5.273195401072370281, 5.116759154198018855, -0.7998128361456481317 ) ) ;
#92775=CARTESIAN_POINT ( 'NONE',  ( 5.550083779947807550, 7.568460058062819407, -1.599625672291283607 ) ) ;
#92780=DIRECTION ( 'NONE',  ( -1.000000000000000000, 0.000000000000000000, 0.000000000000000000 ) ) ;
#92784=CARTESIAN_POINT ( 'NONE',  ( 7.838022202476093270, 8.316983122409855156, 0.7216878364870267237 ) ) ;
#92786=CARTESIAN_POINT ( 'NONE',  ( -6.791708605802965870, 6.888357893050385705, -0.7998128361456362523 ) ) ;
#92787=CARTESIAN_POINT ( 'NONE',  ( 4.044074958626150185, 7.940114228364351767, 0.7998128361456271485 ) ) ;
#92788=ORIENTED_EDGE ( 'NONE', *, *, #30754, .T. ) ;
#92797=CARTESIAN_POINT ( 'NONE',  ( -5.418418667316934112, 6.350518529071726981, -1.199719254218453823 ) ) ;
#92826=CARTESIAN_POINT ( 'NONE',  ( 3.390947817193682656, 6.009837315817661008, -1.082531754730549967 ) ) ;
#92832=CARTESIAN_POINT ( 'NONE',  ( 3.540087506499646874, 7.144202834309300698, -0.7216878364870338292 ) ) ;
#92844=CARTESIAN_POINT ( 'NONE',  ( -6.330731382938325602, 6.350551133041632212, 0.7998128361456281477 ) ) ;
#92846=CARTESIAN_POINT ( 'NONE',  ( -6.934069218746458318, 7.054445274817795486, -0.7998128361456362523 ) ) ;
#92848=CARTESIAN_POINT ( 'NONE',  ( 6.902509602688803980, 9.146290184594002781, -1.443375672974064550 ) ) ;
#92856=CARTESIAN_POINT ( 'NONE',  ( -6.459533842268148973, 6.500820668926428958, 0.000000000000000000 ) ) ;
#92861=DIRECTION ( 'NONE',  ( -0.6507913734559641616, -0.7592566023653004592, 0.000000000000000000 ) ) ;
#92863=CARTESIAN_POINT ( 'NONE',  ( -4.421367491832313590, 6.251624388594711590, 1.443375672974065660 ) ) ;
#92868=CARTESIAN_POINT ( 'NONE',  ( -5.418418667316934112, 6.350518529071726981, -1.199719254218453823 ) ) ;
#92884=CARTESIAN_POINT ( 'NONE',  ( -3.147653791585729444, 8.920000000000001705, -2.419999999999998597 ) ) ;
#92890=CARTESIAN_POINT ( 'NONE',  ( -6.818824913030298696, 6.919993584815607335, 0.7998128361456341429 ) ) ;
#92892=CARTESIAN_POINT ( 'NONE',  ( -5.978219388983010418, 5.939287140093762574, -0.7998128361456362523 ) ) ;
#92918=CARTESIAN_POINT ( 'NONE',  ( -4.782994330570982555, 8.802186828966616972, 0.000000000000000000 ) ) ;
#92920=ORIENTED_EDGE ( 'NONE', *, *, #71027, .T. ) ;
#92945=CARTESIAN_POINT ( 'NONE',  ( 7.075376061485196821, 9.347967719856493218, 1.599625672291268286 ) ) ;
#92959=CARTESIAN_POINT ( 'NONE',  ( 5.794989345469916842, 7.230977472937116346, 1.182549002416101835 ) ) ;
#92961=CARTESIAN_POINT ( 'NONE',  ( 6.888951449519509218, 7.209733910627123876, -0.7216878364870317197 ) ) ;
#92968=CARTESIAN_POINT ( 'NONE',  ( -3.949167883330528372, 7.829389307186077396, 1.214306433183764966E-14 ) ) ;
#92970=VERTEX_POINT ( 'NONE', #109015 ) ;
#92975=CARTESIAN_POINT ( 'NONE',  ( -6.333067150914850174, 8.481940657524365434, 1.443375672974064550 ) ) ;
#92979=CARTESIAN_POINT ( 'NONE',  ( 7.679767667498067496, 7.924426798361372093, 0.000000000000000000 ) ) ;
#92981=CARTESIAN_POINT ( 'NONE',  ( 5.090963066000425030, 4.916608305390635536, -0.1510418726307351800 ) ) ;
#92985=CARTESIAN_POINT ( 'NONE',  ( -2.986538976760251263, 6.706322249520737522, -0.7998128361456481317 ) ) ;
#92995=CARTESIAN_POINT ( 'NONE',  ( 6.587282531393223728, 8.778525268082516320, 1.599625672291268286 ) ) ;
#93011=CARTESIAN_POINT ( 'NONE',  ( -3.794760873454035899, 7.353399519509664195, 0.6126618612011502929 ) ) ;
#93014=CARTESIAN_POINT ( 'NONE',  ( -6.180537922983287302, 8.303989891604203422, -1.599625672291271394 ) ) ;
#93017=CARTESIAN_POINT ( 'NONE',  ( 5.182959862174088883, 9.268813282503625572, 0.7998128361456331437 ) ) ;
#93020=CARTESIAN_POINT ( 'NONE',  ( -6.502161524297833672, 6.757477167027320597, -0.005777863564433716181 ) ) ;
#93037=CARTESIAN_POINT ( 'NONE',  ( 6.238160076063542725, 6.450477308261824305, -0.7216878364870458196 ) ) ;
#93038=ORIENTED_EDGE ( 'NONE', *, *, #186024, .T. ) ;
#93048=CARTESIAN_POINT ( 'NONE',  ( -6.617788377246204945, 6.893376992974917350, -0.7216878364870338292 ) ) ;
#93079=CARTESIAN_POINT ( 'NONE',  ( 3.854260808034858155, 7.718664386007802136, -0.7998128361456362523 ) ) ;
#93091=CARTESIAN_POINT ( 'NONE',  ( -7.607533591043815768, 8.048079742405473525, 0.000000000000000000 ) ) ;
#93093=CARTESIAN_POINT ( 'NONE',  ( 4.001064729364292916, 6.721640380016713934, -1.082531754730548412 ) ) ;
#93115=AXIS2_PLACEMENT_3D ( 'NONE', #2095, #19429, #67097 ) ;
#93139=CARTESIAN_POINT ( 'NONE',  ( 5.584829485406742400, 5.817820313668822685, -0.7485926948523046187 ) ) ;
#93144=CARTESIAN_POINT ( 'NONE',  ( -6.526270840131767059, 8.707344961610770540, -1.599625672291271394 ) ) ;
#93147=CARTESIAN_POINT ( 'NONE',  ( -4.938913097128142304, 8.984092056616635347, -0.7998128361456362523 ) ) ;
#93148=CARTESIAN_POINT ( 'NONE',  ( -5.386518286579200954, 7.671588192869585043, 1.336358942847740927 ) ) ;
#93149=CARTESIAN_POINT ( 'NONE',  ( -4.444040490229336449, 8.406740681901359480, 0.7998128361456350310 ) ) ;
#93160=CARTESIAN_POINT ( 'NONE',  ( -4.899292406491858820, 6.809203455697518947, -1.599625672291271394 ) ) ;
#93170=ORIENTED_EDGE ( 'NONE', *, *, #176689, .T. ) ;
#93176=CARTESIAN_POINT ( 'NONE',  ( 4.199993725183334803, 8.122019456014369254, -0.7998128361456362523 ) ) ;
#93182=LINE ( 'NONE', #106260, #7673 ) ;
#93191=CARTESIAN_POINT ( 'NONE',  ( 3.006787879153326681, 6.373552747333731006, -0.4818892653130519843 ) ) ;
#93200=CARTESIAN_POINT ( 'NONE',  ( 5.367048706163317640, 7.354919138647580290, -1.599625672291281386 ) ) ;
#93201=CARTESIAN_POINT ( 'NONE',  ( 4.224247379109608680, 7.085983154673295203, -1.199719254218452047 ) ) ;
#93203=CARTESIAN_POINT ( 'NONE',  ( 4.472210567661338843, 6.310941310395290493, 1.599625672291261402 ) ) ;
#93215=CARTESIAN_POINT ( 'NONE',  ( 5.141188686642438554, 7.897460914975725998, 1.230089993873971999 ) ) ;
#93217=CARTESIAN_POINT ( 'NONE',  ( -4.299344108864961989, 6.109263775132799168, -1.443375672974066548 ) ) ;
#93244=CARTESIAN_POINT ( 'NONE',  ( 3.390420931869152721, 6.113185632892752075, -1.199719254218452047 ) ) ;
#93264=CARTESIAN_POINT ( 'NONE',  ( -5.759181390754928742, 9.941071732514568993, 0.000000000000000000 ) ) ;
#93276=VERTEX_POINT ( 'NONE', #21804 ) ;
#93277=CARTESIAN_POINT ( 'NONE',  ( 6.073126464278658432, 6.050012061272033392, 0.000000000000000000 ) ) ;
#93290=CARTESIAN_POINT ( 'NONE',  ( 5.279289985772466665, 7.652873027719338417, 1.222721368963412214 ) ) ;
#93311=CARTESIAN_POINT ( 'NONE',  ( -4.959250327548641479, 9.007818825440551791, -0.7998128361456362523 ) ) ;
#93313=CARTESIAN_POINT ( 'NONE',  ( 4.441177836928239309, 7.339068688795062911, 1.199719254218452047 ) ) ;
#93316=CARTESIAN_POINT ( 'NONE',  ( -5.427006627220116286, 9.553534508390610469, -0.7998128361456362523 ) ) ;
#93319=CARTESIAN_POINT ( 'NONE',  ( 7.309781096423290769, 8.557108029695882578, 1.199719254218452935 ) ) ;
#93324=CARTESIAN_POINT ( 'NONE',  ( -5.830795741961422252, 7.309361553235873998, -1.292907557591252088 ) ) ;
#93325=DIRECTION ( 'NONE',  ( 0.000000000000000000, 0.000000000000000000, -1.000000000000000000 ) ) ;
#93334=B_SPLINE_CURVE_WITH_KNOTS ( 'NONE', 3,
 ( #141228, #57795, #140142, #10101 ),
 .UNSPECIFIED., .F., .F.,
 ( 4, 4 ),
 ( 0.0002312911391078497833, 0.0002795137126933823967 ),
 .UNSPECIFIED. ) ;
#93342=CARTESIAN_POINT ( 'NONE',  ( 5.451787166470912993, 6.493411461371761284, -1.082531754730548412 ) ) ;
#93345=CARTESIAN_POINT ( 'NONE',  ( -5.912237504011027767, 9.055304967058290799, 1.199719254218454489 ) ) ;
#93360=CARTESIAN_POINT ( 'NONE',  ( 4.492547798081839794, 6.334668079219206049, 1.599625672291262513 ) ) ;
#93395=B_SPLINE_CURVE_WITH_KNOTS ( 'NONE', 3,
 ( #102929, #70394, #101862, #166869, #185223, #87743, #53107, #18463, #119240, #198276 ),
 .UNSPECIFIED., .F., .F.,
 ( 4, 3, 3, 4 ),
 ( 8.276099466726772067E-17, 3.125225830659262568E-05, 6.250473674881420159E-05, 0.0001070711423775351414 ),
 .UNSPECIFIED. ) ;
#93409=ORIENTED_EDGE ( 'NONE', *, *, #16357, .T. ) ;
#93410=CARTESIAN_POINT ( 'NONE',  ( -3.485854892044998543, 6.120562236477518070, -1.082531754730546636 ) ) ;
#93417=CARTESIAN_POINT ( 'NONE',  ( -4.749098946536820520, 8.762642214260091933, 0.7998128361456281477 ) ) ;
#93425=CARTESIAN_POINT ( 'NONE',  ( -4.980641328173854632, 6.904110530993182948, 1.599625672291263179 ) ) ;
#93427=CARTESIAN_POINT ( 'NONE',  ( 6.225987253121650689, 7.022442755726078900, -1.008712875586889712 ) ) ;
#93432=CARTESIAN_POINT ( 'NONE',  ( 5.559725510055676168, 8.644040974110419384, 1.199719254218451159 ) ) ;
#93439=CARTESIAN_POINT ( 'NONE',  ( -7.761116589180078407, 8.019333873657032541, 0.000000000000000000 ) ) ;
#93444=CARTESIAN_POINT ( 'NONE',  ( -5.743814354044916470, 6.730146830254374990, -1.199719254218453823 ) ) ;
#93445=EDGE_CURVE ( 'NONE', #47959, #52032, #157396, .T. ) ;
#93449=CARTESIAN_POINT ( 'NONE',  ( 5.194182247366868843, 8.113610817686430110, 1.082531754730548412 ) ) ;
#93450=CARTESIAN_POINT ( 'NONE',  ( -4.787437638956920871, 8.599444655509458357, -0.7216878364870338292 ) ) ;
#93459=CARTESIAN_POINT ( 'NONE',  ( 6.052789233858158369, 6.026285292448116948, 0.000000000000000000 ) ) ;
#93485=CARTESIAN_POINT ( 'NONE',  ( 4.605417112443645600, 8.360468292628990383, 0.2083848827989076002 ) ) ;
#93493=CARTESIAN_POINT ( 'NONE',  ( 5.657495238652423097, 9.822437888394988548, 0.000000000000000000 ) ) ;
#93498=CARTESIAN_POINT ( 'NONE',  ( -4.627894000755552462, 8.353582960325299567, 0.3099817540855500653 ) ) ;
#93504=CARTESIAN_POINT ( 'NONE',  ( -6.474900878978163021, 9.711745571186627402, -1.199719254218452047 ) ) ;
#93516=CARTESIAN_POINT ( 'NONE',  ( 7.686546744304875389, 7.932335721302671949, 0.7998128361456291469 ) ) ;
#93521=DIRECTION ( 'NONE',  ( -0.6507913734559640506, -0.7592566023653003482, 0.000000000000000000 ) ) ;
#93524=VERTEX_POINT ( 'NONE', #191790 ) ;
#93526=CARTESIAN_POINT ( 'NONE',  ( 4.203910148689107729, 7.062256385849379647, -1.199719254218448494 ) ) ;
#93529=CARTESIAN_POINT ( 'NONE',  ( 5.112833325684902341, 7.058334528089426740, -1.443375672974078761 ) ) ;
#93536=CARTESIAN_POINT ( 'NONE',  ( -5.520246714036333380, 7.462180650995058784, 1.249303437716933196 ) ) ;
#93539=ORIENTED_EDGE ( 'NONE', *, *, #201026, .T. ) ;
#93542=CARTESIAN_POINT ( 'NONE',  ( -5.093022980588950865, 5.970890227889075419, -1.199719254218453823 ) ) ;
#93543=CARTESIAN_POINT ( 'NONE',  ( 5.695833931516881776, 9.659240330162777610, -0.7216878364870458196 ) ) ;
#93549=ORIENTED_EDGE ( 'NONE', *, *, #162643, .F. ) ;
#93550=FACE_OUTER_BOUND ( 'NONE', #106242, .T. ) ;
#93555=CARTESIAN_POINT ( 'NONE',  ( -6.180537922983287302, 8.303989891604203422, -1.599625672291271394 ) ) ;
#93556=CARTESIAN_POINT ( 'NONE',  ( -5.659602779061863487, 5.567567761852417085, 0.7998128361456281477 ) ) ;
#93558=CARTESIAN_POINT ( 'NONE',  ( 7.471952054462756010, 7.889901283060952508, 0.7216878364870267237 ) ) ;
#93562=CARTESIAN_POINT ( 'NONE',  ( 4.913904330310220558, 4.697586238308844919, 0.000000000000000000 ) ) ;
#93571=CARTESIAN_POINT ( 'NONE',  ( -5.295344997983027824, 7.654313019038245791, -1.225062028442117423 ) ) ;
#93577=CARTESIAN_POINT ( 'NONE',  ( 6.224601922449876312, 6.434659462379210382, 0.000000000000000000 ) ) ;
#93583=CARTESIAN_POINT ( 'NONE',  ( -7.130662446144611977, 7.283804040115648526, 0.000000000000000000 ) ) ;
#93599=CARTESIAN_POINT ( 'NONE',  ( 5.180097208873055692, 8.201141289397330780, -1.199719254218450271 ) ) ;
#93631=CARTESIAN_POINT ( 'NONE',  ( 6.753369913382843315, 8.011924666102361314, -1.082531754730548412 ) ) ;
#93659=B_SPLINE_CURVE_WITH_KNOTS ( 'NONE', 3,
 ( #138797, #69487, #38088, #106335, #104159, #204817, #136665, #7693, #122630, #25019 ),
 .UNSPECIFIED., .F., .F.,
 ( 4, 3, 3, 4 ),
 ( 0.000000000000000000, 3.125366356300422706E-05, 6.250667109586610789E-05, 0.0001104411237298844468 ),
 .UNSPECIFIED. ) ;
#93663=CARTESIAN_POINT ( 'NONE',  ( -6.005335696210345020, 5.970922831858983315, 0.7998128361456281477 ) ) ;
#93665=CARTESIAN_POINT ( 'NONE',  ( 6.170369307550823912, 7.331757292631694511, 1.082531754730549967 ) ) ;
#93670=CARTESIAN_POINT ( 'NONE',  ( -4.793689830883590020, 7.750332681742931662, 1.199719254218452935 ) ) ;
#93676=CARTESIAN_POINT ( 'NONE',  ( -4.390861645979385663, 6.216034235099629157, -1.599625672291271394 ) ) ;
#93683=CARTESIAN_POINT ( 'NONE',  ( -4.423703259808839938, 8.383013913077441259, 0.7998128361456352531 ) ) ;
#93692=CARTESIAN_POINT ( 'NONE',  ( -3.298376509874564988, 7.070132704820777825, 0.000000000000000000 ) ) ;
#93696=CARTESIAN_POINT ( 'NONE',  ( -6.319508997745553636, 6.545384383557486530, 0.7216878364870257245 ) ) ;
#93698=CARTESIAN_POINT ( 'NONE',  ( -5.763624699140882157, 7.817591130454727200, -1.443375672974066548 ) ) ;
#93699=CARTESIAN_POINT ( 'NONE',  ( 4.688087255275310561, 8.691461907788344377, -0.7998128361456381397 ) ) ;
#93700=CARTESIAN_POINT ( 'NONE',  ( -6.794571259104023930, 7.956029886156682274, 1.199719254218452047 ) ) ;
#93720=CARTESIAN_POINT ( 'NONE',  ( 6.607619761813720238, 8.802252036906432764, 1.599625672291268286 ) ) ;
#93739=CARTESIAN_POINT ( 'NONE',  ( 4.937886321289528979, 7.980522944944189234, -1.013380012275147291 ) ) ;
#93752=CARTESIAN_POINT ( 'NONE',  ( 5.905458427204159477, 9.047396044116986502, 1.199719254218452047 ) ) ;
#93758=CARTESIAN_POINT ( 'NONE',  ( -5.763624699140868834, 9.738329559057408602, -0.7216878364870338292 ) ) ;
#93770=CARTESIAN_POINT ( 'NONE',  ( 6.535912570239620578, 9.782925877658371405, 1.199719254218452047 ) ) ;
#93771=CARTESIAN_POINT ( 'NONE',  ( 6.852720297064418986, 6.959538199522133262, 0.7998128361456331437 ) ) ;
#93789=CARTESIAN_POINT ( 'NONE',  ( 5.013482942003290255, 9.071090208970993274, -0.7998128361456481317 ) ) ;
#93801=CARTESIAN_POINT ( 'NONE',  ( -5.153507786970276783, 6.145418851954329575, -1.082531754730549967 ) ) ;
#93802=CARTESIAN_POINT ( 'NONE',  ( -6.237633190739009237, 9.434933268240943249, 1.199719254218452047 ) ) ;
#93813=FACE_OUTER_BOUND ( 'NONE', #174428, .T. ) ;
#93814=CARTESIAN_POINT ( 'NONE',  ( 7.038618024149998043, 8.240751112043669835, -1.199719254218452047 ) ) ;
#93817=CARTESIAN_POINT ( 'NONE',  ( 5.533136087708556694, 5.627949321847663278, 0.000000000000000000 ) ) ;
#93819=VERTEX_POINT ( 'NONE', #111694 ) ;
#93825=DIRECTION ( 'NONE',  ( 0.000000000000000000, 0.000000000000000000, 1.000000000000000000 ) ) ;
#93837=CARTESIAN_POINT ( 'NONE',  ( 5.422335090822693715, 5.290755458906732933, 0.000000000000000000 ) ) ;
#93839=CARTESIAN_POINT ( 'NONE',  ( -4.516801452008150086, 5.298631777878131111, 1.199719254218452935 ) ) ;
#93843=CARTESIAN_POINT ( 'NONE',  ( 6.249382461256315580, 6.255644057745969988, -0.7998128361456481317 ) ) ;
#93848=CARTESIAN_POINT ( 'NONE',  ( 0.000000000000000000, 0.08000000000000020983, 2.080000000000000071 ) ) ;
#93853=CARTESIAN_POINT ( 'NONE',  ( 5.668717624289557833, 8.667235424096215723, -1.082531754730548412 ) ) ;
#93855=CARTESIAN_POINT ( 'NONE',  ( -5.986807348886189040, 9.142303119412650503, -1.199719254218452047 ) ) ;
#93856=CARTESIAN_POINT ( 'NONE',  ( 3.542423274920540432, 7.354853930707762721, -1.734723475976807094E-15 ) ) ;
#93866=CARTESIAN_POINT ( 'NONE',  ( -5.971440312176176768, 5.931378217152456500, 0.000000000000000000 ) ) ;
#93870=EDGE_LOOP ( 'NONE', ( #99346, #83108, #181664, #10909 ) ) ;
#93891=VECTOR ( 'NONE', #22892, 1000.000000000000114 ) ;
#93896=CARTESIAN_POINT ( 'NONE',  ( 4.421367491832282504, 5.291255174293369556, 1.082531754730549078 ) ) ;
#93901=DIRECTION ( 'NONE',  ( -0.6029061840396265914, 0.7978120914393163066, 0.000000000000000000 ) ) ;
#93902=CARTESIAN_POINT ( 'NONE',  ( 4.597623488365603528, 5.496887170248887067, -1.082531754730548412 ) ) ;
#93913=CARTESIAN_POINT ( 'NONE',  ( -5.829079699232685208, 5.765290835385048496, 0.000000000000000000 ) ) ;
#93915=CARTESIAN_POINT ( 'NONE',  ( -5.586841817283045408, 8.675676665875643678, 1.199719254218454489 ) ) ;
#93917=CARTESIAN_POINT ( 'NONE',  ( 5.492461626867537916, 9.421972641405202964, -0.7216878364870458196 ) ) ;
#93926=CARTESIAN_POINT ( 'NONE',  ( -4.938913097128142304, 8.984092056616635347, -0.7998128361456362523 ) ) ;
#93933=CARTESIAN_POINT ( 'NONE',  ( -5.695833931516914639, 6.778132687258748845, 1.082531754730549078 ) ) ;
#93938=CARTESIAN_POINT ( 'NONE',  ( -4.339491684825780737, 7.220434844675483355, -1.199719254218455378 ) ) ;
#93953=LINE ( 'NONE', #206595, #20032 ) ;
#93958=CARTESIAN_POINT ( 'NONE',  ( -6.306477729012051725, 7.386587434382707151, 1.199719254218452047 ) ) ;
#93960=CARTESIAN_POINT ( 'NONE',  ( -5.679940009482361774, 5.591294530676332641, 0.7998128361456281477 ) ) ;
#93976=CARTESIAN_POINT ( 'NONE',  ( -0.1216878429548678975, 3.463015919485879834, -1.996294584693599994 ) ) ;
#93986=CARTESIAN_POINT ( 'NONE',  ( -5.661411662158206681, 8.762674818229999829, -1.199719254218452047 ) ) ;
#94014=CARTESIAN_POINT ( 'NONE',  ( 6.373214726875630731, 9.593111727067046957, 1.199719254218452047 ) ) ;
#94026=CARTESIAN_POINT ( 'NONE',  ( 6.137634773950260580, 6.983624353001562923, 0.9378011681944794509 ) ) ;
#94029=CARTESIAN_POINT ( 'NONE',  ( 7.349928672384120176, 7.747540670635879145, 0.7216878364870267237 ) ) ;
#94036=CARTESIAN_POINT ( 'NONE',  ( -3.637330350216213759, 7.465578851886037093, -0.7998128361456481317 ) ) ;
#94043=CARTESIAN_POINT ( 'NONE',  ( -5.261973015435229328, 9.153069261400824885, 0.000000000000000000 ) ) ;
#94051=CARTESIAN_POINT ( 'NONE',  ( -3.149236820124241110, 6.896136400112061970, -0.7998128361456481317 ) ) ;
#94062=CARTESIAN_POINT ( 'NONE',  ( 5.833751235630055376, 10.02806988486892514, 0.7998128361456331437 ) ) ;
#94079=CARTESIAN_POINT ( 'NONE',  ( -3.844188154716629668, 7.347496864717369291, 0.5888589343297395695 ) ) ;
#94085=CARTESIAN_POINT ( 'NONE',  ( 7.517069824134078537, 7.734612647770044092, 0.000000000000000000 ) ) ;
#94087=CARTESIAN_POINT ( 'NONE',  ( -6.344338864096334518, 6.859745832460597548, 0.6559349933493059392 ) ) ;
#94094=CARTESIAN_POINT ( 'NONE',  ( 4.206772801990143584, 8.129928378955675328, 0.7998128361456271485 ) ) ;
#94102=CARTESIAN_POINT ( 'NONE',  ( 3.431622278034673901, 7.017660067766835930, -1.734723475976807094E-15 ) ) ;
#94106=CARTESIAN_POINT ( 'NONE',  ( 4.231553341240963384, 7.950912974840849579, -0.7216878364870357165 ) ) ;
#94117=CARTESIAN_POINT ( 'NONE',  ( -4.312902262922974295, 8.045820050136510915, 0.7216878364870338292 ) ) ;
#94123=CARTESIAN_POINT ( 'NONE',  ( 2.975976995527448654, 6.510311277507367045, -0.5630407789675599961 ) ) ;
#94149=CARTESIAN_POINT ( 'NONE',  ( 5.337069745634900997, 6.255611453776062980, 1.199719254218452047 ) ) ;
#94160=CARTESIAN_POINT ( 'NONE',  ( -6.617788377246196951, 7.853746207276256719, -1.082531754730549967 ) ) ;
#94163=CARTESIAN_POINT ( 'NONE',  ( 5.085717018457579286, 6.066329622022862189, -1.082531754730548412 ) ) ;
#94180=ORIENTED_EDGE ( 'NONE', *, *, #146400, .T. ) ;
#94181=CARTESIAN_POINT ( 'NONE',  ( 4.517335436343452137, 8.499999999999996447, 0.7749999999999996891 ) ) ;
#94184=CARTESIAN_POINT ( 'NONE',  ( 6.183927461164522299, 6.387205924212962849, 0.000000000000000000 ) ) ;
#94206=CARTESIAN_POINT ( 'NONE',  ( 5.588068197455647201, 5.804839949401370269, -0.7313310425167540707 ) ) ;
#94215=CARTESIAN_POINT ( 'NONE',  ( -7.075376061485238566, 9.347967719856493218, 1.599625672291269396 ) ) ;
#94216=CARTESIAN_POINT ( 'NONE',  ( -4.636310691425048702, 8.434871236368708836, 0.4628797641644845084 ) ) ;
#94217=CARTESIAN_POINT ( 'NONE',  ( -6.330731382938326490, 6.350551133041632212, 0.7998128361456282587 ) ) ;
#94229=CARTESIAN_POINT ( 'NONE',  ( -5.490125858891038213, 5.369844688319787451, -0.7998128361456362523 ) ) ;
#94235=CARTESIAN_POINT ( 'NONE',  ( -3.179715765502671321, 5.975770656120749535, 2.499999999999999556 ) ) ;
#94237=CARTESIAN_POINT ( 'NONE',  ( -3.011287625495571607, 6.360174617139689346, -0.7852620323503290978 ) ) ;
#94242=CARTESIAN_POINT ( 'NONE',  ( 3.739016502318667445, 7.584212696005614873, 0.7998128361456271485 ) ) ;
#94246=CARTESIAN_POINT ( 'NONE',  ( -5.000000000000013323, 8.499999999999996447, -0.7750000000000013545 ) ) ;
#94248=ORIENTED_EDGE ( 'NONE', *, *, #170147, .T. ) ;
#94265=CARTESIAN_POINT ( 'NONE',  ( 4.667750024854814050, 8.667735138964429709, -0.7998128361456381397 ) ) ;
#94266=CARTESIAN_POINT ( 'NONE',  ( 3.739016502318667445, 7.584212696005614873, 0.7998128361456271485 ) ) ;
#94268=CARTESIAN_POINT ( 'NONE',  ( 5.415556014015861841, 5.282846535965431300, -0.7998128361456481317 ) ) ;
#94278=ORIENTED_EDGE ( 'NONE', *, *, #184994, .F. ) ;
#94280=CARTESIAN_POINT ( 'NONE',  ( -2.974122065066389098, 6.685841390114815042, -0.001386224338680421084 ) ) ;
#94281=CARTESIAN_POINT ( 'NONE',  ( 5.403926048761924505, 7.658933883257522446, 1.327442161737320436 ) ) ;
#94283=CARTESIAN_POINT ( 'NONE',  ( -5.600926855776901192, 5.707038551260711579, -0.7216878364870338292 ) ) ;
#94284=CARTESIAN_POINT ( 'NONE',  ( 4.909461021924256485, 4.900328411765999981, 0.7216878364870338292 ) ) ;
#94290=LINE ( 'NONE', #23911, #73989 ) ;
#94310=CARTESIAN_POINT ( 'NONE',  ( 4.913904330310220558, 4.697586238308844919, 0.000000000000000000 ) ) ;
#94328=CARTESIAN_POINT ( 'NONE',  ( -7.618755976236585958, 7.853246491889623648, 0.000000000000000000 ) ) ;
#94345=CARTESIAN_POINT ( 'NONE',  ( 6.235824307642648279, 6.239826211863360506, 0.000000000000000000 ) ) ;
#94355=CARTESIAN_POINT ( 'NONE',  ( 5.871284023695358734, 7.173991544917035945, 1.145568358895364458 ) ) ;
#94368=CARTESIAN_POINT ( 'NONE',  ( -6.162041457555802459, 6.982316563411976595, 0.9201402841920912623 ) ) ;
#94374=CARTESIAN_POINT ( 'NONE',  ( -4.132202957115018727, 8.042930226601317401, 0.000000000000000000 ) ) ;
#94376=B_SPLINE_CURVE_WITH_KNOTS ( 'NONE', 3,
 ( #69031, #118941, #184921, #36545, #4025, #105871 ),
 .UNSPECIFIED., .F., .F.,
 ( 4, 2, 4 ),
 ( 0.000000000000000000, 0.0003038051859056658437, 0.0006076103718113316874 ),
 .UNSPECIFIED. ) ;
#94377=CARTESIAN_POINT ( 'NONE',  ( 4.199993725183334803, 8.122019456014369254, -0.7998128361456362523 ) ) ;
#94381=CARTESIAN_POINT ( 'NONE',  ( -7.370792787684826486, 8.628288336167626582, -1.199719254218452047 ) ) ;
#94384=CARTESIAN_POINT ( 'NONE',  ( 7.635176783151273128, 8.936736330878529699, 1.199719254218452935 ) ) ;
#94390=CARTESIAN_POINT ( 'NONE',  ( -5.994696786504495556, 7.186261032347766253, -1.212264510017725394 ) ) ;
#94408=CARTESIAN_POINT ( 'NONE',  ( 4.082413651490639062, 7.776916670132135501, 0.000000000000000000 ) ) ;
#94422=CARTESIAN_POINT ( 'NONE',  ( -3.472296738875691346, 6.104744391113324120, 1.082531754730549967 ) ) ;
#94426=CARTESIAN_POINT ( 'NONE',  ( 4.603875680292229156, 7.528882839386387360, 1.199719254218452047 ) ) ;
#94475=VERTEX_POINT ( 'NONE', #125061 ) ;
#94476=CARTESIAN_POINT ( 'NONE',  ( -4.950135482320929370, 5.908151163196758482, -1.082531754730549967 ) ) ;
#94485=CARTESIAN_POINT ( 'NONE',  ( -5.529746549527323474, 7.544733289238903851, -1.599625672291271394 ) ) ;
#94490=ORIENTED_EDGE ( 'NONE', *, *, #122294, .F. ) ;
#94494=CARTESIAN_POINT ( 'NONE',  ( -4.573896719763875574, 6.429575154514868274, -1.599625672291271394 ) ) ;
#94496=CARTESIAN_POINT ( 'NONE',  ( 6.367678427751853221, 6.924687757192571347, 0.8275186136274095272 ) ) ;
#94501=CARTESIAN_POINT ( 'NONE',  ( 5.367048706163317640, 7.354919138647580290, -1.599625672291281386 ) ) ;
#94508=CARTESIAN_POINT ( 'NONE',  ( -7.533490631048818109, 8.818102486758951031, -1.199719254218452047 ) ) ;
#94513=CARTESIAN_POINT ( 'NONE',  ( -5.906512197408906317, 6.919960980845699439, -1.199719254218453823 ) ) ;
#94517=CARTESIAN_POINT ( 'NONE',  ( 6.360183458142179447, 6.592837920686898556, -0.7216878364870458196 ) ) ;
#94518=CARTESIAN_POINT ( 'NONE',  ( -6.089020385868862739, 8.197219431637373432, -1.443375672974066548 ) ) ;
#94522=CARTESIAN_POINT ( 'NONE',  ( 4.570507181582611267, 8.346359121906111511, 0.000000000000000000 ) ) ;
#94525=CARTESIAN_POINT ( 'NONE',  ( 5.987861119090863049, 7.014868056141362551, 1.199719254218452047 ) ) ;
#94526=ORIENTED_EDGE ( 'NONE', *, *, #38147, .T. ) ;
#94528=CARTESIAN_POINT ( 'NONE',  ( -4.916039773278787273, 4.881957280557857715, 0.5603013081572870702 ) ) ;
#94550=CARTESIAN_POINT ( 'NONE',  ( 8.014278199453780616, 8.522615118883788199, 0.000000000000000000 ) ) ;
#94554=CARTESIAN_POINT ( 'NONE',  ( 5.094250900851895025, 7.824382189606214233, 1.140223938556598871 ) ) ;
#94560=CARTESIAN_POINT ( 'NONE',  ( 6.964048179274811012, 8.153752959689313684, 1.199719254218452047 ) ) ;
#94565=CARTESIAN_POINT ( 'NONE',  ( -4.646665375593996394, 8.329970469126573462, 0.4085986083085801912 ) ) ;
#94571=CARTESIAN_POINT ( 'NONE',  ( -5.004368096775595021, 5.971422546727199077, 1.082531754730549078 ) ) ;
#94582=CARTESIAN_POINT ( 'NONE',  ( -2.830620210203090181, 6.524417021870718258, 0.000000000000000000 ) ) ;
#94584=CARTESIAN_POINT ( 'NONE',  ( 5.525830126021535449, 8.604496359403894346, -1.199719254218452047 ) ) ;
#94593=CARTESIAN_POINT ( 'NONE',  ( 4.369470645354133431, 8.319742529546998000, 0.7998128361456271485 ) ) ;
#94596=CARTESIAN_POINT ( 'NONE',  ( 5.275531169048895741, 7.248148678680751189, -1.443375672974078761 ) ) ;
#94606=CARTESIAN_POINT ( 'NONE',  ( -5.896403733238388511, 7.170697087194168873, 1.136063563240964802 ) ) ;
#94610=ORIENTED_EDGE ( 'NONE', *, *, #111774, .T. ) ;
#94613=CARTESIAN_POINT ( 'NONE',  ( -4.553559489343377287, 6.405848385690952718, -1.599625672291271394 ) ) ;
#94614=ADVANCED_FACE ( 'NONE', ( #112002 ), #90965, .T. ) ;
#94615=CARTESIAN_POINT ( 'NONE',  ( 7.078765600110826561, 8.391552967285011988, -1.082531754730548412 ) ) ;
#94627=CARTESIAN_POINT ( 'NONE',  ( -4.925354943514475003, 8.968274210734028529, 0.000000000000000000 ) ) ;
#94628=CARTESIAN_POINT ( 'NONE',  ( -4.125423880308188629, 8.035021303660014880, -0.7998128361456481317 ) ) ;
#94630=CARTESIAN_POINT ( 'NONE',  ( 7.363486825553451354, 8.723727730301414240, -1.082531754730548412 ) ) ;
#94634=CARTESIAN_POINT ( 'NONE',  ( 3.040771591214902259, 6.769593633051179005, -0.7998128361456362523 ) ) ;
#94640=CARTESIAN_POINT ( 'NONE',  ( -5.310352258326699548, 7.640991054048470232, -1.228972953101372223 ) ) ;
#94649=CARTESIAN_POINT ( 'NONE',  ( -6.257970421159510188, 9.458660037064859694, 1.199719254218452047 ) ) ;
#94667=CARTESIAN_POINT ( 'NONE',  ( 5.855142236255289845, 7.924361590421551860, -1.599625672291281386 ) ) ;
#94702=CARTESIAN_POINT ( 'NONE',  ( 4.927462483923885195, 4.713404084191450849, -0.7998128361456481317 ) ) ;
#94730=CARTESIAN_POINT ( 'NONE',  ( -4.782994330570982555, 8.802186828966616972, 0.000000000000000000 ) ) ;
#94732=CARTESIAN_POINT ( 'NONE',  ( 5.953438849732186178, 8.999410187112612647, -1.082531754730548412 ) ) ;
#94737=CARTESIAN_POINT ( 'NONE',  ( -5.829079699232685208, 5.765290835385048496, 0.000000000000000000 ) ) ;
#94742=CARTESIAN_POINT ( 'NONE',  ( -3.851398154733808088, 6.650992392901508232, -1.199719254218450271 ) ) ;
#94749=CARTESIAN_POINT ( 'NONE',  ( -5.692444392891315097, 7.734547439830227411, -1.599625672291271394 ) ) ;
#94758=CARTESIAN_POINT ( 'NONE',  ( -4.634908411025374875, 6.500755460986618495, 1.599625672291263179 ) ) ;
#94763=CARTESIAN_POINT ( 'NONE',  ( -4.638297949650955765, 8.425448351319163365, 0.7216878364870267237 ) ) ;
#94764=CARTESIAN_POINT ( 'NONE',  ( -5.600926855776877211, 9.548515408466085930, -0.7216878364870338292 ) ) ;
#94765=CARTESIAN_POINT ( 'NONE',  ( 6.710359684120930091, 6.793450817754725257, 0.7998128361456352531 ) ) ;
#94766=CARTESIAN_POINT ( 'NONE',  ( -5.824109505522200081, 8.952488968821326054, -1.199719254218452047 ) ) ;
#94803=CARTESIAN_POINT ( 'NONE',  ( 4.624709440338444111, 8.453137518702421360, 0.3515692964491355932 ) ) ;
#94816=CARTESIAN_POINT ( 'NONE',  ( 5.338878628731272613, 9.450718510153643948, -0.7998128361456481317 ) ) ;
#94819=CARTESIAN_POINT ( 'NONE',  ( -5.167592825464113915, 6.057888380243431570, 1.199719254218452935 ) ) ;
#94823=CARTESIAN_POINT ( 'NONE',  ( -7.878696662872776812, 8.364436659539265406, -0.7216878364870338292 ) ) ;
#94834=CARTESIAN_POINT ( 'NONE',  ( 4.004454267989866700, 5.765225627445230927, 1.599625672291262513 ) ) ;
#94835=CARTESIAN_POINT ( 'NONE',  ( 5.342795052237045539, 8.390955439988655229, -1.199719254218450271 ) ) ;
#94843=CARTESIAN_POINT ( 'NONE',  ( 5.110497557708379546, 4.926945003606695295, -0.7998128361456481317 ) ) ;
#94849=CARTESIAN_POINT ( 'NONE',  ( 5.875479466675786355, 7.948088359245467416, -1.599625672291283607 ) ) ;
#94850=VERTEX_POINT ( 'NONE', #84704 ) ;
#94861=CARTESIAN_POINT ( 'NONE',  ( -4.773879485787619892, 7.623257595843924150, 1.082531754730549967 ) ) ;
#94863=CARTESIAN_POINT ( 'NONE',  ( -6.936931872047518155, 8.122117267924091166, 1.199719254218452047 ) ) ;
#94876=CARTESIAN_POINT ( 'NONE',  ( -3.984117037569407938, 5.741498858621315371, 1.599625672291270506 ) ) ;
#94877=CARTESIAN_POINT ( 'NONE',  ( 6.984385409695311964, 8.177479728513226576, 1.199719254218452935 ) ) ;
#94880=CARTESIAN_POINT ( 'NONE',  ( 4.597623488365603528, 5.496887170248887067, -1.082531754730548412 ) ) ;
#94895=CYLINDRICAL_SURFACE ( 'NONE', #207657, 1.250000000000000000 ) ;
#94896=CARTESIAN_POINT ( 'NONE',  ( -0.4800000000000244071, 2.999999999999999112, 2.420000000000000373 ) ) ;
#94898=CARTESIAN_POINT ( 'NONE',  ( 5.574337433874081427, 6.532423756721743580, -1.199719254218452047 ) ) ;
#94900=CARTESIAN_POINT ( 'NONE',  ( -4.142898457427624415, 6.991076079377632091, 1.199719254218452935 ) ) ;
#94904=CARTESIAN_POINT ( 'NONE',  ( 4.899292406491845497, 6.809203455697518947, -1.599625672291273171 ) ) ;
#94911=ADVANCED_FACE ( 'NONE', ( #170214 ), #23954, .T. ) ;
#94916=CARTESIAN_POINT ( 'NONE',  ( 5.722950238744187956, 9.690876021928001904, 0.7216878364870317197 ) ) ;
#94918=CARTESIAN_POINT ( 'NONE',  ( -7.130662446144611977, 7.283804040115648526, 0.000000000000000000 ) ) ;
#94919=CARTESIAN_POINT ( 'NONE',  ( 3.379725431556547477, 7.165039780116438273, -1.734723475976807094E-15 ) ) ;
#94929=CARTESIAN_POINT ( 'NONE',  ( -4.098307573080856692, 8.003385611894792362, 0.7998128361456352531 ) ) ;
#94955=CARTESIAN_POINT ( 'NONE',  ( 3.906157654512984134, 7.571284673658201569, -0.7216878364870338292 ) ) ;
#94960=DIRECTION ( 'NONE',  ( 0.7978120914393141971, 0.6029061840396293670, 0.000000000000000000 ) ) ;
#94961=CARTESIAN_POINT ( 'NONE',  ( 5.085717018457579286, 6.066329622022862189, -1.082531754730548412 ) ) ;
#94967=TOROIDAL_SURFACE ( 'NONE', #1520, 0.8299999999999999600, 0.08000000000000000167 ) ;
#94975=CARTESIAN_POINT ( 'NONE',  ( -6.479871072688648148, 6.524547437750345402, 0.000000000000000000 ) ) ;
#94977=CARTESIAN_POINT ( 'NONE',  ( -5.725286006720766707, 9.901527117808042178, 0.7998128361456291469 ) ) ;
#94990=CARTESIAN_POINT ( 'NONE',  ( -6.017840079619296567, 8.114175741012878973, -1.599625672291271394 ) ) ;
#94996=CARTESIAN_POINT ( 'NONE',  ( -4.502716413514310290, 6.346531463890372926, -1.443375672974066548 ) ) ;
#95000=CARTESIAN_POINT ( 'NONE',  ( -6.310394152517827315, 6.326824364217716656, 0.7998128361456281477 ) ) ;
#95019=CARTESIAN_POINT ( 'NONE',  ( -7.306918443122272677, 7.489436036589583345, 0.7998128361456341429 ) ) ;
#95021=CARTESIAN_POINT ( 'NONE',  ( -4.492547798081878874, 6.334668079219206049, 1.599625672291263179 ) ) ;
#95022=ORIENTED_EDGE ( 'NONE', *, *, #25859, .F. ) ;
#95046=CARTESIAN_POINT ( 'NONE',  ( -5.769876891067536206, 8.889217585290882795, 1.199719254218454489 ) ) ;
#95048=EDGE_LOOP ( 'NONE', ( #209268, #99788, #57330, #107558, #77283, #68687, #38603 ) ) ;
#95055=CARTESIAN_POINT ( 'NONE',  ( 3.921423297084294823, 8.995353878514519508, 0.7749999999999996891 ) ) ;
#95060=AXIS2_PLACEMENT_3D ( 'NONE', #75981, #93325, #24013 ) ;
#95074=CARTESIAN_POINT ( 'NONE',  ( 6.502017186205484300, 9.743381262951846367, -1.199719254218452047 ) ) ;
#95076=CARTESIAN_POINT ( 'NONE',  ( 7.289443866002793371, 8.533381260871966134, 1.199719254218452047 ) ) ;
#95090=CARTESIAN_POINT ( 'NONE',  ( 5.960708871395055120, 7.108654626955757116, 1.090683939682752124 ) ) ;
#95092=CARTESIAN_POINT ( 'NONE',  ( 6.875393295905841917, 7.193916064744513506, 0.000000000000000000 ) ) ;
#95098=CARTESIAN_POINT ( 'NONE',  ( -5.123001941117347080, 7.070197912760590064, 1.599625672291263179 ) ) ;
#95104=CARTESIAN_POINT ( 'NONE',  ( -5.926322542504872892, 8.007405281046052536, -1.443375672974066548 ) ) ;
#95114=CARTESIAN_POINT ( 'NONE',  ( -3.984117037569407938, 5.741498858621315371, 1.599625672291270506 ) ) ;
#95124=CARTESIAN_POINT ( 'NONE',  ( 7.075376061485196821, 9.347967719856493218, 1.599625672291268286 ) ) ;
#95128=VERTEX_POINT ( 'NONE', #205710 ) ;
#95141=CARTESIAN_POINT ( 'NONE',  ( -6.994027139803241866, 9.253060644560830994, -1.599625672291271394 ) ) ;
#95144=CARTESIAN_POINT ( 'NONE',  ( 7.530627977747744062, 7.750430493652658015, -0.7998128361456341429 ) ) ;
#95145=CARTESIAN_POINT ( 'NONE',  ( 7.013428937081407355, 5.939655416065874327, -2.436399677959149468 ) ) ;
#95146=CARTESIAN_POINT ( 'NONE',  ( -6.041007162748570636, 7.066593642038220935, 1.036256717389577586 ) ) ;
#95152=CARTESIAN_POINT ( 'NONE',  ( 5.879395890181562834, 6.888325289080478697, -1.199719254218452047 ) ) ;
#95156=CARTESIAN_POINT ( 'NONE',  ( -5.579056995618064008, 5.838737027418012815, -0.5808829061496860735 ) ) ;
#95162=CARTESIAN_POINT ( 'NONE',  ( 2.957086901556340575, 6.464035461875470290, 0.7216878364870257245 ) ) ;
#95166=CARTESIAN_POINT ( 'NONE',  ( 5.722950238744209273, 6.809768379023969587, 1.082531754730549967 ) ) ;
#95167=VERTEX_POINT ( 'NONE', #28041 ) ;
#95174=CARTESIAN_POINT ( 'NONE',  ( -8.014278199453791274, 8.522615118883788199, 1.530808498934192557E-16 ) ) ;
#95177=CARTESIAN_POINT ( 'NONE',  ( -5.641601317062247212, 7.675230518029648508, -1.443375672974066548 ) ) ;
#95198=CARTESIAN_POINT ( 'NONE',  ( 4.098537063712264228, 7.253343185014818673, 1.055677455976588686 ) ) ;
#95210=CARTESIAN_POINT ( 'NONE',  ( 6.364626766972446781, 6.390095747748157251, 0.7998128361456352531 ) ) ;
#95212=CARTESIAN_POINT ( 'NONE',  ( 4.850785098639300408, 8.881276058379668825, -0.7998128361456481317 ) ) ;
#95216=CARTESIAN_POINT ( 'NONE',  ( 0.000000000000000000, 0.000000000000000000, 0.000000000000000000 ) ) ;
#95223=CARTESIAN_POINT ( 'NONE',  ( -7.770231434407805615, 8.237893892996801526, 0.000000000000000000 ) ) ;
#95226=CARTESIAN_POINT ( 'NONE',  ( 3.973948422136968084, 5.729635473950147606, -1.443375672974068769 ) ) ;
#95237=CARTESIAN_POINT ( 'NONE',  ( 5.526144005543697446, 7.442112546579989996, -1.248357989223557452 ) ) ;
#95244=CARTESIAN_POINT ( 'NONE',  ( -4.828112100242283766, 7.686528979374367410, -1.082531754730549967 ) ) ;
#95246=CARTESIAN_POINT ( 'NONE',  ( -3.838366886444665393, 7.492195444245147939, 0.000000000000000000 ) ) ;
#95284=CARTESIAN_POINT ( 'NONE',  ( -7.774674742793745708, 8.035151719539642912, 0.7998128361456341429 ) ) ;
#95285=CARTESIAN_POINT ( 'NONE',  ( -5.066182726705734218, 7.967045547422810792, 1.194666625917781611 ) ) ;
#95290=CARTESIAN_POINT ( 'NONE',  ( -6.522881301506166629, 9.663759714182251770, 1.082531754730549967 ) ) ;
#95291=B_SPLINE_CURVE_WITH_KNOTS ( 'NONE', 3,
 ( #174616, #54442, #92307, #120584, #203859, #7799, #171382, #137837, #154077, #106442 ),
 .UNSPECIFIED., .F., .F.,
 ( 4, 3, 3, 4 ),
 ( 0.000000000000000000, 3.125146907026659298E-05, 6.069395767275096592E-05, 9.014634065022558457E-05 ),
 .UNSPECIFIED. ) ;
#95297=CARTESIAN_POINT ( 'NONE',  ( -3.969505113751027547, 7.853116076009993840, 1.214306433183764966E-14 ) ) ;
#95303=CARTESIAN_POINT ( 'NONE',  ( -6.468692700515624949, 6.719432036793461904, 1.751973777778555601E-06 ) ) ;
#95310=CARTESIAN_POINT ( 'NONE',  ( 6.073126464278658432, 6.050012061272033392, 0.000000000000000000 ) ) ;
#95336=CARTESIAN_POINT ( 'NONE',  ( 5.692444392891300886, 7.734547439830227411, -1.599625672291281386 ) ) ;
#95337=CARTESIAN_POINT ( 'NONE',  ( 4.061549535745618833, 6.896169004081968090, -1.199719254218452047 ) ) ;
#95351=CARTESIAN_POINT ( 'NONE',  ( 4.595358334023878832, 8.489709390108890474, -0.01759220550971198060 ) ) ;
#95352=CARTESIAN_POINT ( 'NONE',  ( -5.112833325684916552, 7.058334528089422300, -1.443375672974066548 ) ) ;
#95353=CARTESIAN_POINT ( 'NONE',  ( 4.584065335196271462, 5.481069324884694005, 1.082531754730549078 ) ) ;
#95380=CARTESIAN_POINT ( 'NONE',  ( 4.746236293235721604, 7.694970221153795364, 1.199719254218451159 ) ) ;
#95399=CARTESIAN_POINT ( 'NONE',  ( -7.456058132872594335, 7.663432341298296535, 0.000000000000000000 ) ) ;
#95410=CARTESIAN_POINT ( 'NONE',  ( 5.367048706163317640, 7.354919138647580290, -1.599625672291281386 ) ) ;
#95416=CARTESIAN_POINT ( 'NONE',  ( 5.468734858265785093, 7.473552982767158070, 1.599625672291269396 ) ) ;
#95428=CARTESIAN_POINT ( 'NONE',  ( 4.633164669693822901, 8.325607986553848150, 0.3865003237762173471 ) ) ;
#95438=CARTESIAN_POINT ( 'NONE',  ( 5.206133053153118695, 6.319824444209305447, 1.213385250716643604 ) ) ;
#95446=ORIENTED_EDGE ( 'NONE', *, *, #115968, .F. ) ;
#95450=CARTESIAN_POINT ( 'NONE',  ( -4.932134020321308654, 8.976183133675331050, 0.7998128361456291469 ) ) ;
#95452=CARTESIAN_POINT ( 'NONE',  ( 4.376249722160992839, 8.327651452488305850, 0.000000000000000000 ) ) ;
#95453=CARTESIAN_POINT ( 'NONE',  ( -4.028292277495545193, 3.858391361152785581, 2.500000000000000000 ) ) ;
#95457=CARTESIAN_POINT ( 'NONE',  ( -7.422162748838431412, 7.623887726591770608, -0.7998128361456362523 ) ) ;
#95460=CARTESIAN_POINT ( 'NONE',  ( 6.933015448541703485, 9.181880338089085214, 1.599625672291268286 ) ) ;
#95466=CARTESIAN_POINT ( 'NONE',  ( -6.245422037512663671, 7.006708691962935553, -1.003398212925192157 ) ) ;
#95479=ORIENTED_EDGE ( 'NONE', *, *, #200733, .F. ) ;
#95483=CARTESIAN_POINT ( 'NONE',  ( 7.187230829020130329, 7.557726520044554697, 0.7216878364870267237 ) ) ;
#95497=CARTESIAN_POINT ( 'NONE',  ( -5.017926250833627755, 5.026871178826882947, 0.7216878364870257245 ) ) ;
#95501=CARTESIAN_POINT ( 'NONE',  ( 3.413620815590684199, 7.204584394822967752, 0.7998128361456281477 ) ) ;
#95549=CARTESIAN_POINT ( 'NONE',  ( -5.465345319640241506, 5.548860092434608760, 0.7216878364870257245 ) ) ;
#95551=B_SPLINE_CURVE_WITH_KNOTS ( 'NONE', 3,
 ( #145949, #26822, #162178, #95055, #194657, #161105, #10567 ),
 .UNSPECIFIED., .F., .F.,
 ( 4, 3, 4 ),
 ( 0.000000000000000000, 2.778074687866575757E-05, 5.739355541052443402E-05 ),
 .UNSPECIFIED. ) ;
#95556=CARTESIAN_POINT ( 'NONE',  ( -3.962726036944197894, 7.845207153068690431, -0.7998128361456481317 ) ) ;
#95566=CARTESIAN_POINT ( 'NONE',  ( -4.522526758610270647, 7.433975764090723359, -1.199719254218453823 ) ) ;
#95568=CARTESIAN_POINT ( 'NONE',  ( 6.569431593124095414, 6.790062804044275424, 0.3413723397009699734 ) ) ;
#95573=CARTESIAN_POINT ( 'NONE',  ( 5.692444392891300886, 7.734547439830227411, -1.599625672291281386 ) ) ;
#95581=CARTESIAN_POINT ( 'NONE',  ( -3.654804927335652209, 6.421633627603656080, 1.199719254218452935 ) ) ;
#95586=CARTESIAN_POINT ( 'NONE',  ( -4.990283058281743678, 7.979691447040783814, -1.199719254218453823 ) ) ;
#95590=CARTESIAN_POINT ( 'NONE',  ( 5.790741006368192778, 8.809596036521288198, -1.082531754730548412 ) ) ;
#95593=CARTESIAN_POINT ( 'NONE',  ( -6.604230223188181093, 6.877559146573883453, 0.7216878364870317197 ) ) ;
#95597=CARTESIAN_POINT ( 'NONE',  ( -6.459533842268148973, 6.500820668926428958, 0.000000000000000000 ) ) ;
#95600=CARTESIAN_POINT ( 'NONE',  ( 5.903649544107831382, 5.852288987739402870, -0.7998128361456481317 ) ) ;
#95606=CARTESIAN_POINT ( 'NONE',  ( 6.391743074199809804, 6.421731439513382433, -0.7998128361456481317 ) ) ;
#95628=CARTESIAN_POINT ( 'NONE',  ( 4.596293493935747598, 8.372084169494645067, 0.08663659024946840370 ) ) ;
#95636=CARTESIAN_POINT ( 'NONE',  ( 6.343235766347262938, 8.493804042195527870, -1.599625672291281386 ) ) ;
#95637=VERTEX_POINT ( 'NONE', #42044 ) ;
#95641=CARTESIAN_POINT ( 'NONE',  ( -4.606532530031762995, 8.380852375923623754, -0.1178885281021696541 ) ) ;
#95648=CARTESIAN_POINT ( 'NONE',  ( -3.133342898089680695, 6.669667457830990465, 0.7216878364870338292 ) ) ;
#95651=( BOUNDED_CURVE ( )  B_SPLINE_CURVE ( 2, ( #167074, #145536, #132476 ),
 .UNSPECIFIED., .F., .T. ) 
 B_SPLINE_CURVE_WITH_KNOTS ( ( 3, 3 ),
 ( 0.000000000000000000, 0.005017554178699702196 ),
 .UNSPECIFIED. ) 
 CURVE ( )  GEOMETRIC_REPRESENTATION_ITEM ( )  RATIONAL_B_SPLINE_CURVE ( ( 1.000000000000000000, 0.9193330245902806563, 0.9358062698725861939 ) ) 
 REPRESENTATION_ITEM ( '' )  );
#95659=CARTESIAN_POINT ( 'NONE',  ( -3.156015896931072540, 6.904045323053366268, 0.000000000000000000 ) ) ;
#95668=CARTESIAN_POINT ( 'NONE',  ( 4.797606254389322089, 6.690569611577942943, 1.599625672291268286 ) ) ;
#95670=CARTESIAN_POINT ( 'NONE',  ( 4.041739190205284160, 7.729463131965888856, 0.000000000000000000 ) ) ;
#95684=CARTESIAN_POINT ( 'NONE',  ( -5.483346782084204563, 5.361935765378481378, 0.000000000000000000 ) ) ;
#95685=CARTESIAN_POINT ( 'NONE',  ( 3.715816618597135523, 6.492813934075403637, -1.199719254218453823 ) ) ;
#95695=CARTESIAN_POINT ( 'NONE',  ( -6.394605727500880299, 7.489403432619674561, -1.199719254218452047 ) ) ;
#95696=CARTESIAN_POINT ( 'NONE',  ( 5.559725510055676168, 8.644040974110419384, 1.199719254218451159 ) ) ;
#95698=CARTESIAN_POINT ( 'NONE',  ( 6.983858524370782028, 8.280828045588322084, 1.082531754730549967 ) ) ;
#95704=CARTESIAN_POINT ( 'NONE',  ( 3.054329744828568227, 6.785411478933790264, 0.000000000000000000 ) ) ;
#95711=CARTESIAN_POINT ( 'NONE',  ( -6.005252172667468358, 7.091917859149008407, -1.064983193601161338 ) ) ;
#95720=CARTESIAN_POINT ( 'NONE',  ( -6.084577077482911101, 10.32070003369722144, 0.000000000000000000 ) ) ;
#95733=FACE_OUTER_BOUND ( 'NONE', #101230, .T. ) ;
#95738=CARTESIAN_POINT ( 'NONE',  ( 7.205232291019763480, 7.370802192470005565, -0.7998128361456341429 ) ) ;
#95769=CARTESIAN_POINT ( 'NONE',  ( 3.203469434578891661, 6.959407783642502565, -0.7998128361456362523 ) ) ;
#95770=CARTESIAN_POINT ( 'NONE',  ( -3.201133666602369310, 6.748756687762456963, -0.7216878364870458196 ) ) ;
#95783=PLANE ( 'NONE',  #143491 ) ;
#95798=ORIENTED_EDGE ( 'NONE', *, *, #125182, .T. ) ;
#95799=CARTESIAN_POINT ( 'NONE',  ( -6.317173229324657413, 6.334733287159020954, 0.000000000000000000 ) ) ;
#95801=CARTESIAN_POINT ( 'NONE',  ( 6.997416677984476863, 7.336276677169590421, 0.000000000000000000 ) ) ;
#95806=CARTESIAN_POINT ( 'NONE',  ( -5.818384198920079520, 6.817144982608731141, 1.199719254218452935 ) ) ;
#95811=CARTESIAN_POINT ( 'NONE',  ( -5.144392941742557568, 4.966489618313220333, -0.7998128361456362523 ) ) ;
#95816=CARTESIAN_POINT ( 'NONE',  ( -4.990283058281743678, 7.979691447040783814, -1.199719254218453823 ) ) ;
#95828=CARTESIAN_POINT ( 'NONE',  ( -3.634467696915153034, 6.397906858779740524, 1.199719254218452935 ) ) ;
#95832=CARTESIAN_POINT ( 'NONE',  ( -4.977251789992602760, 8.820894498384422633, 0.000000000000000000 ) ) ;
#95833=CARTESIAN_POINT ( 'NONE',  ( -5.926322542504864899, 8.967774495347393682, -1.082531754730549967 ) ) ;
#95834=CARTESIAN_POINT ( 'NONE',  ( 8.174640274396848483, 8.501778173076651512, 0.7998128361456291469 ) ) ;
#95836=CARTESIAN_POINT ( 'NONE',  ( -6.257970421159510188, 9.458660037064859694, 1.199719254218452047 ) ) ;
#95875=CARTESIAN_POINT ( 'NONE',  ( 5.142555292688428814, 7.778213139218437711, -1.168464917166486039 ) ) ;
#95891=CARTESIAN_POINT ( 'NONE',  ( 5.875479466675786355, 7.948088359245467416, -1.599625672291283607 ) ) ;
#95894=CARTESIAN_POINT ( 'NONE',  ( -4.142898457427624415, 6.991076079377632091, 1.199719254218452935 ) ) ;
#95898=CARTESIAN_POINT ( 'NONE',  ( -6.902509602688821744, 8.185920970292658083, -1.082531754730549967 ) ) ;
#95908=CARTESIAN_POINT ( 'NONE',  ( 4.736594563127852098, 6.619389305106191834, -1.599625672291273171 ) ) ;
#95909=CARTESIAN_POINT ( 'NONE',  ( 5.987861119090863049, 7.014868056141362551, 1.199719254218452047 ) ) ;
#95923=VERTEX_POINT ( 'NONE', #110290 ) ;
#95924=CARTESIAN_POINT ( 'NONE',  ( 5.794130544993763898, 7.853181283949808744, 1.599625672291269396 ) ) ;
#95935=CARTESIAN_POINT ( 'NONE',  ( -3.851925040058333582, 7.508013290127760087, -0.7216878364870458196 ) ) ;
#95936=CARTESIAN_POINT ( 'NONE',  ( 4.529832720741620022, 7.338536369956936589, -1.082531754730548412 ) ) ;
#95949=CARTESIAN_POINT ( 'NONE',  ( -7.295696057929500711, 7.684269287105433222, 0.7216878364870317197 ) ) ;
#95950=CARTESIAN_POINT ( 'NONE',  ( 6.851666526859736983, 9.086973262793417661, -1.599625672291269396 ) ) ;
#95953=CARTESIAN_POINT ( 'NONE',  ( 4.434925645001613681, 5.307073019657559065, -1.082531754730548412 ) ) ;
#95956=ORIENTED_EDGE ( 'NONE', *, *, #139645, .T. ) ;
#95970=CARTESIAN_POINT ( 'NONE',  ( 6.225128807330042591, 7.291680359087043151, -1.199719254218452047 ) ) ;
#95973=CARTESIAN_POINT ( 'NONE',  ( -4.899292406491858820, 6.809203455697518947, -1.599625672291271394 ) ) ;
#95981=CARTESIAN_POINT ( 'NONE',  ( 4.740893929121448025, 8.308742936830851633, 0.7931989123739242586 ) ) ;
#95985=CARTESIAN_POINT ( 'NONE',  ( 5.560252395380198998, 9.501061871336672127, 0.7216878364870317197 ) ) ;
#95987=CARTESIAN_POINT ( 'NONE',  ( -7.442499979258930587, 7.647614495415686164, -0.7998128361456362523 ) ) ;
#95988=CARTESIAN_POINT ( 'NONE',  ( 5.529746549527311039, 7.544733289238903851, -1.599625672291281386 ) ) ;
#95996=CARTESIAN_POINT ( 'NONE',  ( -6.120580001926503755, 6.105374521861167914, -0.7998128361456362523 ) ) ;
#95999=CARTESIAN_POINT ( 'NONE',  ( -0.3911212198684586583, 3.085581642975291139, 2.026362403383771937 ) ) ;
#96025=B_SPLINE_CURVE_WITH_KNOTS ( 'NONE', 3,
 ( #114341, #62319, #45024, #163030, #112207, #13558 ),
 .UNSPECIFIED., .F., .F.,
 ( 4, 2, 4 ),
 ( 0.000000000000000000, 0.5000000000000000000, 1.000000000000000000 ),
 .UNSPECIFIED. ) ;
#96027=CARTESIAN_POINT ( 'NONE',  ( 5.587368702607580673, 5.691220705896524734, -0.7216878364870458196 ) ) ;
#96028=ORIENTED_EDGE ( 'NONE', *, *, #125182, .F. ) ;
#96033=CARTESIAN_POINT ( 'NONE',  ( 5.519577934094861860, 6.572500690266394940, 1.082531754730549078 ) ) ;
#96045=CARTESIAN_POINT ( 'NONE',  ( -6.038177310039794854, 8.137902509836795417, -1.599625672291271394 ) ) ;
#96047=CARTESIAN_POINT ( 'NONE',  ( -6.587282531393266360, 8.778525268082516320, 1.599625672291269396 ) ) ;
#96053=CARTESIAN_POINT ( 'NONE',  ( 7.147083253059300922, 8.367293879104554577, 1.199719254218452935 ) ) ;
#96058=CARTESIAN_POINT ( 'NONE',  ( -5.261446130555064826, 8.296048364692991228, 1.199719254218452935 ) ) ;
#96063=( BOUNDED_CURVE ( )  B_SPLINE_CURVE ( 2, ( #33175, #134964, #49431 ),
 .UNSPECIFIED., .F., .T. ) 
 B_SPLINE_CURVE_WITH_KNOTS ( ( 3, 3 ),
 ( 0.5176136498557766252, 0.5249999999999998002 ),
 .UNSPECIFIED. ) 
 CURVE ( )  GEOMETRIC_REPRESENTATION_ITEM ( )  RATIONAL_B_SPLINE_CURVE ( ( 0.9730109806173230513, 0.8812500066305124502, 0.9999999999999964473 ) ) 
 REPRESENTATION_ITEM ( '' )  );
#96065=CARTESIAN_POINT ( 'NONE',  ( -4.746763178560296836, 6.631252689777363152, 1.443375672974058777 ) ) ;
#96068=CARTESIAN_POINT ( 'NONE',  ( -5.957882158562513908, 5.915560371269843465, -0.7998128361456362523 ) ) ;
#96088=CARTESIAN_POINT ( 'NONE',  ( -3.648552735408990166, 6.310376387068841630, -1.082531754730546636 ) ) ;
#96089=CARTESIAN_POINT ( 'NONE',  ( 3.736153849017632922, 6.516540702899320081, -1.199719254218453823 ) ) ;
#96091=CARTESIAN_POINT ( 'NONE',  ( -3.793249116773374396, 7.647484079536056356, 0.7998128361456352531 ) ) ;
#96100=CARTESIAN_POINT ( 'NONE',  ( 4.055297343818932809, 7.745280977848486792, 0.7216878364870341622 ) ) ;
#96115=CARTESIAN_POINT ( 'NONE',  ( -7.618755976236585958, 7.853246491889623648, 0.000000000000000000 ) ) ;
#96130=CIRCLE ( 'NONE', #16597, 0.4000000000000001332 ) ;
#96144=CARTESIAN_POINT ( 'NONE',  ( 5.826972158823246595, 10.02016096192762085, -0.7998128361456481317 ) ) ;
#96145=CARTESIAN_POINT ( 'NONE',  ( 7.666209513884374438, 7.908608952478760834, 0.7998128361456281477 ) ) ;
#96159=CARTESIAN_POINT ( 'NONE',  ( 6.003728048595398548, 7.077753126805482076, 1.059392881431284961 ) ) ;
#96161=CARTESIAN_POINT ( 'NONE',  ( 7.526184669361807522, 7.953172667109813077, 0.000000000000000000 ) ) ;
#96168=CARTESIAN_POINT ( 'NONE',  ( -3.461074353238556167, 7.259946855412102273, 0.000000000000000000 ) ) ;
#96174=CARTESIAN_POINT ( 'NONE',  ( -5.736508391913536897, 9.706693867292189637, 0.7216878364870267237 ) ) ;
#96177=CARTESIAN_POINT ( 'NONE',  ( -4.790662068211312352, 6.933575286401571169, 1.250027526764455388 ) ) ;
#96181=CARTESIAN_POINT ( 'NONE',  ( -5.008811405605897882, 4.808311159487113073, 0.7998128361456281477 ) ) ;
#96191=CARTESIAN_POINT ( 'NONE',  ( 7.506374323821472849, 8.786466794993730289, -1.199719254218452047 ) ) ;
#96213=CARTESIAN_POINT ( 'NONE',  ( 5.830888582329017744, 8.960397891762626799, -1.199719254218452047 ) ) ;
#96215=CARTESIAN_POINT ( 'NONE',  ( -5.819752210671484960, 7.227523004248635807, 1.175121323085267289 ) ) ;
#96221=CARTESIAN_POINT ( 'NONE',  ( 6.201928923608456046, 6.200281597156833691, 0.7998128361456352531 ) ) ;
#96224=CARTESIAN_POINT ( 'NONE',  ( -5.586581854188635177, 5.810800913040471194, -0.4357733342581562863 ) ) ;
#96228=CARTESIAN_POINT ( 'NONE',  ( 4.746763178560261309, 5.670883475476017566, 1.082531754730549078 ) ) ;
#96232=CARTESIAN_POINT ( 'NONE',  ( 7.377044979611483200, 7.779176362401098999, -0.7216878364870317197 ) ) ;
#96242=CARTESIAN_POINT ( 'NONE',  ( -6.807602527837528505, 7.114826835331461652, 0.7216878364870317197 ) ) ;
#96266=CARTESIAN_POINT ( 'NONE',  ( 5.599506603007033512, 5.747200726622710754, 0.6510759304539673886 ) ) ;
#96269=AXIS2_PLACEMENT_3D ( 'NONE', #96404, #162454, #46575 ) ;
#96278=CARTESIAN_POINT ( 'NONE',  ( 6.150558962454855561, 7.204682206732687000, 1.199719254218452047 ) ) ;
#96280=CARTESIAN_POINT ( 'NONE',  ( 6.249382461256315580, 6.255644057745969988, -0.7998128361456481317 ) ) ;
#96291=CARTESIAN_POINT ( 'NONE',  ( -2.986538976760251263, 6.706322249520737522, -0.7998128361456481317 ) ) ;
#96294=CARTESIAN_POINT ( 'NONE',  ( 3.729901657090938460, 7.365652676665848553, 0.7216878364870257245 ) ) ;
#96307=CARTESIAN_POINT ( 'NONE',  ( -5.424670859243583720, 8.382514198209223721, 1.082531754730550855 ) ) ;
#96309=CARTESIAN_POINT ( 'NONE',  ( -5.072158865288277418, 7.010880990960010273, 1.443375672974058777 ) ) ;
#96326=CARTESIAN_POINT ( 'NONE',  ( -4.496464221587651799, 5.274905009054215554, 1.199719254218452935 ) ) ;
#96337=CARTESIAN_POINT ( 'NONE',  ( -4.842197138736131556, 5.678260079060780008, 1.199719254218452935 ) ) ;
#96348=CARTESIAN_POINT ( 'NONE',  ( -8.100070429521727178, 8.414780020722290033, 0.7998128361456341429 ) ) ;
#96349=CARTESIAN_POINT ( 'NONE',  ( -5.535867093699859964, 7.544539992772745229, 1.349747212490030046 ) ) ;
#96354=LINE ( 'NONE', #144061, #203026 ) ;
#96357=CARTESIAN_POINT ( 'NONE',  ( -4.197131071882288289, 7.054347462908075350, -1.199719254218455378 ) ) ;
#96361=CARTESIAN_POINT ( 'NONE',  ( -3.318713740295064163, 7.093859473644694269, 0.000000000000000000 ) ) ;
#96370=VERTEX_POINT ( 'NONE', #85173 ) ;
#96373=CARTESIAN_POINT ( 'NONE',  ( 6.412080304620304538, 6.445458208337293549, -0.7998128361456481317 ) ) ;
#96387=CARTESIAN_POINT ( 'NONE',  ( 5.073973250452978867, 4.884333311808733313, 0.1550835458496209185 ) ) ;
#96398=CARTESIAN_POINT ( 'NONE',  ( 6.717138760927786834, 6.801359740696030443, -0.7998128361456481317 ) ) ;
#96399=CARTESIAN_POINT ( 'NONE',  ( 5.571474780572990504, 5.464751763615448787, 0.7998128361456352531 ) ) ;
#96401=CARTESIAN_POINT ( 'NONE',  ( 4.927462483923885195, 4.713404084191450849, -0.7998128361456481317 ) ) ;
#96404=CARTESIAN_POINT ( 'NONE',  ( -7.065207446497166366, 9.336104335703744539, 0.000000000000000000 ) ) ;
#96414=CARTESIAN_POINT ( 'NONE',  ( 4.617922728991994852, 8.461530327540957686, 0.3091873533234041904 ) ) ;
#96415=CARTESIAN_POINT ( 'NONE',  ( -4.787437638956920871, 8.599444655509458357, -0.7216878364870338292 ) ) ;
#96416=CARTESIAN_POINT ( 'NONE',  ( -3.147653791585727667, 8.920000000000001705, 2.499999999999999556 ) ) ;
#96445=CARTESIAN_POINT ( 'NONE',  ( 4.203910148689107729, 7.062256385849379647, -1.199719254218448494 ) ) ;
#96449=VERTEX_POINT ( 'NONE', #103568 ) ;
#96465=CARTESIAN_POINT ( 'NONE',  ( -8.106849506328558164, 8.422688943663599659, 0.000000000000000000 ) ) ;
#96470=CARTESIAN_POINT ( 'NONE',  ( 4.858757509019037357, 5.629766575900002401, 2.420000000000000373 ) ) ;
#96478=CARTESIAN_POINT ( 'NONE',  ( 4.830447868218803897, 8.857549289555754157, -0.7998128361456481317 ) ) ;
#96483=CARTESIAN_POINT ( 'NONE',  ( 4.701645408888975197, 8.707279753670952971, 0.000000000000000000 ) ) ;
#96494=CARTESIAN_POINT ( 'NONE',  ( 4.604167169973131912, 8.362045362587558373, -0.1994984680026238300 ) ) ;
#96506=CARTESIAN_POINT ( 'NONE',  ( -6.118005967093342434, 7.012694018530115869, 0.9664715254068743100 ) ) ;
#96514=CARTESIAN_POINT ( 'NONE',  ( -6.479871072688648148, 6.524547437750345402, 0.000000000000000000 ) ) ;
#96516=CARTESIAN_POINT ( 'NONE',  ( 6.723917837734620484, 6.809268663637336516, 0.000000000000000000 ) ) ;
#96520=CARTESIAN_POINT ( 'NONE',  ( -5.887983850084758330, 10.09134126839936840, 0.7998128361456291469 ) ) ;
#96527=CARTESIAN_POINT ( 'NONE',  ( -0.3583907109357110099, 2.793873605144960859, -2.035334756721693061 ) ) ;
#96537=EDGE_CURVE ( 'NONE', #136572, #35662, #124852, .T. ) ;
#96539=CARTESIAN_POINT ( 'NONE',  ( 6.966220764712121927, 6.002124920821316323, 2.500000000000000444 ) ) ;
#96544=CARTESIAN_POINT ( 'NONE',  ( 5.885648082108190238, 7.959951743916638733, 1.443375672974065660 ) ) ;
#96559=CARTESIAN_POINT ( 'NONE',  ( -5.167065940583949413, 5.200867483535597913, 0.000000000000000000 ) ) ;
#96562=CARTESIAN_POINT ( 'NONE',  ( 3.576318658954677598, 7.394398545414291313, 0.7998128361456281477 ) ) ;
#96580=CARTESIAN_POINT ( 'NONE',  ( 6.251718229232841928, 8.387033582228703210, -1.443375672974078761 ) ) ;
#96585=CARTESIAN_POINT ( 'NONE',  ( 6.966220764712121927, 6.002124920821316323, 2.420000000000000373 ) ) ;
#96603=CARTESIAN_POINT ( 'NONE',  ( -5.608633734226008194, 5.643391804966442216, 0.4859901473732997079 ) ) ;
#96612=CARTESIAN_POINT ( 'NONE',  ( -3.472296738431328134, 7.065113604896248845, 0.000000000000000000 ) ) ;
#96613=CARTESIAN_POINT ( 'NONE',  ( 4.597436146581902250, 8.478756905425443691, -0.3710115925776128476 ) ) ;
#96618=CARTESIAN_POINT ( 'NONE',  ( -6.459533842268148973, 6.500820668926428958, 0.000000000000000000 ) ) ;
#96625=CARTESIAN_POINT ( 'NONE',  ( 6.966220764712146796, 6.002124920821316323, -2.420000000000000373 ) ) ;
#96626=CARTESIAN_POINT ( 'NONE',  ( -5.438755897737433287, 6.374245297895642537, -1.199719254218453823 ) ) ;
#96629=CARTESIAN_POINT ( 'NONE',  ( 5.917965873332177829, 7.245500866451762612, 1.242176317587460943 ) ) ;
#96634=CARTESIAN_POINT ( 'NONE',  ( 6.717138760927786834, 6.801359740696030443, -0.7998128361456481317 ) ) ;
#96643=CARTESIAN_POINT ( 'NONE',  ( -5.143339171537843590, 7.093924681584509173, 1.599625672291263179 ) ) ;
#96648=CARTESIAN_POINT ( 'NONE',  ( -5.448397627845328550, 7.449826213943242514, 1.599625672291263179 ) ) ;
#96653=CARTESIAN_POINT ( 'NONE',  ( 6.414416072596830887, 8.576847732820027659, -1.443375672974078761 ) ) ;
#96655=CARTESIAN_POINT ( 'NONE',  ( -6.590672069574513792, 6.861741300691274859, 0.000000000000000000 ) ) ;
#96661=CARTESIAN_POINT ( 'NONE',  ( 5.448397627845284141, 7.449826213943242514, 1.599625672291268286 ) ) ;
#96664=( BOUNDED_SURFACE ( )  B_SPLINE_SURFACE ( 1, 2, ( 
 ( #109658, #208127, #92298, #28326, #175660, #111783, #209186, #59756, #210261, #77065, #94422, #61899, #158342, #143195, #44598, #123792, #91218, #160461, #194016, #95497, #139975, #189750, #41402, #25115, #42469, #108579, #157279, #8868, #141058, #197213, #96559, #97616, #130176, #1126, #53, #33647, #65069, #146373, #148484, #50974, #164721, #162606, #16310, #161544, #112847, #46735, #165793, #196168, #49909, #66116, #117096, #163673, #212388, #132259, #47809, #133325, #98666, #34708, #211327, #13131, #198266, #180967, #83460, #183096, #114967, #99721, #116030, #199328, #182016, #17376, #62952, #14182, #149540, #79208, #67188, #145326, #129121, #147422, #195098, #80275, #31540, #178863, #213447, #48853, #30474, #64030, #15256, #113922, #179918, #81343, #131225, #32589, #82395, #54171, #71458, #2182, #37922, #153808, #70385, #3253, #101852, #69321, #200394, #188427, #204657, #184154, #134391, #137571, #5379, #201453, #100777, #18455, #120310, #186285, #105075, #102920, #53096, #20581, #68258, #84532, #103996, #170040, #21626, #38990, #122468, #88819, #6459, #35777, #203588, #4314, #187360, #150621, #135431, #55240, #56306, #87734, #171114, #121387, #85595, #52042, #151683, #22706, #185213, #138634, #154876, #168981, #118168, #72536, #166859, #167921, #136501, #19518, #202522, #119230, #36837, #86665, #152732, #127799, #155944, #42206, #75751, #40062, #106172, #43274, #108323, #10733, #59493, #76803, #89893, #174343, #141861, #23787, #94160, #142924, #74689, #126718, #7530, #208924, #176455, #58437, #123533, #124590, #25921, #172198, #73613, #60559, #192678, #11802, #206804, #158086, #139712, #190550, #92029, #9674, #207869, #44332, #110454, #24853, #28067, #41142, #125650, #191612, #205736, #109394, #175399, #107252, #26984, #160199, #173273, #90955, #93091, #159132, #57370, #157020, #77877, #140790, #143999, #209991, #61633, #189498, #8606, #132009, #95223, #211059, #12859, #31279, #178594, #148229, #14987, #198019, #80006, #129920, #78934, #99471, #45401, #165530, #161273, #196960, #146111, #97354, #47542 ),
 ( #164467, #145056, #179659, #115770, #46460, #63760, #62684, #163411, #81081, #111517, #49647, #195906, #82137, #96291, #17122, #212122, #214231, #113655, #147168, #16053, #128843, #130968, #32334, #213195, #162343, #194824, #13926, #112582, #66928, #83199, #30203, #64822, #65859, #98402, #48598, #193754, #177523, #114716, #180711, #181759, #33393, #149281, #862, #29135, #116840, #136251, #70139, #4069, #71206, #154628, #121143, #38740, #1936, #37670, #36587, #5131, #182841, #167666, #103746, #88570, #202271, #137322, #152487, #117917, #186034, #101598, #86420, #187106, #100530, #169797, #18194, #199068, #166605, #19267, #203338, #102674, #53922, #120059, #21386, #50714, #87495, #153560, #135192, #6208, #34458, #54991, #104822, #170868, #85349, #168732, #84279, #151430, #118982, #52847, #3003, #22458, #133070, #183910, #150366, #134138, #20334, #201208, #67996, #184961, #69072, #200145, #51799, #35521, #139455, #123288, #90710, #8358, #105916, #205487, #43032, #106995, #124344, #206558, #110206, #89640, #173020, #10486, #188176, #155692, #171941, #190302, #57121, #26743, #108071, #76560, #24601, #74442, #23532, #192432, #138386, #44087, #39810, #75503, #156772, #41959, #140544, #58186, #175157, #174099, #176216, #59242, #25672, #208681, #91779, #92846, #60310, #157836, #9433, #141614, #7275, #73352, #191365, #207624, #125400, #109144, #158890, #189251, #142670, #40890, #126469, #27818, #93915, #159956, #72277, #204404, #56057, #122214, #65609, #64584, #98172, #129676, #210823, #212947, #115521, #14748, #12618, #80840, #11560, #177277, #111274, #15807, #46224, #114468, #130725, #181516, #13689, #162100, #28893, #131759, #77630, #197764, #193519, #146930, #112341, #195661, #79759, #96047, #180469, #47295, #49402, #196716, #145875, #147979, #211883, #32084, #213989, #29961, #113410, #48357, #127548, #94977, #164220, #179416, #31037, #97111, #163163, #45160, #81893, #62448, #178353, #33145, #99225, #161023, #143752, #78691, #63524, #194578, #209747, #61389, #144816, #128611, #150105, #152228, #54722, #168470, #166338 ) ),
 .UNSPECIFIED., .F., .F., .F. ) 
 B_SPLINE_SURFACE_WITH_KNOTS ( ( 2, 2 ),
 ( 3, 2, 2, 2, 2, 2, 2, 2, 2, 2, 2, 2, 2, 2, 2, 2, 2, 2, 2, 2, 2, 2, 2, 2, 2, 2, 2, 2, 2, 2, 2, 2, 2, 2, 2, 2, 2, 2, 2, 2, 2, 2, 2, 2, 2, 2, 2, 2, 2, 2, 2, 2, 2, 2, 2, 2, 2, 2, 2, 2, 2, 2, 2, 2, 2, 2, 2, 2, 2, 2, 2, 2, 2, 2, 2, 2, 2, 2, 2, 2, 2, 2, 2, 2, 2, 2, 2, 2, 2, 2, 2, 2, 2, 2, 2, 2, 2, 2, 2, 2, 2, 2, 2, 2, 2, 2, 2, 2, 2, 2, 2, 2, 2, 2, 2, 2, 2, 2, 2, 2, 3 ),
 ( 0.000000000000000000, 1.000000000000000000 ),
 ( 0.000000000000000000, 0.008333333333333333218, 0.01666666666666666644, 0.02500000000000000139, 0.03333333333333333287, 0.04166666666666666435, 0.05000000000000000278, 0.05833333333333333426, 0.06666666666666666574, 0.07499999999999999722, 0.08333333333333332871, 0.09166666666666666019, 0.1000000000000000056, 0.1083333333333333370, 0.1166666666666666685, 0.1250000000000000000, 0.1333333333333333315, 0.1416666666666666630, 0.1499999999999999944, 0.1583333333333333259, 0.1666666666666666574, 0.1749999999999999889, 0.1833333333333333204, 0.1916666666666666796, 0.2000000000000000111, 0.2083333333333333426, 0.2166666666666666741, 0.2250000000000000056, 0.2333333333333333370, 0.2416666666666666685, 0.2500000000000000000, 0.2583333333333333592, 0.2666666666666666630, 0.2750000000000000222, 0.2833333333333333259, 0.2916666666666666852, 0.2999999999999999889, 0.3083333333333333481, 0.3166666666666666519, 0.3250000000000000111, 0.3333333333333333148, 0.3416666666666666741, 0.3499999999999999778, 0.3583333333333333370, 0.3666666666666666408, 0.3750000000000000000, 0.3833333333333333592, 0.3916666666666666630, 0.4000000000000000222, 0.4083333333333333259, 0.4166666666666666852, 0.4249999999999999889, 0.4333333333333333481, 0.4416666666666666519, 0.4500000000000000111, 0.4583333333333333148, 0.4666666666666666741, 0.4749999999999999778, 0.4833333333333333370, 0.4916666666666666408, 0.5000000000000000000, 0.5083333333333333037, 0.5166666666666667185, 0.5250000000000000222, 0.5333333333333333259, 0.5416666666666666297, 0.5500000000000000444, 0.5583333333333333481, 0.5666666666666666519, 0.5749999999999999556, 0.5833333333333333703, 0.5916666666666666741, 0.5999999999999999778, 0.6083333333333332815, 0.6166666666666666963, 0.6250000000000000000, 0.6333333333333333037, 0.6416666666666667185, 0.6500000000000000222, 0.6583333333333333259, 0.6666666666666666297, 0.6750000000000000444, 0.6833333333333333481, 0.6916666666666666519, 0.6999999999999999556, 0.7083333333333333703, 0.7166666666666666741, 0.7249999999999999778, 0.7333333333333332815, 0.7416666666666666963, 0.7500000000000000000, 0.7583333333333333037, 0.7666666666666667185, 0.7750000000000000222, 0.7833333333333333259, 0.7916666666666666297, 0.8000000000000000444, 0.8083333333333333481, 0.8166666666666666519, 0.8249999999999999556, 0.8333333333333333703, 0.8416666666666666741, 0.8499999999999999778, 0.8583333333333332815, 0.8666666666666666963, 0.8750000000000000000, 0.8833333333333333037, 0.8916666666666667185, 0.9000000000000000222, 0.9083333333333333259, 0.9166666666666666297, 0.9250000000000000444, 0.9333333333333333481, 0.9416666666666666519, 0.9499999999999999556, 0.9583333333333333703, 0.9666666666666666741, 0.9749999999999999778, 0.9833333333333332815, 0.9916666666666666963, 1.000000000000000000 ),
 .UNSPECIFIED. ) 
 GEOMETRIC_REPRESENTATION_ITEM ( )  RATIONAL_B_SPLINE_SURFACE ( (
 ( 1.000000000000000000, 0.8660254037844387076, 1.000000000000000000, 0.8660254037844387076, 1.000000000000000000, 0.8660254037844387076, 1.000000000000000000, 0.8660254037844387076, 1.000000000000000000, 0.8660254037844387076, 1.000000000000000000, 0.8660254037844387076, 1.000000000000000000, 0.8660254037844387076, 1.000000000000000000, 0.8660254037844387076, 1.000000000000000000, 0.8660254037844387076, 1.000000000000000000, 0.8660254037844387076, 1.000000000000000000, 0.8660254037844387076, 1.000000000000000000, 0.8660254037844387076, 1.000000000000000000, 0.8660254037844387076, 1.000000000000000000, 0.8660254037844387076, 1.000000000000000000, 0.8660254037844387076, 1.000000000000000000, 0.8660254037844387076, 1.000000000000000000, 0.8660254037844387076, 1.000000000000000000, 0.8660254037844387076, 1.000000000000000000, 0.8660254037844387076, 1.000000000000000000, 0.8660254037844387076, 1.000000000000000000, 0.8660254037844387076, 1.000000000000000000, 0.8660254037844387076, 1.000000000000000000, 0.8660254037844387076, 1.000000000000000000, 0.8660254037844387076, 1.000000000000000000, 0.8660254037844387076, 1.000000000000000000, 0.8660254037844387076, 1.000000000000000000, 0.8660254037844387076, 1.000000000000000000, 0.8660254037844387076, 1.000000000000000000, 0.8660254037844387076, 1.000000000000000000, 0.8660254037844387076, 1.000000000000000000, 0.8660254037844387076, 1.000000000000000000, 0.8660254037844387076, 1.000000000000000000, 0.8660254037844387076, 1.000000000000000000, 0.8660254037844387076, 1.000000000000000000, 0.8660254037844387076, 1.000000000000000000, 0.8660254037844387076, 1.000000000000000000, 0.8660254037844387076, 1.000000000000000000, 0.8660254037844387076, 1.000000000000000000, 0.8660254037844387076, 1.000000000000000000, 0.8660254037844387076, 1.000000000000000000, 0.8660254037844387076, 1.000000000000000000, 0.8660254037844387076, 1.000000000000000000, 0.8660254037844387076, 1.000000000000000000, 0.8660254037844387076, 1.000000000000000000, 0.8660254037844387076, 1.000000000000000000, 0.8660254037844387076, 1.000000000000000000, 0.8660254037844387076, 1.000000000000000000, 0.8660254037844387076, 1.000000000000000000, 0.8660254037844387076, 1.000000000000000000, 0.8660254037844387076, 1.000000000000000000, 0.8660254037844387076, 1.000000000000000000, 0.8660254037844387076, 1.000000000000000000, 0.8660254037844387076, 1.000000000000000000, 0.8660254037844387076, 1.000000000000000000, 0.8660254037844387076, 1.000000000000000000, 0.8660254037844387076, 1.000000000000000000, 0.8660254037844387076, 1.000000000000000000, 0.8660254037844387076, 1.000000000000000000, 0.8660254037844387076, 1.000000000000000000, 0.8660254037844387076, 1.000000000000000000, 0.8660254037844387076, 1.000000000000000000, 0.8660254037844387076, 1.000000000000000000, 0.8660254037844387076, 1.000000000000000000, 0.8660254037844387076, 1.000000000000000000, 0.8660254037844387076, 1.000000000000000000, 0.8660254037844387076, 1.000000000000000000, 0.8660254037844387076, 1.000000000000000000, 0.8660254037844387076, 1.000000000000000000, 0.8660254037844387076, 1.000000000000000000, 0.8660254037844387076, 1.000000000000000000, 0.8660254037844387076, 1.000000000000000000, 0.8660254037844387076, 1.000000000000000000, 0.8660254037844387076, 1.000000000000000000, 0.8660254037844387076, 1.000000000000000000, 0.8660254037844387076, 1.000000000000000000, 0.8660254037844387076, 1.000000000000000000, 0.8660254037844387076, 1.000000000000000000, 0.8660254037844387076, 1.000000000000000000, 0.8660254037844387076, 1.000000000000000000, 0.8660254037844387076, 1.000000000000000000, 0.8660254037844387076, 1.000000000000000000, 0.8660254037844387076, 1.000000000000000000, 0.8660254037844387076, 1.000000000000000000, 0.8660254037844387076, 1.000000000000000000, 0.8660254037844387076, 1.000000000000000000, 0.8660254037844387076, 1.000000000000000000, 0.8660254037844387076, 1.000000000000000000, 0.8660254037844387076, 1.000000000000000000, 0.8660254037844387076, 1.000000000000000000, 0.8660254037844387076, 1.000000000000000000, 0.8660254037844387076, 1.000000000000000000, 0.8660254037844387076, 1.000000000000000000, 0.8660254037844387076, 1.000000000000000000, 0.8660254037844387076, 1.000000000000000000, 0.8660254037844387076, 1.000000000000000000, 0.8660254037844387076, 1.000000000000000000, 0.8660254037844387076, 1.000000000000000000, 0.8660254037844387076, 1.000000000000000000, 0.8660254037844387076, 1.000000000000000000, 0.8660254037844387076, 1.000000000000000000, 0.8660254037844387076, 1.000000000000000000, 0.8660254037844387076, 1.000000000000000000, 0.8660254037844387076, 1.000000000000000000, 0.8660254037844387076, 1.000000000000000000, 0.8660254037844387076, 1.000000000000000000, 0.8660254037844387076, 1.000000000000000000, 0.8660254037844387076, 1.000000000000000000, 0.8660254037844387076, 1.000000000000000000, 0.8660254037844387076, 1.000000000000000000, 0.8660254037844387076, 1.000000000000000000, 0.8660254037844387076, 1.000000000000000000, 0.8660254037844387076, 1.000000000000000000, 0.8660254037844387076, 1.000000000000000000, 0.8660254037844387076, 1.000000000000000000, 0.8660254037844387076, 1.000000000000000000, 0.8660254037844387076, 1.000000000000000000, 0.8660254037844387076, 1.000000000000000000, 0.8660254037844387076, 1.000000000000000000, 0.8660254037844387076, 1.000000000000000000, 0.8660254037844387076, 1.000000000000000000),
 ( 1.000000000000000000, 0.8660254037844387076, 1.000000000000000000, 0.8660254037844387076, 1.000000000000000000, 0.8660254037844387076, 1.000000000000000000, 0.8660254037844387076, 1.000000000000000000, 0.8660254037844387076, 1.000000000000000000, 0.8660254037844387076, 1.000000000000000000, 0.8660254037844387076, 1.000000000000000000, 0.8660254037844387076, 1.000000000000000000, 0.8660254037844387076, 1.000000000000000000, 0.8660254037844387076, 1.000000000000000000, 0.8660254037844387076, 1.000000000000000000, 0.8660254037844387076, 1.000000000000000000, 0.8660254037844387076, 1.000000000000000000, 0.8660254037844387076, 1.000000000000000000, 0.8660254037844387076, 1.000000000000000000, 0.8660254037844387076, 1.000000000000000000, 0.8660254037844387076, 1.000000000000000000, 0.8660254037844387076, 1.000000000000000000, 0.8660254037844387076, 1.000000000000000000, 0.8660254037844387076, 1.000000000000000000, 0.8660254037844387076, 1.000000000000000000, 0.8660254037844387076, 1.000000000000000000, 0.8660254037844387076, 1.000000000000000000, 0.8660254037844387076, 1.000000000000000000, 0.8660254037844387076, 1.000000000000000000, 0.8660254037844387076, 1.000000000000000000, 0.8660254037844387076, 1.000000000000000000, 0.8660254037844387076, 1.000000000000000000, 0.8660254037844387076, 1.000000000000000000, 0.8660254037844387076, 1.000000000000000000, 0.8660254037844387076, 1.000000000000000000, 0.8660254037844387076, 1.000000000000000000, 0.8660254037844387076, 1.000000000000000000, 0.8660254037844387076, 1.000000000000000000, 0.8660254037844387076, 1.000000000000000000, 0.8660254037844387076, 1.000000000000000000, 0.8660254037844387076, 1.000000000000000000, 0.8660254037844387076, 1.000000000000000000, 0.8660254037844387076, 1.000000000000000000, 0.8660254037844387076, 1.000000000000000000, 0.8660254037844387076, 1.000000000000000000, 0.8660254037844387076, 1.000000000000000000, 0.8660254037844387076, 1.000000000000000000, 0.8660254037844387076, 1.000000000000000000, 0.8660254037844387076, 1.000000000000000000, 0.8660254037844387076, 1.000000000000000000, 0.8660254037844387076, 1.000000000000000000, 0.8660254037844387076, 1.000000000000000000, 0.8660254037844387076, 1.000000000000000000, 0.8660254037844387076, 1.000000000000000000, 0.8660254037844387076, 1.000000000000000000, 0.8660254037844387076, 1.000000000000000000, 0.8660254037844387076, 1.000000000000000000, 0.8660254037844387076, 1.000000000000000000, 0.8660254037844387076, 1.000000000000000000, 0.8660254037844387076, 1.000000000000000000, 0.8660254037844387076, 1.000000000000000000, 0.8660254037844387076, 1.000000000000000000, 0.8660254037844387076, 1.000000000000000000, 0.8660254037844387076, 1.000000000000000000, 0.8660254037844387076, 1.000000000000000000, 0.8660254037844387076, 1.000000000000000000, 0.8660254037844387076, 1.000000000000000000, 0.8660254037844387076, 1.000000000000000000, 0.8660254037844387076, 1.000000000000000000, 0.8660254037844387076, 1.000000000000000000, 0.8660254037844387076, 1.000000000000000000, 0.8660254037844387076, 1.000000000000000000, 0.8660254037844387076, 1.000000000000000000, 0.8660254037844387076, 1.000000000000000000, 0.8660254037844387076, 1.000000000000000000, 0.8660254037844387076, 1.000000000000000000, 0.8660254037844387076, 1.000000000000000000, 0.8660254037844387076, 1.000000000000000000, 0.8660254037844387076, 1.000000000000000000, 0.8660254037844387076, 1.000000000000000000, 0.8660254037844387076, 1.000000000000000000, 0.8660254037844387076, 1.000000000000000000, 0.8660254037844387076, 1.000000000000000000, 0.8660254037844387076, 1.000000000000000000, 0.8660254037844387076, 1.000000000000000000, 0.8660254037844387076, 1.000000000000000000, 0.8660254037844387076, 1.000000000000000000, 0.8660254037844387076, 1.000000000000000000, 0.8660254037844387076, 1.000000000000000000, 0.8660254037844387076, 1.000000000000000000, 0.8660254037844387076, 1.000000000000000000, 0.8660254037844387076, 1.000000000000000000, 0.8660254037844387076, 1.000000000000000000, 0.8660254037844387076, 1.000000000000000000, 0.8660254037844387076, 1.000000000000000000, 0.8660254037844387076, 1.000000000000000000, 0.8660254037844387076, 1.000000000000000000, 0.8660254037844387076, 1.000000000000000000, 0.8660254037844387076, 1.000000000000000000, 0.8660254037844387076, 1.000000000000000000, 0.8660254037844387076, 1.000000000000000000, 0.8660254037844387076, 1.000000000000000000, 0.8660254037844387076, 1.000000000000000000, 0.8660254037844387076, 1.000000000000000000, 0.8660254037844387076, 1.000000000000000000, 0.8660254037844387076, 1.000000000000000000, 0.8660254037844387076, 1.000000000000000000, 0.8660254037844387076, 1.000000000000000000, 0.8660254037844387076, 1.000000000000000000, 0.8660254037844387076, 1.000000000000000000, 0.8660254037844387076, 1.000000000000000000, 0.8660254037844387076, 1.000000000000000000, 0.8660254037844387076, 1.000000000000000000, 0.8660254037844387076, 1.000000000000000000, 0.8660254037844387076, 1.000000000000000000, 0.8660254037844387076, 1.000000000000000000, 0.8660254037844387076, 1.000000000000000000, 0.8660254037844387076, 1.000000000000000000, 0.8660254037844387076, 1.000000000000000000, 0.8660254037844387076, 1.000000000000000000, 0.8660254037844387076, 1.000000000000000000, 0.8660254037844387076, 1.000000000000000000, 0.8660254037844387076, 1.000000000000000000, 0.8660254037844387076, 1.000000000000000000) ) ) 
 REPRESENTATION_ITEM ( '' )  SURFACE ( )  );
#96670=CARTESIAN_POINT ( 'NONE',  ( 5.825163275726873202, 6.825053905550038991, 1.199719254218452047 ) ) ;
#96695=VERTEX_POINT ( 'NONE', #151042 ) ;
#96697=CARTESIAN_POINT ( 'NONE',  ( 4.700249516990034238, 8.244041944096728969, -0.6212051699984559860 ) ) ;
#96706=CARTESIAN_POINT ( 'NONE',  ( 8.005163354226054295, 8.304055099544019214, 0.000000000000000000 ) ) ;
#96711=CARTESIAN_POINT ( 'NONE',  ( -6.357087581413799704, 6.851358791993434671, -0.6307199548913413611 ) ) ;
#96714=ORIENTED_EDGE ( 'NONE', *, *, #117140, .T. ) ;
#96716=CARTESIAN_POINT ( 'NONE',  ( -3.757017964318317471, 6.436919154129725484, 1.082531754730549967 ) ) ;
#96726=CARTESIAN_POINT ( 'NONE',  ( -3.709037541790315640, 6.484905011134099340, -1.199719254218450271 ) ) ;
#96734=( BOUNDED_CURVE ( )  B_SPLINE_CURVE ( 2, ( #81577, #96796, #144494 ),
 .UNSPECIFIED., .F., .T. ) 
 B_SPLINE_CURVE_WITH_KNOTS ( ( 3, 3 ),
 ( 0.2943294064411632327, 0.2999999999999999889 ),
 .UNSPECIFIED. ) 
 CURVE ( )  GEOMETRIC_REPRESENTATION_ITEM ( )  RATIONAL_B_SPLINE_CURVE ( ( 0.9417397705941343844, 0.9088341421182736246, 1.000000000000000000 ) ) 
 REPRESENTATION_ITEM ( '' )  );
#96738=CARTESIAN_POINT ( 'NONE',  ( 4.030516805012513082, 7.924296382481737844, 0.000000000000000000 ) ) ;
#96739=CARTESIAN_POINT ( 'NONE',  ( 5.689503332392597201, 5.810377773979076288, 0.3369718469911698322 ) ) ;
#96741=CARTESIAN_POINT ( 'NONE',  ( 5.411112705185558092, 6.445957923205511086, -1.082531754730548412 ) ) ;
#96753=CARTESIAN_POINT ( 'NONE',  ( -5.204350862799341115, 7.165104988056252289, -1.599625672291271394 ) ) ;
#96754=CARTESIAN_POINT ( 'NONE',  ( 4.420840606507738357, 7.315341919971147355, 1.199719254218451159 ) ) ;
#96764=ORIENTED_EDGE ( 'NONE', *, *, #149705, .T. ) ;
#96765=CARTESIAN_POINT ( 'NONE',  ( -5.586841817283045408, 8.675676665875643678, 1.199719254218454489 ) ) ;
#96766=CARTESIAN_POINT ( 'NONE',  ( 7.367930134383754215, 7.560616343061329125, -0.7998128361456341429 ) ) ;
#96768=CARTESIAN_POINT ( 'NONE',  ( -3.809456170543688458, 8.470288933811595200, -2.500000000000000444 ) ) ;
#96770=VERTEX_POINT ( 'NONE', #117522 ) ;
#96773=CARTESIAN_POINT ( 'NONE',  ( 3.984117037569365305, 5.741498858621315371, 1.599625672291261402 ) ) ;
#96780=CARTESIAN_POINT ( 'NONE',  ( -6.292453103784333202, 6.974073686386621951, 0.9489479220791104952 ) ) ;
#96790=CARTESIAN_POINT ( 'NONE',  ( -6.071018923869249129, 10.30488218781460574, 0.7998128361456291469 ) ) ;
#96796=CARTESIAN_POINT ( 'NONE',  ( 5.727717027299726205, 5.854960418037383540, 0.4679561398535265204 ) ) ;
#96805=CARTESIAN_POINT ( 'NONE',  ( 5.182959862174088883, 9.268813282503625572, 0.7998128361456331437 ) ) ;
#96806=ORIENTED_EDGE ( 'NONE', *, *, #77903, .T. ) ;
#96837=CARTESIAN_POINT ( 'NONE',  ( 4.472210567661338843, 6.310941310395290493, 1.599625672291261402 ) ) ;
#96867=VERTEX_POINT ( 'NONE', #1541 ) ;
#96868=CARTESIAN_POINT ( 'NONE',  ( -4.457598643843001973, 8.422558527783969851, 0.000000000000000000 ) ) ;
#96870=CARTESIAN_POINT ( 'NONE',  ( 5.844973620822835336, 7.912498205750389424, 1.443375672974064550 ) ) ;
#96875=CARTESIAN_POINT ( 'NONE',  ( -5.981082042284069367, 7.006959133200059142, 1.199719254218452935 ) ) ;
#96880=CARTESIAN_POINT ( 'NONE',  ( -3.949167883330528372, 7.829389307186077396, 1.214306433183764966E-14 ) ) ;
#96886=CARTESIAN_POINT ( 'NONE',  ( -4.911796789900812144, 8.952456364851418158, 0.7998128361456291469 ) ) ;
#96898=CARTESIAN_POINT ( 'NONE',  ( -3.122120512896910505, 6.864500708346841229, 0.7998128361456352531 ) ) ;
#96901=CARTESIAN_POINT ( 'NONE',  ( -6.644904684473536882, 6.925012684740138980, 0.7216878364870317197 ) ) ;
#96902=CARTESIAN_POINT ( 'NONE',  ( -5.600926855776882540, 8.588146194164741232, -1.082531754730549967 ) ) ;
#96903=CARTESIAN_POINT ( 'NONE',  ( 7.526711554241970248, 8.810193563817646734, -1.199719254218452047 ) ) ;
#96904=CARTESIAN_POINT ( 'NONE',  ( -7.605197822622922210, 7.837428646007010613, -0.7998128361456362523 ) ) ;
#96913=( BOUNDED_CURVE ( )  B_SPLINE_CURVE ( 2, ( #63814, #11853, #210047, #164521, #214282 ),
 .UNSPECIFIED., .F., .T. ) 
 B_SPLINE_CURVE_WITH_KNOTS ( ( 3, 2, 3 ),
 ( 0.2229596301642877976, 0.2250000000000000056, 0.2273783041757627965 ),
 .UNSPECIFIED. ) 
 CURVE ( )  GEOMETRIC_REPRESENTATION_ITEM ( )  RATIONAL_B_SPLINE_CURVE ( ( 0.9504573706892978091, 0.9671970730156055351, 1.000000000000000000, 0.9617641190049276423, 0.9453530113141472846 ) ) 
 REPRESENTATION_ITEM ( '' )  );
#96931=CARTESIAN_POINT ( 'NONE',  ( -4.370663978927107785, 5.060324124126027279, -2.420000000000000373 ) ) ;
#96943=CARTESIAN_POINT ( 'NONE',  ( 4.653539691347775786, 8.417882268172059312, -0.4891605808478947104 ) ) ;
#96958=CARTESIAN_POINT ( 'NONE',  ( 8.188198428010544205, 8.517596018959260107, 0.000000000000000000 ) ) ;
#96961=CARTESIAN_POINT ( 'NONE',  ( -5.143339171537843590, 7.093924681584509173, 1.599625672291263179 ) ) ;
#96965=CARTESIAN_POINT ( 'NONE',  ( -6.902509602688818191, 9.146290184594002781, -1.443375672974066548 ) ) ;
#96975=CARTESIAN_POINT ( 'NONE',  ( 4.329849954717849947, 6.144853928627882489, 1.599625672291262513 ) ) ;
#96977=CARTESIAN_POINT ( 'NONE',  ( 6.994027139803230320, 9.253060644560830994, -1.599625672291267398 ) ) ;
#96985=CARTESIAN_POINT ( 'NONE',  ( 4.248501033035879004, 6.049946853332221153, -1.599625672291273171 ) ) ;
#96991=CARTESIAN_POINT ( 'NONE',  ( 4.715203562502613188, 8.723097599553565118, 0.7998128361456341429 ) ) ;
#97003=CARTESIAN_POINT ( 'NONE',  ( -6.156811154381562012, 6.355570232966157640, 0.7216878364870257245 ) ) ;
#97004=CARTESIAN_POINT ( 'NONE',  ( 4.909461021924244051, 6.821066840368686712, 1.443375672974065660 ) ) ;
#97006=CARTESIAN_POINT ( 'NONE',  ( -4.791166081694341550, 4.882818525799564213, 0.4357780244859492669 ) ) ;
#97015=CARTESIAN_POINT ( 'NONE',  ( -7.770231434407805615, 8.237893892996801526, 0.000000000000000000 ) ) ;
#97019=CARTESIAN_POINT ( 'NONE',  ( 5.194182247366869731, 7.153241603385088965, 1.443375672974064550 ) ) ;
#97034=CARTESIAN_POINT ( 'NONE',  ( 7.065207446497155708, 9.336104335703744539, 0.000000000000000000 ) ) ;
#97038=CARTESIAN_POINT ( 'NONE',  ( 6.547661840756936691, 6.603636667163397256, 0.7998128361456352531 ) ) ;
#97040=CARTESIAN_POINT ( 'NONE',  ( -3.305155586681401303, 7.078041627762083898, 0.7998128361456352531 ) ) ;
#97051=CARTESIAN_POINT ( 'NONE',  ( 5.709392085130549077, 9.675058176045386205, 0.000000000000000000 ) ) ;
#97053=CARTESIAN_POINT ( 'NONE',  ( -6.903036488013351679, 8.082572653217566128, -1.199719254218452047 ) ) ;
#97054=CARTESIAN_POINT ( 'NONE',  ( 6.378184920586140727, 6.405913593630768510, 0.000000000000000000 ) ) ;
#97063=CARTESIAN_POINT ( 'NONE',  ( -5.285699784481336927, 7.260012063351913625, 1.599625672291263179 ) ) ;
#97090=CARTESIAN_POINT ( 'NONE',  ( 4.584065335196261692, 7.401807753487379848, 1.082531754730549078 ) ) ;
#97097=CARTESIAN_POINT ( 'NONE',  ( 3.567203813726949058, 7.175838526074521440, 0.7216878364870257245 ) ) ;
#97109=CARTESIAN_POINT ( 'NONE',  ( -4.444040490229335560, 8.406740681901359480, 0.7998128361456352531 ) ) ;
#97111=CARTESIAN_POINT ( 'NONE',  ( -6.831329296439251131, 9.063246493969506545, -1.599625672291271394 ) ) ;
#97119=CARTESIAN_POINT ( 'NONE',  ( 7.523848900940885542, 7.742521570711348389, 0.7998128361456291469 ) ) ;
#97123=DIRECTION ( 'NONE',  ( 1.000000000000000000, 0.000000000000000000, 0.000000000000000000 ) ) ;
#97125=CARTESIAN_POINT ( 'NONE',  ( -4.437261413422502798, 8.398831758960053406, 0.000000000000000000 ) ) ;
#97131=CARTESIAN_POINT ( 'NONE',  ( -5.072158865288277418, 7.010880990960010273, 1.443375672974058777 ) ) ;
#97134=CARTESIAN_POINT ( 'NONE',  ( -5.822300622425855110, 5.757381912443740646, 0.7998128361456281477 ) ) ;
#97154=CARTESIAN_POINT ( 'NONE',  ( -3.309598895067336510, 6.875299454304925284, 0.000000000000000000 ) ) ;
#97156=CARTESIAN_POINT ( 'NONE',  ( -5.224688093219839402, 7.188831756880171397, -1.599625672291271394 ) ) ;
#97170=DIRECTION ( 'NONE',  ( 0.000000000000000000, 0.000000000000000000, -1.000000000000000000 ) ) ;
#97180=CARTESIAN_POINT ( 'NONE',  ( -6.257970421159510188, 9.458660037064859694, 1.199719254218452047 ) ) ;
#97208=CARTESIAN_POINT ( 'NONE',  ( 5.671053392266061977, 9.838255734277600695, 0.7998128361456331437 ) ) ;
#97220=CARTESIAN_POINT ( 'NONE',  ( 6.233692552841108458, 6.917895963632635592, 0.8214459722771473293 ) ) ;
#97222=CARTESIAN_POINT ( 'NONE',  ( 5.872089928494542477, 9.864872326636710653, 0.000000000000000000 ) ) ;
#97226=CARTESIAN_POINT ( 'NONE',  ( -4.437261413422502798, 8.398831758960053406, 0.000000000000000000 ) ) ;
#97228=ORIENTED_EDGE ( 'NONE', *, *, #32740, .F. ) ;
#97232=CARTESIAN_POINT ( 'NONE',  ( -7.729556973122450714, 8.190440354830551328, 0.000000000000000000 ) ) ;
#97240=CARTESIAN_POINT ( 'NONE',  ( -3.786470039966538970, 7.639575156594750283, 0.000000000000000000 ) ) ;
#97250=CARTESIAN_POINT ( 'NONE',  ( 3.711900195091365262, 7.552577004240394132, -0.7998128361456362523 ) ) ;
#97272=CARTESIAN_POINT ( 'NONE',  ( -6.129167961829681488, 9.308390501180058507, -1.199719254218452047 ) ) ;
#97277=CARTESIAN_POINT ( 'NONE',  ( -5.012700657095048307, 7.921469694614043711, 1.075264880722737182 ) ) ;
#97283=CARTESIAN_POINT ( 'NONE',  ( 6.039231080244466199, 6.010467446565510130, 0.7998128361456352531 ) ) ;
#97289=CARTESIAN_POINT ( 'NONE',  ( 4.421367491832282504, 5.291255174293369556, 1.082531754730549078 ) ) ;
#97292=CARTESIAN_POINT ( 'NONE',  ( 6.888951449519509218, 7.209733910627123876, -0.7216878364870317197 ) ) ;
#97303=CARTESIAN_POINT ( 'NONE',  ( -5.858531774880906262, 6.967946837850073294, 1.082531754730549078 ) ) ;
#97314=PRODUCT_DEFINITION_FORMATION_WITH_SPECIFIED_SOURCE ( 'ANY', '', #207916, .NOT_KNOWN. ) ;
#97339=CARTESIAN_POINT ( 'NONE',  ( 4.529305835417093640, 7.441884687032027657, -1.199719254218450271 ) ) ;
#97342=CARTESIAN_POINT ( 'NONE',  ( 5.737035277238070385, 6.722237907313067140, -1.199719254218452047 ) ) ;
#97354=CARTESIAN_POINT ( 'NONE',  ( -6.102578539926875933, 10.13377570664109051, 0.7216878364870267237 ) ) ;
#97357=CARTESIAN_POINT ( 'NONE',  ( 5.858531774436539052, 6.007577623030311287, 0.000000000000000000 ) ) ;
#97370=CARTESIAN_POINT ( 'NONE',  ( -6.455090533882206216, 7.663932056684933158, -1.082531754730549967 ) ) ;
#97372=CARTESIAN_POINT ( 'NONE',  ( -4.665414256878293031, 7.496714828783040296, -1.082531754730549967 ) ) ;
#97376=DIRECTION ( 'NONE',  ( -0.000000000000000000, 1.000000000000000000, -0.000000000000000000 ) ) ;
#97377=CARTESIAN_POINT ( 'NONE',  ( -2.428612866367529932E-14, 2.999999999999999112, 7.500000000000000000 ) ) ;
#97380=CARTESIAN_POINT ( 'NONE',  ( -5.188547179131282938, 7.398091417871301978, -1.250000002070928096 ) ) ;
#97401=CARTESIAN_POINT ( 'NONE',  ( -3.156015896931072540, 6.904045323053366268, 0.000000000000000000 ) ) ;
#97402=CARTESIAN_POINT ( 'NONE',  ( -5.608481899782703728, 5.650097288974007981, -0.3354201317723095599 ) ) ;
#97411=CARTESIAN_POINT ( 'NONE',  ( -6.749980374757255319, 8.968339418673846097, 1.599625672291269396 ) ) ;
#97412=CARTESIAN_POINT ( 'NONE',  ( -5.519007765018521638, 7.558588572879005874, 1.349693927849420438 ) ) ;
#97414=CARTESIAN_POINT ( 'NONE',  ( 0.000000000000000000, 2.999999999999999112, -2.420000000000000373 ) ) ;
#97415=VERTEX_POINT ( 'NONE', #194190 ) ;
#97426=LINE ( 'NONE', #15061, #17645 ) ;
#97431=CARTESIAN_POINT ( 'NONE',  ( 5.525830126021535449, 8.604496359403894346, -1.199719254218452047 ) ) ;
#97455=CARTESIAN_POINT ( 'NONE',  ( 5.825163275726873202, 6.825053905550038991, 1.199719254218452047 ) ) ;
#97456=CARTESIAN_POINT ( 'NONE',  ( 5.273195401072370281, 5.116759154198018855, -0.7998128361456481317 ) ) ;
#97458=CARTESIAN_POINT ( 'NONE',  ( 3.393283585170187688, 7.180857625999046867, 0.7998128361456271485 ) ) ;
#97468=CARTESIAN_POINT ( 'NONE',  ( 4.641000714467984345, 8.433135692799648808, 0.4354600853693716411 ) ) ;
#97469=CARTESIAN_POINT ( 'NONE',  ( -5.275531169048901958, 8.208517892982092334, -1.082531754730549967 ) ) ;
#97470=CARTESIAN_POINT ( 'NONE',  ( 2.957086901556340575, 6.464035461875470290, 0.7216878364870257245 ) ) ;
#97484=EDGE_LOOP ( 'NONE', ( #29216, #104355, #187889, #132691, #69211 ) ) ;
#97498=CARTESIAN_POINT ( 'NONE',  ( 4.716257332707354699, 6.595662536282280719, -1.599625672291269396 ) ) ;
#97500=CARTESIAN_POINT ( 'NONE',  ( 4.167152111353856547, 5.955039778036558040, 1.599625672291262513 ) ) ;
#97503=ORIENTED_EDGE ( 'NONE', *, *, #204577, .F. ) ;
#97521=CARTESIAN_POINT ( 'NONE',  ( -7.095713291905736853, 9.371694488680407886, 1.599625672291269396 ) ) ;
#97532=CARTESIAN_POINT ( 'NONE',  ( 4.746236293235721604, 7.694970221153795364, 1.199719254218451159 ) ) ;
#97536=CARTESIAN_POINT ( 'NONE',  ( 4.850785098639300408, 8.881276058379668825, -0.7998128361456481317 ) ) ;
#97547=CARTESIAN_POINT ( 'NONE',  ( 4.684024595049480766, 8.263433789595206136, 0.5754648794667740486 ) ) ;
#97557=CARTESIAN_POINT ( 'NONE',  ( 5.052517032109132167, 6.451495319389863425, 1.297790489534809355 ) ) ;
#97563=CARTESIAN_POINT ( 'NONE',  ( -0.4000000000000243916, 2.999999999999999112, 2.420000000000000373 ) ) ;
#97566=CARTESIAN_POINT ( 'NONE',  ( 3.119784744920330422, 6.653849612466795627, 0.7216878364870257245 ) ) ;
#97571=CARTESIAN_POINT ( 'NONE',  ( -7.293360289508603600, 7.473618190706972086, 0.000000000000000000 ) ) ;
#97573=CARTESIAN_POINT ( 'NONE',  ( 6.387826650694035990, 7.481494509678370264, -1.199719254218452047 ) ) ;
#97576=CARTESIAN_POINT ( 'NONE',  ( -6.912678218121246942, 9.158153569265168770, 1.599625672291269396 ) ) ;
#97584=CARTESIAN_POINT ( 'NONE',  ( -0.2066541192881463374, 3.358188146985714884, -2.068744351199750753 ) ) ;
#97599=CARTESIAN_POINT ( 'NONE',  ( 5.207740401424913124, 9.089797878388800711, -0.7216878364870458196 ) ) ;
#97615=CARTESIAN_POINT ( 'NONE',  ( -3.838459892414017194, 7.492294413340791159, -0.004696343102253854214 ) ) ;
#97616=CARTESIAN_POINT ( 'NONE',  ( -5.180624094197616714, 5.216685329418210948, 0.7216878364870257245 ) ) ;
#97618=CARTESIAN_POINT ( 'NONE',  ( 4.376249722160992839, 8.327651452488305850, 0.000000000000000000 ) ) ;
#97636=CARTESIAN_POINT ( 'NONE',  ( 8.136301581532414673, 8.664975731308866003, 0.000000000000000000 ) ) ;
#97642=CARTESIAN_POINT ( 'NONE',  ( 5.741471521233657782, 5.663081294386209663, 0.3692415420062719611 ) ) ;
#97660=DIRECTION ( 'NONE',  ( 1.000000000000000000, 0.000000000000000000, 0.000000000000000000 ) ) ;
#97661=CARTESIAN_POINT ( 'NONE',  ( 3.933273961740298752, 5.682181936820735579, 1.443375672974058777 ) ) ;
#97666=CARTESIAN_POINT ( 'NONE',  ( 2.891631901464575272, 6.595597328342462262, 0.000000000000000000 ) ) ;
#97671=CARTESIAN_POINT ( 'NONE',  ( -3.973948422136970748, 6.690004688251493192, -1.082531754730546636 ) ) ;
#97676=EDGE_LOOP ( 'NONE', ( #100437, #17831, #75413, #104179 ) ) ;
#97677=CARTESIAN_POINT ( 'NONE',  ( -6.608673532018475960, 6.674816973635147477, -0.7998128361456362523 ) ) ;
#97685=EDGE_CURVE ( 'NONE', #149147, #40830, #31710, .T. ) ;
#97686=CARTESIAN_POINT ( 'NONE',  ( -4.142898457427624415, 6.991076079377632091, 1.199719254218452935 ) ) ;
#97689=CARTESIAN_POINT ( 'NONE',  ( 6.231590709102786008, 7.018523052454695765, 1.002697108273574500 ) ) ;
#97692=CARTESIAN_POINT ( 'NONE',  ( 2.973738742942335200, 6.527870343122186725, 0.4765911511174560911 ) ) ;
#97694=CARTESIAN_POINT ( 'NONE',  ( 5.342795052237045539, 8.390955439988655229, -1.199719254218450271 ) ) ;
#97702=CARTESIAN_POINT ( 'NONE',  ( -5.503684012504701961, 5.385662534202396934, 0.000000000000000000 ) ) ;
#97703=AXIS2_PLACEMENT_3D ( 'NONE', #49726, #77964, #33476 ) ;
#97708=CARTESIAN_POINT ( 'NONE',  ( -5.641074431737709283, 8.738948049406083385, -1.199719254218452047 ) ) ;
#97712=CARTESIAN_POINT ( 'NONE',  ( 5.844973620822835336, 7.912498205750389424, 1.443375672974064550 ) ) ;
#97714=CARTESIAN_POINT ( 'NONE',  ( -6.089020385868850305, 10.11795786024005572, -0.7216878364870338292 ) ) ;
#97720=CARTESIAN_POINT ( 'NONE',  ( 5.017399365509065845, 8.011327138806002779, -1.199719254218450271 ) ) ;
#97729=CARTESIAN_POINT ( 'NONE',  ( -6.966220764712169000, 6.002124920821316323, -2.500000000000000444 ) ) ;
#97758=CARTESIAN_POINT ( 'NONE',  ( 6.912678218121202534, 9.158153569265168770, 1.599625672291268286 ) ) ;
#97763=CARTESIAN_POINT ( 'NONE',  ( -5.095330737579740976, 7.839774693193753308, -1.136590250493845877 ) ) ;
#97780=CARTESIAN_POINT ( 'NONE',  ( -8.086512275908061653, 8.398962174839683215, 0.000000000000000000 ) ) ;
#97792=CARTESIAN_POINT ( 'NONE',  ( 4.908934136599710563, 7.884784371745123366, 1.199719254218451159 ) ) ;
#97795=CARTESIAN_POINT ( 'NONE',  ( 6.170369307550815030, 8.292126506933040986, 1.443375672974064550 ) ) ;
#97808=CARTESIAN_POINT ( 'NONE',  ( -5.798046968499580345, 6.793418213784815585, 1.199719254218452935 ) ) ;
#97809=CARTESIAN_POINT ( 'NONE',  ( 4.472210567661338843, 6.310941310395290493, 1.599625672291261402 ) ) ;
#97820=CARTESIAN_POINT ( 'NONE',  ( -6.129167961829681488, 9.308390501180058507, -1.199719254218452047 ) ) ;
#97821=CARTESIAN_POINT ( 'NONE',  ( 7.517069824134078537, 7.734612647770044092, 0.000000000000000000 ) ) ;
#97823=FACE_OUTER_BOUND ( 'NONE', #102558, .T. ) ;
#97827=CARTESIAN_POINT ( 'NONE',  ( 4.740510986633625024, 5.559626234941203116, -1.199719254218450271 ) ) ;
#97834=CARTESIAN_POINT ( 'NONE',  ( -6.533345026022147728, 6.811601368426168257, 0.5105341503897353750 ) ) ;
#97842=CARTESIAN_POINT ( 'NONE',  ( -4.217995187182965289, 6.014356699837137832, 1.443375672974065660 ) ) ;
#97843=CARTESIAN_POINT ( 'NONE',  ( -5.302647476276252547, 5.359045941843285199, 0.7216878364870257245 ) ) ;
#97897=CARTESIAN_POINT ( 'NONE',  ( 6.943184063974162434, 9.193743722760251202, -1.443375672974064550 ) ) ;
#97907=B_SPLINE_CURVE_WITH_KNOTS ( 'NONE', 3,
 ( #107211, #123495, #90915, #145014 ),
 .UNSPECIFIED., .F., .F.,
 ( 4, 4 ),
 ( 0.000000000000000000, 0.0001589223950334678857 ),
 .UNSPECIFIED. ) ;
#97927=CARTESIAN_POINT ( 'NONE',  ( -5.601453741101424022, 6.564059448486966986, -1.199719254218453823 ) ) ;
#97929=CARTESIAN_POINT ( 'NONE',  ( 5.506019780481205217, 9.437790487287811558, 0.000000000000000000 ) ) ;
#97934=CARTESIAN_POINT ( 'NONE',  ( -5.769876891067536206, 8.889217585290882795, 1.199719254218454489 ) ) ;
#97946=CARTESIAN_POINT ( 'NONE',  ( -5.798046968499580345, 6.793418213784815585, 1.199719254218452935 ) ) ;
#97957=CARTESIAN_POINT ( 'NONE',  ( -6.120580001926503755, 6.105374521861167914, -0.7998128361456362523 ) ) ;
#97960=CARTESIAN_POINT ( 'NONE',  ( -7.160114521792834807, 8.486460042580672436, 1.082531754730549078 ) ) ;
#97962=CARTESIAN_POINT ( 'NONE',  ( -7.566859129758459979, 8.000626204239226880, 0.000000000000000000 ) ) ;
#97963=CARTESIAN_POINT ( 'NONE',  ( 5.365994935958575240, 9.482354201918870018, 0.7998128361456341429 ) ) ;
#97964=CARTESIAN_POINT ( 'NONE',  ( -7.781453819600577582, 8.043060642480948985, 0.000000000000000000 ) ) ;
#97984=CARTESIAN_POINT ( 'NONE',  ( 6.590809034589254267, 6.776089313701147532, -0.2235409772415736240 ) ) ;
#97990=CARTESIAN_POINT ( 'NONE',  ( 5.671814582574529418, 7.426500967315623036, -1.373566114539000793 ) ) ;
#98003=CARTESIAN_POINT ( 'NONE',  ( 6.490673131624099312, 6.748652840683030618, -0.08655830178419705867 ) ) ;
#98015=DIRECTION ( 'NONE',  ( -1.000000000000000000, 0.000000000000000000, 0.000000000000000000 ) ) ;
#98017=EDGE_CURVE ( 'NONE', #96449, #116214, #173908, .T. ) ;
#98018=CIRCLE ( 'NONE', #111987, 0.07999999999999993228 ) ;
#98019=CARTESIAN_POINT ( 'NONE',  ( 5.664274315459256748, 9.830346811336296398, -0.7998128361456481317 ) ) ;
#98022=CARTESIAN_POINT ( 'NONE',  ( -3.630551273409382329, 7.457669928944732796, 0.7998128361456352531 ) ) ;
#98037=CARTESIAN_POINT ( 'NONE',  ( 3.576318658954677598, 7.394398545414291313, 0.7998128361456281477 ) ) ;
#98039=CARTESIAN_POINT ( 'NONE',  ( 5.657495238652423097, 9.822437888394988548, 0.000000000000000000 ) ) ;
#98044=CARTESIAN_POINT ( 'NONE',  ( -7.241463443030476732, 7.620997903056574430, 0.000000000000000000 ) ) ;
#98051=CARTESIAN_POINT ( 'NONE',  ( 7.849244587668864348, 8.122149871893999062, 0.7998128361456291469 ) ) ;
#98062=CARTESIAN_POINT ( 'NONE',  ( -5.560252395380252288, 7.580323442733986283, 1.443375672974058777 ) ) ;
#98063=CARTESIAN_POINT ( 'NONE',  ( 6.211043768836185031, 6.418841616496599123, 0.7216878364870328300 ) ) ;
#98075=CARTESIAN_POINT ( 'NONE',  ( -5.451787166470911217, 9.374519104275787384, 0.7216878364870267237 ) ) ;
#98076=CARTESIAN_POINT ( 'NONE',  ( 7.364013710877980401, 8.620379413226322285, -1.199719254218452047 ) ) ;
#98080=CARTESIAN_POINT ( 'NONE',  ( 5.248414861821569133, 6.256143772614186638, -1.082531754730548412 ) ) ;
#98082=EDGE_LOOP ( 'NONE', ( #37121, #141930, #163949, #44129, #123603 ) ) ;
#98087=AXIS2_PLACEMENT_3D ( 'NONE', #109714, #70974, #78198 ) ;
#98099=CARTESIAN_POINT ( 'NONE',  ( -5.666381855868691808, 5.575476684793721383, 0.000000000000000000 ) ) ;
#98112=CARTESIAN_POINT ( 'NONE',  ( 4.146814880933355596, 5.931313009212638931, 1.599625672291261402 ) ) ;
#98114=CARTESIAN_POINT ( 'NONE',  ( -6.577640801285370209, 7.702944352034914566, -1.199719254218452047 ) ) ;
#98115=CARTESIAN_POINT ( 'NONE',  ( 5.367048706163317640, 7.354919138647580290, -1.599625672291281386 ) ) ;
#98116=ORIENTED_EDGE ( 'NONE', *, *, #3121, .F. ) ;
#98124=CARTESIAN_POINT ( 'NONE',  ( -5.798046968499580345, 6.793418213784815585, 1.199719254218452935 ) ) ;
#98147=LINE ( 'NONE', #15783, #73627 ) ;
#98149=AXIS2_PLACEMENT_3D ( 'NONE', #205174, #107774, #88252 ) ;
#98153=CARTESIAN_POINT ( 'NONE',  ( 5.248414862265931902, 5.295774558831261913, 0.000000000000000000 ) ) ;
#98159=CARTESIAN_POINT ( 'NONE',  ( 5.194182247366878613, 6.192872389083746043, 1.082531754730549078 ) ) ;
#98170=CARTESIAN_POINT ( 'NONE',  ( -5.875479466675803231, 7.948088359245467416, -1.599625672291271394 ) ) ;
#98172=CARTESIAN_POINT ( 'NONE',  ( -7.273023059088104425, 7.449891421883056530, 0.000000000000000000 ) ) ;
#98178=CARTESIAN_POINT ( 'NONE',  ( 7.686546744304875389, 7.932335721302671949, 0.7998128361456291469 ) ) ;
#98184=CARTESIAN_POINT ( 'NONE',  ( -7.425025402139490360, 8.691559719698066289, 1.199719254218452047 ) ) ;
#98190=CARTESIAN_POINT ( 'NONE',  ( -4.828112100242283766, 7.686528979374367410, -1.082531754730549967 ) ) ;
#98193=CARTESIAN_POINT ( 'NONE',  ( -6.231907884136888676, 7.299589282028351001, -1.199719254218453823 ) ) ;
#98211=ORIENTED_EDGE ( 'NONE', *, *, #27310, .F. ) ;
#98212=CARTESIAN_POINT ( 'NONE',  ( -5.745623237141265882, 9.925253886631958622, 0.7998128361456291469 ) ) ;
#98214=CARTESIAN_POINT ( 'NONE',  ( -5.712781623311813384, 7.758274208654143855, -1.599625672291271394 ) ) ;
#98235=CARTESIAN_POINT ( 'NONE',  ( -6.794571259104023930, 7.956029886156682274, 1.199719254218452047 ) ) ;
#98258=CARTESIAN_POINT ( 'NONE',  ( 4.004454267989866700, 5.765225627445230927, 1.599625672291262513 ) ) ;
#98273=CARTESIAN_POINT ( 'NONE',  ( 7.838022202476093270, 8.316983122409855156, 0.7216878364870267237 ) ) ;
#98279=CARTESIAN_POINT ( 'NONE',  ( -4.762657100150483380, 8.778460060142702304, 0.000000000000000000 ) ) ;
#98284=CARTESIAN_POINT ( 'NONE',  ( -5.573810548549546162, 9.516879716700865188, 0.7216878364870267237 ) ) ;
#98294=CARTESIAN_POINT ( 'NONE',  ( -6.134138155540168391, 6.121192367743780949, 0.000000000000000000 ) ) ;
#98302=CARTESIAN_POINT ( 'NONE',  ( 3.739016502318667445, 7.584212696005614873, 0.7998128361456271485 ) ) ;
#98318=CARTESIAN_POINT ( 'NONE',  ( -5.595389610960904037, 5.773517989023353003, 0.3570679098348183422 ) ) ;
#98322=CARTESIAN_POINT ( 'NONE',  ( -8.072954122294394352, 8.383144328957069291, -0.7998128361456362523 ) ) ;
#98325=CARTESIAN_POINT ( 'NONE',  ( 8.005163354226054295, 8.304055099544019214, 0.000000000000000000 ) ) ;
#98332=CARTESIAN_POINT ( 'NONE',  ( 5.071631979963703962, 8.074598522336444262, 1.199719254218451159 ) ) ;
#98337=CARTESIAN_POINT ( 'NONE',  ( -2.889872605471121236, 6.605953636083950364, 2.500000000000000000 ) ) ;
#98339=CARTESIAN_POINT ( 'NONE',  ( 3.418064124421011041, 7.001842221884225559, -0.7216878364870338292 ) ) ;
#98341=CARTESIAN_POINT ( 'NONE',  ( 3.231779075379137556, 6.036511184309975242, -0.9899555337401846344 ) ) ;
#98342=CARTESIAN_POINT ( 'NONE',  ( 5.397554552016212703, 8.350878506444006533, 1.082531754730547524 ) ) ;
#98353=CARTESIAN_POINT ( 'NONE',  ( -5.451787166470911217, 9.374519104275787384, 0.7216878364870267237 ) ) ;
#98377=CARTESIAN_POINT ( 'NONE',  ( 6.021229617800532452, 6.197391773621639288, 0.000000000000000000 ) ) ;
#98384=ORIENTED_EDGE ( 'NONE', *, *, #132650, .T. ) ;
#98388=CARTESIAN_POINT ( 'NONE',  ( 5.204350862799327793, 7.165104988056252289, -1.599625672291281386 ) ) ;
#98390=CARTESIAN_POINT ( 'NONE',  ( 5.037736595929563244, 8.035053907629919223, -1.199719254218452047 ) ) ;
#98395=ORIENTED_EDGE ( 'NONE', *, *, #4999, .T. ) ;
#98402=CARTESIAN_POINT ( 'NONE',  ( -4.309512724297390740, 6.121127159803966933, 1.599625672291270506 ) ) ;
#98405=CARTESIAN_POINT ( 'NONE',  ( 3.892599500454932304, 7.555466827257172113, 0.7216878364870257245 ) ) ;
#98418=CARTESIAN_POINT ( 'NONE',  ( -5.478903473698241378, 9.406154796041011679, -0.7216878364870338292 ) ) ;
#98420=CARTESIAN_POINT ( 'NONE',  ( -5.695833931516914639, 6.778132687258748845, 1.082531754730549078 ) ) ;
#98434=AXIS2_PLACEMENT_3D ( 'NONE', #9905, #208099, #160430 ) ;
#98450=CARTESIAN_POINT ( 'NONE',  ( -4.817943484809863008, 6.714296380401858499, 1.599625672291263179 ) ) ;
#98458=FACE_BOUND ( 'NONE', #104054, .T. ) ;
#98459=CARTESIAN_POINT ( 'NONE',  ( -7.923814432544069142, 8.209148024248356990, 0.000000000000000000 ) ) ;
#98460=CARTESIAN_POINT ( 'NONE',  ( -4.595593225409446703, 8.485229224138180371, -0.2149309537713070539 ) ) ;
#98477=CARTESIAN_POINT ( 'NONE',  ( 4.850785098639300408, 8.881276058379668825, -0.7998128361456481317 ) ) ;
#98504=CARTESIAN_POINT ( 'NONE',  ( 7.042534447655770080, 7.180988041878682004, -0.7998128361456341429 ) ) ;
#98505=CARTESIAN_POINT ( 'NONE',  ( 6.073126464278658432, 6.050012061272033392, 0.000000000000000000 ) ) ;
#98507=CARTESIAN_POINT ( 'NONE',  ( 4.583538449871731757, 7.505156070562471804, 1.199719254218451159 ) ) ;
#98510=CARTESIAN_POINT ( 'NONE',  ( -4.021726917867474604, 3.853862851527702027, -2.500000000000000444 ) ) ;
#98519=CARTESIAN_POINT ( 'NONE',  ( 4.827426732796687325, 8.217478009653898852, -0.9130428269800896501 ) ) ;
#98520=CARTESIAN_POINT ( 'NONE',  ( -5.112833325684908559, 8.018703742390766109, -1.082531754730549967 ) ) ;
#98521=CARTESIAN_POINT ( 'NONE',  ( 4.340018570150304456, 6.156717313299049366, -1.443375672974068769 ) ) ;
#98539=CARTESIAN_POINT ( 'NONE',  ( -4.137364601623837679, 8.820716007809833670, 0.7750000000000002442 ) ) ;
#98540=LINE ( 'NONE', #181894, #147951 ) ;
#98546=CARTESIAN_POINT ( 'NONE',  ( 3.881377115262159894, 7.750300077773022878, 0.7998128361456271485 ) ) ;
#98549=CARTESIAN_POINT ( 'NONE',  ( 5.032011289327418702, 5.899709921417326974, 1.199719254218452935 ) ) ;
#98566=CYLINDRICAL_SURFACE ( 'NONE', #177133, 0.7499999999999997780 ) ;
#98569=CARTESIAN_POINT ( 'NONE',  ( -4.658966671999400511, 7.502878459571090453, -1.089694788465228159 ) ) ;
#98574=FACE_OUTER_BOUND ( 'NONE', #67858, .T. ) ;
#98578=CARTESIAN_POINT ( 'NONE',  ( -2.995508107964761191, 6.411541510041463887, -0.7147908198718248007 ) ) ;
#98580=CARTESIAN_POINT ( 'NONE',  ( 4.532168488718122390, 8.509556680138327778, 0.7998128361456271485 ) ) ;
#98584=CARTESIAN_POINT ( 'NONE',  ( -6.068414747559345734, 7.047288584480712714, 1.012934185448462143 ) ) ;
#98585=CARTESIAN_POINT ( 'NONE',  ( 6.900173834712277632, 7.014900660111269559, -0.7998128361456341429 ) ) ;
#98596=CARTESIAN_POINT ( 'NONE',  ( 4.601545839464173504, 8.365386937211251706, 0.1680730238927778675 ) ) ;
#98618=CARTESIAN_POINT ( 'NONE',  ( -7.282664789195997912, 8.525472337930658284, 1.199719254218452047 ) ) ;
#98620=CARTESIAN_POINT ( 'NONE',  ( 4.877901405866606588, 8.912911750144889567, 0.7998128361456341429 ) ) ;
#98625=CARTESIAN_POINT ( 'NONE',  ( -3.363831509966363598, 5.978201624052440266, -1.082531754730548412 ) ) ;
#98629=CARTESIAN_POINT ( 'NONE',  ( 3.615248252392856632, 3.576401842564421951, -2.500000000000000444 ) ) ;
#98632=FACE_OUTER_BOUND ( 'NONE', #141495, .T. ) ;
#98651=CARTESIAN_POINT ( 'NONE',  ( 6.292392690518195941, 8.434487120394948079, -1.443375672974078761 ) ) ;
#98666=CARTESIAN_POINT ( 'NONE',  ( -5.045042558060949034, 6.018876084893449274, 1.082531754730549078 ) ) ;
#98668=CARTESIAN_POINT ( 'NONE',  ( 7.198453214212898743, 7.362893269528701268, 0.7998128361456291469 ) ) ;
#98671=CARTESIAN_POINT ( 'NONE',  ( -6.071018923869249129, 10.30488218781460574, 0.7998128361456291469 ) ) ;
#98672=CARTESIAN_POINT ( 'NONE',  ( -3.871735385154307263, 6.674719161725423788, -1.199719254218450271 ) ) ;
#98683=CARTESIAN_POINT ( 'NONE',  ( -6.116136693096207999, 6.308116694799911883, 0.7216878364870257245 ) ) ;
#98717=CARTESIAN_POINT ( 'NONE',  ( 3.607351389687783794, 6.366271167014519783, 1.199719254218451159 ) ) ;
#98722=CARTESIAN_POINT ( 'NONE',  ( -4.299344108864949554, 8.030002203735486788, -0.7216878364870338292 ) ) ;
#98723=CARTESIAN_POINT ( 'NONE',  ( -3.719872605471121751, 6.605953636083950364, 7.500000000000000000 ) ) ;
#98729=CARTESIAN_POINT ( 'NONE',  ( -5.264308783856126439, 9.363720357799287797, -0.7998128361456362523 ) ) ;
#98736=CARTESIAN_POINT ( 'NONE',  ( 8.018721507839716267, 8.319872945426633137, -0.7998128361456341429 ) ) ;
#98737=CARTESIAN_POINT ( 'NONE',  ( -6.143779885648060102, 7.196773283791382703, 1.199719254218452047 ) ) ;
#98738=CARTESIAN_POINT ( 'NONE',  ( -3.811250579217344558, 5.539821323877241355, 0.000000000000000000 ) ) ;
#98740=CARTESIAN_POINT ( 'NONE',  ( 5.966021608595377224, 7.209656400309186530, 1.216315744458285719 ) ) ;
#98745=CARTESIAN_POINT ( 'NONE',  ( 7.178115983792402233, 7.339166500704784823, 0.7998128361456281477 ) ) ;
#98746=EDGE_CURVE ( 'NONE', #131991, #141689, #160831, .T. ) ;
#98754=CARTESIAN_POINT ( 'NONE',  ( -5.167592825464113915, 6.057888380243431570, 1.199719254218452935 ) ) ;
#98756=VECTOR ( 'NONE', #104793, 1000.000000000000114 ) ;
#98759=CARTESIAN_POINT ( 'NONE',  ( -7.123883369337781879, 7.275895117174344229, 0.7998128361456341429 ) ) ;
#98764=CARTESIAN_POINT ( 'NONE',  ( 4.855228407025239612, 8.678533884922511987, 0.000000000000000000 ) ) ;
#98766=CARTESIAN_POINT ( 'NONE',  ( -5.438229012412888252, 9.358701257874761481, -0.7216878364870338292 ) ) ;
#98773=CARTESIAN_POINT ( 'NONE',  ( 7.178115983792402233, 7.339166500704784823, 0.7998128361456281477 ) ) ;
#98774=ORIENTED_EDGE ( 'NONE', *, *, #30625, .F. ) ;
#98808=DIRECTION ( 'NONE',  ( 0.6507913734559654939, -0.7592566023652992380, 0.000000000000000000 ) ) ;
#98816=CARTESIAN_POINT ( 'NONE',  ( -5.265531293961836390, 7.681012046988098696, -1.216234931179949186 ) ) ;
#98819=CARTESIAN_POINT ( 'NONE',  ( -6.966220764712169000, 6.002124920821316323, -2.500000000000000444 ) ) ;
#98837=CARTESIAN_POINT ( 'NONE',  ( -4.167152111353897403, 5.955039778036558040, 1.599625672291270506 ) ) ;
#98849=CARTESIAN_POINT ( 'NONE',  ( 5.123001941117305336, 7.070197912760590064, 1.599625672291268286 ) ) ;
#98852=CARTESIAN_POINT ( 'NONE',  ( 5.194182247366861738, 9.073980031987776584, 0.7216878364870317197 ) ) ;
#98865=CARTESIAN_POINT ( 'NONE',  ( -4.613517410400161722, 8.604463755433990002, -0.7998128361456362523 ) ) ;
#98866=CARTESIAN_POINT ( 'NONE',  ( 3.379725431556547477, 7.165039780116438273, -1.734723475976807094E-15 ) ) ;
#98871=ORIENTED_EDGE ( 'NONE', *, *, #20366, .T. ) ;
#98875=CARTESIAN_POINT ( 'NONE',  ( -2.979759899953417612, 6.698413326579433225, 0.7998128361456352531 ) ) ;
#98876=CARTESIAN_POINT ( 'NONE',  ( 7.191674137406095291, 7.354984346587396082, 0.000000000000000000 ) ) ;
#98879=DIRECTION ( 'NONE',  ( -0.6507913734559640506, -0.7592566023653005702, 0.000000000000000000 ) ) ;
#98883=CARTESIAN_POINT ( 'NONE',  ( 4.553559489343365740, 6.405848385690952718, -1.599625672291269396 ) ) ;
#98890=CARTESIAN_POINT ( 'NONE',  ( -6.155278136343885542, 7.070130543739276519, 1.092798041965221900 ) ) ;
#98899=CARTESIAN_POINT ( 'NONE',  ( -8.106849506328558164, 8.422688943663599659, 0.000000000000000000 ) ) ;
#98930=CARTESIAN_POINT ( 'NONE',  ( 5.357406976055401948, 6.279338222599979424, 1.199719254218452935 ) ) ;
#98951=CARTESIAN_POINT ( 'NONE',  ( 5.239300017038202917, 5.077214539491492928, 0.000000000000000000 ) ) ;
#98952=CARTESIAN_POINT ( 'NONE',  ( -3.024877669624710386, 6.543124691288523920, 0.000000000000000000 ) ) ;
#98979=CARTESIAN_POINT ( 'NONE',  ( -6.656127069666307072, 6.730179434224282886, 0.7998128361456341429 ) ) ;
#98981=CARTESIAN_POINT ( 'NONE',  ( 6.414416072596830887, 8.576847732820027659, -1.443375672974078761 ) ) ;
#98986=CARTESIAN_POINT ( 'NONE',  ( -7.117104292530948229, 7.267986194233038155, -0.7998128361456362523 ) ) ;
#98994=CARTESIAN_POINT ( 'NONE',  ( -5.576146316970437944, 9.727530813099326323, 0.000000000000000000 ) ) ;
#99001=CARTESIAN_POINT ( 'NONE',  ( 6.616470431587431200, 6.759375818431882621, 0.1137606100791552777 ) ) ;
#99006=CARTESIAN_POINT ( 'NONE',  ( -4.288121723672178476, 8.224835454251337552, -0.7998128361456362523 ) ) ;
#99009=CARTESIAN_POINT ( 'NONE',  ( -6.536439455564198475, 8.719208346281938304, 1.443375672974064550 ) ) ;
#99011=CARTESIAN_POINT ( 'NONE',  ( -6.360183458142173230, 9.473945563590925545, 1.082531754730549967 ) ) ;
#99012=CARTESIAN_POINT ( 'NONE',  ( 6.556249800660121529, 9.806652646482286073, 1.199719254218452047 ) ) ;
#99013=CARTESIAN_POINT ( 'NONE',  ( -2.984203208339354152, 6.495671153122273722, 0.000000000000000000 ) ) ;
#99015=VERTEX_POINT ( 'NONE', #3162 ) ;
#99035=CARTESIAN_POINT ( 'NONE',  ( 6.604949037901548969, 6.766875157141204689, 0.08182522243922914218 ) ) ;
#99054=CARTESIAN_POINT ( 'NONE',  ( 5.834480046583573554, 7.201333694826374199, -1.164487238324034557 ) ) ;
#99070=CARTESIAN_POINT ( 'NONE',  ( 5.501576472095266901, 9.640532660744973725, -0.7998128361456481317 ) ) ;
#99073=CARTESIAN_POINT ( 'NONE',  ( -5.818384198920079520, 6.817144982608731141, 1.199719254218452935 ) ) ;
#99088=CARTESIAN_POINT ( 'NONE',  ( 4.224247379109608680, 7.085983154673295203, -1.199719254218452047 ) ) ;
#99090=CARTESIAN_POINT ( 'NONE',  ( 6.318982112420993502, 9.529840343536603697, -1.199719254218452047 ) ) ;
#99095=CARTESIAN_POINT ( 'NONE',  ( -6.577113915960841162, 7.806292669110006521, -1.082531754730549967 ) ) ;
#99101=CARTESIAN_POINT ( 'NONE',  ( 7.095713291905693332, 9.371694488680407886, 1.599625672291268286 ) ) ;
#99114=AXIS2_PLACEMENT_3D ( 'NONE', #112242, #129574, #46125 ) ;
#99116=CARTESIAN_POINT ( 'NONE',  ( -5.153507786970262572, 9.026526494858359229, -0.7216878364870338292 ) ) ;
#99117=CARTESIAN_POINT ( 'NONE',  ( 4.556949027968946631, 8.330541276023501140, -0.7216878364870357165 ) ) ;
#99122=ORIENTED_EDGE ( 'NONE', *, *, #105759, .F. ) ;
#99128=CARTESIAN_POINT ( 'NONE',  ( -5.496904935697871863, 5.377753611261092637, 0.7998128361456281477 ) ) ;
#99129=CARTESIAN_POINT ( 'NONE',  ( -6.238160076063538284, 9.331584951165851294, 1.082531754730549967 ) ) ;
#99130=CARTESIAN_POINT ( 'NONE',  ( 1.846545397494917973, 2.494430857982443683, -2.490037463721383126 ) ) ;
#99134=CARTESIAN_POINT ( 'NONE',  ( 6.007671464186837618, 6.181573927739029806, 0.7216878364870328300 ) ) ;
#99148=CARTESIAN_POINT ( 'NONE',  ( -4.326460414921602826, 8.061637894134911164, 8.322892513849239118E-08 ) ) ;
#99149=CARTESIAN_POINT ( 'NONE',  ( 3.390947817193682656, 6.009837315817661008, -1.082531754730549967 ) ) ;
#99152=CARTESIAN_POINT ( 'NONE',  ( -3.318713740295064163, 7.093859473644694269, 0.000000000000000000 ) ) ;
#99162=CARTESIAN_POINT ( 'NONE',  ( 4.415115299905642665, 5.179997933758551554, -1.199719254218450271 ) ) ;
#99165=CARTESIAN_POINT ( 'NONE',  ( 6.042093733545556233, 7.078139439671806699, -1.199719254218452047 ) ) ;
#99175=PLANE ( 'NONE',  #19147 ) ;
#99200=AXIS2_PLACEMENT_3D ( 'NONE', #89655, #140560, #25689 ) ;
#99203=CARTESIAN_POINT ( 'NONE',  ( 4.665414256878284149, 6.536345614481700927, -1.443375672974068769 ) ) ;
#99210=CARTESIAN_POINT ( 'NONE',  ( 6.034787771414195312, 6.213209619504250547, -0.7216878364870458196 ) ) ;
#99223=CARTESIAN_POINT ( 'NONE',  ( -7.306918443122272677, 7.489436036589583345, 0.7998128361456341429 ) ) ;
#99225=CARTESIAN_POINT ( 'NONE',  ( -6.400331034103001748, 9.624747418832267698, 1.199719254218452935 ) ) ;
#99233=CARTESIAN_POINT ( 'NONE',  ( 5.989670002187236442, 10.20997511251894529, -0.7998128361456481317 ) ) ;
#99238=FACE_OUTER_BOUND ( 'NONE', #206064, .T. ) ;
#99239=CARTESIAN_POINT ( 'NONE',  ( -8.072954122294394352, 8.383144328957069291, -0.7998128361456362523 ) ) ;
#99245=CARTESIAN_POINT ( 'NONE',  ( -5.424670859243583720, 8.382514198209223721, 1.082531754730550855 ) ) ;
#99247=( BOUNDED_CURVE ( )  B_SPLINE_CURVE ( 2, ( #155299, #156375, #106599 ),
 .UNSPECIFIED., .F., .T. ) 
 B_SPLINE_CURVE_WITH_KNOTS ( ( 3, 3 ),
 ( 0.5249999999999998002, 0.5283518216537415046 ),
 .UNSPECIFIED. ) 
 CURVE ( )  GEOMETRIC_REPRESENTATION_ITEM ( )  RATIONAL_B_SPLINE_CURVE ( ( 1.000000000000003553, 0.9461129256824096778, 0.9355746183778924641 ) ) 
 REPRESENTATION_ITEM ( '' )  );
#99249=CARTESIAN_POINT ( 'NONE',  ( -6.961185525973791144, 7.086080966583015339, 0.7998128361456341429 ) ) ;
#99269=CARTESIAN_POINT ( 'NONE',  ( -3.187575512988701565, 6.732938841879847480, 0.000000000000000000 ) ) ;
#99272=CARTESIAN_POINT ( 'NONE',  ( -5.126391479298592735, 5.153413945369351268, 0.000000000000000000 ) ) ;
#99273=CARTESIAN_POINT ( 'NONE',  ( 5.585032934186686226, 5.480569609498057382, 0.000000000000000000 ) ) ;
#99274=CARTESIAN_POINT ( 'NONE',  ( -4.633854640820660009, 8.628190524257904670, -0.7998128361456362523 ) ) ;
#99286=ORIENTED_EDGE ( 'NONE', *, *, #8612, .F. ) ;
#99298=CARTESIAN_POINT ( 'NONE',  ( -7.445362632559989535, 8.715286488521982733, 1.199719254218452047 ) ) ;
#99324=CARTESIAN_POINT ( 'NONE',  ( 3.088225128862704949, 6.824956093640315302, 0.7998128361456281477 ) ) ;
#99337=CARTESIAN_POINT ( 'NONE',  ( 4.713861384769566953, 8.227931952640012980, -0.6562286284988675389 ) ) ;
#99339=CARTESIAN_POINT ( 'NONE',  ( 3.770049233051776749, 6.556085317605844232, 1.199719254218451159 ) ) ;
#99344=CARTESIAN_POINT ( 'NONE',  ( -4.776215253764153346, 8.794277906025310898, -0.7998128361456362523 ) ) ;
#99346=ORIENTED_EDGE ( 'NONE', *, *, #20908, .F. ) ;
#99350=CARTESIAN_POINT ( 'NONE',  ( -7.065207446052809814, 9.336104335185325453, -1.443375672974066548 ) ) ;
#99358=CARTESIAN_POINT ( 'NONE',  ( 5.506019780925567986, 8.477421273504887722, -1.082531754730548412 ) ) ;
#99361=CARTESIAN_POINT ( 'NONE',  ( -3.637330350216213759, 7.465578851886037093, -0.7998128361456481317 ) ) ;
#99371=CARTESIAN_POINT ( 'NONE',  ( 5.598591087800349086, 5.496387455380669529, -0.7998128361456481317 ) ) ;
#99392=CARTESIAN_POINT ( 'NONE',  ( 5.044982899572335810, 7.898304261840563001, 1.131119777890549516 ) ) ;
#99401=CARTESIAN_POINT ( 'NONE',  ( 5.345657705538078730, 9.458627433094950021, 0.7998128361456331437 ) ) ;
#99408=CARTESIAN_POINT ( 'NONE',  ( 3.743459811148990291, 7.381470523066878009, -0.7216878364870338292 ) ) ;
#99411=CARTESIAN_POINT ( 'NONE',  ( 4.909461021924231616, 8.741805268971372556, 0.7216878364870317197 ) ) ;
#99423=CARTESIAN_POINT ( 'NONE',  ( -5.478903473698241378, 9.406154796041011679, -0.7216878364870338292 ) ) ;
#99441=ORIENTED_EDGE ( 'NONE', *, *, #25840, .F. ) ;
#99445=EDGE_CURVE ( 'NONE', #36910, #200036, #186464, .T. ) ;
#99457=CARTESIAN_POINT ( 'NONE',  ( 6.530187263637528439, 7.647581891445782709, -1.199719254218452047 ) ) ;
#99459=CARTESIAN_POINT ( 'NONE',  ( 4.688087255275310561, 8.691461907788344377, -0.7998128361456381397 ) ) ;
#99471=CARTESIAN_POINT ( 'NONE',  ( -7.919371124158132602, 8.411890197705517380, -0.7216878364870338292 ) ) ;
#99474=CARTESIAN_POINT ( 'NONE',  ( 6.333067150914820864, 6.561202228921677815, 0.7216878364870328300 ) ) ;
#99490=CARTESIAN_POINT ( 'NONE',  ( -5.302647476720585118, 9.200522799567075083, 0.000000000000000000 ) ) ;
#99492=CARTESIAN_POINT ( 'NONE',  ( -5.668717624289589807, 5.786127781192186958, 0.7216878364870257245 ) ) ;
#99508=EDGE_LOOP ( 'NONE', ( #49030, #133047, #141103, #62054, #107320, #136632 ) ) ;
#99518=CARTESIAN_POINT ( 'NONE',  ( -4.085803189671902480, 5.860132702740892263, -1.599625672291271394 ) ) ;
#99526=DIRECTION ( 'NONE',  ( 0.000000000000000000, 0.000000000000000000, 1.000000000000000000 ) ) ;
#99527=CARTESIAN_POINT ( 'NONE',  ( 7.005397802120315376, 5.950282834973755541, -2.500000000000000444 ) ) ;
#99528=CARTESIAN_POINT ( 'NONE',  ( -5.281148723220589147, 7.765029056575591504, -1.308346332658766986 ) ) ;
#99544=CARTESIAN_POINT ( 'NONE',  ( 7.049313524462606395, 7.188896964819984525, 0.000000000000000000 ) ) ;
#99568=CARTESIAN_POINT ( 'NONE',  ( 7.666209513884374438, 7.908608952478760834, 0.7998128361456281477 ) ) ;
#99569=CARTESIAN_POINT ( 'NONE',  ( 5.520104819419390907, 6.469152373191302985, 1.199719254218452935 ) ) ;
#99571=CARTESIAN_POINT ( 'NONE',  ( 5.228604516725597229, 6.129068686715179126, -1.199719254218450271 ) ) ;
#99574=DIRECTION ( 'NONE',  ( 0.000000000000000000, 0.000000000000000000, 1.000000000000000000 ) ) ;
#99583=CARTESIAN_POINT ( 'NONE',  ( 5.583942420111207561, 7.395222456726187943, -1.242479836444350783 ) ) ;
#99584=CARTESIAN_POINT ( 'NONE',  ( -6.278834536460198734, 6.497930845391236332, 0.7216878364870257245 ) ) ;
#99585=CARTESIAN_POINT ( 'NONE',  ( 5.587368702607580673, 5.691220705896524734, -0.7216878364870458196 ) ) ;
#99600=CARTESIAN_POINT ( 'NONE',  ( -5.606595252507366567, 5.572856915785063592, -0.3451608010808376870 ) ) ;
#99608=CARTESIAN_POINT ( 'NONE',  ( 5.337069745634900997, 6.255611453776062980, 1.199719254218452047 ) ) ;
#99610=CARTESIAN_POINT ( 'NONE',  ( 5.086243903782109221, 5.962981304947771122, -1.199719254218452047 ) ) ;
#99618=SPHERICAL_SURFACE ( 'NONE', #169420, 0.08000000000000000167 ) ;
#99629=CARTESIAN_POINT ( 'NONE',  ( -4.894942725380222015, 7.314395937714276208, -1.216140164365722143 ) ) ;
#99637=CARTESIAN_POINT ( 'NONE',  ( 6.690022453700429139, 6.769724048930809701, 0.7998128361456331437 ) ) ;
#99642=CARTESIAN_POINT ( 'NONE',  ( -6.316227922719336974, 6.878322274790401814, 0.7073135764556655047 ) ) ;
#99643=CARTESIAN_POINT ( 'NONE',  ( 4.552505719138623341, 8.533283448962240669, 0.7998128361456341429 ) ) ;
#99653=CIRCLE ( 'NONE', #155017, 3.970406073902761790 ) ;
#99671=ORIENTED_EDGE ( 'NONE', *, *, #38147, .F. ) ;
#99675=CARTESIAN_POINT ( 'NONE',  ( -5.661411662158206681, 8.762674818229999829, -1.199719254218452047 ) ) ;
#99677=CARTESIAN_POINT ( 'NONE',  ( 6.984385409695311964, 8.177479728513226576, 1.199719254218452935 ) ) ;
#99681=B_SPLINE_CURVE_WITH_KNOTS ( 'NONE', 3,
 ( #112259, #44008, #178273, #63442, #29883, #145798, #129592, #195580, #47216, #80762, #146851, #168398, #52511, #198738, #182497, #100196, #115451, #134858, #33070, #99148 ),
 .UNSPECIFIED., .F., .F.,
 ( 4, 2, 2, 1, 2, 2, 1, 2, 2, 2, 4 ),
 ( 0.6057107753108389447, 0.6187864442436151746, 0.6253242787100032896, 0.6261415080183017068, 0.6265501226724510264, 0.6269587373266002350, 0.6285931959431972915, 0.6318621131763914045, 0.6580134510419443084, 0.6841647889074973232, 0.7103161267730502271 ),
 .UNSPECIFIED. ) ;
#99682=CARTESIAN_POINT ( 'NONE',  ( -4.095971805104331231, 5.871996087412059140, 1.443375672974065660 ) ) ;
#99686=DIRECTION ( 'NONE',  ( 0.7592566023653005702, 0.6507913734559639396, 0.000000000000000000 ) ) ;
#99691=CARTESIAN_POINT ( 'NONE',  ( -6.297925439369929101, 6.970297724909739756, -0.9421744322617598977 ) ) ;
#99708=CARTESIAN_POINT ( 'NONE',  ( 5.397554552016204710, 9.311247720745345902, 0.7216878364870317197 ) ) ;
#99721=CARTESIAN_POINT ( 'NONE',  ( -5.641601317062259646, 5.754492089426966217, -0.7216878364870338292 ) ) ;
#99723=CARTESIAN_POINT ( 'NONE',  ( 6.008198349511364000, 7.038594824965278995, 1.199719254218453823 ) ) ;
#99728=CARTESIAN_POINT ( 'NONE',  ( -5.178288325776719603, 5.006034233019745372, 0.000000000000000000 ) ) ;
#99737=VERTEX_POINT ( 'NONE', #26897 ) ;
#99772=CARTESIAN_POINT ( 'NONE',  ( 2.929970594329034395, 6.432399770110250437, -0.7216878364870338292 ) ) ;
#99777=CARTESIAN_POINT ( 'NONE',  ( 4.390861645979372341, 6.216034235099629157, -1.599625672291269396 ) ) ;
#99779=DIRECTION ( 'NONE',  ( 0.000000000000000000, 0.000000000000000000, 1.000000000000000000 ) ) ;
#99783=CARTESIAN_POINT ( 'NONE',  ( -5.519577934094894722, 7.532869904567736974, 1.443375672974058777 ) ) ;
#99784=CARTESIAN_POINT ( 'NONE',  ( 4.632188385292959509, 8.431376123677011947, -0.5646427909330701267 ) ) ;
#99788=ORIENTED_EDGE ( 'NONE', *, *, #164365, .T. ) ;
#99789=CARTESIAN_POINT ( 'NONE',  ( -5.589704470584107909, 9.743348658981940247, -0.7998128361456362523 ) ) ;
#99795=CARTESIAN_POINT ( 'NONE',  ( 4.726684935852882852, 4.891486930089099516, -0.8194250277325197951 ) ) ;
#99796=DIRECTION ( 'NONE',  ( -0.6029061840396265914, 0.7978120914393163066, 0.000000000000000000 ) ) ;
#99798=CARTESIAN_POINT ( 'NONE',  ( -4.959250327548641479, 9.007818825440551791, -0.7998128361456362523 ) ) ;
#99801=CARTESIAN_POINT ( 'NONE',  ( 4.613585901703492809, 8.466914752176691650, -0.2784627230535564046 ) ) ;
#99806=CARTESIAN_POINT ( 'NONE',  ( 7.991605200612358573, 8.288237253661408843, 0.7998128361456281477 ) ) ;
#99813=CARTESIAN_POINT ( 'NONE',  ( -4.142898457427624415, 6.991076079377632091, 1.199719254218452935 ) ) ;
#99815=AXIS2_PLACEMENT_3D ( 'NONE', #45004, #156615, #172869 ) ;
#99818=CARTESIAN_POINT ( 'NONE',  ( -6.622231685632140596, 6.690634819517756959, 0.000000000000000000 ) ) ;
#99820=DIRECTION ( 'NONE',  ( 0.000000000000000000, 0.000000000000000000, 1.000000000000000000 ) ) ;
#99822=CARTESIAN_POINT ( 'NONE',  ( 5.844973620822823790, 9.833236634353070826, 0.7216878364870317197 ) ) ;
#99824=CARTESIAN_POINT ( 'NONE',  ( -6.902509602688818191, 9.146290184594002781, -1.443375672974066548 ) ) ;
#99830=CARTESIAN_POINT ( 'NONE',  ( 6.180537922983273091, 8.303989891604203422, -1.599625672291281386 ) ) ;
#99839=ADVANCED_FACE ( 'NONE', ( #191523 ), #159045, .F. ) ;
#99846=CARTESIAN_POINT ( 'NONE',  ( 6.252685474373055996, 7.003816019006632310, -0.9791501464874209359 ) ) ;
#99850=( BOUNDED_CURVE ( )  B_SPLINE_CURVE ( 2, ( #69517, #119426, #18646, #84724, #150813, #66311, #135625 ),
 .UNSPECIFIED., .F., .T. ) 
 B_SPLINE_CURVE_WITH_KNOTS ( ( 3, 2, 2, 3 ),
 ( 0.2999999999999999889, 0.3083333333333334036, 0.3166666666666667629, 0.3250000000000001776 ),
 .UNSPECIFIED. ) 
 CURVE ( )  GEOMETRIC_REPRESENTATION_ITEM ( )  RATIONAL_B_SPLINE_CURVE ( ( 1.000000000000000000, 0.8660254037844387076, 1.000000000000000000, 0.8660254037844387076, 1.000000000000000000, 0.8660254037844360431, 1.000000000000002665 ) ) 
 REPRESENTATION_ITEM ( '' )  );
#99862=CARTESIAN_POINT ( 'NONE',  ( -5.939880696118548187, 6.102484698325975288, 0.000000000000000000 ) ) ;
#99869=CARTESIAN_POINT ( 'NONE',  ( 5.820193082016415609, 10.01225203898631655, 0.000000000000000000 ) ) ;
#99874=CARTESIAN_POINT ( 'NONE',  ( -5.018153416333300143, 7.915986710968343054, -1.079799343345327234 ) ) ;
#99878=EDGE_CURVE ( 'NONE', #75117, #138779, #9247, .T. ) ;
#99894=CARTESIAN_POINT ( 'NONE',  ( -5.991777542596674166, 5.955104985976372944, 0.000000000000000000 ) ) ;
#99896=CARTESIAN_POINT ( 'NONE',  ( 8.188198428010544205, 8.517596018959260107, 0.000000000000000000 ) ) ;
#99905=ORIENTED_EDGE ( 'NONE', *, *, #33468, .F. ) ;
#99908=CARTESIAN_POINT ( 'NONE',  ( 7.042534447655770080, 7.180988041878682004, -0.7998128361456341429 ) ) ;
#99910=CARTESIAN_POINT ( 'NONE',  ( 6.983858524370782028, 8.280828045588322084, 1.082531754730549967 ) ) ;
#99925=CARTESIAN_POINT ( 'NONE',  ( -5.960744811863571968, 6.983232364376142698, 1.199719254218452935 ) ) ;
#99926=CARTESIAN_POINT ( 'NONE',  ( 3.528865121306874464, 7.339036084825155015, -0.7998128361456362523 ) ) ;
#99935=CARTESIAN_POINT ( 'NONE',  ( -7.937372586157736443, 8.224965870130965584, 0.7998128361456341429 ) ) ;
#99936=CARTESIAN_POINT ( 'NONE',  ( 7.178115983792402233, 7.339166500704784823, 0.7998128361456281477 ) ) ;
#99942=CARTESIAN_POINT ( 'NONE',  ( 5.551137550152489553, 5.441024994791534120, 0.7998128361456352531 ) ) ;
#99948=CARTESIAN_POINT ( 'NONE',  ( -6.472689817967896886, 6.776322833669464529, -0.2902398332882798471 ) ) ;
#99957=CARTESIAN_POINT ( 'NONE',  ( -4.217995187182965289, 6.014356699837137832, 1.443375672974065660 ) ) ;
#99970=CARTESIAN_POINT ( 'NONE',  ( -6.392116398764494001, 6.567141947923602174, 2.438447736781127695 ) ) ;
#99987=CARTESIAN_POINT ( 'NONE',  ( 4.817943484809818600, 6.714296380401858499, 1.599625672291269396 ) ) ;
#100007=CARTESIAN_POINT ( 'NONE',  ( 0.001169091720979649387, 3.496131414459332731, 2.003411285068362968 ) ) ;
#100008=CARTESIAN_POINT ( 'NONE',  ( 4.960304097753311936, 6.880383762169266504, 1.599625672291268286 ) ) ;
#100009=CARTESIAN_POINT ( 'NONE',  ( -4.177320726786328819, 5.966903162707725805, -1.443375672974066548 ) ) ;
#100023=EDGE_CURVE ( 'NONE', #160372, #19980, #29980, .T. ) ;
#100036=CARTESIAN_POINT ( 'NONE',  ( -6.954406449166956605, 7.078172043641714595, -0.7998128361456362523 ) ) ;
#100050=CARTESIAN_POINT ( 'NONE',  ( -7.774674742793745708, 8.035151719539642912, 0.7998128361456341429 ) ) ;
#100061=FACE_OUTER_BOUND ( 'NONE', #131482, .T. ) ;
#100062=CARTESIAN_POINT ( 'NONE',  ( -6.283277845290492714, 6.295188672452495915, -0.7998128361456362523 ) ) ;
#100065=CARTESIAN_POINT ( 'NONE',  ( -7.295696057929500711, 7.684269287105433222, 0.7216878364870317197 ) ) ;
#100068=CARTESIAN_POINT ( 'NONE',  ( 4.882344714252594642, 4.868692719482363707, 0.000000000000000000 ) ) ;
#100069=CARTESIAN_POINT ( 'NONE',  ( -3.811250578772981346, 6.500190537660166079, -1.082531754730546636 ) ) ;
#100089=CARTESIAN_POINT ( 'NONE',  ( 6.184762415132515123, 7.051423785172313607, -1.050594063207562545 ) ) ;
#100095=CARTESIAN_POINT ( 'NONE',  ( 5.835368547082574686, 7.298705356223742058, -1.329342603381425958 ) ) ;
#100096=VERTEX_POINT ( 'NONE', #35424 ) ;
#100098=( GEOMETRIC_REPRESENTATION_CONTEXT ( 3 ) GLOBAL_UNCERTAINTY_ASSIGNED_CONTEXT ( ( #37695 ) ) GLOBAL_UNIT_ASSIGNED_CONTEXT ( ( #169790, #183903, #33386 ) ) REPRESENTATION_CONTEXT ( 'NONE', 'WORKASPACE' ) );
#100109=CARTESIAN_POINT ( 'NONE',  ( 5.348725299209624140, 7.591689785053232775, -1.238827213252717163 ) ) ;
#100125=CARTESIAN_POINT ( 'NONE',  ( -5.498713818794216834, 8.572860667638675380, -1.199719254218452047 ) ) ;
#100137=CARTESIAN_POINT ( 'NONE',  ( 3.413620815590684199, 7.204584394822967752, 0.7998128361456281477 ) ) ;
#100139=CARTESIAN_POINT ( 'NONE',  ( 6.964048179274811012, 8.153752959689313684, 1.199719254218452047 ) ) ;
#100144=CARTESIAN_POINT ( 'NONE',  ( -7.282137903871469753, 8.628820655005750240, 1.082531754730549078 ) ) ;
#100150=CARTESIAN_POINT ( 'NONE',  ( 4.895902867866261055, 4.884510565364971413, -0.7216878364870458196 ) ) ;
#100160=DIRECTION ( 'NONE',  ( 0.000000000000000000, 0.000000000000000000, 1.000000000000000000 ) ) ;
#100166=CARTESIAN_POINT ( 'NONE',  ( -5.139949633356594383, 9.010708648975750634, 0.000000000000000000 ) ) ;
#100167=CARTESIAN_POINT ( 'NONE',  ( 5.722950238744209273, 6.809768379023969587, 1.082531754730549967 ) ) ;
#100177=CARTESIAN_POINT ( 'NONE',  ( -5.483346782084204563, 5.361935765378481378, 0.000000000000000000 ) ) ;
#100178=CARTESIAN_POINT ( 'NONE',  ( -5.126391479742927970, 8.994890803093138487, 0.7216878364870267237 ) ) ;
#100179=CARTESIAN_POINT ( 'NONE',  ( 1.872311050889111650, 2.480935488296869273, -2.470734331491561520 ) ) ;
#100182=CARTESIAN_POINT ( 'NONE',  ( 5.031484404002879884, 6.963427452793765404, 1.443375672974065660 ) ) ;
#100196=CARTESIAN_POINT ( 'NONE',  ( -4.891544523420352952, 7.514763430510271291, 1.198184914803653633 ) ) ;
#100200=CARTESIAN_POINT ( 'NONE',  ( -4.782994330570982555, 8.802186828966616972, 0.000000000000000000 ) ) ;
#100211=CARTESIAN_POINT ( 'NONE',  ( 5.401997860402196316, 5.267028690082820930, 0.000000000000000000 ) ) ;
#100246=CYLINDRICAL_SURFACE ( 'NONE', #170419, 1.250000000000000000 ) ;
#100249=CARTESIAN_POINT ( 'NONE',  ( 4.882344714696929877, 8.710169577206153591, -0.7216878364870458196 ) ) ;
#100255=CARTESIAN_POINT ( 'NONE',  ( 7.146556367734776316, 7.510272981878305387, 0.7216878364870267237 ) ) ;
#100271=CARTESIAN_POINT ( 'NONE',  ( -4.782994330570982555, 8.802186828966616972, 0.000000000000000000 ) ) ;
#100281=CARTESIAN_POINT ( 'NONE',  ( 5.528692779322568640, 9.672168352510192690, 0.7998128361456341429 ) ) ;
#100287=CARTESIAN_POINT ( 'NONE',  ( -5.589704470584107909, 9.743348658981940247, -0.7998128361456362523 ) ) ;
#100293=CARTESIAN_POINT ( 'NONE',  ( -6.943184063974186415, 7.273005294157565359, -0.7216878364870338292 ) ) ;
#100296=CARTESIAN_POINT ( 'NONE',  ( -7.123883369337781879, 7.275895117174344229, 0.7998128361456341429 ) ) ;
#100313=CARTESIAN_POINT ( 'NONE',  ( -6.495588733991166208, 6.829233952181008149, 0.6942782964225120423 ) ) ;
#100317=CARTESIAN_POINT ( 'NONE',  ( -3.174017359375036929, 6.717120995997236221, 0.7216878364870338292 ) ) ;
#100319=CARTESIAN_POINT ( 'NONE',  ( -5.596483547390937119, 9.751257581923240991, 0.000000000000000000 ) ) ;
#100320=CARTESIAN_POINT ( 'NONE',  ( 4.598150373690133463, 5.393538853173795111, -1.199719254218452047 ) ) ;
#100321=CARTESIAN_POINT ( 'NONE',  ( -5.113360211009450040, 5.994616996712990975, -1.199719254218453823 ) ) ;
#100322=CARTESIAN_POINT ( 'NONE',  ( -6.469175572376043348, 7.576401584974034265, 1.199719254218452047 ) ) ;
#100339=CARTESIAN_POINT ( 'NONE',  ( -5.534330892379054845, 5.955497452077792353, -0.9177112583351170194 ) ) ;
#100342=CARTESIAN_POINT ( 'NONE',  ( -3.147653791585727667, 8.920000000000001705, -2.499999999999998668 ) ) ;
#100372=ORIENTED_EDGE ( 'NONE', *, *, #23766, .T. ) ;
#100375=CARTESIAN_POINT ( 'NONE',  ( 4.329849954717849947, 6.144853928627882489, 1.599625672291262513 ) ) ;
#100377=CARTESIAN_POINT ( 'NONE',  ( 4.647606103345025552, 8.407977806742819027, 0.6343139517084724899 ) ) ;
#100388=CARTESIAN_POINT ( 'NONE',  ( 4.702859892337409420, 8.240897811179339172, 0.6291740908887258898 ) ) ;
#100391=CARTESIAN_POINT ( 'NONE',  ( 6.373741612200160667, 9.489763409991955001, 1.082531754730549078 ) ) ;
#100395=ORIENTED_EDGE ( 'NONE', *, *, #148090, .F. ) ;
#100396=CARTESIAN_POINT ( 'NONE',  ( -5.152980901645737077, 8.169505597632108262, -1.199719254218453823 ) ) ;
#100403=CARTESIAN_POINT ( 'NONE',  ( -6.739811759324828344, 8.956476034002674780, -1.443375672974066548 ) ) ;
#100405=CARTESIAN_POINT ( 'NONE',  ( -5.276698331947687670, 7.500886158655696967, 1.250003795154420061 ) ) ;
#100407=DIRECTION ( 'NONE',  ( -0.5620411653127326268, -0.8271092603120251407, 0.000000000000000000 ) ) ;
#100410=CARTESIAN_POINT ( 'NONE',  ( 6.400857919427532572, 6.640291458853147866, -0.7216878364870458196 ) ) ;
#100413=CARTESIAN_POINT ( 'NONE',  ( -6.147696309153835692, 6.137010213626392208, 0.7998128361456281477 ) ) ;
#100423=CARTESIAN_POINT ( 'NONE',  ( 4.472210567661338843, 6.310941310395290493, 1.599625672291261402 ) ) ;
#100424=CARTESIAN_POINT ( 'NONE',  ( 5.357406976055401948, 6.279338222599979424, 1.199719254218452935 ) ) ;
#100437=ORIENTED_EDGE ( 'NONE', *, *, #167257, .T. ) ;
#100448=CARTESIAN_POINT ( 'NONE',  ( 6.373214726875630731, 9.593111727067046957, 1.199719254218452047 ) ) ;
#100455=CARTESIAN_POINT ( 'NONE',  ( 6.424584688029230328, 8.588711117491191871, 1.599625672291268286 ) ) ;
#100460=CARTESIAN_POINT ( 'NONE',  ( 4.990809943606266508, 6.915973915664348937, -1.443375672974068769 ) ) ;
#100464=CARTESIAN_POINT ( 'NONE',  ( 6.373741612200171325, 7.569024981389272710, 1.082531754730549967 ) ) ;
#100476=CARTESIAN_POINT ( 'NONE',  ( 6.266472554743693912, 6.895788939045927712, 0.7740814723603481884 ) ) ;
#100477=CARTESIAN_POINT ( 'NONE',  ( -5.966997003790228682, 8.054858819212300958, -1.443375672974066548 ) ) ;
#100485=DIRECTION ( 'NONE',  ( 0.6507913734559596097, 0.7592566023653043450, 0.000000000000000000 ) ) ;
#100510=ORIENTED_EDGE ( 'NONE', *, *, #106930, .F. ) ;
#100514=CARTESIAN_POINT ( 'NONE',  ( 4.993145711582793744, 9.047363440147082159, -0.7998128361456481317 ) ) ;
#100515=CARTESIAN_POINT ( 'NONE',  ( -4.299344108864988634, 8.030002203735456590, -0.7216878364870615847 ) ) ;
#100516=CARTESIAN_POINT ( 'NONE',  ( 6.013923656113508542, 9.173938811177871244, -1.199719254218452047 ) ) ;
#100530=CARTESIAN_POINT ( 'NONE',  ( -5.309953438407606363, 6.223975762010839574, 1.199719254218452935 ) ) ;
#100532=EDGE_CURVE ( 'NONE', #45344, #30079, #158004, .T. ) ;
#100533=CARTESIAN_POINT ( 'NONE',  ( 4.543390873910894356, 8.314723429622471684, 0.7216878364870317197 ) ) ;
#100541=CARTESIAN_POINT ( 'NONE',  ( -5.008811405605897882, 4.808311159487113073, 0.7998128361456281477 ) ) ;
#100547=CARTESIAN_POINT ( 'NONE',  ( -6.617788377246193399, 8.814115421577600529, -1.443375672974066548 ) ) ;
#100549=CARTESIAN_POINT ( 'NONE',  ( -5.858531774880906262, 6.967946837850073294, 1.082531754730549078 ) ) ;
#100575=CARTESIAN_POINT ( 'NONE',  ( -4.573896719763875574, 6.429575154514868274, -1.599625672291271394 ) ) ;
#100578=CARTESIAN_POINT ( 'NONE',  ( 5.113477980681966351, 7.841710745841885100, -1.181108758208327725 ) ) ;
#100587=CARTESIAN_POINT ( 'NONE',  ( -4.979135478818752958, 8.054126424104152804, -1.119915745145182440 ) ) ;
#100603=CARTESIAN_POINT ( 'NONE',  ( 6.225128807330042591, 7.291680359087043151, -1.199719254218452047 ) ) ;
#100609=CARTESIAN_POINT ( 'NONE',  ( 1.890105089649192216, 8.991484090553308661, -0.7749999999999996891 ) ) ;
#100625=CARTESIAN_POINT ( 'NONE',  ( 7.517069824134078537, 7.734612647770044092, 0.000000000000000000 ) ) ;
#100626=CARTESIAN_POINT ( 'NONE',  ( 5.899733120602060232, 6.912052057904395141, -1.199719254218452047 ) ) ;
#100628=CARTESIAN_POINT ( 'NONE',  ( 5.041653019435334393, 6.975290837464928728, -1.599625672291269396 ) ) ;
#100641=CARTESIAN_POINT ( 'NONE',  ( 4.613585901703492809, 8.466914752176691650, -0.2784627230535564046 ) ) ;
#100643=CARTESIAN_POINT ( 'NONE',  ( -4.611181641979265500, 8.393812659035525314, 0.000000000000000000 ) ) ;
#100644=CARTESIAN_POINT ( 'NONE',  ( 4.367134877377630175, 7.148722219365612141, -1.082531754730548412 ) ) ;
#100663=CARTESIAN_POINT ( 'NONE',  ( -4.136646265500964148, 6.879818838842817641, -1.082531754730551743 ) ) ;
#100668=CARTESIAN_POINT ( 'NONE',  ( 6.261886844665240481, 8.398896966899865646, 1.599625672291268286 ) ) ;
#100688=CARTESIAN_POINT ( 'NONE',  ( -5.753162853856577108, 6.626890507991352486, -1.008109661457639694 ) ) ;
#100698=CARTESIAN_POINT ( 'NONE',  ( 5.643937085038755797, 9.806620042512378177, -0.7998128361456481317 ) ) ;
#100703=CARTESIAN_POINT ( 'NONE',  ( -5.710744021720588925, 7.310394840978843511, 1.216594670743395445 ) ) ;
#100704=CARTESIAN_POINT ( 'NONE',  ( 6.363572996767764778, 8.517530811019446091, -1.599625672291283607 ) ) ;
#100723=SPHERICAL_SURFACE ( 'NONE', #12156, 0.08000000000000000167 ) ;
#100730=EDGE_LOOP ( 'NONE', ( #46718, #104722, #200049, #162968 ) ) ;
#100734=CARTESIAN_POINT ( 'NONE',  ( -5.121948170912633991, 9.197632976031879792, -0.7998128361456362523 ) ) ;
#100736=CARTESIAN_POINT ( 'NONE',  ( 5.742760583840166966, 8.857581893525663830, 1.199719254218452047 ) ) ;
#100739=CARTESIAN_POINT ( 'NONE',  ( -5.004368097219957789, 5.011053332944274352, 0.000000000000000000 ) ) ;
#100755=CARTESIAN_POINT ( 'NONE',  ( 5.993586425693011144, 9.150212042353954800, -1.199719254218452047 ) ) ;
#100764=CARTESIAN_POINT ( 'NONE',  ( 7.512626515748109135, 8.897724035528543851, 1.082531754730549967 ) ) ;
#100777=CARTESIAN_POINT ( 'NONE',  ( -4.828112100242283766, 7.686528979374367410, -1.082531754730549967 ) ) ;
#100780=CARTESIAN_POINT ( 'NONE',  ( 5.956828388357757298, 8.042995434541133193, 1.599625672291269396 ) ) ;
#100783=CARTESIAN_POINT ( 'NONE',  ( -5.935437387732586778, 10.14670372898850381, -0.7998128361456362523 ) ) ;
#100785=CARTESIAN_POINT ( 'NONE',  ( -4.842197138736131556, 5.678260079060780008, 1.199719254218452935 ) ) ;
#100787=DIRECTION ( 'NONE',  ( 1.000000000000000000, 0.000000000000000000, 0.000000000000000000 ) ) ;
#100797=CARTESIAN_POINT ( 'NONE',  ( -0.3898781600097490641, 2.718687676624831351, -1.963392457971794514 ) ) ;
#100825=CARTESIAN_POINT ( 'NONE',  ( 5.248414862265931902, 5.295774558831261913, 0.000000000000000000 ) ) ;
#100830=CARTESIAN_POINT ( 'NONE',  ( 3.040771591214902259, 6.769593633051179005, -0.7998128361456362523 ) ) ;
#100833=CARTESIAN_POINT ( 'NONE',  ( -6.445975688654487001, 6.485002823043819475, -0.7998128361456362523 ) ) ;
#100837=CARTESIAN_POINT ( 'NONE',  ( -4.895902867866254837, 7.765618208269001066, 1.082531754730549967 ) ) ;
#100838=CARTESIAN_POINT ( 'NONE',  ( 0.4800000000000000933, 2.999999999999999112, -2.500000000000000444 ) ) ;
#100843=CARTESIAN_POINT ( 'NONE',  ( -6.720001414228860881, 7.869031733802326123, -1.199719254218452047 ) ) ;
#100852=CARTESIAN_POINT ( 'NONE',  ( -6.414942957921379474, 7.513130201443591005, -1.199719254218452047 ) ) ;
#100853=VERTEX_POINT ( 'NONE', #143660 ) ;
#100854=CARTESIAN_POINT ( 'NONE',  ( 4.614865537624940117, 8.465324746759504748, 0.2878883051726736086 ) ) ;
#100860=CARTESIAN_POINT ( 'NONE',  ( 5.332099551924443404, 9.442809587212341427, 0.000000000000000000 ) ) ;
#100867=CARTESIAN_POINT ( 'NONE',  ( -3.820365424000704557, 7.679119771301277098, -0.7998128361456481317 ) ) ;
#100871=CARTESIAN_POINT ( 'NONE',  ( -6.961185525973791144, 7.086080966583015339, 0.7998128361456341429 ) ) ;
#100875=CARTESIAN_POINT ( 'NONE',  ( 7.146556367734771875, 8.470642196179646533, 1.082531754730549967 ) ) ;
#100877=CARTESIAN_POINT ( 'NONE',  ( -7.282137903871469753, 8.628820655005750240, 1.082531754730549078 ) ) ;
#100883=CARTESIAN_POINT ( 'NONE',  ( 5.155843554946782703, 9.237177590738404831, -0.7998128361456481317 ) ) ;
#100896=CARTESIAN_POINT ( 'NONE',  ( 6.546060204425600659, 6.805396270974036987, -0.4351356575816138772 ) ) ;
#100924=CARTESIAN_POINT ( 'NONE',  ( -6.005252172667468358, 7.091917859149008407, -1.064983193601161338 ) ) ;
#100941=CARTESIAN_POINT ( 'NONE',  ( -6.168033539574333979, 6.160736982450306876, 0.7998128361456281477 ) ) ;
#100954=CARTESIAN_POINT ( 'NONE',  ( 6.367489420273535039, 7.457767740854454708, -1.199719254218452047 ) ) ;
#100957=CARTESIAN_POINT ( 'NONE',  ( 5.519577934094840543, 9.453608333170423705, 0.7216878364870317197 ) ) ;
#100972=CARTESIAN_POINT ( 'NONE',  ( -5.581116510680924847, 6.540332679663050541, -1.199719254218453823 ) ) ;
#100973=CARTESIAN_POINT ( 'NONE',  ( 5.529746549527311039, 7.544733289238903851, -1.599625672291281386 ) ) ;
#100982=CARTESIAN_POINT ( 'NONE',  ( -3.492107083971660586, 6.231819477012331632, 1.199719254218452935 ) ) ;
#100983=CARTESIAN_POINT ( 'NONE',  ( 5.083381250481017410, 4.895309311841474553, 0.7998128361456352531 ) ) ;
#100985=CARTESIAN_POINT ( 'NONE',  ( -7.006746397889348721, 6.052176462752765218, -2.500000000000000000 ) ) ;
#100989=ORIENTED_EDGE ( 'NONE', *, *, #207178, .F. ) ;
#100991=CARTESIAN_POINT ( 'NONE',  ( 3.230585741806197841, 6.991043475407723307, 0.7998128361456271485 ) ) ;
#100993=CARTESIAN_POINT ( 'NONE',  ( 6.384963997392946844, 6.413822516572072807, 0.7998128361456352531 ) ) ;
#100999=CARTESIAN_POINT ( 'NONE',  ( -6.454776619733716636, 6.787828609132271929, -0.3692292702514640146 ) ) ;
#101009=CARTESIAN_POINT ( 'NONE',  ( -3.485854892044994102, 7.080931450778859215, -0.7216878364870458196 ) ) ;
#101018=CARTESIAN_POINT ( 'NONE',  ( 4.095971805104288599, 5.871996087412059140, 1.443375672974058777 ) ) ;
#101028=CARTESIAN_POINT ( 'NONE',  ( -3.469446951953614189E-15, 8.920000000000001705, -2.420000000000000373 ) ) ;
#101033=ADVANCED_FACE ( 'NONE', ( #125313 ), #191272, .F. ) ;
#101039=CARTESIAN_POINT ( 'NONE',  ( 4.549643065837591038, 7.465611455855944101, -1.199719254218452047 ) ) ;
#101061=CARTESIAN_POINT ( 'NONE',  ( 4.366607992053101128, 7.252070536440704096, -1.199719254218448494 ) ) ;
#101062=CARTESIAN_POINT ( 'NONE',  ( -4.285785955695645910, 7.053815144069948140, 1.082531754730549967 ) ) ;
#101085=CARTESIAN_POINT ( 'NONE',  ( -7.144220599758281054, 7.299621885998258897, 0.7998128361456341429 ) ) ;
#101087=CARTESIAN_POINT ( 'NONE',  ( 6.739811759324814133, 8.956476034002680109, -1.443375672974078761 ) ) ;
#101100=CARTESIAN_POINT ( 'NONE',  ( -7.099629715411508890, 8.311931418515415615, 1.199719254218452047 ) ) ;
#101108=CARTESIAN_POINT ( 'NONE',  ( 6.222152418221221559, 7.023474430343600083, -1.033429630759775675 ) ) ;
#101112=CARTESIAN_POINT ( 'NONE',  ( -4.423703259808839938, 8.383013913077441259, 0.7998128361456352531 ) ) ;
#101115=CARTESIAN_POINT ( 'NONE',  ( -6.617788377246193399, 8.814115421577600529, -1.443375672974066548 ) ) ;
#101119=CARTESIAN_POINT ( 'NONE',  ( 5.045042557616584489, 5.058506870073687267, 0.000000000000000000 ) ) ;
#101120=CARTESIAN_POINT ( 'NONE',  ( -3.133342898089680695, 6.669667457830990465, 0.7216878364870338292 ) ) ;
#101134=CARTESIAN_POINT ( 'NONE',  ( 0.1024722964814587939, 2.599067505215466589, 1.999601597966877309 ) ) ;
#101139=CARTESIAN_POINT ( 'NONE',  ( 6.580239226864286195, 6.782991656975736028, -0.2881480849740332140 ) ) ;
#101146=ORIENTED_EDGE ( 'NONE', *, *, #76635, .T. ) ;
#101160=CARTESIAN_POINT ( 'NONE',  ( 6.435429789636040177, 6.784273175954743884, -0.4071148367965071735 ) ) ;
#101176=CARTESIAN_POINT ( 'NONE',  ( 7.095713291905693332, 9.371694488680407886, 1.599625672291268286 ) ) ;
#101179=CARTESIAN_POINT ( 'NONE',  ( -6.642568916052639771, 6.714361588341672515, 0.000000000000000000 ) ) ;
#101192=CARTESIAN_POINT ( 'NONE',  ( 6.737475991348287785, 6.825086509519945999, -0.7998128361456481317 ) ) ;
#101195=CARTESIAN_POINT ( 'NONE',  ( 7.842465510862060896, 8.114240948952696542, 0.000000000000000000 ) ) ;
#101201=CARTESIAN_POINT ( 'NONE',  ( -5.112833325684904118, 8.979072956692109031, -0.7216878364870338292 ) ) ;
#101206=EDGE_CURVE ( 'NONE', #29321, #114168, #171288, .T. ) ;
#101207=CARTESIAN_POINT ( 'NONE',  ( 6.526270840131753737, 8.707344961610770540, -1.599625672291283607 ) ) ;
#101210=CIRCLE ( 'NONE', #104644, 7.424569270082293393 ) ;
#101223=CARTESIAN_POINT ( 'NONE',  ( -4.638297949650955765, 8.425448351319163365, 0.7216878364870267237 ) ) ;
#101224=CARTESIAN_POINT ( 'NONE',  ( 4.719646871332936477, 8.520355426614829142, -0.7216878364870357165 ) ) ;
#101226=CARTESIAN_POINT ( 'NONE',  ( 3.147653791585693028, 8.920000000000001705, 2.419999999999999485 ) ) ;
#101230=EDGE_LOOP ( 'NONE', ( #170417, #11352, #206497, #53942 ) ) ;
#101234=ORIENTED_EDGE ( 'NONE', *, *, #34519, .T. ) ;
#101235=CARTESIAN_POINT ( 'NONE',  ( -4.716257332707368910, 6.595662536282280719, -1.599625672291271394 ) ) ;
#101236=CARTESIAN_POINT ( 'NONE',  ( -5.171509248969888617, 4.998125310078441075, 0.7998128361456281477 ) ) ;
#101239=CARTESIAN_POINT ( 'NONE',  ( 5.356880090730863131, 7.343055753976412525, 1.443375672974064550 ) ) ;
#101251=CARTESIAN_POINT ( 'NONE',  ( -5.773214272755326171, 7.262619621122762048, 1.194638459467006530 ) ) ;
#101256=CARTESIAN_POINT ( 'NONE',  ( 4.475600106286968582, 5.354526557823810151, -1.082531754730548412 ) ) ;
#101259=CARTESIAN_POINT ( 'NONE',  ( -5.387385936583832802, 7.378645907471495846, -1.599625672291271394 ) ) ;
#101270=CARTESIAN_POINT ( 'NONE',  ( 3.553118775233146120, 6.302999783484076524, -1.199719254218453823 ) ) ;
#101278=B_SPLINE_CURVE_WITH_KNOTS ( 'NONE', 3,
 ( #164847, #16439, #51098, #198392 ),
 .UNSPECIFIED., .F., .F.,
 ( 4, 4 ),
 ( 2.941991273438700769E-15, 0.0007499567245562745437 ),
 .UNSPECIFIED. ) ;
#101283=FACE_OUTER_BOUND ( 'NONE', #27133, .T. ) ;
#101310=CARTESIAN_POINT ( 'NONE',  ( 5.777182853198898904, 6.873039762554409293, -1.082531754730548412 ) ) ;
#101316=CARTESIAN_POINT ( 'NONE',  ( 5.926322542504858681, 8.007405281046052536, -1.443375672974078761 ) ) ;
#101330=CARTESIAN_POINT ( 'NONE',  ( -7.065734331377342414, 8.272386803808890576, -1.199719254218452047 ) ) ;
#101342=CARTESIAN_POINT ( 'NONE',  ( 5.085717018457579286, 6.066329622022862189, -1.082531754730548412 ) ) ;
#101349=CARTESIAN_POINT ( 'NONE',  ( -7.937372586157736443, 8.224965870130965584, 0.7998128361456341429 ) ) ;
#101355=CARTESIAN_POINT ( 'NONE',  ( -5.261973015879593873, 8.192700047617899273, 1.082531754730549967 ) ) ;
#101358=CARTESIAN_POINT ( 'NONE',  ( -6.774234028683526532, 7.932303117332766718, 1.199719254218452047 ) ) ;
#101380=CARTESIAN_POINT ( 'NONE',  ( -3.851925040058345573, 5.587274861525073355, -1.443375672974078761 ) ) ;
#101382=CARTESIAN_POINT ( 'NONE',  ( -4.462041952228944730, 7.259447140025469203, -1.082531754730549967 ) ) ;
#101384=CARTESIAN_POINT ( 'NONE',  ( 4.817943484809818600, 6.714296380401858499, 1.599625672291269396 ) ) ;
#101385=CARTESIAN_POINT ( 'NONE',  ( -3.793249116773374396, 7.647484079536056356, 0.7998128361456352531 ) ) ;
#101386=CARTESIAN_POINT ( 'NONE',  ( -4.620296487206990932, 8.612372678375294299, 0.000000000000000000 ) ) ;
#101390=CONICAL_SURFACE ( 'NONE', #70283, 3.999999999999998224, 0.8621700546672330656 ) ;
#101393=VERTEX_POINT ( 'NONE', #94522 ) ;
#101399=ORIENTED_EDGE ( 'NONE', *, *, #61843, .F. ) ;
#101432=CARTESIAN_POINT ( 'NONE',  ( 2.995319178684289430, 6.412246817072642102, -0.4997136395867556868 ) ) ;
#101440=CARTESIAN_POINT ( 'NONE',  ( 3.061108821635398769, 6.793320401875094561, -0.7998128361456362523 ) ) ;
#101454=CARTESIAN_POINT ( 'NONE',  ( 4.594558193676899549, 8.374302254291812631, 0.02480325318809234458 ) ) ;
#101457=CARTESIAN_POINT ( 'NONE',  ( 6.861835142292135536, 9.098836647464588978, 1.443375672974065660 ) ) ;
#101464=CARTESIAN_POINT ( 'NONE',  ( -5.478376588373717659, 8.549133898814758936, -1.199719254218452047 ) ) ;
#101471=CARTESIAN_POINT ( 'NONE',  ( -6.199677282185614757, 6.647997080169443684, 0.6295152255529173901 ) ) ;
#101474=EDGE_CURVE ( 'NONE', #130628, #31895, #13499, .T. ) ;
#101477=CARTESIAN_POINT ( 'NONE',  ( 6.387299765813869712, 6.624473612970537495, 0.000000000000000000 ) ) ;
#101481=CARTESIAN_POINT ( 'NONE',  ( -5.483346782084204563, 5.361935765378481378, 0.000000000000000000 ) ) ;
#101493=CARTESIAN_POINT ( 'NONE',  ( 3.555981428534177091, 7.370671776590375757, 0.7998128361456271485 ) ) ;
#101494=CARTESIAN_POINT ( 'NONE',  ( 3.562760505341037831, 7.378580699531681830, -1.734723475976807094E-15 ) ) ;
#101514=DIRECTION ( 'NONE',  ( 0.7927788072560210120, 0.000000000000000000, 0.6095094443613819912 ) ) ;
#101528=CARTESIAN_POINT ( 'NONE',  ( 4.830447868218803897, 8.857549289555754157, -0.7998128361456481317 ) ) ;
#101533=CARTESIAN_POINT ( 'NONE',  ( 5.885648082108200896, 6.039213315313952002, 0.7216878364870328300 ) ) ;
#101537=CARTESIAN_POINT ( 'NONE',  ( 7.512626515748109135, 8.897724035528543851, 1.082531754730549967 ) ) ;
#101547=B_SPLINE_CURVE_WITH_KNOTS ( 'NONE', 3,
 ( #173162, #208815, #24743, #123424 ),
 .UNSPECIFIED., .F., .F.,
 ( 4, 4 ),
 ( 0.000000000000000000, 0.0005936488266206346861 ),
 .UNSPECIFIED. ) ;
#101549=CARTESIAN_POINT ( 'NONE',  ( 6.396603524444617328, 6.809554808131969672, -0.5206029305389828776 ) ) ;
#101550=CARTESIAN_POINT ( 'NONE',  ( -5.966997003790221576, 9.015228033513643879, -1.082531754730549967 ) ) ;
#101583=CARTESIAN_POINT ( 'NONE',  ( 5.668190738965027897, 8.770583741171307679, -1.199719254218452047 ) ) ;
#101585=CARTESIAN_POINT ( 'NONE',  ( 7.147083253059300922, 8.367293879104554577, 1.199719254218452935 ) ) ;
#101598=CARTESIAN_POINT ( 'NONE',  ( -5.795184315198522285, 5.725746220678519904, -0.7998128361456362523 ) ) ;
#101600=CARTESIAN_POINT ( 'NONE',  ( 5.004368096775565711, 8.852530189631227842, -0.7216878364870458196 ) ) ;
#101617=CARTESIAN_POINT ( 'NONE',  ( -7.932929277771797238, 8.427708043588125975, 0.000000000000000000 ) ) ;
#101619=CARTESIAN_POINT ( 'NONE',  ( -6.631346530859867805, 6.909194838857525944, 0.000000000000000000 ) ) ;
#101627=EDGE_CURVE ( 'NONE', #199688, #44672, #21127, .T. ) ;
#101644=CARTESIAN_POINT ( 'NONE',  ( -4.847922445338252118, 7.813604065273374921, -1.199719254218453823 ) ) ;
#101654=CARTESIAN_POINT ( 'NONE',  ( 2.300251978943730791, 2.674522988693084358, -2.456405383529883135 ) ) ;
#101655=CARTESIAN_POINT ( 'NONE',  ( -5.526470424545159688, 7.552361116859303891, -1.349762019914104272 ) ) ;
#101671=CARTESIAN_POINT ( 'NONE',  ( 6.550524494058025837, 7.671308660269694712, -1.199719254218452047 ) ) ;
#101694=CARTESIAN_POINT ( 'NONE',  ( 6.692885107001518286, 7.837396042037102717, -1.199719254218452047 ) ) ;
#101695=CARTESIAN_POINT ( 'NONE',  ( 4.199993725183334803, 8.122019456014369254, -0.7998128361456362523 ) ) ;
#101697=CARTESIAN_POINT ( 'NONE',  ( 6.364626766972446781, 6.390095747748157251, 0.7998128361456352531 ) ) ;
#101709=CARTESIAN_POINT ( 'NONE',  ( 4.745935331938881951, 8.308991367555595531, -0.7587592799198628057 ) ) ;
#101710=CARTESIAN_POINT ( 'NONE',  ( -7.078765599666485997, 7.431183752465250869, 0.000000000000000000 ) ) ;
#101711=CARTESIAN_POINT ( 'NONE',  ( 3.445180431648313224, 7.033477913649446300, 0.7216878364870257245 ) ) ;
#101733=CARTESIAN_POINT ( 'NONE',  ( -3.485854892044994102, 7.080931450778859215, -0.7216878364870458196 ) ) ;
#101739=CARTESIAN_POINT ( 'NONE',  ( 5.505492895601038938, 8.580769590579979678, -1.199719254218452047 ) ) ;
#101756=CARTESIAN_POINT ( 'NONE',  ( 0.000000000000000000, 0.08000000000000020983, -2.000000000000000000 ) ) ;
#101767=CARTESIAN_POINT ( 'NONE',  ( 5.806634928402749196, 9.996434193103704402, -0.7998128361456481317 ) ) ;
#101771=CARTESIAN_POINT ( 'NONE',  ( -5.171754443046126859, 7.767122556988016235, 1.178735681042131667 ) ) ;
#101772=CARTESIAN_POINT ( 'NONE',  ( 6.984385409695311964, 8.177479728513226576, 1.199719254218452935 ) ) ;
#101799=CARTESIAN_POINT ( 'NONE',  ( 3.553645660557675612, 6.199651466408984568, -1.082531754730549967 ) ) ;
#101803=CARTESIAN_POINT ( 'NONE',  ( -5.108390017298964914, 9.181815130149269422, 0.000000000000000000 ) ) ;
#101805=CARTESIAN_POINT ( 'NONE',  ( 6.444921918449731280, 8.612437886315108315, 1.599625672291268286 ) ) ;
#101821=CARTESIAN_POINT ( 'NONE',  ( -5.438229012412903352, 6.477593614970734492, -1.082531754730549967 ) ) ;
#101828=CARTESIAN_POINT ( 'NONE',  ( 6.318982112420993502, 9.529840343536603697, -1.199719254218452047 ) ) ;
#101839=CARTESIAN_POINT ( 'NONE',  ( 5.872089928494542477, 9.864872326636710653, 0.000000000000000000 ) ) ;
#101852=CARTESIAN_POINT ( 'NONE',  ( -5.641601317062248988, 6.714861303728305586, -1.082531754730549967 ) ) ;
#101855=CARTESIAN_POINT ( 'NONE',  ( 6.398522151006641678, 6.429640362454684954, 0.000000000000000000 ) ) ;
#101858=CARTESIAN_POINT ( 'NONE',  ( -5.921879234118920365, 10.13088588310589699, 0.000000000000000000 ) ) ;
#101860=CARTESIAN_POINT ( 'NONE',  ( -3.709037541790315640, 6.484905011134099340, -1.199719254218450271 ) ) ;
#101862=CARTESIAN_POINT ( 'NONE',  ( 3.927105836647628134, 7.326788671016230658, -0.8738547742103716098 ) ) ;
#101907=CARTESIAN_POINT ( 'NONE',  ( 4.472210567661338843, 6.310941310395290493, 1.599625672291261402 ) ) ;
#101910=CARTESIAN_POINT ( 'NONE',  ( -3.800028193580205382, 7.655393002477360653, -0.7998128361456481317 ) ) ;
#101911=CARTESIAN_POINT ( 'NONE',  ( -4.899292406491859708, 6.809203455697520724, -1.599625672291271394 ) ) ;
#101914=CARTESIAN_POINT ( 'NONE',  ( -5.926322542504872892, 8.007405281046052536, -1.443375672974066548 ) ) ;
#101916=CARTESIAN_POINT ( 'NONE',  ( 2.969881706132979637, 6.595290641185153291, 0.3483476683807932295 ) ) ;
#101920=CARTESIAN_POINT ( 'NONE',  ( -5.586841817283045408, 8.675676665875643678, 1.199719254218454489 ) ) ;
#101926=CARTESIAN_POINT ( 'NONE',  ( -5.000000000000013323, 11.39843543023555661, 0.7750000000000004663 ) ) ;
#101928=CARTESIAN_POINT ( 'NONE',  ( -6.642568916052639771, 6.714361588341672515, 0.000000000000000000 ) ) ;
#101930=CARTESIAN_POINT ( 'NONE',  ( 4.616554244727909762, 8.463227371007752353, -0.2998622348379786362 ) ) ;
#101936=CARTESIAN_POINT ( 'NONE',  ( 7.354371980770088690, 7.544798497178720531, 0.000000000000000000 ) ) ;
#101942=CARTESIAN_POINT ( 'NONE',  ( -6.252245114557387851, 7.323316050852266557, -1.199719254218453823 ) ) ;
#101947=CARTESIAN_POINT ( 'NONE',  ( -7.422162748838431412, 7.623887726591770608, -0.7998128361456362523 ) ) ;
#101949=CARTESIAN_POINT ( 'NONE',  ( 4.516274566683618374, 8.283087737857229627, -0.7216878364870552565 ) ) ;
#101952=CARTESIAN_POINT ( 'NONE',  ( -6.577113915960828727, 9.727031097712693253, -1.082531754730549967 ) ) ;
#101959=CARTESIAN_POINT ( 'NONE',  ( 6.801350335910821165, 7.963938809097990124, 1.199719254218452047 ) ) ;
#101969=LINE ( 'NONE', #52155, #111972 ) ;
#101973=CARTESIAN_POINT ( 'NONE',  ( 6.480989489388473856, 6.848452138476523565, -0.6157061703677743081 ) ) ;
#101986=VERTEX_POINT ( 'NONE', #178915 ) ;
#102002=CARTESIAN_POINT ( 'NONE',  ( -6.429665931644899857, 6.880618766637560668, 0.7446329532827021813 ) ) ;
#102022=CARTESIAN_POINT ( 'NONE',  ( -5.764151584465413869, 6.753873599078290546, -1.199719254218453823 ) ) ;
#102038=CARTESIAN_POINT ( 'NONE',  ( 6.313256805818848960, 7.394496357324014113, 1.199719254218452047 ) ) ;
#102041=CARTESIAN_POINT ( 'NONE',  ( 4.868786560638878491, 8.694351730805124134, 0.7216878364870317197 ) ) ;
#102053=B_SPLINE_CURVE_WITH_KNOTS ( 'NONE', 3,
 ( #154059, #71706, #121637, #187606, #105325, #173531 ),
 .UNSPECIFIED., .F., .F.,
 ( 4, 2, 4 ),
 ( 0.000000000000000000, 0.0002821277059972537317, 0.0005642554119945074635 ),
 .UNSPECIFIED. ) ;
#102056=CARTESIAN_POINT ( 'NONE',  ( -5.424143973919053785, 8.485862515284315677, 1.199719254218454489 ) ) ;
#102058=CARTESIAN_POINT ( 'NONE',  ( 5.879395890181562834, 6.888325289080478697, -1.199719254218452047 ) ) ;
#102066=CARTESIAN_POINT ( 'NONE',  ( -3.923105346307911745, 5.670318552149568703, -1.599625672291283607 ) ) ;
#102067=CARTESIAN_POINT ( 'NONE',  ( 7.856023664475727308, 8.130058794835305136, -0.7998128361456341429 ) ) ;
#102073=CARTESIAN_POINT ( 'NONE',  ( 6.333594036239346359, 7.418223126147930557, 1.199719254218453823 ) ) ;
#102078=CARTESIAN_POINT ( 'NONE',  ( -5.337921042252067316, 7.714266718146587820, 1.325459453385816833 ) ) ;
#102088=CARTESIAN_POINT ( 'NONE',  ( -4.055297343818976330, 5.824542549245813383, 1.443375672974065660 ) ) ;
#102097=CARTESIAN_POINT ( 'NONE',  ( 5.424670859243587273, 5.501406555305196733, -0.7216878364870458196 ) ) ;
#102100=CARTESIAN_POINT ( 'NONE',  ( -6.622231685632140596, 6.690634819517756959, 0.000000000000000000 ) ) ;
#102118=CARTESIAN_POINT ( 'NONE',  ( 4.899292406491845497, 6.809203455697520724, -1.599625672291273393 ) ) ;
#102138=CARTESIAN_POINT ( 'NONE',  ( -0.3565558069077310321, 3.212289187162292503, 1.969079779732920032 ) ) ;
#102141=CARTESIAN_POINT ( 'NONE',  ( 5.065906673361608270, 5.939254536123854677, -1.199719254218450271 ) ) ;
#102142=CARTESIAN_POINT ( 'NONE',  ( -5.966997003790240228, 6.134120390609613338, -0.7216878364870338292 ) ) ;
#102167=CARTESIAN_POINT ( 'NONE',  ( -5.108390017298964914, 9.181815130149269422, 0.000000000000000000 ) ) ;
#102181=CARTESIAN_POINT ( 'NONE',  ( -7.449279056065764237, 7.655523418356991350, 0.7998128361456341429 ) ) ;
#102188=CARTESIAN_POINT ( 'NONE',  ( 6.590425141155737521, 6.776330403399432711, -0.3092786388759184990 ) ) ;
#102193=CARTESIAN_POINT ( 'NONE',  ( -5.261446130555064826, 8.296048364692991228, 1.199719254218452935 ) ) ;
#102197=CARTESIAN_POINT ( 'NONE',  ( -7.431277594066152403, 8.802816960232885179, -1.082531754730549967 ) ) ;
#102200=CARTESIAN_POINT ( 'NONE',  ( -8.068510813464099485, 8.585886501895810596, 0.7216878364870317197 ) ) ;
#102201=CARTESIAN_POINT ( 'NONE',  ( 4.787437638956922648, 6.678706226906775179, -1.443375672974068769 ) ) ;
#102203=CARTESIAN_POINT ( 'NONE',  ( -5.139949632912262700, 5.169231791251960750, 0.7216878364870257245 ) ) ;
#102221=CARTESIAN_POINT ( 'NONE',  ( 6.576141308597898139, 6.785670920958930985, -0.3094590540993913952 ) ) ;
#102227=ORIENTED_EDGE ( 'NONE', *, *, #14726, .T. ) ;
#102238=CARTESIAN_POINT ( 'NONE',  ( 6.474762296362193581, 6.758873339713582062, -0.2294044474360455721 ) ) ;
#102255=CARTESIAN_POINT ( 'NONE',  ( -4.956387674247580755, 7.940146832334256111, 1.199719254218452935 ) ) ;
#102266=CARTESIAN_POINT ( 'NONE',  ( 5.631432701629774051, 7.663367133358481631, 1.599625672291269396 ) ) ;
#102272=CARTESIAN_POINT ( 'NONE',  ( -5.546694241322218666, 8.524874810634301525, 1.082531754730550855 ) ) ;
#102277=CARTESIAN_POINT ( 'NONE',  ( 7.550965208168244125, 7.774157262476569130, -0.7998128361456341429 ) ) ;
#102283=CARTESIAN_POINT ( 'NONE',  ( 1.850900803405173489, 8.952907405788534945, 0.7750000000000004663 ) ) ;
#102294=CARTESIAN_POINT ( 'NONE',  ( -5.289089323106922258, 9.184704953684462936, 0.7216878364870267237 ) ) ;
#102295=CARTESIAN_POINT ( 'NONE',  ( 6.563555762791525972, 6.830105609444471426, -0.7216878364870458196 ) ) ;
#102300=ORIENTED_EDGE ( 'NONE', *, *, #82643, .F. ) ;
#102301=PLANE ( 'NONE',  #28545 ) ;
#102305=CARTESIAN_POINT ( 'NONE',  ( -3.786470039966538970, 7.639575156594750283, 0.000000000000000000 ) ) ;
#102306=CARTESIAN_POINT ( 'NONE',  ( -3.311934663488232733, 7.085950550703385531, -0.7998128361456481317 ) ) ;
#102308=CARTESIAN_POINT ( 'NONE',  ( 5.167065940139554669, 9.042344340222555843, -0.7216878364870458196 ) ) ;
#102321=CARTESIAN_POINT ( 'NONE',  ( -4.807049873888117553, 8.139959938814184781, 0.8294007104595437774 ) ) ;
#102326=CARTESIAN_POINT ( 'NONE',  ( 3.933273961740298752, 5.682181936820735579, 1.443375672974058777 ) ) ;
#102329=CARTESIAN_POINT ( 'NONE',  ( -4.444040490229335560, 8.406740681901359480, 0.7998128361456352531 ) ) ;
#102343=CARTESIAN_POINT ( 'NONE',  ( 5.578253857379852576, 5.472660686556754861, -0.7998128361456481317 ) ) ;
#102369=ORIENTED_EDGE ( 'NONE', *, *, #21723, .T. ) ;
#102380=CARTESIAN_POINT ( 'NONE',  ( 5.153507786970260796, 7.105788066255672497, -1.443375672974078761 ) ) ;
#102382=ORIENTED_EDGE ( 'NONE', *, *, #25508, .F. ) ;
#102387=CARTESIAN_POINT ( 'NONE',  ( 5.844973620822835336, 7.912498205750389424, 1.443375672974064550 ) ) ;
#102400=CARTESIAN_POINT ( 'NONE',  ( -6.903036488013351679, 8.082572653217566128, -1.199719254218452047 ) ) ;
#102412=CARTESIAN_POINT ( 'NONE',  ( 4.326460416092276162, 7.101268681199365496, -1.082531754730548412 ) ) ;
#102418=CARTESIAN_POINT ( 'NONE',  ( -6.587282531393266360, 8.778525268082516320, 1.599625672291269396 ) ) ;
#102423=CARTESIAN_POINT ( 'NONE',  ( -5.126391479742927970, 8.994890803093138487, 0.7216878364870267237 ) ) ;
#102426=CARTESIAN_POINT ( 'NONE',  ( -7.761116589180078407, 8.019333873657032541, 0.000000000000000000 ) ) ;
#102448=CARTESIAN_POINT ( 'NONE',  ( -3.689227196694346400, 6.357829925235092716, -1.082531754730546636 ) ) ;
#102450=CARTESIAN_POINT ( 'NONE',  ( -3.797692425159308716, 7.444741906078900406, 0.000000000000000000 ) ) ;
#102451=EDGE_CURVE ( 'NONE', #201520, #173093, #200359, .T. ) ;
#102453=CARTESIAN_POINT ( 'NONE',  ( 5.411639590510088027, 6.342609606130419131, -1.199719254218452047 ) ) ;
#102454=CARTESIAN_POINT ( 'NONE',  ( -4.630991987519598396, 7.560518531151607213, 1.199719254218452935 ) ) ;
#102455=CARTESIAN_POINT ( 'NONE',  ( -7.781453819600577582, 8.043060642480948985, 0.000000000000000000 ) ) ;
#102511=CARTESIAN_POINT ( 'NONE',  ( 4.224247379109608680, 7.085983154673295203, -1.199719254218452047 ) ) ;
#102524=CARTESIAN_POINT ( 'NONE',  ( 4.611577566919329740, 8.352668595566711929, -0.2595669225248058432 ) ) ;
#102527=CARTESIAN_POINT ( 'NONE',  ( 3.366167277942881064, 7.149221934233827014, -0.7998128361456362523 ) ) ;
#102534=CARTESIAN_POINT ( 'NONE',  ( -7.598418745816086783, 7.829519723065708092, 0.000000000000000000 ) ) ;
#102539=CARTESIAN_POINT ( 'NONE',  ( 3.147653791585717453, 8.920000000000001705, -2.420000000000002149 ) ) ;
#102545=CARTESIAN_POINT ( 'NONE',  ( 5.234856708652222856, 8.161064355852680308, 1.082531754730549078 ) ) ;
#102547=EDGE_CURVE ( 'NONE', #141689, #105686, #33813, .T. ) ;
#102549=CARTESIAN_POINT ( 'NONE',  ( -4.990283058281743678, 7.979691447040783814, -1.199719254218453823 ) ) ;
#102554=( BOUNDED_SURFACE ( )  B_SPLINE_SURFACE ( 3, 2, ( 
 ( #30685, #100985, #149759 ),
 ( #181179, #260, #66330 ),
 ( #198478, #50123, #67397 ),
 ( #133538, #199545, #14396 ),
 ( #51187, #117310, #96768 ),
 ( #211534, #63169, #129335 ) ),
 .UNSPECIFIED., .F., .F., .T. ) 
 B_SPLINE_SURFACE_WITH_KNOTS ( ( 4, 2, 4 ),
 ( 3, 3 ),
 ( 6.938893903907228378E-18, 0.002403677751102689057, 0.004807355502205371174 ),
 ( 0.000000000000000000, 1.000000000000000000 ),
 .UNSPECIFIED. ) 
 GEOMETRIC_REPRESENTATION_ITEM ( )  RATIONAL_B_SPLINE_SURFACE ( (
 ( 1.000000000000000000, 0.7789607113619948509, 1.000000000000000000),
 ( 1.000000000000000000, 0.7844575505954939354, 1.000000000000000000),
 ( 1.000000000000000000, 0.7910273759756237810, 1.000000000000000000),
 ( 1.000000000000000000, 0.8087931444444614870, 1.000000000000000000),
 ( 1.000000000000000000, 0.8199986536752678079, 1.000000000000000000),
 ( 1.000000000000000000, 0.8356624583022104202, 1.000000000000000000) ) ) 
 REPRESENTATION_ITEM ( '' )  SURFACE ( )  );
#102558=EDGE_LOOP ( 'NONE', ( #180161, #173900, #161311, #89807, #199007, #20825, #98871, #140040, #176590 ) ) ;
#102563=CARTESIAN_POINT ( 'NONE',  ( 3.366167277942881064, 7.149221934233827014, -0.7998128361456362523 ) ) ;
#102564=CARTESIAN_POINT ( 'NONE',  ( 5.254667053748194760, 8.288139441751686931, 1.199719254218452047 ) ) ;
#102586=CARTESIAN_POINT ( 'NONE',  ( 6.127784903196001665, 7.091900248975262500, -1.102264294108054266 ) ) ;
#102594=CIRCLE ( 'NONE', #99200, 4.022469383779238683 ) ;
#102598=CARTESIAN_POINT ( 'NONE',  ( 3.953084306836263995, 6.769626237021087789, 1.199719254218452047 ) ) ;
#102604=CARTESIAN_POINT ( 'NONE',  ( 6.964048179274811012, 8.153752959689313684, 1.199719254218452047 ) ) ;
#102609=CARTESIAN_POINT ( 'NONE',  ( 4.746763178560254204, 6.631252689777363152, 1.443375672974065660 ) ) ;
#102612=CARTESIAN_POINT ( 'NONE',  ( 4.523580528814945545, 5.306540700819438960, 1.199719254218452047 ) ) ;
#102624=CARTESIAN_POINT ( 'NONE',  ( 6.486339200172205999, 6.751434215916642501, 0.1376000389162572446 ) ) ;
#102625=CARTESIAN_POINT ( 'NONE',  ( -7.024532985656169792, 9.288650798055913427, 1.443375672974064550 ) ) ;
#102658=CARTESIAN_POINT ( 'NONE',  ( 7.530627977747744062, 7.750430493652658015, -0.7998128361456341429 ) ) ;
#102660=CARTESIAN_POINT ( 'NONE',  ( 5.851225812749518695, 8.984124660586543243, -1.199719254218452047 ) ) ;
#102674=CARTESIAN_POINT ( 'NONE',  ( -4.878955176071358757, 6.785476686873604280, -1.599625672291271394 ) ) ;
#102676=CARTESIAN_POINT ( 'NONE',  ( 6.834718834620487016, 7.146462526578263308, 0.000000000000000000 ) ) ;
#102685=CARTESIAN_POINT ( 'NONE',  ( -4.228163802615396705, 6.026220084508304708, -1.599625672291271394 ) ) ;
#102692=CARTESIAN_POINT ( 'NONE',  ( -6.780486220610184134, 9.003929572168926754, -1.443375672974066548 ) ) ;
#102694=CARTESIAN_POINT ( 'NONE',  ( -5.478903473698247595, 8.445785581739666981, -1.082531754730549967 ) ) ;
#102717=CARTESIAN_POINT ( 'NONE',  ( -4.308458954092677651, 8.248562223075252220, -0.7998128361456362523 ) ) ;
#102727=CARTESIAN_POINT ( 'NONE',  ( 1.793740946118090429, 2.512284051036407728, -2.500000000000000444 ) ) ;
#102728=CARTESIAN_POINT ( 'NONE',  ( -5.018240346111991990, 8.014652766117364990, -1.155606277404798821 ) ) ;
#102730=AXIS2_PLACEMENT_3D ( 'NONE', #119251, #36858, #102942 ) ;
#102744=CARTESIAN_POINT ( 'NONE',  ( 3.614985261928882032, 3.508924507032078477, 2.500000000000000444 ) ) ;
#102763=CARTESIAN_POINT ( 'NONE',  ( 3.888156192069020634, 7.758209000714329839, 1.040834085586084257E-14 ) ) ;
#102770=CARTESIAN_POINT ( 'NONE',  ( 5.037736595929563244, 8.035053907629919223, -1.199719254218452047 ) ) ;
#102772=CARTESIAN_POINT ( 'NONE',  ( 6.201928923608456046, 6.200281597156833691, 0.7998128361456352531 ) ) ;
#102780=CARTESIAN_POINT ( 'NONE',  ( 4.370663978927085580, 5.060324124126027279, 7.500000000000000000 ) ) ;
#102784=CARTESIAN_POINT ( 'NONE',  ( 4.913571454530422322, 8.125067815752732514, -1.031885869761673069 ) ) ;
#102786=CARTESIAN_POINT ( 'NONE',  ( -5.926322542504877333, 7.047036066744706950, -1.082531754730549967 ) ) ;
#102787=CARTESIAN_POINT ( 'NONE',  ( 5.573810548993915148, 5.675402860013913475, 0.000000000000000000 ) ) ;
#102798=ORIENTED_EDGE ( 'NONE', *, *, #61052, .F. ) ;
#102806=CARTESIAN_POINT ( 'NONE',  ( -4.597623488365601752, 8.377994813152914944, 0.7216878364870267237 ) ) ;
#102811=CARTESIAN_POINT ( 'NONE',  ( 5.397027666691686321, 8.454226823519094935, 1.199719254218451159 ) ) ;
#102831=CARTESIAN_POINT ( 'NONE',  ( -5.884327782891165093, 6.523468454024004437, -0.8610041489593980302 ) ) ;
#102840=CARTESIAN_POINT ( 'NONE',  ( 6.668631453075247073, 8.873432343378178544, -1.599625672291281386 ) ) ;
#102847=ORIENTED_EDGE ( 'NONE', *, *, #30754, .F. ) ;
#102854=CARTESIAN_POINT ( 'NONE',  ( 1.822139829856954441, 2.508700120398218214, 2.498486944294420642 ) ) ;
#102869=CARTESIAN_POINT ( 'NONE',  ( 4.258669648468281110, 6.061810238003387141, 1.443375672974058777 ) ) ;
#102875=CARTESIAN_POINT ( 'NONE',  ( -6.583366107887490770, 9.838288338247510367, 1.199719254218452935 ) ) ;
#102877=CARTESIAN_POINT ( 'NONE',  ( 6.363572996767764778, 8.517530811019446091, -1.599625672291283607 ) ) ;
#102881=CARTESIAN_POINT ( 'NONE',  ( -2.862179826260718762, 6.353310540697199471, 0.000000000000000000 ) ) ;
#102897=CARTESIAN_POINT ( 'NONE',  ( 7.180978637093494044, 8.406838493811077839, -1.199719254218452047 ) ) ;
#102903=ORIENTED_EDGE ( 'NONE', *, *, #71839, .F. ) ;
#102906=CARTESIAN_POINT ( 'NONE',  ( 6.536439455564150514, 9.679577560583279450, 1.082531754730549078 ) ) ;
#102918=CARTESIAN_POINT ( 'NONE',  ( 0.000000000000000000, 8.499999999999996447, 0.000000000000000000 ) ) ;
#102920=CARTESIAN_POINT ( 'NONE',  ( -6.319508997745553636, 6.545384383557486530, 0.7216878364870257245 ) ) ;
#102922=CARTESIAN_POINT ( 'NONE',  ( 6.339319342841494453, 9.553567112360518365, -1.199719254218452047 ) ) ;
#102925=CARTESIAN_POINT ( 'NONE',  ( -7.930593509350902792, 8.217056947189661287, -0.7998128361456362523 ) ) ;
#102927=CARTESIAN_POINT ( 'NONE',  ( -3.546339698426324460, 6.295090860542775779, -1.199719254218450271 ) ) ;
#102929=CARTESIAN_POINT ( 'NONE',  ( 3.913815762669449416, 7.330443837381343641, -0.8582294057540799104 ) ) ;
#102942=DIRECTION ( 'NONE',  ( 0.7592566023653005702, -0.6507913734559639396, 0.000000000000000000 ) ) ;
#102974=CARTESIAN_POINT ( 'NONE',  ( -5.281783360975562225, 8.319775133516907673, 1.199719254218452935 ) ) ;
#102978=CARTESIAN_POINT ( 'NONE',  ( -4.274563570058511175, 8.209017608368725405, 0.000000000000000000 ) ) ;
#102979=CARTESIAN_POINT ( 'NONE',  ( -4.685224601974262271, 7.623789914682047808, -1.199719254218453823 ) ) ;
#102981=ORIENTED_EDGE ( 'NONE', *, *, #7522, .F. ) ;
#102982=CARTESIAN_POINT ( 'NONE',  ( -5.356880090730904875, 7.343055753976412525, 1.443375672974058777 ) ) ;
#102988=CARTESIAN_POINT ( 'NONE',  ( -5.966470118465691641, 9.118576350588734059, -1.199719254218452047 ) ) ;
#102995=CARTESIAN_POINT ( 'NONE',  ( 3.577053382146960558, 7.342256794902024986, 0.3077596360769136452 ) ) ;
#102998=CARTESIAN_POINT ( 'NONE',  ( -5.284646014276622950, 9.387447126623207794, -0.7998128361456362523 ) ) ;
#103000=CARTESIAN_POINT ( 'NONE',  ( 4.624709440338444111, 8.453137518702421360, 0.3515692964491355932 ) ) ;
#103003=CARTESIAN_POINT ( 'NONE',  ( 1.843739406749204335, 9.999999999999998224, 0.7750000000000004663 ) ) ;
#103005=CARTESIAN_POINT ( 'NONE',  ( 7.343676480457483002, 8.596652644402405841, -1.199719254218452047 ) ) ;
#103017=CARTESIAN_POINT ( 'NONE',  ( -5.725286006720766707, 9.901527117808042178, 0.7998128361456291469 ) ) ;
#103029=CARTESIAN_POINT ( 'NONE',  ( 5.885121196783658526, 9.023669275293071834, 1.199719254218452047 ) ) ;
#103044=CARTESIAN_POINT ( 'NONE',  ( 5.544801429207002030, 7.539493339695484408, -1.337888636821100041 ) ) ;
#103067=CARTESIAN_POINT ( 'NONE',  ( -4.525370967935856470, 8.233940877497639477, -0.3192380598915856571 ) ) ;
#103074=CARTESIAN_POINT ( 'NONE',  ( -6.486107617800834113, 6.842887492708185526, 0.6303255377333163434 ) ) ;
#103090=CARTESIAN_POINT ( 'NONE',  ( -4.305596300791617814, 7.180890229968955651, 1.199719254218452935 ) ) ;
#103107=CARTESIAN_POINT ( 'NONE',  ( -5.385662150563701900, 6.164098921825184263, 1.139024650766025548 ) ) ;
#103123=CARTESIAN_POINT ( 'NONE',  ( -5.315678745009726924, 8.359319748223434487, -1.199719254218453823 ) ) ;
#103125=CARTESIAN_POINT ( 'NONE',  ( 5.611095471209277541, 7.639640364534566075, 1.599625672291268286 ) ) ;
#103129=EDGE_CURVE ( 'NONE', #107579, #85668, #168089, .T. ) ;
#103135=CARTESIAN_POINT ( 'NONE',  ( -5.738844160334429567, 9.917344963690652548, 0.000000000000000000 ) ) ;
#103136=CARTESIAN_POINT ( 'NONE',  ( 7.506374323821472849, 8.786466794993730289, -1.199719254218452047 ) ) ;
#103142=CARTESIAN_POINT ( 'NONE',  ( 5.515134625708930649, 9.656350506627580543, 0.000000000000000000 ) ) ;
#103147=CARTESIAN_POINT ( 'NONE',  ( -5.025714415505916577, 8.007183762769660262, 1.161964715574652196 ) ) ;
#103153=AXIS2_PLACEMENT_3D ( 'NONE', #60193, #105791, #124229 ) ;
#103157=CARTESIAN_POINT ( 'NONE',  ( -4.285785955251283141, 8.014184357852876417, 0.000000000000000000 ) ) ;
#103160=CARTESIAN_POINT ( 'NONE',  ( -3.578681416171278329, 3.551814636441860351, 2.500000000000000444 ) ) ;
#103166=CARTESIAN_POINT ( 'NONE',  ( 5.573810548993915148, 5.675402860013913475, 0.000000000000000000 ) ) ;
#103170=CARTESIAN_POINT ( 'NONE',  ( -4.450819567036169211, 8.414649604842665553, -0.7998128361456362523 ) ) ;
#103174=EDGE_CURVE ( 'NONE', #8487, #25034, #181133, .T. ) ;
#103189=CARTESIAN_POINT ( 'NONE',  ( 4.712340909201580885, 7.655425606447271214, -1.199719254218452047 ) ) ;
#103195=AXIS2_PLACEMENT_3D ( 'NONE', #70349, #118133, #37882 ) ;
#103200=ORIENTED_EDGE ( 'NONE', *, *, #144483, .F. ) ;
#103209=CARTESIAN_POINT ( 'NONE',  ( 0.001013208909606179041, 3.413442832661036430, 2.083547725167233633 ) ) ;
#103211=CARTESIAN_POINT ( 'NONE',  ( 5.204350862799327793, 7.165104988056252289, -1.599625672291281386 ) ) ;
#103214=CARTESIAN_POINT ( 'NONE',  ( -5.072158865288277418, 7.010880990960010273, 1.443375672974058777 ) ) ;
#103238=CARTESIAN_POINT ( 'NONE',  ( -7.456058132872594335, 7.663432341298296535, 0.000000000000000000 ) ) ;
#103240=CARTESIAN_POINT ( 'NONE',  ( 7.648208051440442468, 8.095533279534887328, 0.000000000000000000 ) ) ;
#103245=CARTESIAN_POINT ( 'NONE',  ( -4.442231607132987925, 5.211633625523774960, -1.199719254218453823 ) ) ;
#103252=CARTESIAN_POINT ( 'NONE',  ( -5.413448473606448985, 9.537716662508005427, 0.000000000000000000 ) ) ;
#103259=CARTESIAN_POINT ( 'NONE',  ( 3.902768115887398803, 5.646591783325653147, -1.599625672291269396 ) ) ;
#103264=CARTESIAN_POINT ( 'NONE',  ( -6.424584688029276514, 8.588711117491191871, 1.599625672291269396 ) ) ;
#103268=CARTESIAN_POINT ( 'NONE',  ( -5.171509248969888617, 4.998125310078441075, 0.7998128361456281477 ) ) ;
#103271=CARTESIAN_POINT ( 'NONE',  ( 3.390947816749319443, 6.970206529600588397, -1.734723475976807094E-15 ) ) ;
#103272=CARTESIAN_POINT ( 'NONE',  ( -3.485854892044994102, 7.080931450778859215, -0.7216878364870458196 ) ) ;
#103274=ORIENTED_EDGE ( 'NONE', *, *, #210003, .T. ) ;
#103277=CARTESIAN_POINT ( 'NONE',  ( -6.296835998904160014, 6.311006518335105397, 0.000000000000000000 ) ) ;
#103286=CARTESIAN_POINT ( 'NONE',  ( 4.878955176071344546, 6.785476686873604280, -1.599625672291269396 ) ) ;
#103290=CARTESIAN_POINT ( 'NONE',  ( 0.1895306985669804323, 2.637130183346470869, -2.069997288510221800 ) ) ;
#103291=CARTESIAN_POINT ( 'NONE',  ( 5.043764445095213489, 7.992138250556588552, 1.161813593947092382 ) ) ;
#103295=CARTESIAN_POINT ( 'NONE',  ( 0.2053016774634074115, 2.557622706723280182, 1.991036163670555359 ) ) ;
#103300=CARTESIAN_POINT ( 'NONE',  ( 6.821687566331318564, 7.987665577921906568, 1.199719254218452935 ) ) ;
#103311=CARTESIAN_POINT ( 'NONE',  ( 6.276967689384127524, 6.888745287521969907, 0.7578909454171089966 ) ) ;
#103325=CARTESIAN_POINT ( 'NONE',  ( 4.072979602660211640, 7.274571027119063338, -0.9456576254009234628 ) ) ;
#103328=CARTESIAN_POINT ( 'NONE',  ( -5.094831863685302942, 9.165997284266655498, 0.7998128361456291469 ) ) ;
#103340=CARTESIAN_POINT ( 'NONE',  ( 4.715203562502613188, 8.723097599553565118, 0.7998128361456341429 ) ) ;
#103353=CARTESIAN_POINT ( 'NONE',  ( 4.163762572728282763, 6.911454530608037494, -1.082531754730548412 ) ) ;
#103354=DIRECTION ( 'NONE',  ( -0.6507913734559640506, -0.7592566023653003482, 0.000000000000000000 ) ) ;
#103365=ORIENTED_EDGE ( 'NONE', *, *, #55251, .T. ) ;
#103368=CARTESIAN_POINT ( 'NONE',  ( -6.997416678428844072, 8.296645891989347987, 1.082531754730549078 ) ) ;
#103369=CARTESIAN_POINT ( 'NONE',  ( 6.590672070018850803, 7.822110515511036866, -1.082531754730548412 ) ) ;
#103380=CARTESIAN_POINT ( 'NONE',  ( -5.971440312176176768, 5.931378217152456500, 0.000000000000000000 ) ) ;
#103381=CARTESIAN_POINT ( 'NONE',  ( -4.995253251992230581, 4.792493313604505367, 0.000000000000000000 ) ) ;
#103383=CARTESIAN_POINT ( 'NONE',  ( 4.692530563661249765, 8.488719734331187539, 0.000000000000000000 ) ) ;
#103385=ORIENTED_EDGE ( 'NONE', *, *, #117140, .F. ) ;
#103395=CARTESIAN_POINT ( 'NONE',  ( -4.740694425254917910, 8.216228820413899570, 0.6995903363472668612 ) ) ;
#103404=CARTESIAN_POINT ( 'NONE',  ( -5.550083779947821760, 7.568460058062819407, -1.599625672291271394 ) ) ;
#103417=CARTESIAN_POINT ( 'NONE',  ( 5.716698046817569434, 6.698511138489155137, -1.199719254218452047 ) ) ;
#103444=CONICAL_SURFACE ( 'NONE', #124266, 1249.999999999991587, 0.8960553845713407073 ) ;
#103454=CARTESIAN_POINT ( 'NONE',  ( 6.075462232699553766, 6.260663157670496304, -0.7216878364870458196 ) ) ;
#103459=CARTESIAN_POINT ( 'NONE',  ( 7.160114521348466710, 7.526090827760914870, 0.000000000000000000 ) ) ;
#103473=CARTESIAN_POINT ( 'NONE',  ( -6.770317605177755382, 8.992066187497757213, 1.599625672291269396 ) ) ;
#103485=CARTESIAN_POINT ( 'NONE',  ( -4.004454267989906668, 5.765225627445230927, 1.599625672291270506 ) ) ;
#103487=CARTESIAN_POINT ( 'NONE',  ( 4.380693030546916944, 6.204170850428461392, 1.443375672974058777 ) ) ;
#103493=CARTESIAN_POINT ( 'NONE',  ( -5.327428015527048366, 5.180030537728460338, -0.7998128361456362523 ) ) ;
#103498=CARTESIAN_POINT ( 'NONE',  ( -7.444835747679825033, 7.858265591814152629, 0.000000000000000000 ) ) ;
#103502=CARTESIAN_POINT ( 'NONE',  ( -5.413448473606448985, 9.537716662508005427, 0.000000000000000000 ) ) ;
#103507=B_SPLINE_CURVE_WITH_KNOTS ( 'NONE', 3,
 ( #24631, #143783, #142704, #11589, #77662, #90738 ),
 .UNSPECIFIED., .F., .F.,
 ( 4, 2, 4 ),
 ( 0.000000000000000000, 0.3573083853819281064, 0.7146167707638562128 ),
 .UNSPECIFIED. ) ;
#103508=CARTESIAN_POINT ( 'NONE',  ( -2.959422669532919326, 6.674686557755516780, 0.7998128361456352531 ) ) ;
#103522=CARTESIAN_POINT ( 'NONE',  ( -2.862179826260718762, 6.353310540697199471, 0.000000000000000000 ) ) ;
#103524=CARTESIAN_POINT ( 'NONE',  ( -5.790741006368224753, 5.928488393617260321, 0.7216878364870257245 ) ) ;
#103526=CARTESIAN_POINT ( 'NONE',  ( 4.736594563127852098, 6.619389305106191834, -1.599625672291273171 ) ) ;
#103527=CARTESIAN_POINT ( 'NONE',  ( -5.492988512192097161, 6.437516681426083132, 1.199719254218452935 ) ) ;
#103528=CARTESIAN_POINT ( 'NONE',  ( -6.444921918449773024, 8.612437886315108315, 1.599625672291269396 ) ) ;
#103554=CARTESIAN_POINT ( 'NONE',  ( -7.608060475923978494, 8.905100639113307182, 1.199719254218452047 ) ) ;
#103568=CARTESIAN_POINT ( 'NONE',  ( 4.517335436343476118, 8.499999999999996447, -0.7749999999999996891 ) ) ;
#103577=CARTESIAN_POINT ( 'NONE',  ( -6.966220764712148572, 6.002124920821316323, 2.420000000000000373 ) ) ;
#103585=CARTESIAN_POINT ( 'NONE',  ( 3.711900195091365262, 7.552577004240394132, -0.7998128361456362523 ) ) ;
#103586=CARTESIAN_POINT ( 'NONE',  ( 6.400857919427532572, 6.640291458853147866, -0.7216878364870458196 ) ) ;
#103600=CARTESIAN_POINT ( 'NONE',  ( 4.960304097753311936, 6.880383762169266504, 1.599625672291268286 ) ) ;
#103608=CARTESIAN_POINT ( 'NONE',  ( -7.273023059088104425, 7.449891421883056530, 0.000000000000000000 ) ) ;
#103613=CARTESIAN_POINT ( 'NONE',  ( 3.250922972226694352, 7.014770244231638863, 0.7998128361456281477 ) ) ;
#103626=CARTESIAN_POINT ( 'NONE',  ( 6.536439455564168277, 6.798469917679251573, 0.7216878364870328300 ) ) ;
#103628=CARTESIAN_POINT ( 'NONE',  ( -3.526529353330350336, 7.128384988945109413, -0.7216878364870458196 ) ) ;
#103629=CARTESIAN_POINT ( 'NONE',  ( -6.771371375382467583, 6.864631124226471037, -0.7998128361456362523 ) ) ;
#103641=CARTESIAN_POINT ( 'NONE',  ( 5.713835393516482952, 5.630839145382857680, 0.7998128361456352531 ) ) ;
#103642=CARTESIAN_POINT ( 'NONE',  ( 6.873057527484919937, 6.983264968346048818, 0.7998128361456352531 ) ) ;
#103657=( BOUNDED_SURFACE ( )  B_SPLINE_SURFACE ( 1, 2, ( 
 ( #38485, #20076, #202005, #150112, #138131, #170607, #37409, #1685, #199895, #103485, #117666, #87231, #3807, #204140, #121950, #51542, #183659, #35263, #134940, #23273, #124096, #190060, #172767, #159705, #208432, #43847, #155433, #141368, #89384, #24340, #76318, #9183, #74195, #139195, #75254, #140289, #173847, #60066, #90450, #123042, #109961, #156516, #41712, #7018, #73094, #206308, #77382, #40636, #59001, #209494, #205225, #107822, #106738, #188993, #56866, #158644, #25423, #207380, #193267, #175971, #92601, #191116, #44913, #171676, #125157, #8107, #42782, #91530, #108891, #174914, #57932, #157588, #27565, #26494, #10242, #142423, #126222, #192183, #11304, #93663, #143499, #61135, #127297, #177026, #178100, #15560, #162918, #148786, #97927, #29717, #82707, #112098, #14498, #65372, #197522, #163985, #28643, #12369, #131519, #78449, #49166, #179165, #95799, #47044, #115284, #129431, #45977, #81647, #113161, #80590, #48118, #111021, #62211, #30789, #147734, #146686, #128368, #144567, #114230, #212702, #96868, #64343, #130488, #181275, #31851, #161855, #32901, #98979, #63270, #165032, #180228, #194335, #210580, #13444, #79521, #145639, #196476, #356, #211634, #16625, #195415, #213749, #66429, #132572, #94730, #160776, #198574, #117414, #183410, #100036, #71770, #134698, #67499, #69638, #51289, #35014, #200703, #116341, #37160, #20882, #166098, #199643, #185532, #101085, #149865, #167174, #36084, #2497, #102167, #86981, #53409, #153051, #70697, #184466, #202838, #52354, #5693, #136811, #1433, #3565, #18761, #84846, #54486, #118481, #120631, #168235, #103238, #137886, #19834, #50221, #4626, #150936, #21942, #38235, #186608, #133642, #201769, #182332, #119547, #85918, #88052, #17686, #154123, #83772, #68571, #151991, #169298, #135746, #33960, #104309, #170357, #208183, #175713, #41460, #89138, #172514, #140030, #190867, #159447, #204975, #76067, #157334, #173603, #171433, #188745, #56621, #25175, #125970, #58751, #138955, #121707, #122785, #72849, #207126, #40384, #203906, #27304, #57690, #124904, #75006, #174662 ),
 ( #108635, #107568, #93410, #42531, #106487, #11045, #24100, #91277, #158392, #142166, #26237, #187670, #105393, #9989, #23021, #59815, #123847, #90203, #206055, #191926, #7849, #156267, #92354, #189808, #8925, #141115, #55553, #155192, #43591, #109709, #77124, #6773, #73936, #39300, #30532, #145385, #96612, #211383, #97671, #210318, #94476, #81397, #128113, #95549, #127040, #193000, #177847, #48909, #12120, #162666, #181027, #209236, #13190, #78194, #160517, #28382, #130230, #79268, #46792, #164781, #147481, #64087, #14235, #16372, #143247, #112906, #144320, #178917, #161601, #80330, #146431, #110767, #111843, #213501, #60881, #44653, #63010, #129180, #61954, #131281, #179974, #15309, #176766, #212445, #194071, #45724, #47866, #195158, #32645, #196224, #29460, #115029, #113977, #31595, #163728, #65124, #197269, #98722, #198325, #36900, #49965, #169040, #150682, #83517, #18516, #102982, #100837, #17434, #135492, #84594, #134451, #19585, #82450, #33706, #2243, #119291, #118227, #99783, #116083, #85657, #184213, #68320, #35836, #200454, #20637, #3314, #67248, #86726, #152795, #34763, #4375, #151744, #165848, #182074, #133383, #149598, #1184, #52100, #120373, #199388, #70446, #166922, #117157, #69384, #51034, #148540, #66173, #101914, #183160, #167979, #132319, #104056, #201514, #53162, #185277, #136562, #202583, #54235, #107, #186348, #37983, #170102, #203649, #73674, #138697, #23844, #124652, #157079, #75810, #74749, #206864, #109454, #153872, #172257, #71520, #189555, #8668, #57430, #56364, #92088, #191671, #87798, #123591, #122527, #106231, #171175, #91017, #204715, #188490, #140852, #41202, #43335, #72596, #40120, #139773, #58496, #24911, #107309, #39050, #108380, #22765, #89952, #173333, #156002, #190609, #21688, #174403, #42267, #25981, #158144, #9735, #7589, #141918, #137632, #88882, #207930, #154935, #121450, #6520, #205799, #59552, #125711, #5441, #55300, #187419, #105135, #95290, #113719, #45462, #131031, #47605, #126782, #128908, #11862, #28127, #195971, #29201, #179723, #161339, #13987, #197021 ) ),
 .UNSPECIFIED., .F., .F., .T. ) 
 B_SPLINE_SURFACE_WITH_KNOTS ( ( 2, 2 ),
 ( 3, 2, 2, 2, 2, 2, 2, 2, 2, 2, 2, 2, 2, 2, 2, 2, 2, 2, 2, 2, 2, 2, 2, 2, 2, 2, 2, 2, 2, 2, 2, 2, 2, 2, 2, 2, 2, 2, 2, 2, 2, 2, 2, 2, 2, 2, 2, 2, 2, 2, 2, 2, 2, 2, 2, 2, 2, 2, 2, 2, 2, 2, 2, 2, 2, 2, 2, 2, 2, 2, 2, 2, 2, 2, 2, 2, 2, 2, 2, 2, 2, 2, 2, 2, 2, 2, 2, 2, 2, 2, 2, 2, 2, 2, 2, 2, 2, 2, 2, 2, 2, 2, 2, 2, 2, 2, 2, 2, 2, 2, 2, 2, 2, 2, 2, 2, 2, 2, 2, 2, 3 ),
 ( 0.000000000000000000, 1.000000000000000000 ),
 ( 0.000000000000000000, 0.008333333333333333218, 0.01666666666666666644, 0.02500000000000000139, 0.03333333333333333287, 0.04166666666666666435, 0.05000000000000000278, 0.05833333333333333426, 0.06666666666666666574, 0.07499999999999999722, 0.08333333333333332871, 0.09166666666666666019, 0.1000000000000000056, 0.1083333333333333370, 0.1166666666666666685, 0.1250000000000000000, 0.1333333333333333315, 0.1416666666666666630, 0.1499999999999999944, 0.1583333333333333259, 0.1666666666666666574, 0.1749999999999999889, 0.1833333333333333204, 0.1916666666666666796, 0.2000000000000000111, 0.2083333333333333426, 0.2166666666666666741, 0.2250000000000000056, 0.2333333333333333370, 0.2416666666666666685, 0.2500000000000000000, 0.2583333333333333592, 0.2666666666666666630, 0.2750000000000000222, 0.2833333333333333259, 0.2916666666666666852, 0.2999999999999999889, 0.3083333333333333481, 0.3166666666666666519, 0.3250000000000000111, 0.3333333333333333148, 0.3416666666666666741, 0.3499999999999999778, 0.3583333333333333370, 0.3666666666666666408, 0.3750000000000000000, 0.3833333333333333592, 0.3916666666666666630, 0.4000000000000000222, 0.4083333333333333259, 0.4166666666666666852, 0.4249999999999999889, 0.4333333333333333481, 0.4416666666666666519, 0.4500000000000000111, 0.4583333333333333148, 0.4666666666666666741, 0.4749999999999999778, 0.4833333333333333370, 0.4916666666666666408, 0.5000000000000000000, 0.5083333333333333037, 0.5166666666666667185, 0.5250000000000000222, 0.5333333333333333259, 0.5416666666666666297, 0.5500000000000000444, 0.5583333333333333481, 0.5666666666666666519, 0.5749999999999999556, 0.5833333333333333703, 0.5916666666666666741, 0.5999999999999999778, 0.6083333333333332815, 0.6166666666666666963, 0.6250000000000000000, 0.6333333333333333037, 0.6416666666666667185, 0.6500000000000000222, 0.6583333333333333259, 0.6666666666666666297, 0.6750000000000000444, 0.6833333333333333481, 0.6916666666666666519, 0.6999999999999999556, 0.7083333333333333703, 0.7166666666666666741, 0.7249999999999999778, 0.7333333333333332815, 0.7416666666666666963, 0.7500000000000000000, 0.7583333333333333037, 0.7666666666666667185, 0.7750000000000000222, 0.7833333333333333259, 0.7916666666666666297, 0.8000000000000000444, 0.8083333333333333481, 0.8166666666666666519, 0.8249999999999999556, 0.8333333333333333703, 0.8416666666666666741, 0.8499999999999999778, 0.8583333333333332815, 0.8666666666666666963, 0.8750000000000000000, 0.8833333333333333037, 0.8916666666666667185, 0.9000000000000000222, 0.9083333333333333259, 0.9166666666666666297, 0.9250000000000000444, 0.9333333333333333481, 0.9416666666666666519, 0.9499999999999999556, 0.9583333333333333703, 0.9666666666666666741, 0.9749999999999999778, 0.9833333333333332815, 0.9916666666666666963, 1.000000000000000000 ),
 .UNSPECIFIED. ) 
 GEOMETRIC_REPRESENTATION_ITEM ( )  RATIONAL_B_SPLINE_SURFACE ( (
 ( 1.000000000000000000, 0.8660254037844387076, 1.000000000000000000, 0.8660254037844387076, 1.000000000000000000, 0.8660254037844387076, 1.000000000000000000, 0.8660254037844387076, 1.000000000000000000, 0.8660254037844387076, 1.000000000000000000, 0.8660254037844387076, 1.000000000000000000, 0.8660254037844387076, 1.000000000000000000, 0.8660254037844387076, 1.000000000000000000, 0.8660254037844387076, 1.000000000000000000, 0.8660254037844387076, 1.000000000000000000, 0.8660254037844387076, 1.000000000000000000, 0.8660254037844387076, 1.000000000000000000, 0.8660254037844387076, 1.000000000000000000, 0.8660254037844387076, 1.000000000000000000, 0.8660254037844387076, 1.000000000000000000, 0.8660254037844387076, 1.000000000000000000, 0.8660254037844387076, 1.000000000000000000, 0.8660254037844387076, 1.000000000000000000, 0.8660254037844387076, 1.000000000000000000, 0.8660254037844387076, 1.000000000000000000, 0.8660254037844387076, 1.000000000000000000, 0.8660254037844387076, 1.000000000000000000, 0.8660254037844387076, 1.000000000000000000, 0.8660254037844387076, 1.000000000000000000, 0.8660254037844387076, 1.000000000000000000, 0.8660254037844387076, 1.000000000000000000, 0.8660254037844387076, 1.000000000000000000, 0.8660254037844387076, 1.000000000000000000, 0.8660254037844387076, 1.000000000000000000, 0.8660254037844387076, 1.000000000000000000, 0.8660254037844387076, 1.000000000000000000, 0.8660254037844387076, 1.000000000000000000, 0.8660254037844387076, 1.000000000000000000, 0.8660254037844387076, 1.000000000000000000, 0.8660254037844387076, 1.000000000000000000, 0.8660254037844387076, 1.000000000000000000, 0.8660254037844387076, 1.000000000000000000, 0.8660254037844387076, 1.000000000000000000, 0.8660254037844387076, 1.000000000000000000, 0.8660254037844387076, 1.000000000000000000, 0.8660254037844387076, 1.000000000000000000, 0.8660254037844387076, 1.000000000000000000, 0.8660254037844387076, 1.000000000000000000, 0.8660254037844387076, 1.000000000000000000, 0.8660254037844387076, 1.000000000000000000, 0.8660254037844387076, 1.000000000000000000, 0.8660254037844387076, 1.000000000000000000, 0.8660254037844387076, 1.000000000000000000, 0.8660254037844387076, 1.000000000000000000, 0.8660254037844387076, 1.000000000000000000, 0.8660254037844387076, 1.000000000000000000, 0.8660254037844387076, 1.000000000000000000, 0.8660254037844387076, 1.000000000000000000, 0.8660254037844387076, 1.000000000000000000, 0.8660254037844387076, 1.000000000000000000, 0.8660254037844387076, 1.000000000000000000, 0.8660254037844387076, 1.000000000000000000, 0.8660254037844387076, 1.000000000000000000, 0.8660254037844387076, 1.000000000000000000, 0.8660254037844387076, 1.000000000000000000, 0.8660254037844387076, 1.000000000000000000, 0.8660254037844387076, 1.000000000000000000, 0.8660254037844387076, 1.000000000000000000, 0.8660254037844387076, 1.000000000000000000, 0.8660254037844387076, 1.000000000000000000, 0.8660254037844387076, 1.000000000000000000, 0.8660254037844387076, 1.000000000000000000, 0.8660254037844387076, 1.000000000000000000, 0.8660254037844387076, 1.000000000000000000, 0.8660254037844387076, 1.000000000000000000, 0.8660254037844387076, 1.000000000000000000, 0.8660254037844387076, 1.000000000000000000, 0.8660254037844387076, 1.000000000000000000, 0.8660254037844387076, 1.000000000000000000, 0.8660254037844387076, 1.000000000000000000, 0.8660254037844387076, 1.000000000000000000, 0.8660254037844387076, 1.000000000000000000, 0.8660254037844387076, 1.000000000000000000, 0.8660254037844387076, 1.000000000000000000, 0.8660254037844387076, 1.000000000000000000, 0.8660254037844387076, 1.000000000000000000, 0.8660254037844387076, 1.000000000000000000, 0.8660254037844387076, 1.000000000000000000, 0.8660254037844387076, 1.000000000000000000, 0.8660254037844387076, 1.000000000000000000, 0.8660254037844387076, 1.000000000000000000, 0.8660254037844387076, 1.000000000000000000, 0.8660254037844387076, 1.000000000000000000, 0.8660254037844387076, 1.000000000000000000, 0.8660254037844387076, 1.000000000000000000, 0.8660254037844387076, 1.000000000000000000, 0.8660254037844387076, 1.000000000000000000, 0.8660254037844387076, 1.000000000000000000, 0.8660254037844387076, 1.000000000000000000, 0.8660254037844387076, 1.000000000000000000, 0.8660254037844387076, 1.000000000000000000, 0.8660254037844387076, 1.000000000000000000, 0.8660254037844387076, 1.000000000000000000, 0.8660254037844387076, 1.000000000000000000, 0.8660254037844387076, 1.000000000000000000, 0.8660254037844387076, 1.000000000000000000, 0.8660254037844387076, 1.000000000000000000, 0.8660254037844387076, 1.000000000000000000, 0.8660254037844387076, 1.000000000000000000, 0.8660254037844387076, 1.000000000000000000, 0.8660254037844387076, 1.000000000000000000, 0.8660254037844387076, 1.000000000000000000, 0.8660254037844387076, 1.000000000000000000, 0.8660254037844387076, 1.000000000000000000, 0.8660254037844387076, 1.000000000000000000, 0.8660254037844387076, 1.000000000000000000, 0.8660254037844387076, 1.000000000000000000, 0.8660254037844387076, 1.000000000000000000, 0.8660254037844387076, 1.000000000000000000, 0.8660254037844387076, 1.000000000000000000, 0.8660254037844387076, 1.000000000000000000, 0.8660254037844387076, 1.000000000000000000, 0.8660254037844387076, 1.000000000000000000, 0.8660254037844387076, 1.000000000000000000, 0.8660254037844387076, 1.000000000000000000),
 ( 1.000000000000000000, 0.8660254037844387076, 1.000000000000000000, 0.8660254037844387076, 1.000000000000000000, 0.8660254037844387076, 1.000000000000000000, 0.8660254037844387076, 1.000000000000000000, 0.8660254037844387076, 1.000000000000000000, 0.8660254037844387076, 1.000000000000000000, 0.8660254037844387076, 1.000000000000000000, 0.8660254037844387076, 1.000000000000000000, 0.8660254037844387076, 1.000000000000000000, 0.8660254037844387076, 1.000000000000000000, 0.8660254037844387076, 1.000000000000000000, 0.8660254037844387076, 1.000000000000000000, 0.8660254037844387076, 1.000000000000000000, 0.8660254037844387076, 1.000000000000000000, 0.8660254037844387076, 1.000000000000000000, 0.8660254037844387076, 1.000000000000000000, 0.8660254037844387076, 1.000000000000000000, 0.8660254037844387076, 1.000000000000000000, 0.8660254037844387076, 1.000000000000000000, 0.8660254037844387076, 1.000000000000000000, 0.8660254037844387076, 1.000000000000000000, 0.8660254037844387076, 1.000000000000000000, 0.8660254037844387076, 1.000000000000000000, 0.8660254037844387076, 1.000000000000000000, 0.8660254037844387076, 1.000000000000000000, 0.8660254037844387076, 1.000000000000000000, 0.8660254037844387076, 1.000000000000000000, 0.8660254037844387076, 1.000000000000000000, 0.8660254037844387076, 1.000000000000000000, 0.8660254037844387076, 1.000000000000000000, 0.8660254037844387076, 1.000000000000000000, 0.8660254037844387076, 1.000000000000000000, 0.8660254037844387076, 1.000000000000000000, 0.8660254037844387076, 1.000000000000000000, 0.8660254037844387076, 1.000000000000000000, 0.8660254037844387076, 1.000000000000000000, 0.8660254037844387076, 1.000000000000000000, 0.8660254037844387076, 1.000000000000000000, 0.8660254037844387076, 1.000000000000000000, 0.8660254037844387076, 1.000000000000000000, 0.8660254037844387076, 1.000000000000000000, 0.8660254037844387076, 1.000000000000000000, 0.8660254037844387076, 1.000000000000000000, 0.8660254037844387076, 1.000000000000000000, 0.8660254037844387076, 1.000000000000000000, 0.8660254037844387076, 1.000000000000000000, 0.8660254037844387076, 1.000000000000000000, 0.8660254037844387076, 1.000000000000000000, 0.8660254037844387076, 1.000000000000000000, 0.8660254037844387076, 1.000000000000000000, 0.8660254037844387076, 1.000000000000000000, 0.8660254037844387076, 1.000000000000000000, 0.8660254037844387076, 1.000000000000000000, 0.8660254037844387076, 1.000000000000000000, 0.8660254037844387076, 1.000000000000000000, 0.8660254037844387076, 1.000000000000000000, 0.8660254037844387076, 1.000000000000000000, 0.8660254037844387076, 1.000000000000000000, 0.8660254037844387076, 1.000000000000000000, 0.8660254037844387076, 1.000000000000000000, 0.8660254037844387076, 1.000000000000000000, 0.8660254037844387076, 1.000000000000000000, 0.8660254037844387076, 1.000000000000000000, 0.8660254037844387076, 1.000000000000000000, 0.8660254037844387076, 1.000000000000000000, 0.8660254037844387076, 1.000000000000000000, 0.8660254037844387076, 1.000000000000000000, 0.8660254037844387076, 1.000000000000000000, 0.8660254037844387076, 1.000000000000000000, 0.8660254037844387076, 1.000000000000000000, 0.8660254037844387076, 1.000000000000000000, 0.8660254037844387076, 1.000000000000000000, 0.8660254037844387076, 1.000000000000000000, 0.8660254037844387076, 1.000000000000000000, 0.8660254037844387076, 1.000000000000000000, 0.8660254037844387076, 1.000000000000000000, 0.8660254037844387076, 1.000000000000000000, 0.8660254037844387076, 1.000000000000000000, 0.8660254037844387076, 1.000000000000000000, 0.8660254037844387076, 1.000000000000000000, 0.8660254037844387076, 1.000000000000000000, 0.8660254037844387076, 1.000000000000000000, 0.8660254037844387076, 1.000000000000000000, 0.8660254037844387076, 1.000000000000000000, 0.8660254037844387076, 1.000000000000000000, 0.8660254037844387076, 1.000000000000000000, 0.8660254037844387076, 1.000000000000000000, 0.8660254037844387076, 1.000000000000000000, 0.8660254037844387076, 1.000000000000000000, 0.8660254037844387076, 1.000000000000000000, 0.8660254037844387076, 1.000000000000000000, 0.8660254037844387076, 1.000000000000000000, 0.8660254037844387076, 1.000000000000000000, 0.8660254037844387076, 1.000000000000000000, 0.8660254037844387076, 1.000000000000000000, 0.8660254037844387076, 1.000000000000000000, 0.8660254037844387076, 1.000000000000000000, 0.8660254037844387076, 1.000000000000000000, 0.8660254037844387076, 1.000000000000000000, 0.8660254037844387076, 1.000000000000000000, 0.8660254037844387076, 1.000000000000000000, 0.8660254037844387076, 1.000000000000000000, 0.8660254037844387076, 1.000000000000000000, 0.8660254037844387076, 1.000000000000000000, 0.8660254037844387076, 1.000000000000000000, 0.8660254037844387076, 1.000000000000000000, 0.8660254037844387076, 1.000000000000000000, 0.8660254037844387076, 1.000000000000000000, 0.8660254037844387076, 1.000000000000000000, 0.8660254037844387076, 1.000000000000000000, 0.8660254037844387076, 1.000000000000000000, 0.8660254037844387076, 1.000000000000000000, 0.8660254037844387076, 1.000000000000000000, 0.8660254037844387076, 1.000000000000000000, 0.8660254037844387076, 1.000000000000000000, 0.8660254037844387076, 1.000000000000000000, 0.8660254037844387076, 1.000000000000000000, 0.8660254037844387076, 1.000000000000000000, 0.8660254037844387076, 1.000000000000000000, 0.8660254037844387076, 1.000000000000000000) ) ) 
 REPRESENTATION_ITEM ( '' )  SURFACE ( )  );
#103664=CARTESIAN_POINT ( 'NONE',  ( 6.083581728852979431, 7.123651168416324175, -1.137916992902558100 ) ) ;
#103668=DIRECTION ( 'NONE',  ( 0.7592566023652995710, -0.6507913734559650498, -0.000000000000000000 ) ) ;
#103673=CARTESIAN_POINT ( 'NONE',  ( 5.194709132691408549, 6.089524072008651423, 1.199719254218452935 ) ) ;
#103678=CARTESIAN_POINT ( 'NONE',  ( 5.182959862174088883, 9.268813282503625572, 0.7998128361456331437 ) ) ;
#103682=CARTESIAN_POINT ( 'NONE',  ( 5.058600711674583472, 8.915801573680086634, 0.000000000000000000 ) ) ;
#103685=CARTESIAN_POINT ( 'NONE',  ( 7.688882512725796481, 8.142986817701137525, 0.000000000000000000 ) ) ;
#103686=VERTEX_POINT ( 'NONE', #96931 ) ;
#103696=CARTESIAN_POINT ( 'NONE',  ( 6.335378924966214242, 6.849830188997488634, 0.6565068261209184852 ) ) ;
#103697=CARTESIAN_POINT ( 'NONE',  ( -6.292392690518202159, 9.394856334696294553, -1.082531754730549967 ) ) ;
#103705=CARTESIAN_POINT ( 'NONE',  ( 0.2798451837294911870, 3.302884587574776099, -1.982903847885383763 ) ) ;
#103730=CARTESIAN_POINT ( 'NONE',  ( 4.857564175446106525, 8.889184981320973122, 0.7998128361456331437 ) ) ;
#103732=CARTESIAN_POINT ( 'NONE',  ( 7.876360894896227371, 8.153785563659219804, -0.7998128361456341429 ) ) ;
#103739=FILL_AREA_STYLE_COLOUR ( '', #37786 ) ;
#103746=CARTESIAN_POINT ( 'NONE',  ( -4.122561227007127016, 6.967349310553715647, 1.199719254218452935 ) ) ;
#103748=CARTESIAN_POINT ( 'NONE',  ( 4.692530563661249765, 8.488719734331187539, 0.000000000000000000 ) ) ;
#103759=CARTESIAN_POINT ( 'NONE',  ( -3.797165540279144214, 6.587721009371067638, 1.199719254218452935 ) ) ;
#103766=CARTESIAN_POINT ( 'NONE',  ( -3.471769853551161411, 6.208092708188416076, 1.199719254218452935 ) ) ;
#103768=CARTESIAN_POINT ( 'NONE',  ( -4.502716413514296079, 8.267269892493059658, -0.7216878364870338292 ) ) ;
#103778=AXIS2_PLACEMENT_3D ( 'NONE', #19966, #184601, #117549 ) ;
#103790=CARTESIAN_POINT ( 'NONE',  ( -4.606738333593328072, 8.596554832492683929, 0.7998128361456281477 ) ) ;
#103793=CARTESIAN_POINT ( 'NONE',  ( -3.492107083971660586, 6.231819477012331632, 1.199719254218452935 ) ) ;
#103802=CARTESIAN_POINT ( 'NONE',  ( -6.335246490290919574, 6.944623119882351148, -0.8941629942194727620 ) ) ;
#103831=CARTESIAN_POINT ( 'NONE',  ( 6.086684617892325733, 6.065829907154645539, -0.7998128361456481317 ) ) ;
#103839=CARTESIAN_POINT ( 'NONE',  ( 6.658989722967328717, 7.797851427330578566, 1.199719254218452935 ) ) ;
#103841=CARTESIAN_POINT ( 'NONE',  ( 5.611095471209277541, 7.639640364534566075, 1.599625672291268286 ) ) ;
#103843=( BOUNDED_SURFACE ( )  B_SPLINE_SURFACE ( 1, 2, ( 
 ( #54528, #120673, #186651, #10036, #90242, #7892, #76110, #156308, #190911, #142214, #106530, #206098, #91321, #203945, #171476, #207170, #57732, #123889, #41500, #107613, #121747, #55592, #157379, #188792, #189855, #73980, #172556, #138999, #173644, #208228, #140074, #25217, #59860, #8973, #42576, #126012, #24140, #75047, #141162, #187715, #23066, #58794, #124949, #108679, #174707, #26283, #39344, #92397, #205021, #122831, #158435, #191972, #175764, #43639, #109754, #88096, #56667, #154169, #5735, #71814, #137924, #72893, #105440, #89182, #155234, #6815, #40427, #27357, #193051, #127088, #31643, #44705, #29507, #95600, #178965, #161648, #12171, #80381, #210366, #195203, #15357, #209284, #212496, #110812, #93459, #60931, #128162, #78243, #194123, #144365, #143293, #112954, #159496, #30580, #146477, #13243, #115078, #11095, #130281, #196269, #213548, #45773, #145432, #176817, #111890, #79316, #211432, #177894, #64137, #114027, #62006, #47916, #28432, #63063, #129230, #77171, #46840, #96661, #94525, #162714, #147527, #160563, #14286, #180022, #97720, #163778, #81450, #65171, #131326, #197320, #48960, #4420, #198371, #1229, #119339, #82499, #50011, #155, #18561, #165896, #135537, #2288, #185326, #67291, #117205, #66222, #86774, #32692, #152845, #134498, #52144, #133430, #53207, #19629, #150728, #83565, #182124, #149648, #132369, #54281, #70490, #116135, #33753, #151788, #85700, #199437, #181074, #98773, #200501, #51080, #118272, #99830, #148586, #100883, #17481, #164829, #184257, #35883, #101959, #36949, #202631, #169084, #136606, #183202, #3362, #16419, #34808, #166970, #103029, #69432, #84637, #168025, #20683, #201562, #68364, #170150, #105181, #91062, #204759, #158189, #139816, #188534, #5486, #123637, #189600, #124693, #23888, #74796, #7633, #39096, #89994, #141961, #171217, #207973, #21736, #122572, #156045, #120418, #186392, #41246, #40164, #157122, #205845, #8711, #87845, #106278, #73719, #104100, #174448, #140897, #154980, #206907, #153916, #58538, #42312, #138741, #203696, #56411, #172299, #92134, #57478 ),
 ( #107354, #190651, #108428, #9781, #24960, #173376, #26024, #75853, #38029, #71567, #137675, #55342, #121494, #187466, #22811, #88926, #6565, #72645, #45508, #161386, #125758, #130022, #61740, #162449, #176560, #97456, #11910, #14025, #77983, #175504, #145162, #191719, #211167, #178700, #127907, #147264, #43376, #80111, #146216, #31380, #144106, #177637, #27094, #210100, #111624, #193859, #29245, #96399, #212234, #44441, #63867, #60663, #95337, #12970, #59600, #79046, #62792, #126826, #128954, #179764, #192783, #110559, #194933, #46570, #93201, #28170, #30314, #94266, #112689, #196013, #163511, #76907, #160306, #47649, #159232, #143033, #10833, #113760, #15097, #81186, #109497, #209028, #99569, #149383, #98505, #119077, #64922, #185058, #180811, #2027, #165633, #116939, #67030, #83298, #49748, #84379, #135286, #965, #133167, #201300, #199167, #101695, #52940, #17221, #182939, #68096, #114812, #82237, #118013, #34555, #100626, #166702, #18293, #32437, #150466, #115875, #33496, #167765, #36683, #86512, #50813, #85442, #134231, #181860, #102770, #51890, #151527, #200240, #198117, #184002, #168825, #35617, #214328, #19362, #213296, #164567, #16152, #3096, #148328, #69166, #20429, #131072, #197060, #48698, #65960, #132109, #106021, #140641, #120156, #123381, #37767, #4164, #186132, #38835, #137414, #104918, #55087, #72381, #124442, #90803, #189346, #54017, #138480, #74541, #5227, #22559, #103839, #204502, #39912, #70234, #8453, #154724, #40986, #121236, #190400, #170959, #107097, #88664, #172042, #23635, #6307, #24701, #205584, #122314, #187206, #153658, #56152, #169888, #25770, #42058, #21477, #87586, #173120, #57221, #188271, #152577, #136346, #89743, #155792, #7376, #71301, #203433, #73455, #139557, #202368, #156867, #206654, #58286, #108171, #174197, #79857, #211976, #175254, #210915, #157937, #125502, #113504, #30054, #62542, #47391, #28988, #96144, #111370, #76658, #141714, #142773, #128704, #176312, #129771, #177374, #160051, #191465, #95074, #161123, #162195, #209842, #46317, #193610, #10584, #61481, #179512 ) ),
 .UNSPECIFIED., .F., .F., .F. ) 
 B_SPLINE_SURFACE_WITH_KNOTS ( ( 2, 2 ),
 ( 3, 2, 2, 2, 2, 2, 2, 2, 2, 2, 2, 2, 2, 2, 2, 2, 2, 2, 2, 2, 2, 2, 2, 2, 2, 2, 2, 2, 2, 2, 2, 2, 2, 2, 2, 2, 2, 2, 2, 2, 2, 2, 2, 2, 2, 2, 2, 2, 2, 2, 2, 2, 2, 2, 2, 2, 2, 2, 2, 2, 2, 2, 2, 2, 2, 2, 2, 2, 2, 2, 2, 2, 2, 2, 2, 2, 2, 2, 2, 2, 2, 2, 2, 2, 2, 2, 2, 2, 2, 2, 2, 2, 2, 2, 2, 2, 2, 2, 2, 2, 2, 2, 2, 2, 2, 2, 2, 2, 2, 2, 2, 2, 2, 2, 2, 2, 2, 2, 2, 2, 3 ),
 ( 0.000000000000000000, 1.000000000000000000 ),
 ( 0.000000000000000000, 0.008333333333333333218, 0.01666666666666666644, 0.02500000000000000139, 0.03333333333333333287, 0.04166666666666666435, 0.05000000000000000278, 0.05833333333333333426, 0.06666666666666666574, 0.07499999999999999722, 0.08333333333333332871, 0.09166666666666666019, 0.1000000000000000056, 0.1083333333333333370, 0.1166666666666666685, 0.1250000000000000000, 0.1333333333333333315, 0.1416666666666666630, 0.1499999999999999944, 0.1583333333333333259, 0.1666666666666666574, 0.1749999999999999889, 0.1833333333333333204, 0.1916666666666666796, 0.2000000000000000111, 0.2083333333333333426, 0.2166666666666666741, 0.2250000000000000056, 0.2333333333333333370, 0.2416666666666666685, 0.2500000000000000000, 0.2583333333333333592, 0.2666666666666666630, 0.2750000000000000222, 0.2833333333333333259, 0.2916666666666666852, 0.2999999999999999889, 0.3083333333333333481, 0.3166666666666666519, 0.3250000000000000111, 0.3333333333333333148, 0.3416666666666666741, 0.3499999999999999778, 0.3583333333333333370, 0.3666666666666666408, 0.3750000000000000000, 0.3833333333333333592, 0.3916666666666666630, 0.4000000000000000222, 0.4083333333333333259, 0.4166666666666666852, 0.4249999999999999889, 0.4333333333333333481, 0.4416666666666666519, 0.4500000000000000111, 0.4583333333333333148, 0.4666666666666666741, 0.4749999999999999778, 0.4833333333333333370, 0.4916666666666666408, 0.5000000000000000000, 0.5083333333333333037, 0.5166666666666667185, 0.5250000000000000222, 0.5333333333333333259, 0.5416666666666666297, 0.5500000000000000444, 0.5583333333333333481, 0.5666666666666666519, 0.5749999999999999556, 0.5833333333333333703, 0.5916666666666666741, 0.5999999999999999778, 0.6083333333333332815, 0.6166666666666666963, 0.6250000000000000000, 0.6333333333333333037, 0.6416666666666667185, 0.6500000000000000222, 0.6583333333333333259, 0.6666666666666666297, 0.6750000000000000444, 0.6833333333333333481, 0.6916666666666666519, 0.6999999999999999556, 0.7083333333333333703, 0.7166666666666666741, 0.7249999999999999778, 0.7333333333333332815, 0.7416666666666666963, 0.7500000000000000000, 0.7583333333333333037, 0.7666666666666667185, 0.7750000000000000222, 0.7833333333333333259, 0.7916666666666666297, 0.8000000000000000444, 0.8083333333333333481, 0.8166666666666666519, 0.8249999999999999556, 0.8333333333333333703, 0.8416666666666666741, 0.8499999999999999778, 0.8583333333333332815, 0.8666666666666666963, 0.8750000000000000000, 0.8833333333333333037, 0.8916666666666667185, 0.9000000000000000222, 0.9083333333333333259, 0.9166666666666666297, 0.9250000000000000444, 0.9333333333333333481, 0.9416666666666666519, 0.9499999999999999556, 0.9583333333333333703, 0.9666666666666666741, 0.9749999999999999778, 0.9833333333333332815, 0.9916666666666666963, 1.000000000000000000 ),
 .UNSPECIFIED. ) 
 GEOMETRIC_REPRESENTATION_ITEM ( )  RATIONAL_B_SPLINE_SURFACE ( (
 ( 1.000000000000000000, 0.8660254037844387076, 1.000000000000000000, 0.8660254037844387076, 1.000000000000000000, 0.8660254037844387076, 1.000000000000000000, 0.8660254037844387076, 1.000000000000000000, 0.8660254037844387076, 1.000000000000000000, 0.8660254037844387076, 1.000000000000000000, 0.8660254037844387076, 1.000000000000000000, 0.8660254037844387076, 1.000000000000000000, 0.8660254037844387076, 1.000000000000000000, 0.8660254037844387076, 1.000000000000000000, 0.8660254037844387076, 1.000000000000000000, 0.8660254037844387076, 1.000000000000000000, 0.8660254037844387076, 1.000000000000000000, 0.8660254037844387076, 1.000000000000000000, 0.8660254037844387076, 1.000000000000000000, 0.8660254037844387076, 1.000000000000000000, 0.8660254037844387076, 1.000000000000000000, 0.8660254037844387076, 1.000000000000000000, 0.8660254037844387076, 1.000000000000000000, 0.8660254037844387076, 1.000000000000000000, 0.8660254037844387076, 1.000000000000000000, 0.8660254037844387076, 1.000000000000000000, 0.8660254037844387076, 1.000000000000000000, 0.8660254037844387076, 1.000000000000000000, 0.8660254037844387076, 1.000000000000000000, 0.8660254037844387076, 1.000000000000000000, 0.8660254037844387076, 1.000000000000000000, 0.8660254037844387076, 1.000000000000000000, 0.8660254037844387076, 1.000000000000000000, 0.8660254037844387076, 1.000000000000000000, 0.8660254037844387076, 1.000000000000000000, 0.8660254037844387076, 1.000000000000000000, 0.8660254037844387076, 1.000000000000000000, 0.8660254037844387076, 1.000000000000000000, 0.8660254037844387076, 1.000000000000000000, 0.8660254037844387076, 1.000000000000000000, 0.8660254037844387076, 1.000000000000000000, 0.8660254037844387076, 1.000000000000000000, 0.8660254037844387076, 1.000000000000000000, 0.8660254037844387076, 1.000000000000000000, 0.8660254037844387076, 1.000000000000000000, 0.8660254037844387076, 1.000000000000000000, 0.8660254037844387076, 1.000000000000000000, 0.8660254037844387076, 1.000000000000000000, 0.8660254037844387076, 1.000000000000000000, 0.8660254037844387076, 1.000000000000000000, 0.8660254037844387076, 1.000000000000000000, 0.8660254037844387076, 1.000000000000000000, 0.8660254037844387076, 1.000000000000000000, 0.8660254037844387076, 1.000000000000000000, 0.8660254037844387076, 1.000000000000000000, 0.8660254037844387076, 1.000000000000000000, 0.8660254037844387076, 1.000000000000000000, 0.8660254037844387076, 1.000000000000000000, 0.8660254037844387076, 1.000000000000000000, 0.8660254037844387076, 1.000000000000000000, 0.8660254037844387076, 1.000000000000000000, 0.8660254037844387076, 1.000000000000000000, 0.8660254037844387076, 1.000000000000000000, 0.8660254037844387076, 1.000000000000000000, 0.8660254037844387076, 1.000000000000000000, 0.8660254037844387076, 1.000000000000000000, 0.8660254037844387076, 1.000000000000000000, 0.8660254037844387076, 1.000000000000000000, 0.8660254037844387076, 1.000000000000000000, 0.8660254037844387076, 1.000000000000000000, 0.8660254037844387076, 1.000000000000000000, 0.8660254037844387076, 1.000000000000000000, 0.8660254037844387076, 1.000000000000000000, 0.8660254037844387076, 1.000000000000000000, 0.8660254037844387076, 1.000000000000000000, 0.8660254037844387076, 1.000000000000000000, 0.8660254037844387076, 1.000000000000000000, 0.8660254037844387076, 1.000000000000000000, 0.8660254037844387076, 1.000000000000000000, 0.8660254037844387076, 1.000000000000000000, 0.8660254037844387076, 1.000000000000000000, 0.8660254037844387076, 1.000000000000000000, 0.8660254037844387076, 1.000000000000000000, 0.8660254037844387076, 1.000000000000000000, 0.8660254037844387076, 1.000000000000000000, 0.8660254037844387076, 1.000000000000000000, 0.8660254037844387076, 1.000000000000000000, 0.8660254037844387076, 1.000000000000000000, 0.8660254037844387076, 1.000000000000000000, 0.8660254037844387076, 1.000000000000000000, 0.8660254037844387076, 1.000000000000000000, 0.8660254037844387076, 1.000000000000000000, 0.8660254037844387076, 1.000000000000000000, 0.8660254037844387076, 1.000000000000000000, 0.8660254037844387076, 1.000000000000000000, 0.8660254037844387076, 1.000000000000000000, 0.8660254037844387076, 1.000000000000000000, 0.8660254037844387076, 1.000000000000000000, 0.8660254037844387076, 1.000000000000000000, 0.8660254037844387076, 1.000000000000000000, 0.8660254037844387076, 1.000000000000000000, 0.8660254037844387076, 1.000000000000000000, 0.8660254037844387076, 1.000000000000000000, 0.8660254037844387076, 1.000000000000000000, 0.8660254037844387076, 1.000000000000000000, 0.8660254037844387076, 1.000000000000000000, 0.8660254037844387076, 1.000000000000000000, 0.8660254037844387076, 1.000000000000000000, 0.8660254037844387076, 1.000000000000000000, 0.8660254037844387076, 1.000000000000000000, 0.8660254037844387076, 1.000000000000000000, 0.8660254037844387076, 1.000000000000000000, 0.8660254037844387076, 1.000000000000000000, 0.8660254037844387076, 1.000000000000000000, 0.8660254037844387076, 1.000000000000000000, 0.8660254037844387076, 1.000000000000000000, 0.8660254037844387076, 1.000000000000000000, 0.8660254037844387076, 1.000000000000000000, 0.8660254037844387076, 1.000000000000000000, 0.8660254037844387076, 1.000000000000000000, 0.8660254037844387076, 1.000000000000000000, 0.8660254037844387076, 1.000000000000000000, 0.8660254037844387076, 1.000000000000000000, 0.8660254037844387076, 1.000000000000000000),
 ( 1.000000000000000000, 0.8660254037844387076, 1.000000000000000000, 0.8660254037844387076, 1.000000000000000000, 0.8660254037844387076, 1.000000000000000000, 0.8660254037844387076, 1.000000000000000000, 0.8660254037844387076, 1.000000000000000000, 0.8660254037844387076, 1.000000000000000000, 0.8660254037844387076, 1.000000000000000000, 0.8660254037844387076, 1.000000000000000000, 0.8660254037844387076, 1.000000000000000000, 0.8660254037844387076, 1.000000000000000000, 0.8660254037844387076, 1.000000000000000000, 0.8660254037844387076, 1.000000000000000000, 0.8660254037844387076, 1.000000000000000000, 0.8660254037844387076, 1.000000000000000000, 0.8660254037844387076, 1.000000000000000000, 0.8660254037844387076, 1.000000000000000000, 0.8660254037844387076, 1.000000000000000000, 0.8660254037844387076, 1.000000000000000000, 0.8660254037844387076, 1.000000000000000000, 0.8660254037844387076, 1.000000000000000000, 0.8660254037844387076, 1.000000000000000000, 0.8660254037844387076, 1.000000000000000000, 0.8660254037844387076, 1.000000000000000000, 0.8660254037844387076, 1.000000000000000000, 0.8660254037844387076, 1.000000000000000000, 0.8660254037844387076, 1.000000000000000000, 0.8660254037844387076, 1.000000000000000000, 0.8660254037844387076, 1.000000000000000000, 0.8660254037844387076, 1.000000000000000000, 0.8660254037844387076, 1.000000000000000000, 0.8660254037844387076, 1.000000000000000000, 0.8660254037844387076, 1.000000000000000000, 0.8660254037844387076, 1.000000000000000000, 0.8660254037844387076, 1.000000000000000000, 0.8660254037844387076, 1.000000000000000000, 0.8660254037844387076, 1.000000000000000000, 0.8660254037844387076, 1.000000000000000000, 0.8660254037844387076, 1.000000000000000000, 0.8660254037844387076, 1.000000000000000000, 0.8660254037844387076, 1.000000000000000000, 0.8660254037844387076, 1.000000000000000000, 0.8660254037844387076, 1.000000000000000000, 0.8660254037844387076, 1.000000000000000000, 0.8660254037844387076, 1.000000000000000000, 0.8660254037844387076, 1.000000000000000000, 0.8660254037844387076, 1.000000000000000000, 0.8660254037844387076, 1.000000000000000000, 0.8660254037844387076, 1.000000000000000000, 0.8660254037844387076, 1.000000000000000000, 0.8660254037844387076, 1.000000000000000000, 0.8660254037844387076, 1.000000000000000000, 0.8660254037844387076, 1.000000000000000000, 0.8660254037844387076, 1.000000000000000000, 0.8660254037844387076, 1.000000000000000000, 0.8660254037844387076, 1.000000000000000000, 0.8660254037844387076, 1.000000000000000000, 0.8660254037844387076, 1.000000000000000000, 0.8660254037844387076, 1.000000000000000000, 0.8660254037844387076, 1.000000000000000000, 0.8660254037844387076, 1.000000000000000000, 0.8660254037844387076, 1.000000000000000000, 0.8660254037844387076, 1.000000000000000000, 0.8660254037844387076, 1.000000000000000000, 0.8660254037844387076, 1.000000000000000000, 0.8660254037844387076, 1.000000000000000000, 0.8660254037844387076, 1.000000000000000000, 0.8660254037844387076, 1.000000000000000000, 0.8660254037844387076, 1.000000000000000000, 0.8660254037844387076, 1.000000000000000000, 0.8660254037844387076, 1.000000000000000000, 0.8660254037844387076, 1.000000000000000000, 0.8660254037844387076, 1.000000000000000000, 0.8660254037844387076, 1.000000000000000000, 0.8660254037844387076, 1.000000000000000000, 0.8660254037844387076, 1.000000000000000000, 0.8660254037844387076, 1.000000000000000000, 0.8660254037844387076, 1.000000000000000000, 0.8660254037844387076, 1.000000000000000000, 0.8660254037844387076, 1.000000000000000000, 0.8660254037844387076, 1.000000000000000000, 0.8660254037844387076, 1.000000000000000000, 0.8660254037844387076, 1.000000000000000000, 0.8660254037844387076, 1.000000000000000000, 0.8660254037844387076, 1.000000000000000000, 0.8660254037844387076, 1.000000000000000000, 0.8660254037844387076, 1.000000000000000000, 0.8660254037844387076, 1.000000000000000000, 0.8660254037844387076, 1.000000000000000000, 0.8660254037844387076, 1.000000000000000000, 0.8660254037844387076, 1.000000000000000000, 0.8660254037844387076, 1.000000000000000000, 0.8660254037844387076, 1.000000000000000000, 0.8660254037844387076, 1.000000000000000000, 0.8660254037844387076, 1.000000000000000000, 0.8660254037844387076, 1.000000000000000000, 0.8660254037844387076, 1.000000000000000000, 0.8660254037844387076, 1.000000000000000000, 0.8660254037844387076, 1.000000000000000000, 0.8660254037844387076, 1.000000000000000000, 0.8660254037844387076, 1.000000000000000000, 0.8660254037844387076, 1.000000000000000000, 0.8660254037844387076, 1.000000000000000000, 0.8660254037844387076, 1.000000000000000000, 0.8660254037844387076, 1.000000000000000000, 0.8660254037844387076, 1.000000000000000000, 0.8660254037844387076, 1.000000000000000000, 0.8660254037844387076, 1.000000000000000000, 0.8660254037844387076, 1.000000000000000000, 0.8660254037844387076, 1.000000000000000000, 0.8660254037844387076, 1.000000000000000000, 0.8660254037844387076, 1.000000000000000000, 0.8660254037844387076, 1.000000000000000000, 0.8660254037844387076, 1.000000000000000000, 0.8660254037844387076, 1.000000000000000000, 0.8660254037844387076, 1.000000000000000000, 0.8660254037844387076, 1.000000000000000000, 0.8660254037844387076, 1.000000000000000000, 0.8660254037844387076, 1.000000000000000000, 0.8660254037844387076, 1.000000000000000000, 0.8660254037844387076, 1.000000000000000000) ) ) 
 REPRESENTATION_ITEM ( '' )  SURFACE ( )  );
#103855=CARTESIAN_POINT ( 'NONE',  ( 6.039396378094620488, 7.052381734106362821, -1.030794243266313082 ) ) ;
#103857=CARTESIAN_POINT ( 'NONE',  ( -6.766928066552171828, 7.067373297165212342, 0.7216878364870317197 ) ) ;
#103858=CARTESIAN_POINT ( 'NONE',  ( 6.238160076063542725, 6.450477308261824305, -0.7216878364870458196 ) ) ;
#103867=FACE_OUTER_BOUND ( 'NONE', #150655, .T. ) ;
#103877=CARTESIAN_POINT ( 'NONE',  ( -4.434925645001610128, 8.188180662561590495, 0.7216878364870338292 ) ) ;
#103882=CARTESIAN_POINT ( 'NONE',  ( 7.015418140428412386, 7.149352350113456822, 0.7998128361456331437 ) ) ;
#103925=DIRECTION ( 'NONE',  ( 0.000000000000000000, 0.000000000000000000, -1.000000000000000000 ) ) ;
#103944=CARTESIAN_POINT ( 'NONE',  ( 3.770576118376306241, 6.452737000530752276, 1.082531754730549078 ) ) ;
#103951=CARTESIAN_POINT ( 'NONE',  ( 6.851666526859736983, 9.086973262793417661, -1.599625672291269396 ) ) ;
#103954=CARTESIAN_POINT ( 'NONE',  ( -3.187575512988701565, 6.732938841879847480, 0.000000000000000000 ) ) ;
#103964=CARTESIAN_POINT ( 'NONE',  ( -5.438229012412899799, 7.437962829272074750, -1.443375672974066770 ) ) ;
#103967=DIRECTION ( 'NONE',  ( 0.6507913734559650498, 0.7592566023652995710, -0.000000000000000000 ) ) ;
#103975=CARTESIAN_POINT ( 'NONE',  ( 6.505933609711257226, 8.683618192786854095, -1.599625672291281386 ) ) ;
#103984=CARTESIAN_POINT ( 'NONE',  ( 4.415115299905642665, 5.179997933758551554, -1.199719254218450271 ) ) ;
#103996=CARTESIAN_POINT ( 'NONE',  ( -4.489158259900630554, 8.251452046610447510, 0.000000000000000000 ) ) ;
#103999=CARTESIAN_POINT ( 'NONE',  ( 5.501576472095266901, 9.640532660744973725, -0.7998128361456481317 ) ) ;
#104004=CARTESIAN_POINT ( 'NONE',  ( -5.764151584465413869, 6.753873599078290546, -1.199719254218453823 ) ) ;
#104044=CARTESIAN_POINT ( 'NONE',  ( 4.421367491832270957, 6.251624388594711590, 1.443375672974058777 ) ) ;
#104047=CARTESIAN_POINT ( 'NONE',  ( -6.038177310039794854, 8.137902509836795417, -1.599625672291271394 ) ) ;
#104051=CARTESIAN_POINT ( 'NONE',  ( -5.041653019435350380, 6.975290837464928728, -1.599625672291271394 ) ) ;
#104052=CARTESIAN_POINT ( 'NONE',  ( -4.305596300791617814, 7.180890229968955651, 1.199719254218452935 ) ) ;
#104054=EDGE_LOOP ( 'NONE', ( #202429, #176779 ) ) ;
#104056=CARTESIAN_POINT ( 'NONE',  ( -6.929625909916163451, 7.257187447756535903, 0.7216878364870317197 ) ) ;
#104061=CARTESIAN_POINT ( 'NONE',  ( -3.546339698426324460, 6.295090860542775779, -1.199719254218450271 ) ) ;
#104069=CARTESIAN_POINT ( 'NONE',  ( -7.282664789195997912, 8.525472337930658284, 1.199719254218452047 ) ) ;
#104071=CARTESIAN_POINT ( 'NONE',  ( 5.126881573038487794, 7.911131357477594328, 1.221340741751137493 ) ) ;
#104076=CARTESIAN_POINT ( 'NONE',  ( 3.898851692381625877, 6.706354853490643642, -1.199719254218452047 ) ) ;
#104084=DIRECTION ( 'NONE',  ( -0.7592566023652995710, -0.6507913734559651608, 0.000000000000000000 ) ) ;
#104088=CARTESIAN_POINT ( 'NONE',  ( -7.598418745816086783, 7.829519723065708092, 0.000000000000000000 ) ) ;
#104090=VERTEX_POINT ( 'NONE', #1495 ) ;
#104100=CARTESIAN_POINT ( 'NONE',  ( 7.991605200612358573, 8.288237253661408843, 0.7998128361456281477 ) ) ;
#104114=CARTESIAN_POINT ( 'NONE',  ( 6.170730229783032428, 7.061345527190763249, -1.063955632616358615 ) ) ;
#104118=CIRCLE ( 'NONE', #48772, 0.08000000000000041800 ) ;
#104143=CARTESIAN_POINT ( 'NONE',  ( -6.035068427865825313, 7.156668563632000435, 1.186355232826277417 ) ) ;
#104159=CARTESIAN_POINT ( 'NONE',  ( 3.565173639196337341, 7.339832546762534271, -0.2726055590975334786 ) ) ;
#104163=CARTESIAN_POINT ( 'NONE',  ( -5.815521545619021460, 5.749472989502435460, -0.7998128361456362523 ) ) ;
#104179=ORIENTED_EDGE ( 'NONE', *, *, #165266, .T. ) ;
#104181=CARTESIAN_POINT ( 'NONE',  ( -5.366912616075431686, 6.182013390275966636, 1.156538041605560174 ) ) ;
#104183=CARTESIAN_POINT ( 'NONE',  ( 6.333067150914805765, 9.442309871825708356, 1.082531754730549967 ) ) ;
#104194=ADVANCED_FACE ( 'NONE', ( #61747 ), #206674, .T. ) ;
#104198=CARTESIAN_POINT ( 'NONE',  ( 5.234329823327693809, 8.264412672927770487, 1.199719254218451159 ) ) ;
#104208=CARTESIAN_POINT ( 'NONE',  ( -3.980200614063634568, 6.801261928786307642, 1.199719254218452935 ) ) ;
#104209=CARTESIAN_POINT ( 'NONE',  ( 5.806634928402749196, 9.996434193103704402, -0.7998128361456481317 ) ) ;
#104213=CARTESIAN_POINT ( 'NONE',  ( -5.424143973919053785, 8.485862515284315677, 1.199719254218454489 ) ) ;
#104216=CARTESIAN_POINT ( 'NONE',  ( 7.686546744304875389, 7.932335721302671949, 0.7998128361456291469 ) ) ;
#104222=CARTESIAN_POINT ( 'NONE',  ( -4.587973201513257493, 8.494803767824503637, 0.1163994284540965235 ) ) ;
#104232=CARTESIAN_POINT ( 'NONE',  ( -3.634994581795317536, 7.254927755487573293, 0.000000000000000000 ) ) ;
#104241=CARTESIAN_POINT ( 'NONE',  ( 3.716343503921665459, 6.389465617000312569, -1.082531754730549967 ) ) ;
#104245=CARTESIAN_POINT ( 'NONE',  ( -4.749098946536820520, 8.762642214260091933, 0.7998128361456281477 ) ) ;
#104253=CARTESIAN_POINT ( 'NONE',  ( 4.318600669050584706, 4.999583595936801572, 2.499999999999999556 ) ) ;
#104261=CARTESIAN_POINT ( 'NONE',  ( -2.810282979782591006, 6.500690253046801814, 0.000000000000000000 ) ) ;
#104285=CARTESIAN_POINT ( 'NONE',  ( -4.163762573172648196, 7.871823745427799501, 0.000000000000000000 ) ) ;
#104309=CARTESIAN_POINT ( 'NONE',  ( -7.767895665986912057, 8.027242796598338614, -0.7998128361456362523 ) ) ;
#104315=CARTESIAN_POINT ( 'NONE',  ( -5.093022980588950865, 5.970890227889075419, -1.199719254218453823 ) ) ;
#104324=CARTESIAN_POINT ( 'NONE',  ( -7.075376061485238566, 9.347967719856493218, 1.599625672291269396 ) ) ;
#104330=CARTESIAN_POINT ( 'NONE',  ( 4.095444919779759552, 6.935713618788495793, 1.199719254218451159 ) ) ;
#104337=CARTESIAN_POINT ( 'NONE',  ( -7.096767062110449942, 7.244259425409119046, -0.7998128361456362523 ) ) ;
#104341=CARTESIAN_POINT ( 'NONE',  ( -3.284818356260900796, 7.054314858938165678, 0.7998128361456352531 ) ) ;
#104345=CARTESIAN_POINT ( 'NONE',  ( 4.055297343818931033, 6.784911763547157193, 1.082531754730549078 ) ) ;
#104346=CARTESIAN_POINT ( 'NONE',  ( -5.614485009390564940, 5.722856397143323726, 0.000000000000000000 ) ) ;
#104351=CARTESIAN_POINT ( 'NONE',  ( -4.447956913735107598, 7.346977611736363656, 1.199719254218452935 ) ) ;
#104355=ORIENTED_EDGE ( 'NONE', *, *, #171151, .F. ) ;
#104360=CARTESIAN_POINT ( 'NONE',  ( 4.016958651398847557, 7.908478536599130138, -0.7998128361456361413 ) ) ;
#104364=CARTESIAN_POINT ( 'NONE',  ( 0.4000000000062943761, 2.913060511812307407, -2.023857702505970302 ) ) ;
#104365=CARTESIAN_POINT ( 'NONE',  ( 5.997720278586790243, 7.186234674792547850, 1.197368251494409286 ) ) ;
#104367=VECTOR ( 'NONE', #162634, 1000.000000000000000 ) ;
#104375=CARTESIAN_POINT ( 'NONE',  ( 5.580062740476173566, 8.667767742934335828, 1.199719254218451159 ) ) ;
#104385=CARTESIAN_POINT ( 'NONE',  ( 6.210774601750883583, 6.933448576277219111, 0.8519936491524527922 ) ) ;
#104398=EDGE_CURVE ( 'NONE', #202042, #176704, #193867, .T. ) ;
#104402=CARTESIAN_POINT ( 'NONE',  ( -5.173318132066234476, 8.193232366456022930, -1.199719254218453823 ) ) ;
#104407=CARTESIAN_POINT ( 'NONE',  ( -3.735410078681058010, 7.355792676762846760, 0.6188595546183575102 ) ) ;
#104415=CARTESIAN_POINT ( 'NONE',  ( 4.864343252252968597, 8.897093904262280972, 0.000000000000000000 ) ) ;
#104428=CARTESIAN_POINT ( 'NONE',  ( 4.136646265500957043, 5.919449624541475607, -1.443375672974068769 ) ) ;
#104442=CARTESIAN_POINT ( 'NONE',  ( -3.471769853551161411, 6.208092708188416076, 1.199719254218452935 ) ) ;
#104443=CARTESIAN_POINT ( 'NONE',  ( 7.051649292883499953, 7.399548061218447437, -0.7216878364870317197 ) ) ;
#104447=( BOUNDED_CURVE ( )  B_SPLINE_CURVE ( 2, ( #119932, #67869, #166475, #200023, #185908, #71082, #20208 ),
 .UNSPECIFIED., .F., .T. ) 
 B_SPLINE_CURVE_WITH_KNOTS ( ( 3, 2, 2, 3 ),
 ( 0.2999999999999993783, 0.3083333333333330151, 0.3166666666666665408, 0.3250000000000001776 ),
 .UNSPECIFIED. ) 
 CURVE ( )  GEOMETRIC_REPRESENTATION_ITEM ( )  RATIONAL_B_SPLINE_CURVE ( ( 1.000000000000009770, 0.8660254037844289376, 1.000000000000000000, 0.8660254037844387076, 1.000000000000000000, 0.8660254037844360431, 1.000000000000002665 ) ) 
 REPRESENTATION_ITEM ( '' )  );
#104456=CARTESIAN_POINT ( 'NONE',  ( -4.261005416444848315, 8.193199762486115034, 0.7998128361456352531 ) ) ;
#104457=CARTESIAN_POINT ( 'NONE',  ( -4.930325137224961907, 5.781076077297750970, -1.199719254218453823 ) ) ;
#104460=CARTESIAN_POINT ( 'NONE',  ( 5.926322542504858681, 8.007405281046052536, -1.443375672974078761 ) ) ;
#104472=CARTESIAN_POINT ( 'NONE',  ( -4.756313517479579644, 8.198030745052275137, 0.7332552394410801755 ) ) ;
#104476=CARTESIAN_POINT ( 'NONE',  ( 4.068855497876973537, 7.761098824249525130, -0.7216878364870338292 ) ) ;
#104481=CARTESIAN_POINT ( 'NONE',  ( -6.154475385960665790, 6.144919136567696505, 0.000000000000000000 ) ) ;
#104484=EDGE_CURVE ( 'NONE', #182295, #101986, #159148, .T. ) ;
#104495=CARTESIAN_POINT ( 'NONE',  ( 3.718679271898170491, 7.560485927181699317, 0.7998128361456271485 ) ) ;
#104521=EDGE_LOOP ( 'NONE', ( #117168, #148098, #15467, #65123 ) ) ;
#104531=CARTESIAN_POINT ( 'NONE',  ( 6.888951449519509218, 7.209733910627123876, -0.7216878364870317197 ) ) ;
#104536=CARTESIAN_POINT ( 'NONE',  ( 5.465345319640213972, 8.429967735338637524, -1.082531754730548412 ) ) ;
#104552=CARTESIAN_POINT ( 'NONE',  ( -7.553827861469316396, 8.841829255582865699, -1.199719254218452047 ) ) ;
#104564=CARTESIAN_POINT ( 'NONE',  ( 5.872089928050205465, 6.023395468912922546, -0.7216878364870458196 ) ) ;
#104570=CARTESIAN_POINT ( 'NONE',  ( -4.679499295372141709, 5.488445928469455559, 1.199719254218452935 ) ) ;
#104575=CARTESIAN_POINT ( 'NONE',  ( -5.289089323106922258, 9.184704953684462936, 0.7216878364870267237 ) ) ;
#104579=CARTESIAN_POINT ( 'NONE',  ( -5.562588163356775972, 9.711712967216715953, 0.7998128361456291469 ) ) ;
#104584=CARTESIAN_POINT ( 'NONE',  ( -4.309512724297390740, 6.121127159803966933, 1.599625672291270506 ) ) ;
#104598=CARTESIAN_POINT ( 'NONE',  ( -5.207740401424942434, 6.208690235484773723, 1.082531754730549078 ) ) ;
#104600=CARTESIAN_POINT ( 'NONE',  ( -3.811250578772981346, 6.500190537660166079, -1.082531754730546636 ) ) ;
#104601=CARTESIAN_POINT ( 'NONE',  ( 4.899292406491845497, 6.809203455697518947, -1.599625672291273171 ) ) ;
#104602=CARTESIAN_POINT ( 'NONE',  ( -6.089547271193396227, 7.133501900260939443, -1.199719254218453823 ) ) ;
#104603=CARTESIAN_POINT ( 'NONE',  ( -5.596483547390937119, 9.751257581923240991, 0.000000000000000000 ) ) ;
#104604=CARTESIAN_POINT ( 'NONE',  ( -6.638014823939186293, 6.741195553212168790, -0.1154932285401210346 ) ) ;
#104607=ADVANCED_FACE ( 'NONE', ( #174118 ), #185178, .T. ) ;
#104644=AXIS2_PLACEMENT_3D ( 'NONE', #191449, #139538, #43114 ) ;
#104660=CARTESIAN_POINT ( 'NONE',  ( 5.682802662783380754, 6.658966523782627434, 1.199719254218452935 ) ) ;
#104677=CARTESIAN_POINT ( 'NONE',  ( 5.564695703766185275, 5.456842840674144490, 0.000000000000000000 ) ) ;
#104683=CARTESIAN_POINT ( 'NONE',  ( -7.747558435566414659, 8.003516027774422170, -0.7998128361456362523 ) ) ;
#104688=CARTESIAN_POINT ( 'NONE',  ( 4.736594563127852098, 6.619389305106191834, -1.599625672291273171 ) ) ;
#104699=CARTESIAN_POINT ( 'NONE',  ( 6.373741612200162443, 8.529394195690610303, 1.443375672974065660 ) ) ;
#104700=CARTESIAN_POINT ( 'NONE',  ( -4.340018570150318666, 6.156717313299049366, -1.443375672974066548 ) ) ;
#104701=CARTESIAN_POINT ( 'NONE',  ( -6.394605727500880299, 7.489403432619674561, -1.199719254218452047 ) ) ;
#104712=ADVANCED_FACE ( 'NONE', ( #134188 ), #30216, .T. ) ;
#104715=CARTESIAN_POINT ( 'NONE',  ( 3.881377115262159894, 7.750300077773022878, 0.7998128361456271485 ) ) ;
#104716=CARTESIAN_POINT ( 'NONE',  ( 4.389807875774629942, 8.343469298370917997, 0.7998128361456271485 ) ) ;
#104722=ORIENTED_EDGE ( 'NONE', *, *, #100023, .T. ) ;
#104735=CARTESIAN_POINT ( 'NONE',  ( 5.011754246625688580, 8.023990808224052529, -1.135194352273690255 ) ) ;
#104744=CARTESIAN_POINT ( 'NONE',  ( 4.573896719763862251, 6.429575154514868274, -1.599625672291273171 ) ) ;
#104748=CARTESIAN_POINT ( 'NONE',  ( 5.996449078994045223, 10.21788403546024782, 0.7998128361456331437 ) ) ;
#104753=CARTESIAN_POINT ( 'NONE',  ( 6.549997609177859559, 6.814287763561861944, 0.000000000000000000 ) ) ;
#104755=CARTESIAN_POINT ( 'NONE',  ( -6.303615075710993665, 6.318915441276411471, -0.7998128361456362523 ) ) ;
#104757=CARTESIAN_POINT ( 'NONE',  ( 5.252858170651868441, 5.093032385374103299, -0.7998128361456481317 ) ) ;
#104758=ORIENTED_EDGE ( 'NONE', *, *, #169187, .F. ) ;
#104768=CARTESIAN_POINT ( 'NONE',  ( 6.357275476766607980, 6.835366726881293431, -0.6123070361637416026 ) ) ;
#104769=CARTESIAN_POINT ( 'NONE',  ( -6.780486220610184134, 9.003929572168926754, -1.443375672974066548 ) ) ;
#104779=CARTESIAN_POINT ( 'NONE',  ( -0.004779991008855831794, 3.496248221084442775, -2.003420919873224904 ) ) ;
#104793=DIRECTION ( 'NONE',  ( 0.7592566023653004592, -0.6507913734559639396, -0.000000000000000000 ) ) ;
#104806=CARTESIAN_POINT ( 'NONE',  ( 7.452141709366786770, 8.723195411463290583, 1.199719254218452047 ) ) ;
#104808=CARTESIAN_POINT ( 'NONE',  ( 6.851666526859736983, 9.086973262793417661, -1.599625672291269396 ) ) ;
#104822=CARTESIAN_POINT ( 'NONE',  ( -4.502189528189771472, 7.410248995266807803, -1.199719254218453823 ) ) ;
#104824=CARTESIAN_POINT ( 'NONE',  ( 5.031484404002867450, 8.884165881396448583, 0.7216878364870317197 ) ) ;
#104833=CARTESIAN_POINT ( 'NONE',  ( -3.959863383643135393, 6.777535159962392086, 1.199719254218452935 ) ) ;
#104836=CARTESIAN_POINT ( 'NONE',  ( -4.719646871332968452, 5.639247783710797712, 1.082531754730549078 ) ) ;
#104839=CARTESIAN_POINT ( 'NONE',  ( -3.688700311369816909, 6.461178242310183784, -1.199719254218450271 ) ) ;
#104863=CARTESIAN_POINT ( 'NONE',  ( -4.471156797456668386, 8.438376373666578445, -0.7998128361456362523 ) ) ;
#104865=CARTESIAN_POINT ( 'NONE',  ( -3.156015896931072540, 6.904045323053366268, 0.000000000000000000 ) ) ;
#104874=CARTESIAN_POINT ( 'NONE',  ( -6.204128743306504212, 7.035606015609114472, -1.046755002246579469 ) ) ;
#104877=ORIENTED_EDGE ( 'NONE', *, *, #191207, .T. ) ;
#104898=CARTESIAN_POINT ( 'NONE',  ( 6.983858524370772258, 9.241197259889668558, 1.443375672974063439 ) ) ;
#104910=CARTESIAN_POINT ( 'NONE',  ( 3.386504508363381571, 7.172948703057747011, -0.7998128361456362523 ) ) ;
#104918=CARTESIAN_POINT ( 'NONE',  ( 7.035755370848908896, 7.173079118937375931, 0.7998128361456352531 ) ) ;
#104920=CARTESIAN_POINT ( 'NONE',  ( 6.527324610336440180, 6.579909898339485252, 0.7998128361456331437 ) ) ;
#104933=CARTESIAN_POINT ( 'NONE',  ( 6.330867959801246059, 6.852818249511213544, -0.6651261847785728820 ) ) ;
#104936=CARTESIAN_POINT ( 'NONE',  ( 4.258669648468268676, 7.982548666606070320, 0.7216878364870257245 ) ) ;
#104938=( BOUNDED_CURVE ( )  B_SPLINE_CURVE ( 2, ( #39968, #126616, #142822, #207771, #172098 ),
 .UNSPECIFIED., .F., .T. ) 
 B_SPLINE_CURVE_WITH_KNOTS ( ( 3, 2, 3 ),
 ( 0.2230065254996309865, 0.2250000000000000056, 0.2273705207416776009 ),
 .UNSPECIFIED. ) 
 CURVE ( )  GEOMETRIC_REPRESENTATION_ITEM ( )  RATIONAL_B_SPLINE_CURVE ( ( 0.9512353381494595972, 0.9679510070496450957, 1.000000000000000000, 0.9618892528975757639, 0.9454606617520617817 ) ) 
 REPRESENTATION_ITEM ( '' )  );
#104944=CARTESIAN_POINT ( 'NONE',  ( 2.969872605471105320, 6.605953636083950364, 7.500000000000000000 ) ) ;
#104955=CARTESIAN_POINT ( 'NONE',  ( -4.950135482320926705, 6.868520377498098739, -1.443375672974066548 ) ) ;
#104960=CARTESIAN_POINT ( 'NONE',  ( 7.042534447655770080, 7.180988041878682004, -0.7998128361456341429 ) ) ;
#104993=CARTESIAN_POINT ( 'NONE',  ( 4.760321332173959696, 4.726332107057286791, 0.000000000000000000 ) ) ;
#105016=CARTESIAN_POINT ( 'NONE',  ( 5.099275172515607579, 5.121778254122544283, -0.7216878364870458196 ) ) ;
#105029=CARTESIAN_POINT ( 'NONE',  ( -4.584065335196305213, 6.441438539186039591, 1.443375672974058777 ) ) ;
#105034=CARTESIAN_POINT ( 'NONE',  ( 4.744428268735178200, 8.268600469562487731, 0.7448146739494916346 ) ) ;
#105040=CARTESIAN_POINT ( 'NONE',  ( -5.010594053901753497, 4.810390915832282843, -0.2947457133052544531 ) ) ;
#105053=CARTESIAN_POINT ( 'NONE',  ( 5.671053392266061977, 9.838255734277600695, 0.7998128361456331437 ) ) ;
#105063=CARTESIAN_POINT ( 'NONE',  ( 5.560252395380198998, 9.501061871336672127, 0.7216878364870317197 ) ) ;
#105075=CARTESIAN_POINT ( 'NONE',  ( -6.305950844131887223, 6.529566537674873494, 0.000000000000000000 ) ) ;
#105078=CARTESIAN_POINT ( 'NONE',  ( 5.905458427204159477, 9.047396044116986502, 1.199719254218452047 ) ) ;
#105083=CARTESIAN_POINT ( 'NONE',  ( -5.655686355556086120, 6.627330832017406692, 1.199719254218452935 ) ) ;
#105084=FACE_OUTER_BOUND ( 'NONE', #5300, .T. ) ;
#105096=CARTESIAN_POINT ( 'NONE',  ( 3.876876046179563051, 7.339504906929419370, -0.7537628779380199928 ) ) ;
#105122=CARTESIAN_POINT ( 'NONE',  ( 4.665414256878284149, 6.536345614481700927, -1.443375672974068769 ) ) ;
#105126=CARTESIAN_POINT ( 'NONE',  ( -6.791708605802965870, 6.888357893050385705, -0.7998128361456362523 ) ) ;
#105130=CARTESIAN_POINT ( 'NONE',  ( -4.776215253764153346, 8.794277906025310898, -0.7998128361456362523 ) ) ;
#105131=CARTESIAN_POINT ( 'NONE',  ( -5.829079699232685208, 5.765290835385048496, 0.000000000000000000 ) ) ;
#105135=CARTESIAN_POINT ( 'NONE',  ( -6.983858524370814003, 9.241197259889665006, 1.443375672974064550 ) ) ;
#105142=CARTESIAN_POINT ( 'NONE',  ( -5.725286006720766707, 9.901527117808042178, 0.7998128361456291469 ) ) ;
#105149=CARTESIAN_POINT ( 'NONE',  ( -6.282224075085783177, 8.422623735723785643, 1.599625672291269396 ) ) ;
#105151=CARTESIAN_POINT ( 'NONE',  ( 5.880365472892705725, 7.167286867907723291, -1.140585135024022811 ) ) ;
#105157=CARTESIAN_POINT ( 'NONE',  ( 4.573896719763862251, 6.429575154514868274, -1.599625672291273171 ) ) ;
#105166=CARTESIAN_POINT ( 'NONE',  ( -5.901542003698421190, 10.10715911428198055, 0.000000000000000000 ) ) ;
#105170=ORIENTED_EDGE ( 'NONE', *, *, #63569, .F. ) ;
#105181=CARTESIAN_POINT ( 'NONE',  ( 5.993586425693011144, 9.150212042353954800, -1.199719254218452047 ) ) ;
#105194=CARTESIAN_POINT ( 'NONE',  ( 5.966021608595377224, 7.209656400309186530, 1.216315744458285719 ) ) ;
#105220=CARTESIAN_POINT ( 'NONE',  ( -6.419388467533182485, 6.810688026658763938, -0.4840902626340077841 ) ) ;
#105240=CARTESIAN_POINT ( 'NONE',  ( -4.945692173934974178, 8.992000979557944973, 0.000000000000000000 ) ) ;
#105257=CARTESIAN_POINT ( 'NONE',  ( 3.790386463472274148, 6.579812086429759788, 1.199719254218452047 ) ) ;
#105259=CARTESIAN_POINT ( 'NONE',  ( 6.170369307550806148, 10.21286493553572328, 0.7216878364870317197 ) ) ;
#105260=CARTESIAN_POINT ( 'NONE',  ( 5.098048262872540981, 4.912420826298216525, -0.06541299864657826313 ) ) ;
#105276=CARTESIAN_POINT ( 'NONE',  ( 6.852720297064418986, 6.959538199522133262, 0.7998128361456331437 ) ) ;
#105287=CARTESIAN_POINT ( 'NONE',  ( -5.167592825464113915, 6.057888380243431570, 1.199719254218452935 ) ) ;
#105289=CARTESIAN_POINT ( 'NONE',  ( 3.223806664999388172, 6.983134552466421674, -0.7998128361456362523 ) ) ;
#105293=CARTESIAN_POINT ( 'NONE',  ( -6.099189001301292379, 8.209082816308541197, 1.599625672291263179 ) ) ;
#105296=CARTESIAN_POINT ( 'NONE',  ( 4.877901405866606588, 8.912911750144889567, 0.7998128361456341429 ) ) ;
#105301=CARTESIAN_POINT ( 'NONE',  ( -4.702355942707336034, 8.355867970554191615, 0.6817663069898479700 ) ) ;
#105311=CARTESIAN_POINT ( 'NONE',  ( -3.960390268523300339, 7.634556056670224855, 1.214306433183764966E-14 ) ) ;
#105313=AXIS2_PLACEMENT_3D ( 'NONE', #128132, #162686, #123074 ) ;
#105322=CARTESIAN_POINT ( 'NONE',  ( 4.421367491832270957, 6.251624388594711590, 1.443375672974058777 ) ) ;
#105325=CARTESIAN_POINT ( 'NONE',  ( 5.026762865062591068, 4.898582544318342613, 0.2131414487870288976 ) ) ;
#105326=CARTESIAN_POINT ( 'NONE',  ( -7.286581212701773502, 7.465709267765667789, 0.7998128361456341429 ) ) ;
#105328=VERTEX_POINT ( 'NONE', #104993 ) ;
#105340=CARTESIAN_POINT ( 'NONE',  ( 4.947799714344386146, 4.737130853015369958, -0.7998128361456481317 ) ) ;
#105345=CARTESIAN_POINT ( 'NONE',  ( 5.387385936583817703, 7.378645907471495846, -1.599625672291283607 ) ) ;
#105361=EDGE_CURVE ( 'NONE', #86356, #199688, #138553, .T. ) ;
#105369=CARTESIAN_POINT ( 'NONE',  ( -5.207740401424942434, 6.208690235484773723, 1.082531754730549078 ) ) ;
#105392=ORIENTED_EDGE ( 'NONE', *, *, #41220, .F. ) ;
#105393=CARTESIAN_POINT ( 'NONE',  ( -3.146901051703345331, 6.685485303713597283, 0.000000000000000000 ) ) ;
#105401=CARTESIAN_POINT ( 'NONE',  ( -4.339491684825780737, 7.220434844675483355, -1.199719254218455378 ) ) ;
#105404=DIRECTION ( 'NONE',  ( 0.000000000000000000, 0.000000000000000000, -1.000000000000000000 ) ) ;
#105406=EDGE_LOOP ( 'NONE', ( #81806, #110666, #27893, #55850, #92496 ) ) ;
#105410=CARTESIAN_POINT ( 'NONE',  ( -5.178288325776719603, 5.006034233019745372, 0.000000000000000000 ) ) ;
#105412=CARTESIAN_POINT ( 'NONE',  ( 6.606590233575550641, 6.765807905838774339, 0.03828827652692379235 ) ) ;
#105416=CARTESIAN_POINT ( 'NONE',  ( 3.393283585170187688, 7.180857625999046867, 0.7998128361456271485 ) ) ;
#105421=CARTESIAN_POINT ( 'NONE',  ( -5.912237504011027767, 9.055304967058290799, 1.199719254218454489 ) ) ;
#105426=CARTESIAN_POINT ( 'NONE',  ( -2.810282979782591006, 6.500690253046801814, 0.000000000000000000 ) ) ;
#105432=CARTESIAN_POINT ( 'NONE',  ( 4.706088717274906408, 5.623429937309770921, 1.082531754730549078 ) ) ;
#105433=CARTESIAN_POINT ( 'NONE',  ( -5.194182247366913252, 7.153241603385088965, 1.443375672974058777 ) ) ;
#105440=CARTESIAN_POINT ( 'NONE',  ( 5.228604516725597229, 6.129068686715179126, -1.199719254218450271 ) ) ;
#105446=CARTESIAN_POINT ( 'NONE',  ( 5.890091390494168522, 5.836471141856793388, 0.000000000000000000 ) ) ;
#105451=CARTESIAN_POINT ( 'NONE',  ( 5.098657496608274720, 7.938328561423579011, 1.202842226815619142 ) ) ;
#105462=CARTESIAN_POINT ( 'NONE',  ( 6.737475991348287785, 6.825086509519945999, -0.7998128361456481317 ) ) ;
#105472=CARTESIAN_POINT ( 'NONE',  ( 6.059270238282111087, 7.038290852966752276, 1.014332888565868229 ) ) ;
#105488=CARTESIAN_POINT ( 'NONE',  ( -5.433785704026946384, 9.561443431331920095, 0.000000000000000000 ) ) ;
#105495=CARTESIAN_POINT ( 'NONE',  ( -3.895996091634230218, 7.334980739573080832, 0.5863762202383783206 ) ) ;
#105502=CARTESIAN_POINT ( 'NONE',  ( 6.008198349511364000, 7.038594824965278995, 1.199719254218453823 ) ) ;
#105512=CARTESIAN_POINT ( 'NONE',  ( 4.624739795592929248, 6.488892076315451618, -1.443375672974068769 ) ) ;
#105513=DIRECTION ( 'NONE',  ( -1.776356839400250465E-15, 0.000000000000000000, 1.000000000000000000 ) ) ;
#105518=FACE_OUTER_BOUND ( 'NONE', #28433, .T. ) ;
#105525=CARTESIAN_POINT ( 'NONE',  ( -7.919371124158132602, 8.411890197705517380, -0.7216878364870338292 ) ) ;
#105526=CARTESIAN_POINT ( 'NONE',  ( 5.804299160426222848, 7.865044668620976509, -1.443375672974078761 ) ) ;
#105536=CARTESIAN_POINT ( 'NONE',  ( -4.773352600463090845, 7.726605912919016106, 1.199719254218452935 ) ) ;
#105537=CARTESIAN_POINT ( 'NONE',  ( -5.469788628470539926, 5.346117919495872783, -0.7998128361456362523 ) ) ;
#105540=CARTESIAN_POINT ( 'NONE',  ( 6.848276988234151652, 7.162280372460873679, -0.7216878364870317197 ) ) ;
#105550=DIRECTION ( 'NONE',  ( -0.000000000000000000, -1.000000000000000000, -0.000000000000000000 ) ) ;
#105553=CARTESIAN_POINT ( 'NONE',  ( -4.652699544748355898, 8.322425126176462129, -0.4365168051920116365 ) ) ;
#105558=CARTESIAN_POINT ( 'NONE',  ( 5.411112705629925301, 5.485588709422586362, 0.000000000000000000 ) ) ;
#105561=LINE ( 'NONE', #171594, #207503 ) ;
#105562=CARTESIAN_POINT ( 'NONE',  ( -4.932134020321308654, 8.976183133675331050, 0.7998128361456291469 ) ) ;
#105577=CARTESIAN_POINT ( 'NONE',  ( 6.364626766972446781, 6.390095747748157251, 0.7998128361456352531 ) ) ;
#105615=CARTESIAN_POINT ( 'NONE',  ( 6.861835142292143530, 8.138467433163244280, 1.082531754730549967 ) ) ;
#105622=CARTESIAN_POINT ( 'NONE',  ( 5.994113310573177422, 10.00723293906178846, 0.000000000000000000 ) ) ;
#105631=EDGE_CURVE ( 'NONE', #198620, #22926, #193069, .T. ) ;
#105645=PRODUCT_CONTEXT ( 'NONE', #212288, 'mechanical' ) ;
#105650=CARTESIAN_POINT ( 'NONE',  ( 3.553645660113312399, 7.160020680191912845, -1.734723475976807094E-15 ) ) ;
#105656=CARTESIAN_POINT ( 'NONE',  ( -5.029148636026397945, 4.832037928311032182, 0.7998128361456281477 ) ) ;
#105660=EDGE_CURVE ( 'NONE', #36910, #41289, #146989, .T. ) ;
#105662=CARTESIAN_POINT ( 'NONE',  ( -7.295696057929500711, 7.684269287105433222, 0.7216878364870317197 ) ) ;
#105664=CARTESIAN_POINT ( 'NONE',  ( -6.391719935120312890, 6.567462711928212293, 2.438448603877958032 ) ) ;
#105665=CARTESIAN_POINT ( 'NONE',  ( -6.563028877466991595, 9.814561569423593923, 1.199719254218452935 ) ) ;
#105670=CARTESIAN_POINT ( 'NONE',  ( -4.176793841461789114, 7.030620694084159794, -1.199719254218455378 ) ) ;
#105678=CARTESIAN_POINT ( 'NONE',  ( -3.752568318859959007, 7.355240624044412812, 0.6449737300090957470 ) ) ;
#105684=CARTESIAN_POINT ( 'NONE',  ( -5.478903473698260029, 6.525047153136981137, -1.082531754730549967 ) ) ;
#105686=VERTEX_POINT ( 'NONE', #29055 ) ;
#105687=CARTESIAN_POINT ( 'NONE',  ( -4.380693030546956912, 6.204170850428461392, 1.443375672974065660 ) ) ;
#105688=CARTESIAN_POINT ( 'NONE',  ( 4.549643065837591038, 7.465611455855944101, -1.199719254218452047 ) ) ;
#105689=CARTESIAN_POINT ( 'NONE',  ( -5.550083779947821760, 7.568460058062819407, -1.599625672291271394 ) ) ;
#105690=CARTESIAN_POINT ( 'NONE',  ( -5.121948170912633991, 9.197632976031879792, -0.7998128361456362523 ) ) ;
#105692=EDGE_CURVE ( 'NONE', #154238, #157478, #118629, .T. ) ;
#105710=CARTESIAN_POINT ( 'NONE',  ( 6.393551957296131683, 9.616838495890963401, 1.199719254218452047 ) ) ;
#105715=CARTESIAN_POINT ( 'NONE',  ( -5.823017895876262173, 7.308274721394978357, -1.333157625313810879 ) ) ;
#105733=CARTESIAN_POINT ( 'NONE',  ( 6.313256805818848960, 7.394496357324014113, 1.199719254218452047 ) ) ;
#105735=DIRECTION ( 'NONE',  ( 0.000000000000000000, 0.000000000000000000, 1.000000000000000000 ) ) ;
#105742=CARTESIAN_POINT ( 'NONE',  ( -1.879585681373379114, 8.984805382992709255, -0.7749999999999996891 ) ) ;
#105751=CARTESIAN_POINT ( 'NONE',  ( 5.688757509019037428, 5.629766575900002401, 2.420000000000000373 ) ) ;
#105752=CARTESIAN_POINT ( 'NONE',  ( 6.062430963966053632, 7.101866208495718702, -1.199719254218452047 ) ) ;
#105759=EDGE_CURVE ( 'NONE', #123208, #105686, #105987, .T. ) ;
#105768=CARTESIAN_POINT ( 'NONE',  ( 4.450808633097238953, 7.987047222781201938, 2.500000000000000000 ) ) ;
#105771=CARTESIAN_POINT ( 'NONE',  ( 5.391302360089590628, 6.318882837306503575, -1.199719254218452047 ) ) ;
#105777=VERTEX_POINT ( 'NONE', #134054 ) ;
#105779=CARTESIAN_POINT ( 'NONE',  ( -6.668631453075260396, 8.873432343378178544, -1.599625672291271394 ) ) ;
#105784=CARTESIAN_POINT ( 'NONE',  ( 5.306037014901791693, 7.283738832175834510, 1.599625672291269396 ) ) ;
#105790=TOROIDAL_SURFACE ( 'NONE', #81157, 2.080000000000000071, 0.08000000000000000167 ) ;
#105791=DIRECTION ( 'NONE',  ( 0.000000000000000000, -1.000000000000000000, 0.000000000000000000 ) ) ;
#105797=CARTESIAN_POINT ( 'NONE',  ( 5.722950238744187956, 9.690876021928001904, 0.7216878364870317197 ) ) ;
#105798=CARTESIAN_POINT ( 'NONE',  ( -4.925354943514475003, 8.968274210734028529, 0.000000000000000000 ) ) ;
#105809=CARTESIAN_POINT ( 'NONE',  ( 4.854701522145073334, 7.821512988214679218, -1.199719254218450271 ) ) ;
#105810=CARTESIAN_POINT ( 'NONE',  ( 5.737035277238070385, 6.722237907313067140, -1.199719254218452047 ) ) ;
#105813=CARTESIAN_POINT ( 'NONE',  ( 7.198453214212898743, 7.362893269528701268, 0.7998128361456291469 ) ) ;
#105827=CARTESIAN_POINT ( 'NONE',  ( 5.364607279338250656, 7.693244595681929532, -1.319704323257679057 ) ) ;
#105831=CARTESIAN_POINT ( 'NONE',  ( 5.086243903782109221, 5.962981304947771122, -1.199719254218452047 ) ) ;
#105835=CARTESIAN_POINT ( 'NONE',  ( 3.386504508363381571, 7.172948703057747011, -0.7998128361456362523 ) ) ;
#105840=CARTESIAN_POINT ( 'NONE',  ( 7.075376061485196821, 9.347967719856493218, 1.599625672291268286 ) ) ;
#105845=CARTESIAN_POINT ( 'NONE',  ( 6.048345925472183637, 8.149765894507963182, 1.443375672974065660 ) ) ;
#105848=CARTESIAN_POINT ( 'NONE',  ( -4.782994330570982555, 8.802186828966616972, 0.000000000000000000 ) ) ;
#105850=CARTESIAN_POINT ( 'NONE',  ( 4.309512724297349884, 6.121127159803966933, 1.599625672291261402 ) ) ;
#105862=CARTESIAN_POINT ( 'NONE',  ( -5.144392941742557568, 4.966489618313220333, -0.7998128361456362523 ) ) ;
#105871=CARTESIAN_POINT ( 'NONE',  ( -5.436182321379713578, 6.108390213082993903, 1.083092214668917919 ) ) ;
#105872=CARTESIAN_POINT ( 'NONE',  ( 0.2075773638182398517, 2.642062557107526022, -2.068677247530675611 ) ) ;
#105891=AXIS2_PLACEMENT_3D ( 'NONE', #39309, #6782, #105404 ) ;
#105902=CARTESIAN_POINT ( 'NONE',  ( 5.356880090730874677, 5.422317325373725794, 0.7216878364870328300 ) ) ;
#105916=CARTESIAN_POINT ( 'NONE',  ( -5.906512197408906317, 6.919960980845699439, -1.199719254218453823 ) ) ;
#105918=CARTESIAN_POINT ( 'NONE',  ( 6.848276988234151652, 7.162280372460873679, -0.7216878364870317197 ) ) ;
#105930=CARTESIAN_POINT ( 'NONE',  ( -5.743814354044916470, 6.730146830254374990, -1.199719254218453823 ) ) ;
#105938=CARTESIAN_POINT ( 'NONE',  ( -4.122561227007127016, 6.967349310553715647, 1.199719254218452935 ) ) ;
#105939=VERTEX_POINT ( 'NONE', #182751 ) ;
#105947=CARTESIAN_POINT ( 'NONE',  ( 0.3999999999999719891, 3.096232863981052574, 2.023857702508392364 ) ) ;
#105962=ADVANCED_FACE ( 'NONE', ( #68987 ), #179178, .T. ) ;
#105965=CARTESIAN_POINT ( 'NONE',  ( -4.685224601974262271, 7.623789914682047808, -1.199719254218453823 ) ) ;
#105967=CARTESIAN_POINT ( 'NONE',  ( -4.516801452008150086, 5.298631777878131111, 1.199719254218452935 ) ) ;
#105977=DIRECTION ( 'NONE',  ( 0.6507913734559641616, -0.7592566023653004592, 0.000000000000000000 ) ) ;
#105987=B_SPLINE_CURVE_WITH_KNOTS ( 'NONE', 3,
 ( #770, #118895, #98318, #115683 ),
 .UNSPECIFIED., .F., .F.,
 ( 4, 4 ),
 ( 0.0006145506151576765911, 0.0009333549826883593510 ),
 .UNSPECIFIED. ) ;
#105993=CARTESIAN_POINT ( 'NONE',  ( -5.306037014901836990, 7.283738832175834510, 1.599625672291263179 ) ) ;
#106012=CARTESIAN_POINT ( 'NONE',  ( 4.923546060418115822, 5.773167154356443120, -1.199719254218452047 ) ) ;
#106021=CARTESIAN_POINT ( 'NONE',  ( 6.387826650694035990, 7.481494509678370264, -1.199719254218452047 ) ) ;
#106023=CARTESIAN_POINT ( 'NONE',  ( 6.017840079619279692, 8.114175741012878973, -1.599625672291281386 ) ) ;
#106035=CARTESIAN_POINT ( 'NONE',  ( 6.455362170788604637, 6.771378801287749383, -0.3290997004737963860 ) ) ;
#106037=CARTESIAN_POINT ( 'NONE',  ( 6.075462232699553766, 6.260663157670496304, -0.7216878364870458196 ) ) ;
#106054=CARTESIAN_POINT ( 'NONE',  ( -4.462041952228944730, 7.259447140025469203, -1.082531754730549967 ) ) ;
#106059=CARTESIAN_POINT ( 'NONE',  ( 8.018721507839716267, 8.319872945426633137, -0.7998128361456341429 ) ) ;
#106060=CARTESIAN_POINT ( 'NONE',  ( 5.094532678321557206, 4.917790403868676385, -0.1305349544365452807 ) ) ;
#106077=CARTESIAN_POINT ( 'NONE',  ( 5.397027666691686321, 8.454226823519094935, 1.199719254218451159 ) ) ;
#106118=CARTESIAN_POINT ( 'NONE',  ( 4.421367491832270957, 6.251624388594711590, 1.443375672974058777 ) ) ;
#106123=CARTESIAN_POINT ( 'NONE',  ( -5.935437387732586778, 10.14670372898850381, -0.7998128361456362523 ) ) ;
#106129=CARTESIAN_POINT ( 'NONE',  ( -3.838366886444665393, 7.492195444245147939, 0.000000000000000000 ) ) ;
#106134=CARTESIAN_POINT ( 'NONE',  ( 4.674199705399083804, 8.286630605821020623, 0.5482284608372268719 ) ) ;
#106139=FACE_OUTER_BOUND ( 'NONE', #117087, .T. ) ;
#106145=CARTESIAN_POINT ( 'NONE',  ( -3.836074819041962236, 7.488154855499102425, 0.1510019874590182165 ) ) ;
#106159=CARTESIAN_POINT ( 'NONE',  ( 3.553118775233146120, 6.302999783484076524, -1.199719254218453823 ) ) ;
#106172=CARTESIAN_POINT ( 'NONE',  ( -6.956742217587851052, 7.288823140040177506, 0.000000000000000000 ) ) ;
#106175=CARTESIAN_POINT ( 'NONE',  ( 7.526711554241970248, 8.810193563817646734, -1.199719254218452047 ) ) ;
#106223=CARTESIAN_POINT ( 'NONE',  ( -5.745623237141265882, 9.925253886631958622, 0.7998128361456291469 ) ) ;
#106226=CARTESIAN_POINT ( 'NONE',  ( -5.264308783856126439, 9.363720357799287797, -0.7998128361456362523 ) ) ;
#106227=CARTESIAN_POINT ( 'NONE',  ( -4.294900800479008574, 8.232744377192641849, 0.000000000000000000 ) ) ;
#106231=CARTESIAN_POINT ( 'NONE',  ( -6.902509602688821744, 8.185920970292658083, -1.082531754730549967 ) ) ;
#106238=CARTESIAN_POINT ( 'NONE',  ( -4.167152111353897403, 5.955039778036558040, 1.599625672291270506 ) ) ;
#106242=EDGE_LOOP ( 'NONE', ( #119, #70517, #113826, #13675 ) ) ;
#106247=CARTESIAN_POINT ( 'NONE',  ( -6.794571259104023930, 7.956029886156682274, 1.199719254218452047 ) ) ;
#106248=ORIENTED_EDGE ( 'NONE', *, *, #173321, .T. ) ;
#106249=CARTESIAN_POINT ( 'NONE',  ( 5.258270873920524835, 7.671714958958308017, -1.216365610458163715 ) ) ;
#106252=CARTESIAN_POINT ( 'NONE',  ( 4.475125623951746512, 4.983947107165113799, -0.9081682986131468516 ) ) ;
#106254=CARTESIAN_POINT ( 'NONE',  ( 5.096939404094710468, 4.911127157724081371, 0.000000000000000000 ) ) ;
#106260=CARTESIAN_POINT ( 'NONE',  ( -2.428612866367529932E-14, 8.999999999999998224, 0.7749999999999996891 ) ) ;
#106262=EDGE_CURVE ( 'NONE', #13123, #28052, #93953, .T. ) ;
#106265=CARTESIAN_POINT ( 'NONE',  ( -6.563028877466991595, 9.814561569423593923, 1.199719254218452935 ) ) ;
#106278=CARTESIAN_POINT ( 'NONE',  ( 6.912678218121202534, 9.158153569265168770, 1.599625672291268286 ) ) ;
#106287=CARTESIAN_POINT ( 'NONE',  ( 3.147653791585713901, 8.920000000000001705, -2.420000000000002149 ) ) ;
#106293=CARTESIAN_POINT ( 'NONE',  ( 6.344829475870412239, 6.940264737885684987, 0.8615092103797560297 ) ) ;
#106294=CARTESIAN_POINT ( 'NONE',  ( -5.289089322662584358, 5.343228095960675716, 0.000000000000000000 ) ) ;
#106305=ORIENTED_EDGE ( 'NONE', *, *, #67920, .F. ) ;
#106319=CARTESIAN_POINT ( 'NONE',  ( 5.388439706788500594, 5.251210844200210559, 0.7998128361456352531 ) ) ;
#106335=CARTESIAN_POINT ( 'NONE',  ( 3.562078172017826727, 7.339166372451206399, -0.2626806445317174665 ) ) ;
#106339=CARTESIAN_POINT ( 'NONE',  ( -7.293360289508603600, 7.473618190706972086, 0.000000000000000000 ) ) ;
#106356=CARTESIAN_POINT ( 'NONE',  ( 3.413620815590684199, 7.204584394822967752, 0.7998128361456281477 ) ) ;
#106358=CARTESIAN_POINT ( 'NONE',  ( 7.146556367734771875, 8.470642196179646533, 1.082531754730549967 ) ) ;
#106365=CARTESIAN_POINT ( 'NONE',  ( 4.663288057535367237, 8.288536188413402783, 0.5084364831346009916 ) ) ;
#106368=CARTESIAN_POINT ( 'NONE',  ( 4.876420697298537554, 8.045338245374718866, 0.9427337716215690167 ) ) ;
#106370=CARTESIAN_POINT ( 'NONE',  ( -3.666689614532284924, 7.355176389186829589, 0.3694189123316319878 ) ) ;
#106385=CARTESIAN_POINT ( 'NONE',  ( -5.503684012504701961, 5.385662534202396934, 0.000000000000000000 ) ) ;
#106387=CARTESIAN_POINT ( 'NONE',  ( 6.059568310664962709, 6.034194215389424798, 0.7998128361456352531 ) ) ;
#106389=CARTESIAN_POINT ( 'NONE',  ( -3.231779075379147770, 6.036511184309971689, 7.500000000000000000 ) ) ;
#106390=CARTESIAN_POINT ( 'NONE',  ( -5.261446130555064826, 8.296048364692991228, 1.199719254218452935 ) ) ;
#106393=CARTESIAN_POINT ( 'NONE',  ( 6.068156270568149324, 9.237210194708310951, 1.199719254218452047 ) ) ;
#106398=CARTESIAN_POINT ( 'NONE',  ( -4.973494386576447823, 8.059877448926631160, 1.114414082037382236 ) ) ;
#106409=CARTESIAN_POINT ( 'NONE',  ( -4.123088111887291518, 7.824370207261548416, 0.000000000000000000 ) ) ;
#106419=CARTESIAN_POINT ( 'NONE',  ( 5.289089323106923146, 6.303597310780433283, -1.082531754730548412 ) ) ;
#106423=CARTESIAN_POINT ( 'NONE',  ( -6.668631453075260396, 8.873432343378178544, -1.599625672291271394 ) ) ;
#106437=CARTESIAN_POINT ( 'NONE',  ( 5.096939404094710468, 4.911127157724081371, 0.000000000000000000 ) ) ;
#106442=CARTESIAN_POINT ( 'NONE',  ( -4.864214080903581205, 4.879786425613829692, -0.6392378712632117432 ) ) ;
#106463=CARTESIAN_POINT ( 'NONE',  ( -6.021229618244897885, 7.157760988441397743, 1.082531754730548412 ) ) ;
#106487=CARTESIAN_POINT ( 'NONE',  ( -4.462041952228957165, 5.338708711422782471, -1.082531754730549967 ) ) ;
#106488=EDGE_CURVE ( 'NONE', #101986, #22926, #26997, .T. ) ;
#106494=CARTESIAN_POINT ( 'NONE',  ( -4.014095998097799267, 6.840806543492835345, -1.199719254218450271 ) ) ;
#106497=CARTESIAN_POINT ( 'NONE',  ( 4.909461021924240498, 7.781436054670031410, 1.082531754730549078 ) ) ;
#106502=CARTESIAN_POINT ( 'NONE',  ( -8.086512275908061653, 8.398962174839683215, 0.000000000000000000 ) ) ;
#106504=CARTESIAN_POINT ( 'NONE',  ( 5.943507298343291723, 7.226397084328657350, -1.228854570503196575 ) ) ;
#106508=CARTESIAN_POINT ( 'NONE',  ( 6.201928923608456046, 6.200281597156833691, 0.7998128361456352531 ) ) ;
#106513=CARTESIAN_POINT ( 'NONE',  ( -5.088052786878465739, 9.158088361325352977, 0.000000000000000000 ) ) ;
#106517=CARTESIAN_POINT ( 'NONE',  ( -5.646044625448194410, 5.551749915969804938, 0.000000000000000000 ) ) ;
#106522=CARTESIAN_POINT ( 'NONE',  ( 6.346625304528514810, 6.577020074804287297, 0.000000000000000000 ) ) ;
#106523=CARTESIAN_POINT ( 'NONE',  ( -5.763624699140883934, 6.857221916153382502, -1.082531754730549967 ) ) ;
#106527=CARTESIAN_POINT ( 'NONE',  ( -3.800028193580205826, 7.655393002477361541, -0.7998128361456481317 ) ) ;
#106530=CARTESIAN_POINT ( 'NONE',  ( 4.523580528814945545, 5.306540700819438960, 1.199719254218452047 ) ) ;
#106537=DIRECTION ( 'NONE',  ( 0.000000000000000000, 1.000000000000000000, 0.000000000000000000 ) ) ;
#106542=CARTESIAN_POINT ( 'NONE',  ( 4.895464504754282409, 8.144056917144915531, 1.010406422583273178 ) ) ;
#106551=CARTESIAN_POINT ( 'NONE',  ( 5.254667053748194760, 8.288139441751686931, 1.199719254218452047 ) ) ;
#106563=CARTESIAN_POINT ( 'NONE',  ( 6.465908158583062892, 6.764574590967027845, 0.2795716154820517829 ) ) ;
#106581=CARTESIAN_POINT ( 'NONE',  ( -6.095272577795516789, 9.268845886473535245, 1.199719254218452047 ) ) ;
#106584=FACE_OUTER_BOUND ( 'NONE', #25579, .T. ) ;
#106595=CARTESIAN_POINT ( 'NONE',  ( 6.038177310039780643, 8.137902509836795417, -1.599625672291283607 ) ) ;
#106599=CARTESIAN_POINT ( 'NONE',  ( 4.663288057535368125, 8.288536188413402783, 0.5084364831346009916 ) ) ;
#106603=CARTESIAN_POINT ( 'NONE',  ( 4.686278372178935392, 5.496354851410763409, 1.199719254218452047 ) ) ;
#106606=EDGE_CURVE ( 'NONE', #51151, #134523, #85200, .T. ) ;
#106607=CARTESIAN_POINT ( 'NONE',  ( 3.865483193227626124, 7.523831135491951372, -0.7216878364870338292 ) ) ;
#106620=CARTESIAN_POINT ( 'NONE',  ( -2.810282979782591006, 6.500690253046801814, 0.000000000000000000 ) ) ;
#106622=CARTESIAN_POINT ( 'NONE',  ( 8.000720045840086669, 8.506797273001177828, 0.7216878364870267237 ) ) ;
#106633=CARTESIAN_POINT ( 'NONE',  ( -4.664887371553763096, 7.600063145858131364, -1.199719254218453823 ) ) ;
#106634=CARTESIAN_POINT ( 'NONE',  ( -5.472651281771599763, 6.413789912602166687, 1.199719254218452935 ) ) ;
#106636=CARTESIAN_POINT ( 'NONE',  ( 5.356880090730850696, 9.263794182579101033, 0.7216878364870317197 ) ) ;
#106643=CARTESIAN_POINT ( 'NONE',  ( -4.596923820214036560, 8.483565078729160547, 0.2266403168418751335 ) ) ;
#106648=CARTESIAN_POINT ( 'NONE',  ( -4.603881723180708541, 8.384271979250147666, 0.04571010684512218092 ) ) ;
#106652=CARTESIAN_POINT ( 'NONE',  ( 3.757017964762656703, 7.397288368949487491, -1.734723475976807094E-15 ) ) ;
#106657=CARTESIAN_POINT ( 'NONE',  ( -5.769876891067536206, 8.889217585290882795, 1.199719254218454489 ) ) ;
#106663=B_SPLINE_CURVE_WITH_KNOTS ( 'NONE', 3,
 ( #18989, #69858, #120857, #22168, #85071, #185753, #38461 ),
 .UNSPECIFIED., .F., .F.,
 ( 4, 3, 4 ),
 ( 0.000000000000000000, 2.757963454290271384E-05, 5.739065715766676189E-05 ),
 .UNSPECIFIED. ) ;
#106673=CARTESIAN_POINT ( 'NONE',  ( 6.215487077222150880, 6.216099443039444949, 0.000000000000000000 ) ) ;
#106683=CARTESIAN_POINT ( 'NONE',  ( 6.021229617800532452, 6.197391773621639288, 0.000000000000000000 ) ) ;
#106699=ORIENTED_EDGE ( 'NONE', *, *, #38876, .F. ) ;
#106709=CARTESIAN_POINT ( 'NONE',  ( 5.234856708652215751, 9.121433570154021453, 0.7216878364870317197 ) ) ;
#106714=CARTESIAN_POINT ( 'NONE',  ( 6.821160681006781523, 9.051383109298340557, 1.443375672974063439 ) ) ;
#106738=CARTESIAN_POINT ( 'NONE',  ( -5.113360211009450040, 5.994616996712990975, -1.199719254218453823 ) ) ;
#106740=CARTESIAN_POINT ( 'NONE',  ( 4.217995187182915551, 7.935095128439824563, 0.7216878364870257245 ) ) ;
#106747=CARTESIAN_POINT ( 'NONE',  ( -3.467853430045390706, 7.267855778353407459, 0.7998128361456352531 ) ) ;
#106752=CARTESIAN_POINT ( 'NONE',  ( -6.211043768836215229, 8.339580045099285854, 1.443375672974064550 ) ) ;
#106755=CARTESIAN_POINT ( 'NONE',  ( -6.831329296439251131, 9.063246493969506545, -1.599625672291271394 ) ) ;
#106759=CARTESIAN_POINT ( 'NONE',  ( -4.634908411025374875, 6.500755460986618495, 1.599625672291263179 ) ) ;
#106773=CARTESIAN_POINT ( 'NONE',  ( -5.533136088152923904, 6.588318536667425285, 1.082531754730549078 ) ) ;
#106775=CARTESIAN_POINT ( 'NONE',  ( -5.438229012412899799, 7.437962829272074750, -1.443375672974066548 ) ) ;
#106776=CARTESIAN_POINT ( 'NONE',  ( 7.388267364804250725, 7.584343111885245570, -0.7998128361456341429 ) ) ;
#106777=CARTESIAN_POINT ( 'NONE',  ( -5.444481204339554736, 8.509589284108232121, 1.199719254218454489 ) ) ;
#106797=CARTESIAN_POINT ( 'NONE',  ( 6.556249800660121529, 9.806652646482286073, 1.199719254218452047 ) ) ;
#106835=CARTESIAN_POINT ( 'NONE',  ( 4.037295881819344956, 7.932205305423046582, -0.7998128361456362523 ) ) ;
#106838=CARTESIAN_POINT ( 'NONE',  ( -4.787964524281469458, 5.614988695530339413, -1.199719254218453823 ) ) ;
#106852=CARTESIAN_POINT ( 'NONE',  ( 5.551137550152489553, 5.441024994791534120, 0.7998128361456352531 ) ) ;
#106862=CARTESIAN_POINT ( 'NONE',  ( -5.589704470584107909, 9.743348658981940247, -0.7998128361456362523 ) ) ;
#106866=ORIENTED_EDGE ( 'NONE', *, *, #45431, .T. ) ;
#106867=CARTESIAN_POINT ( 'NONE',  ( 4.376249722160992839, 8.327651452488305850, 0.000000000000000000 ) ) ;
#106873=DIRECTION ( 'NONE',  ( 0.7592566023653016805, 0.6507913734559627184, 4.115938288792103177E-15 ) ) ;
#106879=CARTESIAN_POINT ( 'NONE',  ( 7.200788982633824276, 7.573544365927161515, 0.000000000000000000 ) ) ;
#106880=CARTESIAN_POINT ( 'NONE',  ( -4.719646871332968452, 5.639247783710797712, 1.082531754730549078 ) ) ;
#106882=CARTESIAN_POINT ( 'NONE',  ( -6.473091995881817162, 6.516638514809040217, 0.7998128361456281477 ) ) ;
#106892=CARTESIAN_POINT ( 'NONE',  ( 6.099189001301251523, 8.209082816308541197, 1.599625672291268286 ) ) ;
#106893=ORIENTED_EDGE ( 'NONE', *, *, #61884, .F. ) ;
#106894=CARTESIAN_POINT ( 'NONE',  ( 4.960304097753311936, 6.880383762169266504, 1.599625672291268286 ) ) ;
#106895=CARTESIAN_POINT ( 'NONE',  ( 4.376249722160992839, 8.327651452488305850, 0.000000000000000000 ) ) ;
#106898=CARTESIAN_POINT ( 'NONE',  ( 6.821687566331318564, 7.987665577921906568, 1.199719254218452935 ) ) ;
#106903=AXIS2_PLACEMENT_3D ( 'NONE', #70979, #116622, #182615 ) ;
#106913=CARTESIAN_POINT ( 'NONE',  ( 1.808247988047292143, 2.517446015412736493, 2.499984125739858065 ) ) ;
#106918=CARTESIAN_POINT ( 'NONE',  ( 0.3866926556111174862, 2.897682894409570054, 2.027578619373079594 ) ) ;
#106919=CARTESIAN_POINT ( 'NONE',  ( 3.576318658954677598, 7.394398545414291313, 0.7998128361456281477 ) ) ;
#106923=CARTESIAN_POINT ( 'NONE',  ( 3.237364818613055473, 6.998952398349030268, -1.734723475976807094E-15 ) ) ;
#106928=CARTESIAN_POINT ( 'NONE',  ( 5.481239241674765950, 9.616805891921051952, -0.7998128361456481317 ) ) ;
#106930=EDGE_CURVE ( 'NONE', #95637, #190177, #20339, .T. ) ;
#106933=EDGE_CURVE ( 'NONE', #148211, #92970, #209011, .T. ) ;
#106934=CARTESIAN_POINT ( 'NONE',  ( 5.017926250833595780, 7.907978821730911712, -1.082531754730548412 ) ) ;
#106936=CARTESIAN_POINT ( 'NONE',  ( -6.954406449166956605, 7.078172043641714595, -0.7998128361456362523 ) ) ;
#106938=CARTESIAN_POINT ( 'NONE',  ( 4.016958651398847557, 7.908478536599129249, -0.7998128361456362523 ) ) ;
#106948=CARTESIAN_POINT ( 'NONE',  ( -7.946487431385463651, 8.443525889470736345, 0.7216878364870317197 ) ) ;
#106976=CARTESIAN_POINT ( 'NONE',  ( 4.760321332173959696, 4.726332107057286791, 0.000000000000000000 ) ) ;
#106983=CARTESIAN_POINT ( 'NONE',  ( 6.016786309414542622, 10.24161080428416426, 0.7998128361456341429 ) ) ;
#106995=CARTESIAN_POINT ( 'NONE',  ( -6.473091995881817162, 6.516638514809040217, 0.7998128361456281477 ) ) ;
#106997=CARTESIAN_POINT ( 'NONE',  ( 7.200788982189461507, 8.533913579710086239, -1.082531754730548412 ) ) ;
#107006=CARTESIAN_POINT ( 'NONE',  ( -5.093022980588950865, 5.970890227889075419, -1.199719254218453823 ) ) ;
#107007=COLOUR_RGB ( '', 0.09019608, 0.27058824, 0.51372549) ;
#107010=DIRECTION ( 'NONE',  ( 0.7592566023653005702, -0.6507913734559639396, 0.000000000000000000 ) ) ;
#107016=CARTESIAN_POINT ( 'NONE',  ( -4.228163802615396705, 6.026220084508304708, -1.599625672291271394 ) ) ;
#107038=CARTESIAN_POINT ( 'NONE',  ( -6.200875153403786477, 8.327716660428123419, -1.599625672291271394 ) ) ;
#107040=ORIENTED_EDGE ( 'NONE', *, *, #58752, .F. ) ;
#107044=ORIENTED_EDGE ( 'NONE', *, *, #18201, .T. ) ;
#107050=CARTESIAN_POINT ( 'NONE',  ( -6.567035442730039030, 6.789466400107097677, -0.3981859287331638297 ) ) ;
#107063=DIRECTION ( 'NONE',  ( 0.7592566023652989049, 0.6507913734559658270, 0.000000000000000000 ) ) ;
#107066=CARTESIAN_POINT ( 'NONE',  ( -5.336015975430226099, 8.383046517047350932, -1.199719254218453823 ) ) ;
#107077=CARTESIAN_POINT ( 'NONE',  ( 7.648208051440442468, 8.095533279534887328, 0.000000000000000000 ) ) ;
#107086=CARTESIAN_POINT ( 'NONE',  ( -4.671932466396476968, 7.377723763423310821, 1.128687292116478114 ) ) ;
#107090=CARTESIAN_POINT ( 'NONE',  ( 5.435893244436359240, 5.306573304789342416, -0.7998128361456481317 ) ) ;
#107097=CARTESIAN_POINT ( 'NONE',  ( 5.742760583840166966, 8.857581893525663830, 1.199719254218452047 ) ) ;
#107099=CARTESIAN_POINT ( 'NONE',  ( 5.722423353419669567, 8.833855124701747386, 1.199719254218451159 ) ) ;
#107112=CARTESIAN_POINT ( 'NONE',  ( 6.297309100973213170, 6.875137029808006339, 0.7249047842670247599 ) ) ;
#107114=CARTESIAN_POINT ( 'NONE',  ( 5.072158865288233009, 7.010880990960010273, 1.443375672974065660 ) ) ;
#107122=CARTESIAN_POINT ( 'NONE',  ( -3.797165540279144214, 6.587721009371067638, 1.199719254218452935 ) ) ;
#107133=CARTESIAN_POINT ( 'NONE',  ( -4.109529958273628658, 7.808552361378938045, 0.7216878364870338292 ) ) ;
#107137=CARTESIAN_POINT ( 'NONE',  ( 7.693325821111733021, 7.940244644243982464, -0.7998128361456341429 ) ) ;
#107153=CARTESIAN_POINT ( 'NONE',  ( 5.345657705538078730, 9.458627433094950021, 0.7998128361456331437 ) ) ;
#107171=CARTESIAN_POINT ( 'NONE',  ( -5.264308783856126439, 9.363720357799287797, -0.7998128361456362523 ) ) ;
#107172=VECTOR ( 'NONE', #76960, 1000.000000000000114 ) ;
#107174=DIRECTION ( 'NONE',  ( 0.000000000000000000, -1.000000000000000000, 0.000000000000000000 ) ) ;
#107176=CARTESIAN_POINT ( 'NONE',  ( -6.486551268120854807, 6.767445667853342783, -0.2095380678983837508 ) ) ;
#107183=EDGE_CURVE ( 'NONE', #136751, #31895, #118250, .T. ) ;
#107194=CARTESIAN_POINT ( 'NONE',  ( 5.234856708652235291, 5.279956712948652431, 0.7216878364870338292 ) ) ;
#107195=ORIENTED_EDGE ( 'NONE', *, *, #15512, .F. ) ;
#107199=CARTESIAN_POINT ( 'NONE',  ( 3.588273936444265289, 7.344317902764286643, -0.3372145678562175064 ) ) ;
#107206=CARTESIAN_POINT ( 'NONE',  ( -5.831415467653581430, 5.975941931783510519, 0.7216878364870257245 ) ) ;
#107211=CARTESIAN_POINT ( 'NONE',  ( 5.594708818112484217, 5.774250729507365953, 0.6894988139244705438 ) ) ;
#107241=CARTESIAN_POINT ( 'NONE',  ( 5.011674058906918638, 5.875983152593414971, 1.199719254218452047 ) ) ;
#107243=LINE ( 'NONE', #73602, #37091 ) ;
#107252=CARTESIAN_POINT ( 'NONE',  ( -5.641601317062233001, 9.595968946632336127, -0.7216878364870338292 ) ) ;
#107255=CARTESIAN_POINT ( 'NONE',  ( 4.706088717274906408, 5.623429937309770921, 1.082531754730549078 ) ) ;
#107269=CARTESIAN_POINT ( 'NONE',  ( 5.076602173674213070, 4.887400388900169368, 0.000000000000000000 ) ) ;
#107271=CARTESIAN_POINT ( 'NONE',  ( -5.316205630334276400, 5.374863788244313767, -0.7216878364870338292 ) ) ;
#107301=CARTESIAN_POINT ( 'NONE',  ( -5.932574734431526942, 9.079031735882207244, 1.199719254218454489 ) ) ;
#107304=CARTESIAN_POINT ( 'NONE',  ( -5.936491157937300756, 8.019268665717216749, 1.599625672291263179 ) ) ;
#107309=CARTESIAN_POINT ( 'NONE',  ( -7.553300976144794454, 7.984808358356614733, -0.7216878364870338292 ) ) ;
#107315=CARTESIAN_POINT ( 'NONE',  ( -8.086512275908061653, 8.398962174839683215, 0.000000000000000000 ) ) ;
#107320=ORIENTED_EDGE ( 'NONE', *, *, #88039, .F. ) ;
#107323=CARTESIAN_POINT ( 'NONE',  ( -5.921879234118920365, 10.13088588310589699, 0.000000000000000000 ) ) ;
#107325=CARTESIAN_POINT ( 'NONE',  ( 4.701115458738250652, 8.361069499448168685, -0.6471830670988186762 ) ) ;
#107328=CARTESIAN_POINT ( 'NONE',  ( 3.853900823548666921, 8.531065964594311879, 2.447540105570115809 ) ) ;
#107330=CARTESIAN_POINT ( 'NONE',  ( 7.506374323821472849, 8.786466794993730289, -1.199719254218452047 ) ) ;
#107334=EDGE_CURVE ( 'NONE', #123356, #199128, #71540, .T. ) ;
#107335=AXIS2_PLACEMENT_3D ( 'NONE', #184051, #69217, #179813 ) ;
#107341=CARTESIAN_POINT ( 'NONE',  ( -7.761116589180078407, 8.019333873657032541, 0.000000000000000000 ) ) ;
#107354=CARTESIAN_POINT ( 'NONE',  ( 4.934241560730721510, 4.721313007132757811, 0.000000000000000000 ) ) ;
#107371=CARTESIAN_POINT ( 'NONE',  ( 6.596403382356258227, 6.772441155557838321, -0.1798620802159808241 ) ) ;
#107372=CARTESIAN_POINT ( 'NONE',  ( -4.570507181138272479, 7.385989907086349504, 1.082531754730549967 ) ) ;
#107380=B_SPLINE_CURVE_WITH_KNOTS ( 'NONE', 3,
 ( #135367, #35703, #186214, #202447, #36766, #122393, #20511, #169969, #86596, #53023 ),
 .UNSPECIFIED., .F., .F.,
 ( 4, 3, 3, 4 ),
 ( 3.112925509940513280E-16, 3.125186881574499746E-05, 5.993688232072589769E-05, 8.863274572801039055E-05 ),
 .UNSPECIFIED. ) ;
#107397=EDGE_LOOP ( 'NONE', ( #31006, #59581, #39863, #133603, #10718, #92167, #135857, #51586, #68055, #19584, #37172, #199398, #77277, #75549 ) ) ;
#107401=CARTESIAN_POINT ( 'NONE',  ( 4.065465959251388206, 5.836405933916976707, -1.599625672291269396 ) ) ;
#107419=CARTESIAN_POINT ( 'NONE',  ( -6.805266759416629618, 6.904175738932996964, 0.000000000000000000 ) ) ;
#107429=ORIENTED_EDGE ( 'NONE', *, *, #153998, .F. ) ;
#107436=CARTESIAN_POINT ( 'NONE',  ( 5.086243903782109221, 5.962981304947771122, -1.199719254218452047 ) ) ;
#107438=CARTESIAN_POINT ( 'NONE',  ( 7.634649897826744080, 9.040084647953621655, 1.082531754730549078 ) ) ;
#107441=ORIENTED_EDGE ( 'NONE', *, *, #173426, .T. ) ;
#107446=CARTESIAN_POINT ( 'NONE',  ( 4.801282209253342259, 8.127660309270595462, 0.8325795361681764817 ) ) ;
#107448=CARTESIAN_POINT ( 'NONE',  ( 5.094250900851895025, 7.824382189606214233, 1.140223938556598871 ) ) ;
#107469=CARTESIAN_POINT ( 'NONE',  ( -5.815521545619021460, 5.749472989502435460, -0.7998128361456362523 ) ) ;
#107471=CARTESIAN_POINT ( 'NONE',  ( 4.411198876399872404, 6.239761003923544713, -1.599625672291273171 ) ) ;
#107475=CARTESIAN_POINT ( 'NONE',  ( -4.776215253764153346, 8.794277906025310898, -0.7998128361456362523 ) ) ;
#107477=CARTESIAN_POINT ( 'NONE',  ( 3.097897175693991478, 6.151267098325809535, -0.8540112008112433761 ) ) ;
#107478=CARTESIAN_POINT ( 'NONE',  ( 4.864343252252968597, 8.897093904262280972, 0.000000000000000000 ) ) ;
#107480=( BOUNDED_SURFACE ( )  B_SPLINE_SURFACE ( 1, 2, ( 
 ( #133663, #150955, #18781, #103259, #202858, #120650, #83793, #378, #50243, #132594, #2519, #149888, #20904, #134718, #87000, #153072, #16648, #82733, #4649, #70719, #198596, #200724, #116363, #182353, #52375, #35034, #118504, #135768, #184486, #1453, #19854, #199664, #117436, #183433, #36103, #85941, #152014, #69660, #189831, #75026, #56643, #156286, #107591, #105416, #208204, #8946, #10011, #92374, #23043, #76087, #72870, #24119, #173623, #121727, #187692, #59836, #104330, #170378, #25195, #91299, #174684, #89159, #171454, #142189, #41480, #39321, #157357, #186629, #137906, #71791, #190887, #141138, #42553, #155212, #207148, #58771, #108656, #204999, #55573, #122807, #40406, #158411, #123866, #38256, #124926, #140050, #6793, #203925, #21965, #138976, #26258, #88073, #188766, #5714, #154147, #106508, #172535, #90222, #7870, #73958, #206075, #57709, #77149, #111865, #128134, #194098, #146453, #47889, #125989, #46814, #15331, #94501, #193026, #176792, #160539, #28407, #109730, #78218, #143270, #210341, #212468, #29482, #12145, #61980, #64112, #144341, #80354, #44678, #45747, #177870, #110790, #209260, #159472, #96634, #178941, #95573, #191946, #43612, #79289, #112928, #162688, #147502, #161623, #13216, #145407, #211407, #63037, #11070, #97694, #179996, #129204, #195181, #30555, #14263, #130254, #196245, #114001, #175737, #31620, #60905, #163752, #81421, #213523, #27330, #93432, #127064, #49988, #98745, #133406, #201536, #181050, #134473, #65146, #169061, #131302, #83542, #200477, #32666, #197293, #135514, #101936, #52123, #183181, #152820, #164803, #67267, #100860, #1205, #18537, #35857, #199411, #16395, #115052, #150703, #2265, #51056, #166944, #48934, #119312, #117180, #185298, #116106, #69407, #168001, #53184, #66198, #33728, #19607, #36922, #68341, #85679, #118252, #82474, #184233, #34785, #17457, #148564, #151767, #103005, #20658, #84614, #3336, #86748, #130, #132342, #198348, #182097, #99806, #165871, #149623, #107330, #26001, #5462, #189577, #73696, #157099, #140874, #124672, #173354, #91039, #23865 ),
 ( #120394, #6542, #40141, #154956, #172278, #41225, #72620, #186369, #54257, #89972, #156024, #138719, #106254, #202604, #58517, #56386, #190629, #55321, #24936, #8688, #206885, #22786, #87821, #88903, #204737, #42290, #7613, #108401, #74770, #139794, #153893, #170124, #174425, #71542, #205821, #123614, #39070, #38004, #92110, #4396, #104076, #137652, #70467, #136584, #121472, #203672, #21710, #122549, #188511, #57454, #187443, #105157, #171196, #79021, #47621, #126803, #10811, #209004, #192759, #60641, #141939, #110535, #109473, #28147, #30288, #61715, #44416, #94242, #178673, #176536, #112665, #76886, #160281, #11883, #143006, #27068, #191693, #128930, #211144, #77959, #158165, #75832, #144080, #43353, #95310, #210076, #127883, #177608, #193833, #207952, #45484, #175481, #111600, #80086, #59575, #12942, #9757, #113733, #125732, #29220, #145138, #93176, #159210, #14002, #194907, #62766, #161359, #31356, #46545, #96373, #162425, #146190, #212205, #63841, #129998, #195988, #179739, #182916, #34532, #17197, #133143, #81160, #151503, #149359, #6012, #148305, #134207, #51868, #19340, #115850, #180788, #181835, #165607, #72082, #100603, #138193, #117989, #50787, #32411, #48671, #204203, #164543, #166679, #2005, #132084, #131046, #35593, #200216, #213270, #98477, #68071, #183982, #214304, #16128, #114788, #83271, #99544, #941, #101671, #85419, #97431, #18271, #55857, #65935, #82212, #198094, #49721, #33470, #147243, #67006, #199143, #116916, #167741, #84353, #150443, #122013, #187980, #163486, #15068, #64899, #197036, #206364, #24397, #123100, #73152, #10296, #92656, #140346, #39606, #171738, #207433, #26548, #76370, #61193, #74252, #25484, #157642, #9239, #8168, #139258, #11357, #93720, #57991, #41769, #158698, #124154, #142477, #75311, #126280, #89444, #190115, #205289, #191172, #107882, #141427, #59052, #90509, #155496, #156574, #56927, #173909, #176027, #7079, #108946, #105710, #143555, #23335, #91590, #174966, #189057, #40694, #110014, #208485, #60121, #125210, #127352, #106797, #42839, #192238, #43900, #27619 ) ),
 .UNSPECIFIED., .F., .F., .F. ) 
 B_SPLINE_SURFACE_WITH_KNOTS ( ( 2, 2 ),
 ( 3, 2, 2, 2, 2, 2, 2, 2, 2, 2, 2, 2, 2, 2, 2, 2, 2, 2, 2, 2, 2, 2, 2, 2, 2, 2, 2, 2, 2, 2, 2, 2, 2, 2, 2, 2, 2, 2, 2, 2, 2, 2, 2, 2, 2, 2, 2, 2, 2, 2, 2, 2, 2, 2, 2, 2, 2, 2, 2, 2, 2, 2, 2, 2, 2, 2, 2, 2, 2, 2, 2, 2, 2, 2, 2, 2, 2, 2, 2, 2, 2, 2, 2, 2, 2, 2, 2, 2, 2, 2, 2, 2, 2, 2, 2, 2, 2, 2, 2, 2, 2, 2, 2, 2, 2, 2, 2, 2, 2, 2, 2, 2, 2, 2, 2, 2, 2, 2, 2, 2, 3 ),
 ( 0.000000000000000000, 1.000000000000000000 ),
 ( 0.000000000000000000, 0.008333333333333333218, 0.01666666666666666644, 0.02500000000000000139, 0.03333333333333333287, 0.04166666666666666435, 0.05000000000000000278, 0.05833333333333333426, 0.06666666666666666574, 0.07499999999999999722, 0.08333333333333332871, 0.09166666666666666019, 0.1000000000000000056, 0.1083333333333333370, 0.1166666666666666685, 0.1250000000000000000, 0.1333333333333333315, 0.1416666666666666630, 0.1499999999999999944, 0.1583333333333333259, 0.1666666666666666574, 0.1749999999999999889, 0.1833333333333333204, 0.1916666666666666796, 0.2000000000000000111, 0.2083333333333333426, 0.2166666666666666741, 0.2250000000000000056, 0.2333333333333333370, 0.2416666666666666685, 0.2500000000000000000, 0.2583333333333333592, 0.2666666666666666630, 0.2750000000000000222, 0.2833333333333333259, 0.2916666666666666852, 0.2999999999999999889, 0.3083333333333333481, 0.3166666666666666519, 0.3250000000000000111, 0.3333333333333333148, 0.3416666666666666741, 0.3499999999999999778, 0.3583333333333333370, 0.3666666666666666408, 0.3750000000000000000, 0.3833333333333333592, 0.3916666666666666630, 0.4000000000000000222, 0.4083333333333333259, 0.4166666666666666852, 0.4249999999999999889, 0.4333333333333333481, 0.4416666666666666519, 0.4500000000000000111, 0.4583333333333333148, 0.4666666666666666741, 0.4749999999999999778, 0.4833333333333333370, 0.4916666666666666408, 0.5000000000000000000, 0.5083333333333333037, 0.5166666666666667185, 0.5250000000000000222, 0.5333333333333333259, 0.5416666666666666297, 0.5500000000000000444, 0.5583333333333333481, 0.5666666666666666519, 0.5749999999999999556, 0.5833333333333333703, 0.5916666666666666741, 0.5999999999999999778, 0.6083333333333332815, 0.6166666666666666963, 0.6250000000000000000, 0.6333333333333333037, 0.6416666666666667185, 0.6500000000000000222, 0.6583333333333333259, 0.6666666666666666297, 0.6750000000000000444, 0.6833333333333333481, 0.6916666666666666519, 0.6999999999999999556, 0.7083333333333333703, 0.7166666666666666741, 0.7249999999999999778, 0.7333333333333332815, 0.7416666666666666963, 0.7500000000000000000, 0.7583333333333333037, 0.7666666666666667185, 0.7750000000000000222, 0.7833333333333333259, 0.7916666666666666297, 0.8000000000000000444, 0.8083333333333333481, 0.8166666666666666519, 0.8249999999999999556, 0.8333333333333333703, 0.8416666666666666741, 0.8499999999999999778, 0.8583333333333332815, 0.8666666666666666963, 0.8750000000000000000, 0.8833333333333333037, 0.8916666666666667185, 0.9000000000000000222, 0.9083333333333333259, 0.9166666666666666297, 0.9250000000000000444, 0.9333333333333333481, 0.9416666666666666519, 0.9499999999999999556, 0.9583333333333333703, 0.9666666666666666741, 0.9749999999999999778, 0.9833333333333332815, 0.9916666666666666963, 1.000000000000000000 ),
 .UNSPECIFIED. ) 
 GEOMETRIC_REPRESENTATION_ITEM ( )  RATIONAL_B_SPLINE_SURFACE ( (
 ( 1.000000000000000000, 0.8660254037844387076, 1.000000000000000000, 0.8660254037844387076, 1.000000000000000000, 0.8660254037844387076, 1.000000000000000000, 0.8660254037844387076, 1.000000000000000000, 0.8660254037844387076, 1.000000000000000000, 0.8660254037844387076, 1.000000000000000000, 0.8660254037844387076, 1.000000000000000000, 0.8660254037844387076, 1.000000000000000000, 0.8660254037844387076, 1.000000000000000000, 0.8660254037844387076, 1.000000000000000000, 0.8660254037844387076, 1.000000000000000000, 0.8660254037844387076, 1.000000000000000000, 0.8660254037844387076, 1.000000000000000000, 0.8660254037844387076, 1.000000000000000000, 0.8660254037844387076, 1.000000000000000000, 0.8660254037844387076, 1.000000000000000000, 0.8660254037844387076, 1.000000000000000000, 0.8660254037844387076, 1.000000000000000000, 0.8660254037844387076, 1.000000000000000000, 0.8660254037844387076, 1.000000000000000000, 0.8660254037844387076, 1.000000000000000000, 0.8660254037844387076, 1.000000000000000000, 0.8660254037844387076, 1.000000000000000000, 0.8660254037844387076, 1.000000000000000000, 0.8660254037844387076, 1.000000000000000000, 0.8660254037844387076, 1.000000000000000000, 0.8660254037844387076, 1.000000000000000000, 0.8660254037844387076, 1.000000000000000000, 0.8660254037844387076, 1.000000000000000000, 0.8660254037844387076, 1.000000000000000000, 0.8660254037844387076, 1.000000000000000000, 0.8660254037844387076, 1.000000000000000000, 0.8660254037844387076, 1.000000000000000000, 0.8660254037844387076, 1.000000000000000000, 0.8660254037844387076, 1.000000000000000000, 0.8660254037844387076, 1.000000000000000000, 0.8660254037844387076, 1.000000000000000000, 0.8660254037844387076, 1.000000000000000000, 0.8660254037844387076, 1.000000000000000000, 0.8660254037844387076, 1.000000000000000000, 0.8660254037844387076, 1.000000000000000000, 0.8660254037844387076, 1.000000000000000000, 0.8660254037844387076, 1.000000000000000000, 0.8660254037844387076, 1.000000000000000000, 0.8660254037844387076, 1.000000000000000000, 0.8660254037844387076, 1.000000000000000000, 0.8660254037844387076, 1.000000000000000000, 0.8660254037844387076, 1.000000000000000000, 0.8660254037844387076, 1.000000000000000000, 0.8660254037844387076, 1.000000000000000000, 0.8660254037844387076, 1.000000000000000000, 0.8660254037844387076, 1.000000000000000000, 0.8660254037844387076, 1.000000000000000000, 0.8660254037844387076, 1.000000000000000000, 0.8660254037844387076, 1.000000000000000000, 0.8660254037844387076, 1.000000000000000000, 0.8660254037844387076, 1.000000000000000000, 0.8660254037844387076, 1.000000000000000000, 0.8660254037844387076, 1.000000000000000000, 0.8660254037844387076, 1.000000000000000000, 0.8660254037844387076, 1.000000000000000000, 0.8660254037844387076, 1.000000000000000000, 0.8660254037844387076, 1.000000000000000000, 0.8660254037844387076, 1.000000000000000000, 0.8660254037844387076, 1.000000000000000000, 0.8660254037844387076, 1.000000000000000000, 0.8660254037844387076, 1.000000000000000000, 0.8660254037844387076, 1.000000000000000000, 0.8660254037844387076, 1.000000000000000000, 0.8660254037844387076, 1.000000000000000000, 0.8660254037844387076, 1.000000000000000000, 0.8660254037844387076, 1.000000000000000000, 0.8660254037844387076, 1.000000000000000000, 0.8660254037844387076, 1.000000000000000000, 0.8660254037844387076, 1.000000000000000000, 0.8660254037844387076, 1.000000000000000000, 0.8660254037844387076, 1.000000000000000000, 0.8660254037844387076, 1.000000000000000000, 0.8660254037844387076, 1.000000000000000000, 0.8660254037844387076, 1.000000000000000000, 0.8660254037844387076, 1.000000000000000000, 0.8660254037844387076, 1.000000000000000000, 0.8660254037844387076, 1.000000000000000000, 0.8660254037844387076, 1.000000000000000000, 0.8660254037844387076, 1.000000000000000000, 0.8660254037844387076, 1.000000000000000000, 0.8660254037844387076, 1.000000000000000000, 0.8660254037844387076, 1.000000000000000000, 0.8660254037844387076, 1.000000000000000000, 0.8660254037844387076, 1.000000000000000000, 0.8660254037844387076, 1.000000000000000000, 0.8660254037844387076, 1.000000000000000000, 0.8660254037844387076, 1.000000000000000000, 0.8660254037844387076, 1.000000000000000000, 0.8660254037844387076, 1.000000000000000000, 0.8660254037844387076, 1.000000000000000000, 0.8660254037844387076, 1.000000000000000000, 0.8660254037844387076, 1.000000000000000000, 0.8660254037844387076, 1.000000000000000000, 0.8660254037844387076, 1.000000000000000000, 0.8660254037844387076, 1.000000000000000000, 0.8660254037844387076, 1.000000000000000000, 0.8660254037844387076, 1.000000000000000000, 0.8660254037844387076, 1.000000000000000000, 0.8660254037844387076, 1.000000000000000000, 0.8660254037844387076, 1.000000000000000000, 0.8660254037844387076, 1.000000000000000000, 0.8660254037844387076, 1.000000000000000000, 0.8660254037844387076, 1.000000000000000000, 0.8660254037844387076, 1.000000000000000000, 0.8660254037844387076, 1.000000000000000000, 0.8660254037844387076, 1.000000000000000000, 0.8660254037844387076, 1.000000000000000000, 0.8660254037844387076, 1.000000000000000000, 0.8660254037844387076, 1.000000000000000000, 0.8660254037844387076, 1.000000000000000000, 0.8660254037844387076, 1.000000000000000000, 0.8660254037844387076, 1.000000000000000000, 0.8660254037844387076, 1.000000000000000000, 0.8660254037844387076, 1.000000000000000000),
 ( 1.000000000000000000, 0.8660254037844387076, 1.000000000000000000, 0.8660254037844387076, 1.000000000000000000, 0.8660254037844387076, 1.000000000000000000, 0.8660254037844387076, 1.000000000000000000, 0.8660254037844387076, 1.000000000000000000, 0.8660254037844387076, 1.000000000000000000, 0.8660254037844387076, 1.000000000000000000, 0.8660254037844387076, 1.000000000000000000, 0.8660254037844387076, 1.000000000000000000, 0.8660254037844387076, 1.000000000000000000, 0.8660254037844387076, 1.000000000000000000, 0.8660254037844387076, 1.000000000000000000, 0.8660254037844387076, 1.000000000000000000, 0.8660254037844387076, 1.000000000000000000, 0.8660254037844387076, 1.000000000000000000, 0.8660254037844387076, 1.000000000000000000, 0.8660254037844387076, 1.000000000000000000, 0.8660254037844387076, 1.000000000000000000, 0.8660254037844387076, 1.000000000000000000, 0.8660254037844387076, 1.000000000000000000, 0.8660254037844387076, 1.000000000000000000, 0.8660254037844387076, 1.000000000000000000, 0.8660254037844387076, 1.000000000000000000, 0.8660254037844387076, 1.000000000000000000, 0.8660254037844387076, 1.000000000000000000, 0.8660254037844387076, 1.000000000000000000, 0.8660254037844387076, 1.000000000000000000, 0.8660254037844387076, 1.000000000000000000, 0.8660254037844387076, 1.000000000000000000, 0.8660254037844387076, 1.000000000000000000, 0.8660254037844387076, 1.000000000000000000, 0.8660254037844387076, 1.000000000000000000, 0.8660254037844387076, 1.000000000000000000, 0.8660254037844387076, 1.000000000000000000, 0.8660254037844387076, 1.000000000000000000, 0.8660254037844387076, 1.000000000000000000, 0.8660254037844387076, 1.000000000000000000, 0.8660254037844387076, 1.000000000000000000, 0.8660254037844387076, 1.000000000000000000, 0.8660254037844387076, 1.000000000000000000, 0.8660254037844387076, 1.000000000000000000, 0.8660254037844387076, 1.000000000000000000, 0.8660254037844387076, 1.000000000000000000, 0.8660254037844387076, 1.000000000000000000, 0.8660254037844387076, 1.000000000000000000, 0.8660254037844387076, 1.000000000000000000, 0.8660254037844387076, 1.000000000000000000, 0.8660254037844387076, 1.000000000000000000, 0.8660254037844387076, 1.000000000000000000, 0.8660254037844387076, 1.000000000000000000, 0.8660254037844387076, 1.000000000000000000, 0.8660254037844387076, 1.000000000000000000, 0.8660254037844387076, 1.000000000000000000, 0.8660254037844387076, 1.000000000000000000, 0.8660254037844387076, 1.000000000000000000, 0.8660254037844387076, 1.000000000000000000, 0.8660254037844387076, 1.000000000000000000, 0.8660254037844387076, 1.000000000000000000, 0.8660254037844387076, 1.000000000000000000, 0.8660254037844387076, 1.000000000000000000, 0.8660254037844387076, 1.000000000000000000, 0.8660254037844387076, 1.000000000000000000, 0.8660254037844387076, 1.000000000000000000, 0.8660254037844387076, 1.000000000000000000, 0.8660254037844387076, 1.000000000000000000, 0.8660254037844387076, 1.000000000000000000, 0.8660254037844387076, 1.000000000000000000, 0.8660254037844387076, 1.000000000000000000, 0.8660254037844387076, 1.000000000000000000, 0.8660254037844387076, 1.000000000000000000, 0.8660254037844387076, 1.000000000000000000, 0.8660254037844387076, 1.000000000000000000, 0.8660254037844387076, 1.000000000000000000, 0.8660254037844387076, 1.000000000000000000, 0.8660254037844387076, 1.000000000000000000, 0.8660254037844387076, 1.000000000000000000, 0.8660254037844387076, 1.000000000000000000, 0.8660254037844387076, 1.000000000000000000, 0.8660254037844387076, 1.000000000000000000, 0.8660254037844387076, 1.000000000000000000, 0.8660254037844387076, 1.000000000000000000, 0.8660254037844387076, 1.000000000000000000, 0.8660254037844387076, 1.000000000000000000, 0.8660254037844387076, 1.000000000000000000, 0.8660254037844387076, 1.000000000000000000, 0.8660254037844387076, 1.000000000000000000, 0.8660254037844387076, 1.000000000000000000, 0.8660254037844387076, 1.000000000000000000, 0.8660254037844387076, 1.000000000000000000, 0.8660254037844387076, 1.000000000000000000, 0.8660254037844387076, 1.000000000000000000, 0.8660254037844387076, 1.000000000000000000, 0.8660254037844387076, 1.000000000000000000, 0.8660254037844387076, 1.000000000000000000, 0.8660254037844387076, 1.000000000000000000, 0.8660254037844387076, 1.000000000000000000, 0.8660254037844387076, 1.000000000000000000, 0.8660254037844387076, 1.000000000000000000, 0.8660254037844387076, 1.000000000000000000, 0.8660254037844387076, 1.000000000000000000, 0.8660254037844387076, 1.000000000000000000, 0.8660254037844387076, 1.000000000000000000, 0.8660254037844387076, 1.000000000000000000, 0.8660254037844387076, 1.000000000000000000, 0.8660254037844387076, 1.000000000000000000, 0.8660254037844387076, 1.000000000000000000, 0.8660254037844387076, 1.000000000000000000, 0.8660254037844387076, 1.000000000000000000, 0.8660254037844387076, 1.000000000000000000, 0.8660254037844387076, 1.000000000000000000, 0.8660254037844387076, 1.000000000000000000, 0.8660254037844387076, 1.000000000000000000, 0.8660254037844387076, 1.000000000000000000, 0.8660254037844387076, 1.000000000000000000, 0.8660254037844387076, 1.000000000000000000, 0.8660254037844387076, 1.000000000000000000, 0.8660254037844387076, 1.000000000000000000, 0.8660254037844387076, 1.000000000000000000, 0.8660254037844387076, 1.000000000000000000, 0.8660254037844387076, 1.000000000000000000) ) ) 
 REPRESENTATION_ITEM ( '' )  SURFACE ( )  );
#107484=CARTESIAN_POINT ( 'NONE',  ( -4.593509350353649268, 8.487843406384373068, -0.1931319778552646749 ) ) ;
#107492=CARTESIAN_POINT ( 'NONE',  ( -6.116136693096208887, 6.308116694799912771, 0.7216878364870257245 ) ) ;
#107500=CARTESIAN_POINT ( 'NONE',  ( 5.885648082108199119, 6.999582529615296700, 1.082531754730549967 ) ) ;
#107504=CARTESIAN_POINT ( 'NONE',  ( -7.422162748838431412, 7.623887726591770608, -0.7998128361456362523 ) ) ;
#107517=CARTESIAN_POINT ( 'NONE',  ( 4.598150373690133463, 5.393538853173795111, -1.199719254218452047 ) ) ;
#107544=CARTESIAN_POINT ( 'NONE',  ( -6.292392690518223475, 6.513748691792265788, -0.7216878364870338292 ) ) ;
#107558=ORIENTED_EDGE ( 'NONE', *, *, #42400, .F. ) ;
#107568=CARTESIAN_POINT ( 'NONE',  ( -2.997761361953021009, 6.511488999004883205, -0.7216878364870458196 ) ) ;
#107575=CARTESIAN_POINT ( 'NONE',  ( -3.851398154733808088, 6.650992392901508232, -1.199719254218450271 ) ) ;
#107579=VERTEX_POINT ( 'NONE', #7611 ) ;
#107584=CARTESIAN_POINT ( 'NONE',  ( -4.167152111353897403, 5.955039778036558040, 1.599625672291270506 ) ) ;
#107586=CARTESIAN_POINT ( 'NONE',  ( 6.127784903196001665, 7.091900248975262500, -1.102264294108054266 ) ) ;
#107591=CARTESIAN_POINT ( 'NONE',  ( 3.379725431556547477, 7.165039780116438273, -1.734723475976807094E-15 ) ) ;
#107594=EDGE_CURVE ( 'NONE', #104090, #172895, #113265, .T. ) ;
#107597=CARTESIAN_POINT ( 'NONE',  ( -5.562588163356775972, 9.711712967216715953, 0.7998128361456291469 ) ) ;
#107601=CARTESIAN_POINT ( 'NONE',  ( -5.147255595043616516, 6.034161611419515125, 1.199719254218452935 ) ) ;
#107606=CARTESIAN_POINT ( 'NONE',  ( 6.034787771414195312, 6.213209619504250547, -0.7216878364870458196 ) ) ;
#107607=CARTESIAN_POINT ( 'NONE',  ( -4.434925645001610128, 8.188180662561590495, 0.7216878364870338292 ) ) ;
#107613=CARTESIAN_POINT ( 'NONE',  ( 3.067887898442204442, 6.801229324816399746, 0.7998128361456271485 ) ) ;
#107624=CARTESIAN_POINT ( 'NONE',  ( 5.469253881944042384, 7.602781119232224327, 1.336104631850141944 ) ) ;
#107633=CARTESIAN_POINT ( 'NONE',  ( 7.212011367826596242, 7.378711115411311638, 0.000000000000000000 ) ) ;
#107643=CARTESIAN_POINT ( 'NONE',  ( 4.771497086726927073, 8.161215468402982509, 0.7801120568680236511 ) ) ;
#107649=AXIS2_PLACEMENT_3D ( 'NONE', #56578, #42479, #55504 ) ;
#107652=CARTESIAN_POINT ( 'NONE',  ( 6.156284269057003655, 9.340026192945279249, -1.199719254218452047 ) ) ;
#107657=CARTESIAN_POINT ( 'NONE',  ( -4.603364586660168456, 8.384938909114524108, 0.004600842637982396899 ) ) ;
#107665=CARTESIAN_POINT ( 'NONE',  ( -6.607619761813764647, 8.802252036906432764, 1.599625672291269396 ) ) ;
#107678=CARTESIAN_POINT ( 'NONE',  ( 7.862802741282558294, 8.137967717776607657, 0.000000000000000000 ) ) ;
#107685=CARTESIAN_POINT ( 'NONE',  ( -6.577113915960828727, 9.727031097712693253, -1.082531754730549967 ) ) ;
#107687=CARTESIAN_POINT ( 'NONE',  ( 5.564695703766185275, 5.456842840674144490, 0.000000000000000000 ) ) ;
#107690=CARTESIAN_POINT ( 'NONE',  ( 4.380693030546916944, 6.204170850428461392, 1.443375672974058777 ) ) ;
#107705=CARTESIAN_POINT ( 'NONE',  ( -7.607533591043815768, 8.048079742405473525, 0.000000000000000000 ) ) ;
#107706=CARTESIAN_POINT ( 'NONE',  ( 7.851580356089786328, 8.332800968292465527, 0.000000000000000000 ) ) ;
#107718=CARTESIAN_POINT ( 'NONE',  ( -3.962726036944197894, 7.845207153068690431, -0.7998128361456481317 ) ) ;
#107719=CARTESIAN_POINT ( 'NONE',  ( -4.285259070371116863, 7.157163461145040095, 1.199719254218452935 ) ) ;
#107721=CARTESIAN_POINT ( 'NONE',  ( 6.170369307550806148, 10.21286493553572328, 0.7216878364870317197 ) ) ;
#107722=ADVANCED_FACE ( 'NONE', ( #88901 ), #207331, .T. ) ;
#107734=CARTESIAN_POINT ( 'NONE',  ( -5.265531293961836390, 7.681012046988098696, -1.216234931179949186 ) ) ;
#107738=CIRCLE ( 'NONE', #14260, 0.4800000000000000933 ) ;
#107740=CARTESIAN_POINT ( 'NONE',  ( 5.261973015879598314, 5.311592404713873172, -0.7216878364870458196 ) ) ;
#107745=CARTESIAN_POINT ( 'NONE',  ( -7.306918443122272677, 7.489436036589583345, 0.7998128361456341429 ) ) ;
#107758=CARTESIAN_POINT ( 'NONE',  ( 5.554000203453580475, 6.508696987897830688, -1.199719254218452047 ) ) ;
#107768=CARTESIAN_POINT ( 'NONE',  ( -2.830620210203090181, 6.524417021870718258, 0.000000000000000000 ) ) ;
#107772=DIRECTION ( 'NONE',  ( -0.7592566023652990159, 0.6507913734559659380, -9.407858945810539579E-15 ) ) ;
#107774=DIRECTION ( 'NONE',  ( 0.6507913734559641616, 0.7592566023653004592, 0.000000000000000000 ) ) ;
#107794=CARTESIAN_POINT ( 'NONE',  ( 7.512626515748113576, 7.937354821227203594, 0.7216878364870267237 ) ) ;
#107799=CARTESIAN_POINT ( 'NONE',  ( 7.322812364712459221, 7.715904978352238430, 0.000000000000000000 ) ) ;
#107822=CARTESIAN_POINT ( 'NONE',  ( -4.573896719763875574, 6.429575154514868274, -1.599625672291271394 ) ) ;
#107824=CARTESIAN_POINT ( 'NONE',  ( 4.028181036591620412, 7.713645286083276709, -0.7216878364870338292 ) ) ;
#107830=CARTESIAN_POINT ( 'NONE',  ( -3.546339698426324460, 6.295090860542775779, -1.199719254218450271 ) ) ;
#107835=CARTESIAN_POINT ( 'NONE',  ( -5.912764389335557702, 8.951956649983198844, 1.082531754730550855 ) ) ;
#107841=CARTESIAN_POINT ( 'NONE',  ( -5.646044625448194410, 5.551749915969804938, 0.000000000000000000 ) ) ;
#107849=EDGE_LOOP ( 'NONE', ( #93549, #146992, #27058, #51332, #76360 ) ) ;
#107853=CARTESIAN_POINT ( 'NONE',  ( -4.995253251992230581, 4.792493313604505367, 0.000000000000000000 ) ) ;
#107856=CARTESIAN_POINT ( 'NONE',  ( -3.526529353330350336, 7.128384988945109413, -0.7216878364870458196 ) ) ;
#107857=ORIENTED_EDGE ( 'NONE', *, *, #22239, .T. ) ;
#107858=CARTESIAN_POINT ( 'NONE',  ( -6.739811759324840779, 7.035737605399991601, -0.7216878364870338292 ) ) ;
#107859=CARTESIAN_POINT ( 'NONE',  ( 5.580062740476173566, 8.667767742934335828, 1.199719254218451159 ) ) ;
#107861=CARTESIAN_POINT ( 'NONE',  ( -5.010620288702242853, 8.003418215864698482, -1.199719254218453823 ) ) ;
#107882=CARTESIAN_POINT ( 'NONE',  ( 6.770317605177710085, 8.992066187497757213, 1.599625672291268286 ) ) ;
#107888=CARTESIAN_POINT ( 'NONE',  ( -2.972980823146582186, 6.690504403638126263, 0.000000000000000000 ) ) ;
#107890=AXIS2_PLACEMENT_3D ( 'NONE', #117969, #147223, #99526 ) ;
#107913=CARTESIAN_POINT ( 'NONE',  ( -1.913245249192567110, 8.998828458478531189, -0.7749999999999996891 ) ) ;
#107921=CARTESIAN_POINT ( 'NONE',  ( 4.050854035433010480, 7.948023151305657841, 0.000000000000000000 ) ) ;
#107924=CARTESIAN_POINT ( 'NONE',  ( -4.167152111353897403, 5.955039778036558040, 1.599625672291270506 ) ) ;
#107927=CARTESIAN_POINT ( 'NONE',  ( -6.089020385868862739, 8.197219431637373432, -1.443375672974066548 ) ) ;
#107938=CARTESIAN_POINT ( 'NONE',  ( 4.167152111353856547, 5.955039778036558040, 1.599625672291262513 ) ) ;
#107939=CARTESIAN_POINT ( 'NONE',  ( 6.638652492546827766, 7.774124658506663010, 1.199719254218452047 ) ) ;
#107943=EDGE_LOOP ( 'NONE', ( #194964, #204189, #211346, #7404, #4193 ) ) ;
#107949=CARTESIAN_POINT ( 'NONE',  ( 6.384963997392946844, 6.413822516572072807, 0.7998128361456352531 ) ) ;
#107960=CARTESIAN_POINT ( 'NONE',  ( 5.383996398402570271, 9.295429874862735531, 0.000000000000000000 ) ) ;
#107961=CARTESIAN_POINT ( 'NONE',  ( -4.095971805104331231, 5.871996087412059140, 1.443375672974065660 ) ) ;
#107962=CARTESIAN_POINT ( 'NONE',  ( -7.598418745816086783, 7.829519723065708092, 0.000000000000000000 ) ) ;
#107972=CARTESIAN_POINT ( 'NONE',  ( 7.503511670520385479, 7.718794801887437274, 0.7998128361456281477 ) ) ;
#107973=CARTESIAN_POINT ( 'NONE',  ( 5.987861119090863049, 7.014868056141362551, 1.199719254218452047 ) ) ;
#107974=CARTESIAN_POINT ( 'NONE',  ( 7.537407054554579489, 7.758339416593960536, 0.000000000000000000 ) ) ;
#107977=CARTESIAN_POINT ( 'NONE',  ( 7.526711554241970248, 8.810193563817646734, -1.199719254218452047 ) ) ;
#107982=CARTESIAN_POINT ( 'NONE',  ( 7.065207446497155708, 9.336104335703744539, 0.000000000000000000 ) ) ;
#107997=CARTESIAN_POINT ( 'NONE',  ( 4.386945222473598527, 7.275797305264619652, -1.199719254218452047 ) ) ;
#107999=CARTESIAN_POINT ( 'NONE',  ( -2.844178363816758814, 6.540234867753325076, -0.7998128361456481317 ) ) ;
#108001=CARTESIAN_POINT ( 'NONE',  ( 4.037295881819344956, 7.932205305423046582, -0.7998128361456362523 ) ) ;
#108006=CARTESIAN_POINT ( 'NONE',  ( 3.923105346307896202, 5.670318552149568703, -1.599625672291269396 ) ) ;
#108011=CARTESIAN_POINT ( 'NONE',  ( 4.882344714696929877, 8.710169577206153591, -0.7216878364870458196 ) ) ;
#108013=CARTESIAN_POINT ( 'NONE',  ( -4.281342646865346602, 8.216926531310035031, 0.7998128361456352531 ) ) ;
#108014=CARTESIAN_POINT ( 'NONE',  ( 5.876533236880477240, 5.820653295974182129, 0.7998128361456352531 ) ) ;
#108024=CARTESIAN_POINT ( 'NONE',  ( -3.474632506852224356, 7.275764701294714420, -0.7998128361456481317 ) ) ;
#108044=DIRECTION ( 'NONE',  ( -1.000000000000000000, 0.000000000000000000, 0.000000000000000000 ) ) ;
#108055=CARTESIAN_POINT ( 'NONE',  ( 3.255366281057017197, 6.812028071292901998, -0.7216878364870338292 ) ) ;
#108061=CARTESIAN_POINT ( 'NONE',  ( 5.383996397958233260, 5.453953017138946535, -0.7216878364870458196 ) ) ;
#108071=CARTESIAN_POINT ( 'NONE',  ( -6.123442655227560927, 7.173046514967467147, 1.199719254218452047 ) ) ;
#108073=CARTESIAN_POINT ( 'NONE',  ( 7.810905894804431426, 8.285347430126213553, 0.000000000000000000 ) ) ;
#108083=CARTESIAN_POINT ( 'NONE',  ( -4.716257332707368910, 6.595662536282280719, -1.599625672291271394 ) ) ;
#108089=CARTESIAN_POINT ( 'NONE',  ( -3.187575512988701565, 6.732938841879847480, 0.000000000000000000 ) ) ;
#108093=CARTESIAN_POINT ( 'NONE',  ( -3.447516199624892419, 7.244129009529488350, 0.7998128361456352531 ) ) ;
#108116=CARTESIAN_POINT ( 'NONE',  ( -6.631873415740034083, 7.766215735565355160, 1.199719254218452047 ) ) ;
#108119=CARTESIAN_POINT ( 'NONE',  ( -4.468294144155606773, 7.370704380560280100, 1.199719254218452935 ) ) ;
#108146=CARTESIAN_POINT ( 'NONE',  ( -4.793689830883590020, 7.750332681742931662, 1.199719254218452935 ) ) ;
#108171=CARTESIAN_POINT ( 'NONE',  ( 6.176621499477501054, 9.363752961769195693, -1.199719254218452047 ) ) ;
#108173=CARTESIAN_POINT ( 'NONE',  ( 4.532168488718122390, 8.509556680138327778, 0.7998128361456271485 ) ) ;
#108187=CARTESIAN_POINT ( 'NONE',  ( 6.467812791377033577, 6.763347601114057639, -0.2696018389747659172 ) ) ;
#108189=CARTESIAN_POINT ( 'NONE',  ( 6.563555762791525972, 6.830105609444471426, -0.7216878364870458196 ) ) ;
#108194=AXIS2_PLACEMENT_3D ( 'NONE', #116427, #131607, #98015 ) ;
#108208=CARTESIAN_POINT ( 'NONE',  ( -6.170369307550858551, 8.292126506933035657, 1.443375672974058777 ) ) ;
#108209=DIRECTION ( 'NONE',  ( 1.000000000000000000, 0.000000000000000000, 0.000000000000000000 ) ) ;
#108212=CARTESIAN_POINT ( 'NONE',  ( 7.126746022638799971, 8.343567110280638133, 1.199719254218452047 ) ) ;
#108213=CARTESIAN_POINT ( 'NONE',  ( -4.044020806407789159, 7.347651935747151697, -0.7679206946173640080 ) ) ;
#108217=CARTESIAN_POINT ( 'NONE',  ( -3.298376509874564988, 7.070132704820777825, 0.000000000000000000 ) ) ;
#108226=CARTESIAN_POINT ( 'NONE',  ( 5.820193082016415609, 10.01225203898631655, 0.000000000000000000 ) ) ;
#108234=AXIS2_PLACEMENT_3D ( 'NONE', #65786, #83129, #30133 ) ;
#108245=CARTESIAN_POINT ( 'NONE',  ( -5.912237504011027767, 9.055304967058290799, 1.199719254218454489 ) ) ;
#108251=CARTESIAN_POINT ( 'NONE',  ( -6.466610638350029916, 6.780223854948245865, 0.3187201834274414058 ) ) ;
#108265=VECTOR ( 'NONE', #44609, 1000.000000000000000 ) ;
#108268=CARTESIAN_POINT ( 'NONE',  ( 6.211043768836181478, 7.379210830797944709, 1.082531754730549967 ) ) ;
#108279=CARTESIAN_POINT ( 'NONE',  ( -5.180624094197616714, 5.216685329418210948, 0.7216878364870257245 ) ) ;
#108311=CARTESIAN_POINT ( 'NONE',  ( 3.379725431556547477, 7.165039780116438273, -1.734723475976807094E-15 ) ) ;
#108323=CARTESIAN_POINT ( 'NONE',  ( -6.509323148336870091, 7.727203440215372865, 1.082531754730549078 ) ) ;
#108325=CARTESIAN_POINT ( 'NONE',  ( 3.729901657090948230, 6.405283462364505631, 1.082531754730549078 ) ) ;
#108335=CARTESIAN_POINT ( 'NONE',  ( 4.318600669050608687, 4.999583595936801572, -2.419999999999996820 ) ) ;
#108336=CIRCLE ( 'NONE', #11318, 0.8299999999999999600 ) ;
#108343=CARTESIAN_POINT ( 'NONE',  ( -5.004368097219957789, 5.011053332944274352, 0.000000000000000000 ) ) ;
#108372=CARTESIAN_POINT ( 'NONE',  ( -7.553827861469316396, 8.841829255582865699, -1.199719254218452047 ) ) ;
#108375=CARTESIAN_POINT ( 'NONE',  ( -7.096767062110449942, 7.244259425409119046, -0.7998128361456362523 ) ) ;
#108376=CARTESIAN_POINT ( 'NONE',  ( -5.926849427829407269, 6.943687749669614995, -1.199719254218453823 ) ) ;
#108380=CARTESIAN_POINT ( 'NONE',  ( -7.580417283372126391, 8.016444050121833698, 0.7216878364870317197 ) ) ;
#108385=ORIENTED_EDGE ( 'NONE', *, *, #47358, .T. ) ;
#108386=CARTESIAN_POINT ( 'NONE',  ( -6.050681693448748177, 10.28115541899069463, 0.7998128361456291469 ) ) ;
#108393=ADVANCED_FACE ( 'NONE', ( #70971 ), #128734, .T. ) ;
#108397=CARTESIAN_POINT ( 'NONE',  ( 4.913571454530422322, 8.125067815752732514, -1.031885869761673069 ) ) ;
#108401=CARTESIAN_POINT ( 'NONE',  ( 4.248501033035879004, 6.049946853332221153, -1.599625672291273171 ) ) ;
#108407=LINE ( 'NONE', #94246, #166789 ) ;
#108428=CARTESIAN_POINT ( 'NONE',  ( 4.435452530326143616, 5.203724702582467998, -1.199719254218452047 ) ) ;
#108439=CARTESIAN_POINT ( 'NONE',  ( -1.930226670627066099, 8.999999999999998224, -0.7749999999999996891 ) ) ;
#108443=CARTESIAN_POINT ( 'NONE',  ( 6.231590709102786008, 7.018523052454695765, 1.002697108273574500 ) ) ;
#108444=CARTESIAN_POINT ( 'NONE',  ( -5.438229012412911345, 5.517224400669388018, -0.7216878364870338292 ) ) ;
#108471=CARTESIAN_POINT ( 'NONE',  ( 4.848976215542928792, 5.686169002002086970, 1.199719254218452047 ) ) ;
#108490=CARTESIAN_POINT ( 'NONE',  ( -6.414942957921379474, 7.513130201443591005, -1.199719254218452047 ) ) ;
#108505=CARTESIAN_POINT ( 'NONE',  ( 5.896870467300973750, 5.844380064798101237, 0.7998128361456352531 ) ) ;
#108512=CARTESIAN_POINT ( 'NONE',  ( 4.831967907651305794, 8.093680561842322874, 0.8807274918286764898 ) ) ;
#108514=CARTESIAN_POINT ( 'NONE',  ( 5.510920874727778696, 7.454463421478725316, 1.249874847645112697 ) ) ;
#108533=CARTESIAN_POINT ( 'NONE',  ( -4.630991987519598396, 7.560518531151607213, 1.199719254218452935 ) ) ;
#108535=CARTESIAN_POINT ( 'NONE',  ( 4.329849954717849947, 6.144853928627882489, 1.599625672291262513 ) ) ;
#108538=CARTESIAN_POINT ( 'NONE',  ( -5.074494633264801990, 9.142270515442742607, 0.7998128361456291469 ) ) ;
#108545=CARTESIAN_POINT ( 'NONE',  ( -5.730308518391983519, 7.387375129167091714, -1.324551712912255486 ) ) ;
#108550=EDGE_CURVE ( 'NONE', #71711, #81797, #115935, .T. ) ;
#108565=CARTESIAN_POINT ( 'NONE',  ( 5.722950238744209273, 6.809768379023969587, 1.082531754730549967 ) ) ;
#108569=CARTESIAN_POINT ( 'NONE',  ( -6.774234028683526532, 7.932303117332766718, 1.199719254218452047 ) ) ;
#108579=CARTESIAN_POINT ( 'NONE',  ( -3.201133666602369310, 6.748756687762456963, -0.7216878364870458196 ) ) ;
#108584=CARTESIAN_POINT ( 'NONE',  ( 5.761288931164342486, 5.686201605971993978, -0.7998128361456481317 ) ) ;
#108608=CARTESIAN_POINT ( 'NONE',  ( -5.064290697676250730, 7.960144884870772763, -1.236948567437242907 ) ) ;
#108610=CARTESIAN_POINT ( 'NONE',  ( -4.340018570150306232, 8.077455741901736985, -0.7216878364870338292 ) ) ;
#108635=CARTESIAN_POINT ( 'NONE',  ( -2.984203208339354152, 6.495671153122273722, 0.000000000000000000 ) ) ;
#108641=CARTESIAN_POINT ( 'NONE',  ( -4.821859908315634158, 5.654533310236863564, 1.199719254218452935 ) ) ;
#108645=VERTEX_POINT ( 'NONE', #205555 ) ;
#108650=CARTESIAN_POINT ( 'NONE',  ( -3.709037541790315640, 6.484905011134099340, -1.199719254218450271 ) ) ;
#108652=CARTESIAN_POINT ( 'NONE',  ( 6.489313741793890422, 6.842916442627623219, -0.5960428994750706089 ) ) ;
#108656=CARTESIAN_POINT ( 'NONE',  ( 4.366607992053101128, 7.252070536440704096, -1.199719254218448494 ) ) ;
#108661=CARTESIAN_POINT ( 'NONE',  ( -6.912678218121246942, 9.158153569265168770, 1.599625672291269396 ) ) ;
#108664=CARTESIAN_POINT ( 'NONE',  ( -6.283277845290492714, 6.295188672452495915, -0.7998128361456362523 ) ) ;
#108671=CARTESIAN_POINT ( 'NONE',  ( 5.031484404002879884, 6.963427452793765404, 1.443375672974065660 ) ) ;
#108672=CARTESIAN_POINT ( 'NONE',  ( -5.519577934094894722, 7.532869904567736974, 1.443375672974058777 ) ) ;
#108679=CARTESIAN_POINT ( 'NONE',  ( 3.393283585170187688, 7.180857625999046867, 0.7998128361456271485 ) ) ;
#108687=CARTESIAN_POINT ( 'NONE',  ( 4.908934136599710563, 7.884784371745123366, 1.199719254218451159 ) ) ;
#108688=ADVANCED_FACE ( 'NONE', ( #72351 ), #46677, .T. ) ;
#108711=CARTESIAN_POINT ( 'NONE',  ( 4.816695983655697511, 8.110494931179941247, 0.8576603160085185529 ) ) ;
#108720=CARTESIAN_POINT ( 'NONE',  ( 6.749980374757213575, 8.968339418673846097, 1.599625672291268286 ) ) ;
#108725=CARTESIAN_POINT ( 'NONE',  ( -4.844715248835366417, 8.098060037232425401, 0.8884674472836263659 ) ) ;
#108732=CARTESIAN_POINT ( 'NONE',  ( -6.312203035614172286, 9.521931420595302953, -1.199719254218452047 ) ) ;
#108745=CARTESIAN_POINT ( 'NONE',  ( 6.770317605177710085, 8.992066187497757213, 1.599625672291268286 ) ) ;
#108749=( BOUNDED_SURFACE ( )  B_SPLINE_SURFACE ( 1, 2, ( 
 ( #39858, #186084, #168777, #188218, #38784, #169843, #156815, #87538, #105967, #71253, #103793, #8402, #74487, #21430, #139504, #121186, #171989, #23581, #189294, #42010, #20382, #137367, #120105, #187155, #104865, #89688, #155739, #40934, #7324, #140593, #73401, #86466, #57168, #206604, #152530, #59292, #176262, #157887, #145918, #77676, #110253, #27863, #210867, #143797, #211930, #95021, #44132, #61429, #194623, #127596, #28937, #192480, #177323, #111319, #62492, #93960, #209794, #161071, #195705, #11602, #142720, #79806, #109193, #9479, #12662, #25719, #160001, #78736, #43080, #175205, #46266, #96091, #174146, #193562, #144860, #162146, #158937, #92892, #63564, #128657, #26787, #112383, #108119, #125451, #207673, #178395, #30007, #13733, #10533, #76606, #129721, #91828, #45205, #75551, #141662, #191413, #208729, #60356, #126519, #97156, #32133, #80884, #115567, #183701, #163211, #116632, #47340, #151222, #113454, #68862, #180513, #649, #131807, #117710, #84068, #182626, #165322, #134981, #14793, #49448, #82996, #197816, #66714, #17980, #181563, #146974, #212991, #132858, #198863, #33191, #149071, #31083, #101386, #99274, #167461, #98214, #150157, #1726, #35309, #65659, #130768, #16916, #50510, #19056, #34249, #48406, #64629, #196763, #114518, #164265, #2790, #15854, #100322, #166388, #81940, #148024, #199938, #67783, #214034, #133933, #51585, #85135, #179459, #52637, #53707, #70990, #87273, #153341, #121994, #105690, #200991, #5991, #139236, #119840, #170650, #169587, #185819, #136034, #54774, #187960, #152277, #4913, #39588, #120921, #21170, #72062, #37450, #7059, #138172, #103528, #137103, #203132, #186894, #69923, #86205, #204182, #55838, #38526, #118765, #36378, #22237, #171718, #23317, #184750, #104603, #88348, #154412, #89425, #155476, #202047, #102455, #205267, #73132, #168521, #20120, #3850, #134623, #83692, #52275, #15484, #281, #65295, #117334, #33880, #200628, #131442, #50142, #118402, #149780, #66353, #167098, #32824, #85837, #18687, #98899, #82626, #132497, #164953, #49086, #213671, #150855 ),
 ( #148712, #2419, #151915, #183333, #184388, #84769, #197445, #68496, #1355, #102088, #166022, #115204, #168157, #36007, #67417, #51211, #199567, #182255, #133558, #19756, #16545, #99957, #53335, #31773, #3488, #201690, #181196, #69558, #34937, #135668, #180147, #97843, #163908, #81570, #147655, #198497, #116264, #101009, #17607, #204892, #136734, #119468, #187594, #203825, #120551, #123769, #38159, #171349, #104232, #202758, #173518, #57609, #186529, #90122, #154045, #22942, #39219, #73855, #74924, #8846, #170278, #20810, #54411, #152974, #89058, #21864, #139950, #155115, #189729, #6699, #185456, #121625, #105311, #41382, #70620, #72775, #169218, #157253, #138874, #56543, #122705, #7766, #188669, #141037, #106409, #55469, #40299, #205976, #172432, #24020, #156189, #107492, #25092, #91192, #207044, #37078, #103157, #86906, #4547, #5610, #87972, #71693, #137806, #2042, #37783, #36701, #8208, #182956, #167783, #18310, #70252, #201317, #102786, #152595, #118030, #34571, #184016, #166719, #52957, #58032, #100643, #202385, #133183, #25525, #199183, #157685, #51907, #86529, #3112, #206407, #169907, #54035, #168844, #9283, #84395, #135304, #20447, #69183, #4181, #103857, #119095, #150482, #68112, #136365, #120172, #185075, #186149, #116957, #190159, #21494, #41814, #35633, #90555, #156618, #124196, #151545, #134249, #74293, #140388, #107927, #173951, #200255, #101710, #19379, #85459, #91633, #50830, #142517, #78543, #194430, #110053, #108987, #13543, #178197, #191216, #76408, #46071, #43938, #47142, #141468, #126317, #61235, #77478, #143597, #95898, #211732, #75355, #210675, #179264, #60162, #160874, #176066, #208526, #10334, #193363, #161951, #175006, #159797, #79613, #45008, #27663, #62303, #192277, #195506, #128462, #93758, #11400, #209589, #127390, #158739, #26592, #112192, #29813, #111118, #207476, #59095, #28738, #145732, #63370, #96965, #177121, #94823, #12468, #144660, #129526, #92693, #113259, #30887, #163013, #125255, #42879, #48212, #167272, #117511, #130580, #15661, #199744, #197617, #200799, #80692, #65467 ) ),
 .UNSPECIFIED., .F., .F., .F. ) 
 B_SPLINE_SURFACE_WITH_KNOTS ( ( 2, 2 ),
 ( 3, 2, 2, 2, 2, 2, 2, 2, 2, 2, 2, 2, 2, 2, 2, 2, 2, 2, 2, 2, 2, 2, 2, 2, 2, 2, 2, 2, 2, 2, 2, 2, 2, 2, 2, 2, 2, 2, 2, 2, 2, 2, 2, 2, 2, 2, 2, 2, 2, 2, 2, 2, 2, 2, 2, 2, 2, 2, 2, 2, 2, 2, 2, 2, 2, 2, 2, 2, 2, 2, 2, 2, 2, 2, 2, 2, 2, 2, 2, 2, 2, 2, 2, 2, 2, 2, 2, 2, 2, 2, 2, 2, 2, 2, 2, 2, 2, 2, 2, 2, 2, 2, 2, 2, 2, 2, 2, 2, 2, 2, 2, 2, 2, 2, 2, 2, 2, 2, 2, 2, 3 ),
 ( 0.000000000000000000, 1.000000000000000000 ),
 ( 0.000000000000000000, 0.008333333333333333218, 0.01666666666666666644, 0.02500000000000000139, 0.03333333333333333287, 0.04166666666666666435, 0.05000000000000000278, 0.05833333333333333426, 0.06666666666666666574, 0.07499999999999999722, 0.08333333333333332871, 0.09166666666666666019, 0.1000000000000000056, 0.1083333333333333370, 0.1166666666666666685, 0.1250000000000000000, 0.1333333333333333315, 0.1416666666666666630, 0.1499999999999999944, 0.1583333333333333259, 0.1666666666666666574, 0.1749999999999999889, 0.1833333333333333204, 0.1916666666666666796, 0.2000000000000000111, 0.2083333333333333426, 0.2166666666666666741, 0.2250000000000000056, 0.2333333333333333370, 0.2416666666666666685, 0.2500000000000000000, 0.2583333333333333592, 0.2666666666666666630, 0.2750000000000000222, 0.2833333333333333259, 0.2916666666666666852, 0.2999999999999999889, 0.3083333333333333481, 0.3166666666666666519, 0.3250000000000000111, 0.3333333333333333148, 0.3416666666666666741, 0.3499999999999999778, 0.3583333333333333370, 0.3666666666666666408, 0.3750000000000000000, 0.3833333333333333592, 0.3916666666666666630, 0.4000000000000000222, 0.4083333333333333259, 0.4166666666666666852, 0.4249999999999999889, 0.4333333333333333481, 0.4416666666666666519, 0.4500000000000000111, 0.4583333333333333148, 0.4666666666666666741, 0.4749999999999999778, 0.4833333333333333370, 0.4916666666666666408, 0.5000000000000000000, 0.5083333333333333037, 0.5166666666666667185, 0.5250000000000000222, 0.5333333333333333259, 0.5416666666666666297, 0.5500000000000000444, 0.5583333333333333481, 0.5666666666666666519, 0.5749999999999999556, 0.5833333333333333703, 0.5916666666666666741, 0.5999999999999999778, 0.6083333333333332815, 0.6166666666666666963, 0.6250000000000000000, 0.6333333333333333037, 0.6416666666666667185, 0.6500000000000000222, 0.6583333333333333259, 0.6666666666666666297, 0.6750000000000000444, 0.6833333333333333481, 0.6916666666666666519, 0.6999999999999999556, 0.7083333333333333703, 0.7166666666666666741, 0.7249999999999999778, 0.7333333333333332815, 0.7416666666666666963, 0.7500000000000000000, 0.7583333333333333037, 0.7666666666666667185, 0.7750000000000000222, 0.7833333333333333259, 0.7916666666666666297, 0.8000000000000000444, 0.8083333333333333481, 0.8166666666666666519, 0.8249999999999999556, 0.8333333333333333703, 0.8416666666666666741, 0.8499999999999999778, 0.8583333333333332815, 0.8666666666666666963, 0.8750000000000000000, 0.8833333333333333037, 0.8916666666666667185, 0.9000000000000000222, 0.9083333333333333259, 0.9166666666666666297, 0.9250000000000000444, 0.9333333333333333481, 0.9416666666666666519, 0.9499999999999999556, 0.9583333333333333703, 0.9666666666666666741, 0.9749999999999999778, 0.9833333333333332815, 0.9916666666666666963, 1.000000000000000000 ),
 .UNSPECIFIED. ) 
 GEOMETRIC_REPRESENTATION_ITEM ( )  RATIONAL_B_SPLINE_SURFACE ( (
 ( 1.000000000000000000, 0.8660254037844387076, 1.000000000000000000, 0.8660254037844387076, 1.000000000000000000, 0.8660254037844387076, 1.000000000000000000, 0.8660254037844387076, 1.000000000000000000, 0.8660254037844387076, 1.000000000000000000, 0.8660254037844387076, 1.000000000000000000, 0.8660254037844387076, 1.000000000000000000, 0.8660254037844387076, 1.000000000000000000, 0.8660254037844387076, 1.000000000000000000, 0.8660254037844387076, 1.000000000000000000, 0.8660254037844387076, 1.000000000000000000, 0.8660254037844387076, 1.000000000000000000, 0.8660254037844387076, 1.000000000000000000, 0.8660254037844387076, 1.000000000000000000, 0.8660254037844387076, 1.000000000000000000, 0.8660254037844387076, 1.000000000000000000, 0.8660254037844387076, 1.000000000000000000, 0.8660254037844387076, 1.000000000000000000, 0.8660254037844387076, 1.000000000000000000, 0.8660254037844387076, 1.000000000000000000, 0.8660254037844387076, 1.000000000000000000, 0.8660254037844387076, 1.000000000000000000, 0.8660254037844387076, 1.000000000000000000, 0.8660254037844387076, 1.000000000000000000, 0.8660254037844387076, 1.000000000000000000, 0.8660254037844387076, 1.000000000000000000, 0.8660254037844387076, 1.000000000000000000, 0.8660254037844387076, 1.000000000000000000, 0.8660254037844387076, 1.000000000000000000, 0.8660254037844387076, 1.000000000000000000, 0.8660254037844387076, 1.000000000000000000, 0.8660254037844387076, 1.000000000000000000, 0.8660254037844387076, 1.000000000000000000, 0.8660254037844387076, 1.000000000000000000, 0.8660254037844387076, 1.000000000000000000, 0.8660254037844387076, 1.000000000000000000, 0.8660254037844387076, 1.000000000000000000, 0.8660254037844387076, 1.000000000000000000, 0.8660254037844387076, 1.000000000000000000, 0.8660254037844387076, 1.000000000000000000, 0.8660254037844387076, 1.000000000000000000, 0.8660254037844387076, 1.000000000000000000, 0.8660254037844387076, 1.000000000000000000, 0.8660254037844387076, 1.000000000000000000, 0.8660254037844387076, 1.000000000000000000, 0.8660254037844387076, 1.000000000000000000, 0.8660254037844387076, 1.000000000000000000, 0.8660254037844387076, 1.000000000000000000, 0.8660254037844387076, 1.000000000000000000, 0.8660254037844387076, 1.000000000000000000, 0.8660254037844387076, 1.000000000000000000, 0.8660254037844387076, 1.000000000000000000, 0.8660254037844387076, 1.000000000000000000, 0.8660254037844387076, 1.000000000000000000, 0.8660254037844387076, 1.000000000000000000, 0.8660254037844387076, 1.000000000000000000, 0.8660254037844387076, 1.000000000000000000, 0.8660254037844387076, 1.000000000000000000, 0.8660254037844387076, 1.000000000000000000, 0.8660254037844387076, 1.000000000000000000, 0.8660254037844387076, 1.000000000000000000, 0.8660254037844387076, 1.000000000000000000, 0.8660254037844387076, 1.000000000000000000, 0.8660254037844387076, 1.000000000000000000, 0.8660254037844387076, 1.000000000000000000, 0.8660254037844387076, 1.000000000000000000, 0.8660254037844387076, 1.000000000000000000, 0.8660254037844387076, 1.000000000000000000, 0.8660254037844387076, 1.000000000000000000, 0.8660254037844387076, 1.000000000000000000, 0.8660254037844387076, 1.000000000000000000, 0.8660254037844387076, 1.000000000000000000, 0.8660254037844387076, 1.000000000000000000, 0.8660254037844387076, 1.000000000000000000, 0.8660254037844387076, 1.000000000000000000, 0.8660254037844387076, 1.000000000000000000, 0.8660254037844387076, 1.000000000000000000, 0.8660254037844387076, 1.000000000000000000, 0.8660254037844387076, 1.000000000000000000, 0.8660254037844387076, 1.000000000000000000, 0.8660254037844387076, 1.000000000000000000, 0.8660254037844387076, 1.000000000000000000, 0.8660254037844387076, 1.000000000000000000, 0.8660254037844387076, 1.000000000000000000, 0.8660254037844387076, 1.000000000000000000, 0.8660254037844387076, 1.000000000000000000, 0.8660254037844387076, 1.000000000000000000, 0.8660254037844387076, 1.000000000000000000, 0.8660254037844387076, 1.000000000000000000, 0.8660254037844387076, 1.000000000000000000, 0.8660254037844387076, 1.000000000000000000, 0.8660254037844387076, 1.000000000000000000, 0.8660254037844387076, 1.000000000000000000, 0.8660254037844387076, 1.000000000000000000, 0.8660254037844387076, 1.000000000000000000, 0.8660254037844387076, 1.000000000000000000, 0.8660254037844387076, 1.000000000000000000, 0.8660254037844387076, 1.000000000000000000, 0.8660254037844387076, 1.000000000000000000, 0.8660254037844387076, 1.000000000000000000, 0.8660254037844387076, 1.000000000000000000, 0.8660254037844387076, 1.000000000000000000, 0.8660254037844387076, 1.000000000000000000, 0.8660254037844387076, 1.000000000000000000, 0.8660254037844387076, 1.000000000000000000, 0.8660254037844387076, 1.000000000000000000, 0.8660254037844387076, 1.000000000000000000, 0.8660254037844387076, 1.000000000000000000, 0.8660254037844387076, 1.000000000000000000, 0.8660254037844387076, 1.000000000000000000, 0.8660254037844387076, 1.000000000000000000, 0.8660254037844387076, 1.000000000000000000, 0.8660254037844387076, 1.000000000000000000, 0.8660254037844387076, 1.000000000000000000, 0.8660254037844387076, 1.000000000000000000, 0.8660254037844387076, 1.000000000000000000, 0.8660254037844387076, 1.000000000000000000, 0.8660254037844387076, 1.000000000000000000, 0.8660254037844387076, 1.000000000000000000, 0.8660254037844387076, 1.000000000000000000),
 ( 1.000000000000000000, 0.8660254037844387076, 1.000000000000000000, 0.8660254037844387076, 1.000000000000000000, 0.8660254037844387076, 1.000000000000000000, 0.8660254037844387076, 1.000000000000000000, 0.8660254037844387076, 1.000000000000000000, 0.8660254037844387076, 1.000000000000000000, 0.8660254037844387076, 1.000000000000000000, 0.8660254037844387076, 1.000000000000000000, 0.8660254037844387076, 1.000000000000000000, 0.8660254037844387076, 1.000000000000000000, 0.8660254037844387076, 1.000000000000000000, 0.8660254037844387076, 1.000000000000000000, 0.8660254037844387076, 1.000000000000000000, 0.8660254037844387076, 1.000000000000000000, 0.8660254037844387076, 1.000000000000000000, 0.8660254037844387076, 1.000000000000000000, 0.8660254037844387076, 1.000000000000000000, 0.8660254037844387076, 1.000000000000000000, 0.8660254037844387076, 1.000000000000000000, 0.8660254037844387076, 1.000000000000000000, 0.8660254037844387076, 1.000000000000000000, 0.8660254037844387076, 1.000000000000000000, 0.8660254037844387076, 1.000000000000000000, 0.8660254037844387076, 1.000000000000000000, 0.8660254037844387076, 1.000000000000000000, 0.8660254037844387076, 1.000000000000000000, 0.8660254037844387076, 1.000000000000000000, 0.8660254037844387076, 1.000000000000000000, 0.8660254037844387076, 1.000000000000000000, 0.8660254037844387076, 1.000000000000000000, 0.8660254037844387076, 1.000000000000000000, 0.8660254037844387076, 1.000000000000000000, 0.8660254037844387076, 1.000000000000000000, 0.8660254037844387076, 1.000000000000000000, 0.8660254037844387076, 1.000000000000000000, 0.8660254037844387076, 1.000000000000000000, 0.8660254037844387076, 1.000000000000000000, 0.8660254037844387076, 1.000000000000000000, 0.8660254037844387076, 1.000000000000000000, 0.8660254037844387076, 1.000000000000000000, 0.8660254037844387076, 1.000000000000000000, 0.8660254037844387076, 1.000000000000000000, 0.8660254037844387076, 1.000000000000000000, 0.8660254037844387076, 1.000000000000000000, 0.8660254037844387076, 1.000000000000000000, 0.8660254037844387076, 1.000000000000000000, 0.8660254037844387076, 1.000000000000000000, 0.8660254037844387076, 1.000000000000000000, 0.8660254037844387076, 1.000000000000000000, 0.8660254037844387076, 1.000000000000000000, 0.8660254037844387076, 1.000000000000000000, 0.8660254037844387076, 1.000000000000000000, 0.8660254037844387076, 1.000000000000000000, 0.8660254037844387076, 1.000000000000000000, 0.8660254037844387076, 1.000000000000000000, 0.8660254037844387076, 1.000000000000000000, 0.8660254037844387076, 1.000000000000000000, 0.8660254037844387076, 1.000000000000000000, 0.8660254037844387076, 1.000000000000000000, 0.8660254037844387076, 1.000000000000000000, 0.8660254037844387076, 1.000000000000000000, 0.8660254037844387076, 1.000000000000000000, 0.8660254037844387076, 1.000000000000000000, 0.8660254037844387076, 1.000000000000000000, 0.8660254037844387076, 1.000000000000000000, 0.8660254037844387076, 1.000000000000000000, 0.8660254037844387076, 1.000000000000000000, 0.8660254037844387076, 1.000000000000000000, 0.8660254037844387076, 1.000000000000000000, 0.8660254037844387076, 1.000000000000000000, 0.8660254037844387076, 1.000000000000000000, 0.8660254037844387076, 1.000000000000000000, 0.8660254037844387076, 1.000000000000000000, 0.8660254037844387076, 1.000000000000000000, 0.8660254037844387076, 1.000000000000000000, 0.8660254037844387076, 1.000000000000000000, 0.8660254037844387076, 1.000000000000000000, 0.8660254037844387076, 1.000000000000000000, 0.8660254037844387076, 1.000000000000000000, 0.8660254037844387076, 1.000000000000000000, 0.8660254037844387076, 1.000000000000000000, 0.8660254037844387076, 1.000000000000000000, 0.8660254037844387076, 1.000000000000000000, 0.8660254037844387076, 1.000000000000000000, 0.8660254037844387076, 1.000000000000000000, 0.8660254037844387076, 1.000000000000000000, 0.8660254037844387076, 1.000000000000000000, 0.8660254037844387076, 1.000000000000000000, 0.8660254037844387076, 1.000000000000000000, 0.8660254037844387076, 1.000000000000000000, 0.8660254037844387076, 1.000000000000000000, 0.8660254037844387076, 1.000000000000000000, 0.8660254037844387076, 1.000000000000000000, 0.8660254037844387076, 1.000000000000000000, 0.8660254037844387076, 1.000000000000000000, 0.8660254037844387076, 1.000000000000000000, 0.8660254037844387076, 1.000000000000000000, 0.8660254037844387076, 1.000000000000000000, 0.8660254037844387076, 1.000000000000000000, 0.8660254037844387076, 1.000000000000000000, 0.8660254037844387076, 1.000000000000000000, 0.8660254037844387076, 1.000000000000000000, 0.8660254037844387076, 1.000000000000000000, 0.8660254037844387076, 1.000000000000000000, 0.8660254037844387076, 1.000000000000000000, 0.8660254037844387076, 1.000000000000000000, 0.8660254037844387076, 1.000000000000000000, 0.8660254037844387076, 1.000000000000000000, 0.8660254037844387076, 1.000000000000000000, 0.8660254037844387076, 1.000000000000000000, 0.8660254037844387076, 1.000000000000000000, 0.8660254037844387076, 1.000000000000000000, 0.8660254037844387076, 1.000000000000000000, 0.8660254037844387076, 1.000000000000000000, 0.8660254037844387076, 1.000000000000000000, 0.8660254037844387076, 1.000000000000000000, 0.8660254037844387076, 1.000000000000000000, 0.8660254037844387076, 1.000000000000000000, 0.8660254037844387076, 1.000000000000000000, 0.8660254037844387076, 1.000000000000000000) ) ) 
 REPRESENTATION_ITEM ( '' )  SURFACE ( )  );
#108754=CARTESIAN_POINT ( 'NONE',  ( 3.932747076415766596, 6.745899468197171345, 1.199719254218451159 ) ) ;
#108757=CARTESIAN_POINT ( 'NONE',  ( 4.190878879955609371, 7.903459436674603822, -0.7216878364870338292 ) ) ;
#108758=CARTESIAN_POINT ( 'NONE',  ( 0.08191116107305261573, 2.527130371385647667, -1.998427156035398777 ) ) ;
#108772=CARTESIAN_POINT ( 'NONE',  ( -3.800028193580205382, 7.655393002477360653, -0.7998128361456481317 ) ) ;
#108773=CARTESIAN_POINT ( 'NONE',  ( 6.536439455564155843, 8.719208346281938304, 1.443375672974065660 ) ) ;
#108785=CARTESIAN_POINT ( 'NONE',  ( -5.581116510680924847, 6.540332679663050541, -1.199719254218453823 ) ) ;
#108786=CARTESIAN_POINT ( 'NONE',  ( -4.960304097753355457, 6.880383762169266504, 1.599625672291263179 ) ) ;
#108788=CARTESIAN_POINT ( 'NONE',  ( 6.007671464186812749, 10.02305078494439883, 0.7216878364870317197 ) ) ;
#108800=CARTESIAN_POINT ( 'NONE',  ( -6.152945810502786550, 6.988564382810744213, -0.9301526061148736035 ) ) ;
#108805=CARTESIAN_POINT ( 'NONE',  ( 4.421367491832270957, 6.251624388594711590, 1.443375672974058777 ) ) ;
#108810=CARTESIAN_POINT ( 'NONE',  ( -6.526270840131767059, 8.707344961610770540, -1.599625672291271394 ) ) ;
#108824=CARTESIAN_POINT ( 'NONE',  ( 4.993145711582793744, 9.047363440147082159, -0.7998128361456481317 ) ) ;
#108858=CARTESIAN_POINT ( 'NONE',  ( 7.702440666339465558, 8.158804663583751449, -0.7216878364870317197 ) ) ;
#108864=CARTESIAN_POINT ( 'NONE',  ( 5.343321937117211817, 9.247976336696488886, 0.000000000000000000 ) ) ;
#108891=CARTESIAN_POINT ( 'NONE',  ( -5.330290668828105538, 6.247702530834755130, 1.199719254218452935 ) ) ;
#108893=CARTESIAN_POINT ( 'NONE',  ( 5.682275777458851707, 6.762314840857718501, 1.082531754730549078 ) ) ;
#108898=CARTESIAN_POINT ( 'NONE',  ( -4.685224601974262271, 7.623789914682047808, -1.199719254218453823 ) ) ;
#108903=CARTESIAN_POINT ( 'NONE',  ( -3.984117037569407938, 5.741498858621315371, 1.599625672291270506 ) ) ;
#108905=CARTESIAN_POINT ( 'NONE',  ( -3.853720295264455586, 8.531188044730782849, 2.447541241191873773 ) ) ;
#108911=CARTESIAN_POINT ( 'NONE',  ( -4.502189528189771472, 7.410248995266807803, -1.199719254218453823 ) ) ;
#108919=CARTESIAN_POINT ( 'NONE',  ( -4.767627293860968507, 5.591261926706423857, -1.199719254218453823 ) ) ;
#108923=CARTESIAN_POINT ( 'NONE',  ( -6.482206841109545259, 6.735198534148810090, 0.7216878364870257245 ) ) ;
#108924=CARTESIAN_POINT ( 'NONE',  ( -5.817857313595549584, 6.920493299683823096, 1.082531754730549078 ) ) ;
#108925=CARTESIAN_POINT ( 'NONE',  ( 4.850785098639300408, 8.881276058379668825, -0.7998128361456481317 ) ) ;
#108927=CARTESIAN_POINT ( 'NONE',  ( -4.620296487206990932, 8.612372678375294299, 0.000000000000000000 ) ) ;
#108935=ORIENTED_EDGE ( 'NONE', *, *, #30501, .F. ) ;
#108946=CARTESIAN_POINT ( 'NONE',  ( 5.854088466050551887, 10.05179665369283981, 0.7998128361456341429 ) ) ;
#108965=CARTESIAN_POINT ( 'NONE',  ( 5.273189713885392926, 7.658326211947664497, -1.220946906274408494 ) ) ;
#108981=CARTESIAN_POINT ( 'NONE',  ( 5.851225812749518695, 8.984124660586543243, -1.199719254218452047 ) ) ;
#108984=CARTESIAN_POINT ( 'NONE',  ( -3.332271893908731464, 7.109677319527304640, -0.7998128361456481317 ) ) ;
#108987=CARTESIAN_POINT ( 'NONE',  ( -6.251718229232856139, 8.387033582228697881, -1.443375672974066548 ) ) ;
#108988=CARTESIAN_POINT ( 'NONE',  ( 4.934241560730721510, 4.721313007132757811, 0.000000000000000000 ) ) ;
#108999=CARTESIAN_POINT ( 'NONE',  ( 7.991605200612358573, 8.288237253661408843, 0.7998128361456281477 ) ) ;
#109000=CARTESIAN_POINT ( 'NONE',  ( 6.378184920586140727, 6.405913593630768510, 0.000000000000000000 ) ) ;
#109013=CARTESIAN_POINT ( 'NONE',  ( 6.496291879603339758, 7.608037276739255006, 1.199719254218452935 ) ) ;
#109015=CARTESIAN_POINT ( 'NONE',  ( -4.207966135563104615, 7.175396087857926375, -2.420000000000000373 ) ) ;
#109025=CARTESIAN_POINT ( 'NONE',  ( 7.349928672384120176, 7.747540670635879145, 0.7216878364870267237 ) ) ;
#109026=CARTESIAN_POINT ( 'NONE',  ( -4.936577329151611515, 7.813071746435248599, 1.082531754730549967 ) ) ;
#109027=CARTESIAN_POINT ( 'NONE',  ( -5.413448473606448985, 9.537716662508005427, 0.000000000000000000 ) ) ;
#109033=ORIENTED_EDGE ( 'NONE', *, *, #68466, .T. ) ;
#109039=CARTESIAN_POINT ( 'NONE',  ( 6.042093733545556233, 7.078139439671806699, -1.199719254218452047 ) ) ;
#109040=CARTESIAN_POINT ( 'NONE',  ( 6.821687566331318564, 7.987665577921906568, 1.199719254218452935 ) ) ;
#109043=CARTESIAN_POINT ( 'NONE',  ( 5.383996397958233260, 5.453953017138946535, -0.7216878364870458196 ) ) ;
#109062=CARTESIAN_POINT ( 'NONE',  ( 4.450808633097254052, 7.987047222781193057, -2.500000000000000444 ) ) ;
#109064=CARTESIAN_POINT ( 'NONE',  ( 3.901714345682657292, 7.774026846596938434, 0.7998128361456271485 ) ) ;
#109068=CARTESIAN_POINT ( 'NONE',  ( 6.574778147984297938, 6.635272358928617997, -0.7998128361456481317 ) ) ;
#109073=CARTESIAN_POINT ( 'NONE',  ( 7.452141709366786770, 8.723195411463290583, 1.199719254218452047 ) ) ;
#109080=CARTESIAN_POINT ( 'NONE',  ( 6.780486220610169035, 9.003929572168926754, -1.443375672974078761 ) ) ;
#109082=CARTESIAN_POINT ( 'NONE',  ( -6.317173229324657413, 6.334733287159020954, 0.000000000000000000 ) ) ;
#109083=CARTESIAN_POINT ( 'NONE',  ( 5.564695703766185275, 5.456842840674144490, 0.000000000000000000 ) ) ;
#109093=CARTESIAN_POINT ( 'NONE',  ( -4.125423880308188629, 8.035021303660014880, -0.7998128361456481317 ) ) ;
#109111=DIRECTION ( 'NONE',  ( 0.000000000000000000, 0.000000000000000000, -1.000000000000000000 ) ) ;
#109124=B_SPLINE_CURVE_WITH_KNOTS ( 'NONE', 3,
 ( #114794, #127889, #48677, #193840, #46549, #162430, #146196, #115855 ),
 .UNSPECIFIED., .F., .F.,
 ( 4, 2, 2, 4 ),
 ( 0.001893943459172981250, 0.002262838117583250517, 0.002447285446788384933, 0.002631732775993519350 ),
 .UNSPECIFIED. ) ;
#109131=CARTESIAN_POINT ( 'NONE',  ( 4.001064729364292916, 6.721640380016713934, -1.082531754730548412 ) ) ;
#109142=CARTESIAN_POINT ( 'NONE',  ( -4.522526758610270647, 7.433975764090723359, -1.199719254218453823 ) ) ;
#109144=CARTESIAN_POINT ( 'NONE',  ( -6.017840079619296567, 8.114175741012878973, -1.599625672291271394 ) ) ;
#109146=CARTESIAN_POINT ( 'NONE',  ( 6.156811153937166381, 10.19704708965311468, 0.000000000000000000 ) ) ;
#109156=CARTESIAN_POINT ( 'NONE',  ( -6.448838341955544173, 7.552674816150118708, 1.199719254218452047 ) ) ;
#109163=CARTESIAN_POINT ( 'NONE',  ( -4.584065335196305213, 6.441438539186039591, 1.443375672974058777 ) ) ;
#109165=ORIENTED_EDGE ( 'NONE', *, *, #136379, .F. ) ;
#109167=CARTESIAN_POINT ( 'NONE',  ( -5.448397627845328550, 7.449826213943242514, 1.599625672291263179 ) ) ;
#109177=ORIENTED_EDGE ( 'NONE', *, *, #133456, .F. ) ;
#109191=CARTESIAN_POINT ( 'NONE',  ( -4.932134020321308654, 8.976183133675331050, 0.7998128361456291469 ) ) ;
#109193=CARTESIAN_POINT ( 'NONE',  ( -4.197131071882288289, 7.054347462908075350, -1.199719254218455378 ) ) ;
#109194=ORIENTED_EDGE ( 'NONE', *, *, #191290, .T. ) ;
#109202=CARTESIAN_POINT ( 'NONE',  ( -4.140749582569956289, 7.233010276137757266, -0.9217035184944754045 ) ) ;
#109219=CARTESIAN_POINT ( 'NONE',  ( -4.932134020321308654, 8.976183133675331050, 0.7998128361456291469 ) ) ;
#109248=CARTESIAN_POINT ( 'NONE',  ( 6.912678218121202534, 9.158153569265168770, 1.599625672291268286 ) ) ;
#109257=CARTESIAN_POINT ( 'NONE',  ( 6.266000345369230118, 6.920845220647411367, 0.8521018698646137812 ) ) ;
#109261=CARTESIAN_POINT ( 'NONE',  ( 5.028717893731355026, 7.888467461587344687, 1.094519599958807765 ) ) ;
#109263=CARTESIAN_POINT ( 'NONE',  ( 7.024532985656141371, 7.367912369453226695, 0.7216878364870328300 ) ) ;
#109269=CARTESIAN_POINT ( 'NONE',  ( -4.472210567661380587, 6.310941310395290493, 1.599625672291270506 ) ) ;
#109277=CARTESIAN_POINT ( 'NONE',  ( -6.604230223188181093, 6.877559146573883453, 0.7216878364870317197 ) ) ;
#109281=CARTESIAN_POINT ( 'NONE',  ( 6.587282531393223728, 8.778525268082516320, 1.599625672291268286 ) ) ;
#109282=CARTESIAN_POINT ( 'NONE',  ( -5.814151116872314340, 5.955800188500202985, -0.1636420086626904635 ) ) ;
#109286=CARTESIAN_POINT ( 'NONE',  ( -4.496464221587651799, 5.274905009054215554, 1.199719254218452935 ) ) ;
#109295=CARTESIAN_POINT ( 'NONE',  ( 2.911969131885072670, 6.619324097166378706, 0.000000000000000000 ) ) ;
#109313=VERTEX_POINT ( 'NONE', #165346 ) ;
#109314=CARTESIAN_POINT ( 'NONE',  ( -6.557303570864871034, 7.679217583210999010, -1.199719254218452047 ) ) ;
#109317=CARTESIAN_POINT ( 'NONE',  ( 6.668631453075247073, 8.873432343378178544, -1.599625672291281386 ) ) ;
#109339=CARTESIAN_POINT ( 'NONE',  ( 4.394251184604957672, 8.140727125432173139, -0.7216878364870357165 ) ) ;
#109346=CARTESIAN_POINT ( 'NONE',  ( 8.039058738260216330, 8.343599714250547805, -0.7998128361456341429 ) ) ;
#109350=CARTESIAN_POINT ( 'NONE',  ( -6.319508997745553636, 6.545384383557486530, 0.7216878364870257245 ) ) ;
#109381=CARTESIAN_POINT ( 'NONE',  ( 3.542423274920540432, 7.354853930707762721, -1.734723475976807094E-15 ) ) ;
#109394=CARTESIAN_POINT ( 'NONE',  ( -5.614485009834902840, 9.564333254867113610, 0.7216878364870267237 ) ) ;
#109397=CARTESIAN_POINT ( 'NONE',  ( 4.217995187182922656, 6.014356699837137832, 1.443375672974058777 ) ) ;
#109414=ORIENTED_EDGE ( 'NONE', *, *, #61884, .T. ) ;
#109415=CARTESIAN_POINT ( 'NONE',  ( -3.634994582239682526, 6.294558541704648569, 1.082531754730549967 ) ) ;
#109420=CARTESIAN_POINT ( 'NONE',  ( -6.302510697806719797, 6.525553010488573058, -0.1636245105971004254 ) ) ;
#109447=CARTESIAN_POINT ( 'NONE',  ( -5.237192476628793614, 9.332084666034067055, 0.7998128361456291469 ) ) ;
#109448=CARTESIAN_POINT ( 'NONE',  ( -4.745581203565001793, 8.305819929356548670, 0.7838639097331673300 ) ) ;
#109449=CARTESIAN_POINT ( 'NONE',  ( -4.956387674247580755, 7.940146832334256111, 1.199719254218452935 ) ) ;
#109451=CARTESIAN_POINT ( 'NONE',  ( -4.613268803136618246, 8.378775596900176481, 0.2107346534404584415 ) ) ;
#109454=CARTESIAN_POINT ( 'NONE',  ( -6.251718229232856139, 8.387033582228697881, -1.443375672974066548 ) ) ;
#109460=CARTESIAN_POINT ( 'NONE',  ( -4.817943484809863008, 6.714296380401858499, 1.599625672291263179 ) ) ;
#109469=ORIENTED_EDGE ( 'NONE', *, *, #114198, .T. ) ;
#109473=CARTESIAN_POINT ( 'NONE',  ( 5.248941747146098180, 6.152795455539095570, -1.199719254218452047 ) ) ;
#109496=CARTESIAN_POINT ( 'NONE',  ( 6.215487077222150880, 6.216099443039444949, 0.000000000000000000 ) ) ;
#109497=CARTESIAN_POINT ( 'NONE',  ( 4.441177836928239309, 7.339068688795062911, 1.199719254218452047 ) ) ;
#109504=CARTESIAN_POINT ( 'NONE',  ( -1.833030277982346634, 0.000000000000000000, -2.499999999999998668 ) ) ;
#109511=CARTESIAN_POINT ( 'NONE',  ( 6.148788998471866662, 7.076870205577955986, 1.084632487400632339 ) ) ;
#109512=CARTESIAN_POINT ( 'NONE',  ( -3.634994581795317536, 7.254927755487573293, 0.000000000000000000 ) ) ;
#109513=CARTESIAN_POINT ( 'NONE',  ( 4.936577329151614180, 4.931964103531220722, -0.7216878364870458196 ) ) ;
#109530=CIRCLE ( 'NONE', #206221, 0.07999999999999989064 ) ;
#109536=DIRECTION ( 'NONE',  ( -0.000000000000000000, -1.000000000000000000, -0.000000000000000000 ) ) ;
#109537=CARTESIAN_POINT ( 'NONE',  ( -0.3396678349899239224, 2.756311866119263154, -2.043018440765232313 ) ) ;
#109545=CARTESIAN_POINT ( 'NONE',  ( 3.067887898442204442, 6.801229324816399746, 0.7998128361456271485 ) ) ;
#109564=CARTESIAN_POINT ( 'NONE',  ( -5.121948170912633991, 9.197632976031879792, -0.7998128361456362523 ) ) ;
#109566=ORIENTED_EDGE ( 'NONE', *, *, #135294, .T. ) ;
#109579=CARTESIAN_POINT ( 'NONE',  ( 5.574337433874081427, 6.532423756721743580, -1.199719254218452047 ) ) ;
#109589=CARTESIAN_POINT ( 'NONE',  ( 5.542547785767838242, 7.428594929708664196, 1.247761615041423244 ) ) ;
#109612=CARTESIAN_POINT ( 'NONE',  ( -5.875479466675803231, 7.948088359245467416, -1.599625672291271394 ) ) ;
#109614=CARTESIAN_POINT ( 'NONE',  ( 4.224247379109608680, 7.085983154673295203, -1.199719254218452047 ) ) ;
#109618=CARTESIAN_POINT ( 'NONE',  ( -5.562588163356775972, 9.711712967216715953, 0.7998128361456291469 ) ) ;
#109627=CARTESIAN_POINT ( 'NONE',  ( -5.797436685056675643, 7.335035436452395530, -1.304849551618554981 ) ) ;
#109645=CARTESIAN_POINT ( 'NONE',  ( 4.258669648468268676, 7.982548666606070320, 0.7216878364870257245 ) ) ;
#109648=CARTESIAN_POINT ( 'NONE',  ( -7.273023059088104425, 7.449891421883056530, 0.000000000000000000 ) ) ;
#109658=CARTESIAN_POINT ( 'NONE',  ( -2.862179826260718762, 6.353310540697199471, 0.000000000000000000 ) ) ;
#109663=CARTESIAN_POINT ( 'NONE',  ( 3.400062661977048428, 7.188766548940353829, -1.734723475976807094E-15 ) ) ;
#109699=CARTESIAN_POINT ( 'NONE',  ( -4.318600669050631780, 4.999583595936801572, -2.500000000000000444 ) ) ;
#109709=CARTESIAN_POINT ( 'NONE',  ( -5.275531169048922386, 5.327410250078064458, -0.7216878364870338292 ) ) ;
#109714=CARTESIAN_POINT ( 'NONE',  ( 0.000000000000000000, 9.001999999999998892, 0.000000000000000000 ) ) ;
#109715=CARTESIAN_POINT ( 'NONE',  ( -6.310394152517827315, 6.326824364217716656, 0.7998128361456281477 ) ) ;
#109722=CARTESIAN_POINT ( 'NONE',  ( -3.467853430045390706, 7.267855778353407459, 0.7998128361456352531 ) ) ;
#109725=CARTESIAN_POINT ( 'NONE',  ( 6.053423048675670159, 7.145495228771222784, -1.160209803801291795 ) ) ;
#109728=CARTESIAN_POINT ( 'NONE',  ( 2.972313222866368676, 6.545497292499366182, 0.5012468031770876964 ) ) ;
#109730=CARTESIAN_POINT ( 'NONE',  ( 4.908934136599710563, 7.884784371745123366, 1.199719254218451159 ) ) ;
#109736=CARTESIAN_POINT ( 'NONE',  ( -7.774674742793745708, 8.035151719539642912, 0.7998128361456341429 ) ) ;
#109740=CARTESIAN_POINT ( 'NONE',  ( -5.123001941117347080, 7.070197912760590064, 1.599625672291263179 ) ) ;
#109745=CARTESIAN_POINT ( 'NONE',  ( 5.194182247366869731, 7.153241603385088965, 1.443375672974064550 ) ) ;
#109746=CARTESIAN_POINT ( 'NONE',  ( -5.682275777458886346, 7.722684055159061423, 1.443375672974058777 ) ) ;
#109754=CARTESIAN_POINT ( 'NONE',  ( 3.542423274920540432, 7.354853930707762721, -1.734723475976807094E-15 ) ) ;
#109784=CARTESIAN_POINT ( 'NONE',  ( 4.909045613421183063, 8.010784895652180992, 0.9812996480243344477 ) ) ;
#109793=CARTESIAN_POINT ( 'NONE',  ( 5.481239241674765950, 9.616805891921051952, -0.7998128361456481317 ) ) ;
#109799=CARTESIAN_POINT ( 'NONE',  ( -4.756313517479579644, 8.198030745052275137, 0.7332552394410801755 ) ) ;
#109804=CARTESIAN_POINT ( 'NONE',  ( -5.582925393777276035, 9.735439736040634173, 0.7998128361456291469 ) ) ;
#109816=CARTESIAN_POINT ( 'NONE',  ( 6.526270840131753737, 8.707344961610770540, -1.599625672291283607 ) ) ;
#109826=CARTESIAN_POINT ( 'NONE',  ( 4.523580528814945545, 5.306540700819438960, 1.199719254218452047 ) ) ;
#109829=CARTESIAN_POINT ( 'NONE',  ( 6.509323147892504657, 6.766834225395614411, 0.000000000000000000 ) ) ;
#109831=VERTEX_POINT ( 'NONE', #137128 ) ;
#109836=CARTESIAN_POINT ( 'NONE',  ( -6.482157434489847603, 6.770256554395555959, 0.2388210531332583819 ) ) ;
#109841=CARTESIAN_POINT ( 'NONE',  ( -4.309512724297390740, 6.121127159803966933, 1.599625672291270506 ) ) ;
#109842=CARTESIAN_POINT ( 'NONE',  ( 7.024532985656136930, 8.328281583754568729, 1.082531754730549967 ) ) ;
#109854=ORIENTED_EDGE ( 'NONE', *, *, #122294, .T. ) ;
#109855=CARTESIAN_POINT ( 'NONE',  ( -5.641074431737709283, 8.738948049406083385, -1.199719254218452047 ) ) ;
#109856=CARTESIAN_POINT ( 'NONE',  ( -5.743814354044916470, 6.730146830254374990, -1.199719254218453823 ) ) ;
#109858=CARTESIAN_POINT ( 'NONE',  ( 5.953438849732186178, 8.999410187112612647, -1.082531754730548412 ) ) ;
#109870=CARTESIAN_POINT ( 'NONE',  ( -5.163927922758308142, 7.774463771048841565, -1.174891720174384480 ) ) ;
#109871=CARTESIAN_POINT ( 'NONE',  ( 8.014278199453780616, 8.522615118883788199, 0.000000000000000000 ) ) ;
#109875=CARTESIAN_POINT ( 'NONE',  ( 4.231553341240963384, 7.950912974840849579, -0.7216878364870357165 ) ) ;
#109880=CARTESIAN_POINT ( 'NONE',  ( -6.119526231721793330, 8.232809585132461194, 1.599625672291263179 ) ) ;
#109896=CARTESIAN_POINT ( 'NONE',  ( 5.611095471209277541, 7.639640364534566075, 1.599625672291268286 ) ) ;
#109914=CARTESIAN_POINT ( 'NONE',  ( 5.417547566918786472, 6.138612003838852971, 1.022798779415410753 ) ) ;
#109930=CARTESIAN_POINT ( 'NONE',  ( 6.211043768836170820, 9.299949259400630552, 1.082531754730549967 ) ) ;
#109950=CARTESIAN_POINT ( 'NONE',  ( 4.407809338218622308, 8.156544971314787063, 0.000000000000000000 ) ) ;
#109961=CARTESIAN_POINT ( 'NONE',  ( -4.950662367645459305, 5.804802846121667415, -1.199719254218453823 ) ) ;
#109963=CARTESIAN_POINT ( 'NONE',  ( 5.844973620822844218, 6.952128991449046502, 1.082531754730549967 ) ) ;
#109968=CARTESIAN_POINT ( 'NONE',  ( -5.991777542596674166, 5.955104985976372944, 0.000000000000000000 ) ) ;
#109973=CARTESIAN_POINT ( 'NONE',  ( -7.932929277771797238, 8.427708043588125975, 0.000000000000000000 ) ) ;
#109976=CARTESIAN_POINT ( 'NONE',  ( -1.817552723627640532, 2.511586290612293659, 2.499391979724955526 ) ) ;
#109981=CARTESIAN_POINT ( 'NONE',  ( -6.123442655227560927, 7.173046514967467147, 1.199719254218452047 ) ) ;
#109990=CARTESIAN_POINT ( 'NONE',  ( -5.093022980588950865, 5.970890227889075419, -1.199719254218453823 ) ) ;
#109993=CARTESIAN_POINT ( 'NONE',  ( -4.651856103264620401, 8.441266197201775512, 0.000000000000000000 ) ) ;
#109994=CARTESIAN_POINT ( 'NONE',  ( -4.923019175093582334, 8.757623114335565617, 0.7216878364870267237 ) ) ;
#109995=CARTESIAN_POINT ( 'NONE',  ( 5.176180785367283654, 9.260904359562321275, -0.7998128361456481317 ) ) ;
#109996=CARTESIAN_POINT ( 'NONE',  ( -7.445362632559989535, 8.715286488521982733, 1.199719254218452047 ) ) ;
#110014=CARTESIAN_POINT ( 'NONE',  ( 7.014364370223726830, 9.276787413384745662, -1.599625672291269396 ) ) ;
#110034=CARTESIAN_POINT ( 'NONE',  ( 4.708029738644283313, 8.352945002179891887, -0.6661931671527853149 ) ) ;
#110047=CARTESIAN_POINT ( 'NONE',  ( 6.363572996767764778, 8.517530811019446091, -1.599625672291283607 ) ) ;
#110053=CARTESIAN_POINT ( 'NONE',  ( -5.763624699140874164, 8.777960344756069233, -1.082531754730549967 ) ) ;
#110065=CARTESIAN_POINT ( 'NONE',  ( 6.994027139803230320, 9.253060644560830994, -1.599625672291267398 ) ) ;
#110066=CARTESIAN_POINT ( 'NONE',  ( 5.611095471209277541, 7.639640364534566075, 1.599625672291268286 ) ) ;
#110080=CARTESIAN_POINT ( 'NONE',  ( 4.552505719138623341, 8.533283448962240669, 0.7998128361456341429 ) ) ;
#110095=CARTESIAN_POINT ( 'NONE',  ( -4.665414256878301025, 6.536345614481700927, -1.443375672974066548 ) ) ;
#110096=CARTESIAN_POINT ( 'NONE',  ( -7.747558435566414659, 8.003516027774422170, -0.7998128361456362523 ) ) ;
#110102=ORIENTED_EDGE ( 'NONE', *, *, #5141, .F. ) ;
#110104=FACE_OUTER_BOUND ( 'NONE', #52112, .T. ) ;
#110109=CARTESIAN_POINT ( 'NONE',  ( 6.363572996767764778, 8.517530811019446091, -1.599625672291283607 ) ) ;
#110112=CARTESIAN_POINT ( 'NONE',  ( 5.031484404002889654, 6.003058238492422483, 1.082531754730549078 ) ) ;
#110116=DIRECTION ( 'NONE',  ( -0.6507913734559641616, -0.7592566023653004592, 0.000000000000000000 ) ) ;
#110119=CARTESIAN_POINT ( 'NONE',  ( 7.015401035077362124, 6.062865449010541141, -2.437084766375293921 ) ) ;
#110131=CARTESIAN_POINT ( 'NONE',  ( 5.761288931164342486, 5.686201605971993978, -0.7998128361456481317 ) ) ;
#110133=CARTESIAN_POINT ( 'NONE',  ( -2.979759899953417612, 6.698413326579433225, 0.7998128361456352531 ) ) ;
#110135=CARTESIAN_POINT ( 'NONE',  ( 4.549643065837591038, 7.465611455855944101, -1.199719254218452047 ) ) ;
#110144=CARTESIAN_POINT ( 'NONE',  ( 5.221298555038576872, 9.105615724271411082, 0.000000000000000000 ) ) ;
#110146=CARTESIAN_POINT ( 'NONE',  ( -6.631873415740034083, 7.766215735565355160, 1.199719254218452047 ) ) ;
#110147=CARTESIAN_POINT ( 'NONE',  ( 4.878955176071345434, 6.785476686873604280, -1.599625672291269396 ) ) ;
#110158=CARTESIAN_POINT ( 'NONE',  ( -5.795184315198522285, 5.725746220678519904, -0.7998128361456362523 ) ) ;
#110187=CARTESIAN_POINT ( 'NONE',  ( 3.933273961740298752, 5.682181936820735579, 1.443375672974058777 ) ) ;
#110193=CARTESIAN_POINT ( 'NONE',  ( 4.895902867866261055, 4.884510565364971413, -0.7216878364870458196 ) ) ;
#110201=( BOUNDED_CURVE ( )  B_SPLINE_CURVE ( 2, ( #78959, #76827, #74711, #140814, #42229, #173293, #94184 ),
 .UNSPECIFIED., .F., .T. ) 
 B_SPLINE_CURVE_WITH_KNOTS ( ( 3, 2, 2, 3 ),
 ( 0.3750000000000002776, 0.3833333333333334703, 0.3916666666666665519, 0.3999999999999997446 ),
 .UNSPECIFIED. ) 
 CURVE ( )  GEOMETRIC_REPRESENTATION_ITEM ( )  RATIONAL_B_SPLINE_CURVE ( ( 0.9999999999999955591, 0.8660254037844431485, 1.000000000000000000, 0.8660254037844387076, 1.000000000000000000, 0.8660254037844431485, 0.9999999999999955591 ) ) 
 REPRESENTATION_ITEM ( '' )  );
#110204=CARTESIAN_POINT ( 'NONE',  ( -4.305596300791617814, 7.180890229968955651, 1.199719254218452935 ) ) ;
#110206=CARTESIAN_POINT ( 'NONE',  ( -4.936050443827081580, 7.916420063510339666, 1.199719254218452935 ) ) ;
#110209=CARTESIAN_POINT ( 'NONE',  ( 7.485510208076452621, 7.905719128943566432, 0.000000000000000000 ) ) ;
#110220=CARTESIAN_POINT ( 'NONE',  ( -4.599959256786493533, 8.588645909551377855, 0.000000000000000000 ) ) ;
#110227=CARTESIAN_POINT ( 'NONE',  ( -5.641601317062259646, 5.754492089426966217, -0.7216878364870338292 ) ) ;
#110231=CARTESIAN_POINT ( 'NONE',  ( -3.949167883330528372, 7.829389307186077396, 1.214306433183764966E-14 ) ) ;
#110251=CARTESIAN_POINT ( 'NONE',  ( -4.769436176957319695, 8.786368983084006601, 0.7998128361456281477 ) ) ;
#110253=CARTESIAN_POINT ( 'NONE',  ( -4.950662367645459305, 5.804802846121667415, -1.199719254218453823 ) ) ;
#110262=CARTESIAN_POINT ( 'NONE',  ( -1.806654366501805775, 0.000000000000000000, 2.420000000000000373 ) ) ;
#110278=CARTESIAN_POINT ( 'NONE',  ( -7.957709816578236506, 8.248692638954882028, 0.7998128361456341429 ) ) ;
#110290=CARTESIAN_POINT ( 'NONE',  ( 0.000000000000000000, 9.000000000000000000, 2.080000000000000071 ) ) ;
#110306=CARTESIAN_POINT ( 'NONE',  ( 7.452141709366786770, 8.723195411463290583, 1.199719254218452047 ) ) ;
#110320=CARTESIAN_POINT ( 'NONE',  ( 5.094250900851895025, 7.824382189606214233, 1.140223938556598871 ) ) ;
#110322=CARTESIAN_POINT ( 'NONE',  ( 6.536439455564155843, 8.719208346281938304, 1.443375672974065660 ) ) ;
#110331=CARTESIAN_POINT ( 'NONE',  ( -6.120580001926503755, 6.105374521861167914, -0.7998128361456362523 ) ) ;
#110338=CARTESIAN_POINT ( 'NONE',  ( -5.411112705185557203, 9.327065566109540740, 0.7216878364870267237 ) ) ;
#110342=CARTESIAN_POINT ( 'NONE',  ( 5.993586425693011144, 9.150212042353954800, -1.199719254218452047 ) ) ;
#110348=CARTESIAN_POINT ( 'NONE',  ( -4.065465959251405081, 5.836405933916976707, -1.599625672291271394 ) ) ;
#110357=CARTESIAN_POINT ( 'NONE',  ( 5.996449078994045223, 10.21788403546024782, 0.7998128361456331437 ) ) ;
#110378=CARTESIAN_POINT ( 'NONE',  ( 4.857564175446106525, 8.889184981320973122, 0.7998128361456331437 ) ) ;
#110381=CARTESIAN_POINT ( 'NONE',  ( -5.865985541149716376, 7.193105608424513520, 1.152625159504708119 ) ) ;
#110387=CARTESIAN_POINT ( 'NONE',  ( 5.391302360089590628, 6.318882837306503575, -1.199719254218452047 ) ) ;
#110395=CARTESIAN_POINT ( 'NONE',  ( 3.770576118376306241, 6.452737000530752276, 1.082531754730549078 ) ) ;
#110398=CARTESIAN_POINT ( 'NONE',  ( 4.407809338218622308, 8.156544971314787063, 0.000000000000000000 ) ) ;
#110406=CARTESIAN_POINT ( 'NONE',  ( -4.613268803136618246, 8.378775596900176481, 0.2107346534404584415 ) ) ;
#110410=CARTESIAN_POINT ( 'NONE',  ( -5.533136088152923904, 6.588318536667425285, 1.082531754730549078 ) ) ;
#110414=VECTOR ( 'NONE', #97170, 1000.000000000000000 ) ;
#110432=DIRECTION ( 'NONE',  ( 1.000000000000000000, 0.000000000000000000, 0.000000000000000000 ) ) ;
#110442=CARTESIAN_POINT ( 'NONE',  ( 3.705121118284530279, 7.544668081299086282, -1.734723475976807094E-15 ) ) ;
#110454=CARTESIAN_POINT ( 'NONE',  ( -6.943184063974178422, 8.233374508458908281, -1.082531754730549967 ) ) ;
#110456=CARTESIAN_POINT ( 'NONE',  ( 5.519577934094864524, 5.612131475965050242, 0.7216878364870328300 ) ) ;
#110480=DIRECTION ( 'NONE',  ( 0.000000000000000000, 0.000000000000000000, -1.000000000000000000 ) ) ;
#110501=CARTESIAN_POINT ( 'NONE',  ( 5.589586000038863745, 5.798386900100804375, -0.7226491117988718127 ) ) ;
#110506=CARTESIAN_POINT ( 'NONE',  ( -6.770317605177755382, 8.992066187497757213, 1.599625672291269396 ) ) ;
#110509=CARTESIAN_POINT ( 'NONE',  ( -7.761116589180078407, 8.019333873657032541, 0.000000000000000000 ) ) ;
#110510=CARTESIAN_POINT ( 'NONE',  ( -5.773448424614897156, 7.353550462951784716, 1.313087523158409153 ) ) ;
#110512=CARTESIAN_POINT ( 'NONE',  ( -4.810269800901881609, 8.163507479013537349, 0.8607707128150362541 ) ) ;
#110518=CARTESIAN_POINT ( 'NONE',  ( -3.654804927335652209, 6.421633627603656080, 1.199719254218452935 ) ) ;
#110522=CARTESIAN_POINT ( 'NONE',  ( -3.983063267364693960, 7.868933921892603323, -0.7998128361456481317 ) ) ;
#110530=CARTESIAN_POINT ( 'NONE',  ( -6.071018923869249129, 10.30488218781460574, 0.7998128361456291469 ) ) ;
#110535=CARTESIAN_POINT ( 'NONE',  ( 5.761288931164342486, 5.686201605971993978, -0.7998128361456481317 ) ) ;
#110558=CARTESIAN_POINT ( 'NONE',  ( 4.746236293235721604, 7.694970221153795364, 1.199719254218451159 ) ) ;
#110559=CARTESIAN_POINT ( 'NONE',  ( 5.761288931164342486, 5.686201605971993978, -0.7998128361456481317 ) ) ;
#110573=CARTESIAN_POINT ( 'NONE',  ( 5.275877007301786215, 7.772378248882220397, 1.293907329011657614 ) ) ;
#110574=CIRCLE ( 'NONE', #79276, 1.250000000000000888 ) ;
#110575=CARTESIAN_POINT ( 'NONE',  ( -4.462041952228944730, 7.259447140025469203, -1.082531754730549967 ) ) ;
#110576=CARTESIAN_POINT ( 'NONE',  ( -3.059603515650958450, 6.244770895048625370, 0.7153734454320024305 ) ) ;
#110604=CARTESIAN_POINT ( 'NONE',  ( 3.366167277942881064, 7.149221934233827014, -0.7998128361456362523 ) ) ;
#110623=CARTESIAN_POINT ( 'NONE',  ( -7.119966945832006289, 8.335658187339330283, 1.199719254218452047 ) ) ;
#110637=VERTEX_POINT ( 'NONE', #136613 ) ;
#110638=CARTESIAN_POINT ( 'NONE',  ( 5.571474780572990504, 5.464751763615448787, 0.7998128361456352531 ) ) ;
#110647=DIRECTION ( 'NONE',  ( 1.000000000000000000, 0.000000000000000000, 0.000000000000000000 ) ) ;
#110648=CARTESIAN_POINT ( 'NONE',  ( -0.4461809497497640775, 3.122791860410086606, 1.949595486268987043 ) ) ;
#110649=CARTESIAN_POINT ( 'NONE',  ( 5.234661009243278151, 7.693064604033777343, 1.208367059251337361 ) ) ;
#110662=CARTESIAN_POINT ( 'NONE',  ( -6.170096473061220443, 6.976792551583999469, 0.9111270007488531109 ) ) ;
#110666=ORIENTED_EDGE ( 'NONE', *, *, #98746, .F. ) ;
#110668=CARTESIAN_POINT ( 'NONE',  ( -4.606738333593328072, 8.596554832492683929, 0.7998128361456281477 ) ) ;
#110670=CARTESIAN_POINT ( 'NONE',  ( 3.739016502318667445, 7.584212696005614873, 0.7998128361456271485 ) ) ;
#110674=CARTESIAN_POINT ( 'NONE',  ( -8.100070429521727178, 8.414780020722290033, 0.7998128361456341429 ) ) ;
#110677=CARTESIAN_POINT ( 'NONE',  ( 6.502017186205484300, 9.743381262951846367, -1.199719254218452047 ) ) ;
#110684=CARTESIAN_POINT ( 'NONE',  ( -5.577377183731011101, 7.510248947172004641, -1.348340355397449342 ) ) ;
#110699=CARTESIAN_POINT ( 'NONE',  ( 4.258669648468278446, 7.022179452304728287, 1.082531754730549078 ) ) ;
#110717=CARTESIAN_POINT ( 'NONE',  ( 4.037295881819344956, 7.932205305423046582, -0.7998128361456362523 ) ) ;
#110733=ORIENTED_EDGE ( 'NONE', *, *, #73531, .F. ) ;
#110767=CARTESIAN_POINT ( 'NONE',  ( -3.946832114909637479, 7.618738210787614484, 0.7216878364870338292 ) ) ;
#110774=CARTESIAN_POINT ( 'NONE',  ( -4.261005416444848315, 8.193199762486115034, 0.7998128361456352531 ) ) ;
#110782=CARTESIAN_POINT ( 'NONE',  ( -4.118644803501354978, 8.027112380718707030, 0.7998128361456352531 ) ) ;
#110785=CARTESIAN_POINT ( 'NONE',  ( 5.355371708033295874, 7.701368364266228284, 1.317571137710125351 ) ) ;
#110788=CARTESIAN_POINT ( 'NONE',  ( 2.987092767191504183, 6.445738828830674727, 0.3863172271417950054 ) ) ;
#110790=CARTESIAN_POINT ( 'NONE',  ( 6.150558962454855561, 7.204682206732687000, 1.199719254218452047 ) ) ;
#110795=CARTESIAN_POINT ( 'NONE',  ( -6.749980374757255319, 8.968339418673846097, 1.599625672291269396 ) ) ;
#110800=CARTESIAN_POINT ( 'NONE',  ( -3.772911886352873445, 7.623757310712140800, 0.7998128361456352531 ) ) ;
#110803=CARTESIAN_POINT ( 'NONE',  ( 5.356880090730863131, 7.343055753976412525, 1.443375672974064550 ) ) ;
#110804=CARTESIAN_POINT ( 'NONE',  ( -5.600926855776882540, 8.588146194164741232, -1.082531754730549967 ) ) ;
#110809=CARTESIAN_POINT ( 'NONE',  ( -5.906512197408906317, 6.919960980845699439, -1.199719254218453823 ) ) ;
#110812=CARTESIAN_POINT ( 'NONE',  ( 6.039231080244466199, 6.010467446565510130, 0.7998128361456352531 ) ) ;
#110813=ORIENTED_EDGE ( 'NONE', *, *, #16190, .T. ) ;
#110841=CARTESIAN_POINT ( 'NONE',  ( 4.631618433768171172, 8.327536854573105884, -0.3785340233409782984 ) ) ;
#110848=CARTESIAN_POINT ( 'NONE',  ( 5.397027666691686321, 8.454226823519094935, 1.199719254218451159 ) ) ;
#110853=CARTESIAN_POINT ( 'NONE',  ( -4.629329830860687167, 8.351765225447314478, -0.3187335059142253346 ) ) ;
#110862=CARTESIAN_POINT ( 'NONE',  ( -3.973948422136970748, 6.690004688251493192, -1.082531754730546636 ) ) ;
#110874=CARTESIAN_POINT ( 'NONE',  ( -3.332271893908731464, 7.109677319527304640, -0.7998128361456481317 ) ) ;
#110876=CARTESIAN_POINT ( 'NONE',  ( 7.523848900940885542, 7.742521570711348389, 0.7998128361456291469 ) ) ;
#110879=DIRECTION ( 'NONE',  ( 0.7592566023653005702, -0.6507913734559639396, 0.000000000000000000 ) ) ;
#110884=CARTESIAN_POINT ( 'NONE',  ( 4.960304097753311936, 6.880383762169266504, 1.599625672291268286 ) ) ;
#110887=CARTESIAN_POINT ( 'NONE',  ( 4.814553946184248368, 7.670711132973337065, -1.082531754730548412 ) ) ;
#110888=CARTESIAN_POINT ( 'NONE',  ( 0.1216811705908975721, 2.536982183874236352, -1.996294991408742003 ) ) ;
#110894=CYLINDRICAL_SURFACE ( 'NONE', #3882, 1.250000000000000000 ) ;
#110895=CARTESIAN_POINT ( 'NONE',  ( -5.941092982759174745, 7.138105816550336158, 1.109076209742832164 ) ) ;
#110902=CARTESIAN_POINT ( 'NONE',  ( -5.469788628470539926, 5.346117919495872783, -0.7998128361456362523 ) ) ;
#110903=CARTESIAN_POINT ( 'NONE',  ( 3.902768115887398803, 5.646591783325653147, -1.599625672291269396 ) ) ;
#110914=CARTESIAN_POINT ( 'NONE',  ( -6.611536185319534908, 7.742488966741438716, 1.199719254218452047 ) ) ;
#110915=CARTESIAN_POINT ( 'NONE',  ( -5.418418667316934112, 6.350518529071726981, -1.199719254218453823 ) ) ;
#110917=CARTESIAN_POINT ( 'NONE',  ( 5.492461626867537916, 9.421972641405202964, -0.7216878364870458196 ) ) ;
#110922=CARTESIAN_POINT ( 'NONE',  ( 4.523580528814945545, 5.306540700819438960, 1.199719254218452047 ) ) ;
#110929=CARTESIAN_POINT ( 'NONE',  ( -5.448385796200811981, 7.521903143423984694, -1.249286997217812223 ) ) ;
#110939=CARTESIAN_POINT ( 'NONE',  ( -6.770317605177755382, 8.992066187497757213, 1.599625672291269396 ) ) ;
#110955=CARTESIAN_POINT ( 'NONE',  ( 5.529746549527311039, 7.544733289238903851, -1.599625672291281386 ) ) ;
#110991=CARTESIAN_POINT ( 'NONE',  ( 5.090160327287878594, 4.903218234782778850, -0.7998128361456481317 ) ) ;
#111021=CARTESIAN_POINT ( 'NONE',  ( -5.387385936583832802, 7.378645907471495846, -1.599625672291271394 ) ) ;
#111023=CARTESIAN_POINT ( 'NONE',  ( 4.651856102820254968, 7.480896982382013505, -1.082531754730548412 ) ) ;
#111028=CARTESIAN_POINT ( 'NONE',  ( -5.276058054373441664, 6.184431147304315424, -1.199719254218453823 ) ) ;
#111032=CARTESIAN_POINT ( 'NONE',  ( -6.966220764712169000, 6.002124920821316323, -2.420000000000000373 ) ) ;
#111033=CARTESIAN_POINT ( 'NONE',  ( -4.604929450496978660, 5.401447776115099408, -1.199719254218453823 ) ) ;
#111040=CARTESIAN_POINT ( 'NONE',  ( -4.437261413422502798, 8.398831758960053406, 0.000000000000000000 ) ) ;
#111049=CARTESIAN_POINT ( 'NONE',  ( -4.472210567661380587, 6.310941310395290493, 1.599625672291270506 ) ) ;
#111050=AXIS2_PLACEMENT_3D ( 'NONE', #33951, #198564, #182322 ) ;
#111053=CARTESIAN_POINT ( 'NONE',  ( -5.966997003790232235, 7.094489604910957148, -1.082531754730549967 ) ) ;
#111054=CARTESIAN_POINT ( 'NONE',  ( -5.926322542504872892, 8.007405281046052536, -1.443375672974066548 ) ) ;
#111055=CARTESIAN_POINT ( 'NONE',  ( 5.742760583840166966, 8.857581893525663830, 1.199719254218452047 ) ) ;
#111056=CARTESIAN_POINT ( 'NONE',  ( -5.108390017298964914, 9.181815130149269422, 0.000000000000000000 ) ) ;
#111095=CARTESIAN_POINT ( 'NONE',  ( 4.632842592818133376, 8.443130954262043630, -0.3954830847591808696 ) ) ;
#111110=CARTESIAN_POINT ( 'NONE',  ( 7.062871678076271920, 7.204714810702593120, -0.7998128361456341429 ) ) ;
#111113=CARTESIAN_POINT ( 'NONE',  ( -2.979759899953417612, 6.698413326579433225, 0.7998128361456352531 ) ) ;
#111118=CARTESIAN_POINT ( 'NONE',  ( -6.821160681006823268, 9.051383109298335228, 1.443375672974064550 ) ) ;
#111129=CARTESIAN_POINT ( 'NONE',  ( 6.318982112420993502, 9.529840343536603697, -1.199719254218452047 ) ) ;
#111130=CARTESIAN_POINT ( 'NONE',  ( 6.530187263637528439, 7.647581891445782709, -1.199719254218452047 ) ) ;
#111131=CARTESIAN_POINT ( 'NONE',  ( 0.1216811705908975721, 2.536982183874236352, -1.996294991408742003 ) ) ;
#111137=VECTOR ( 'NONE', #24669, 1000.000000000000000 ) ;
#111141=CARTESIAN_POINT ( 'NONE',  ( 2.925527285498711549, 6.635141943048991742, 0.7998128361456281477 ) ) ;
#111148=CARTESIAN_POINT ( 'NONE',  ( 5.580062740476173566, 8.667767742934335828, 1.199719254218451159 ) ) ;
#111161=CARTESIAN_POINT ( 'NONE',  ( -6.129694847154231852, 6.323934541200937787, -0.7216878364870338292 ) ) ;
#111162=CARTESIAN_POINT ( 'NONE',  ( -7.910256278930404505, 8.193330178365746619, -0.7998128361456362523 ) ) ;
#111175=CARTESIAN_POINT ( 'NONE',  ( 7.035755370848908896, 7.173079118937375931, 0.7998128361456352531 ) ) ;
#111178=CARTESIAN_POINT ( 'NONE',  ( 3.051993976407674225, 6.574760382535328240, -0.7216878364870338292 ) ) ;
#111195=CARTESIAN_POINT ( 'NONE',  ( 5.737035277238070385, 6.722237907313067140, -1.199719254218452047 ) ) ;
#111197=CARTESIAN_POINT ( 'NONE',  ( -5.164730172163054966, 4.990216387137135889, -0.7998128361456362523 ) ) ;
#111201=CARTESIAN_POINT ( 'NONE',  ( 5.520104819419390907, 6.469152373191302985, 1.199719254218452935 ) ) ;
#111212=CARTESIAN_POINT ( 'NONE',  ( 7.404161286838808920, 8.771181268467660885, -1.082531754730548412 ) ) ;
#111214=CARTESIAN_POINT ( 'NONE',  ( -6.688968683495758683, 8.897159112202094988, -1.599625672291271394 ) ) ;
#111215=CARTESIAN_POINT ( 'NONE',  ( 4.553559489343365740, 6.405848385690952718, -1.599625672291269396 ) ) ;
#111225=CARTESIAN_POINT ( 'NONE',  ( -5.635349125135588721, 6.603604063193491136, 1.199719254218452935 ) ) ;
#111231=AXIS2_PLACEMENT_3D ( 'NONE', #57178, #105977, #140602 ) ;
#111253=CARTESIAN_POINT ( 'NONE',  ( 4.421367491832268293, 7.211993602896056288, 1.082531754730549078 ) ) ;
#111259=CARTESIAN_POINT ( 'NONE',  ( 3.892599500454932304, 7.555466827257172113, 0.7216878364870257245 ) ) ;
#111272=CARTESIAN_POINT ( 'NONE',  ( -5.679940009482361774, 5.591294530676332641, 0.7998128361456281477 ) ) ;
#111274=CARTESIAN_POINT ( 'NONE',  ( -6.882699257592852504, 8.058845884393651460, -1.199719254218452047 ) ) ;
#111276=CARTESIAN_POINT ( 'NONE',  ( 5.831415467209187575, 9.817418788470464008, 0.000000000000000000 ) ) ;
#111285=CARTESIAN_POINT ( 'NONE',  ( -5.424143973919053785, 8.485862515284315677, 1.199719254218454489 ) ) ;
#111290=( BOUNDED_SURFACE ( )  B_SPLINE_SURFACE ( 1, 2, ( 
 ( #47664, #61757, #177652, #46587, #126842, #207990, #31396, #97470, #191736, #192800, #43392, #94284, #193878, #109513, #209044, #44459, #175521, #159249, #10849, #160324, #127926, #29261, #95353, #161403, #12987, #211185, #82253, #84396, #81202, #32452, #180826, #85460, #184017, #151546, #148344, #49765, #214345, #83313, #165649, #98521, #68113, #164583, #17238, #101711, #198134, #35634, #65975, #115891, #33512, #132123, #16168, #114827, #51908, #134250, #181876, #147280, #213312, #34572, #200256, #118031, #102787, #99585, #149399, #135305, #50831, #167784, #982, #19380, #199184, #67047, #64937, #3113, #52958, #69184, #116958, #166720, #100644, #133184, #182957, #201318, #18311, #150483, #168845, #131087, #119096, #197077, #2043, #185076, #36702, #48714, #156884, #140658, #123399, #107114, #39928, #21495, #6324, #106037, #121253, #172059, #37784, #20448, #88682, #104936, #87605, #24719, #153675, #72398, #5243, #103858, #74557, #173137, #71319, #205601, #55104, #138498, #154741, #189363, #190418, #124459, #137432, #41004, #204520, #187224, #56167, #203450, #90821, #122331, #8471, #206672, #86530, #42076, #58304, #108189, #186150, #188288, #70253, #152596, #23653, #22576, #89761, #4182, #155810, #136366, #7394, #38852, #202386, #170977, #73473, #139574, #57239, #54036, #120173, #169908, #44201, #143866, #95092, #92961, #195769, #210931, #211993, #79872, #10600, #63634, #60427, #11671, #161140, #109263, #175271, #47408, #129788, #159007, #194692, #209859, #208797, #77745, #76677, #128721, #61497, #178462, #112449, #174215, #25788, #46334, #30071, #125521, #27935, #9547, #91899, #127664, #176328, #94029, #62557, #193626, #157955, #12728, #142791, #75623, #26856, #126587, #78801, #110322, #29005, #177391, #96161, #160067, #45268, #144925, #192548, #141732, #162213, #207740, #145982, #111389, #59365, #13798, #191482, #43150, #48469, #114584, #201064, #31148, #97222, #166461, #100391, #101457, #164331, #98273, #2861, #116697, #180575, #182696, #113520, #64690, #213060, #117781, #1798, #183773, #32197, #82004, #150227 ),
 ( #115631, #18053, #148092, #84139, #16983, #200009, #163275, #214097, #130835, #50575, #181626, #83062, #132924, #15921, #14856, #65724, #147038, #33255, #35383, #80946, #34315, #179529, #68931, #196827, #131872, #67855, #197881, #49511, #167529, #134003, #51659, #149138, #99339, #165388, #720, #66784, #198929, #19127, #85206, #151290, #135051, #102527, #138247, #204261, #186967, #88424, #36452, #106852, #104677, #189113, #168589, #122070, #52706, #156631, #118836, #71063, #188033, #20189, #184822, #123156, #89502, #39663, #170725, #140401, #86277, #54850, #154490, #203203, #6069, #23391, #121000, #152347, #3925, #55912, #105771, #38599, #72139, #69995, #172882, #22311, #24456, #103600, #155557, #136107, #7137, #202123, #21243, #137179, #171797, #90570, #73209, #8220, #139316, #205345, #53782, #119915, #74305, #185891, #56982, #40747, #87350, #37525, #169658, #153416, #4987, #207488, #177134, #160886, #109000, #59107, #157698, #192290, #208538, #60174, #12481, #128474, #206420, #127403, #95909, #175017, #125267, #42891, #26604, #92705, #190172, #158751, #9295, #76420, #78555, #110066, #10346, #142531, #144673, #126331, #210686, #191228, #43950, #176078, #27676, #75368, #25537, #28751, #45020, #93771, #58044, #124209, #159811, #193375, #94835, #13553, #11415, #77490, #143609, #209602, #61246, #91645, #178210, #46084, #111130, #62315, #194442, #112203, #29826, #161963, #79625, #41826, #107939, #141480, #173964, #213860, #49274, #165142, #130593, #195519, #196582, #179277, #65480, #116447, #64448, #147842, #18868, #211745, #34068, #167283, #146795, #182441, #467, #83880, #67602, #51401, #100139, #17792, #16733, #212811, #131630, #82818, #31955, #148894, #163025, #145744, #197629, #15673, #48224, #149971, #114337, #115395, #180332, #14608, #199756, #1540, #98039, #166202, #164092, #181388, #33011, #133748, #101195, #35123, #81760, #117521, #99090, #66537, #132678, #198684, #183514, #50329, #63383, #129538, #47156, #113272, #30900, #96977, #80705, #153158, #134802, #125813, #54592, #87088, #4733, #190709, #120739 ) ),
 .UNSPECIFIED., .F., .F., .F. ) 
 B_SPLINE_SURFACE_WITH_KNOTS ( ( 2, 2 ),
 ( 3, 2, 2, 2, 2, 2, 2, 2, 2, 2, 2, 2, 2, 2, 2, 2, 2, 2, 2, 2, 2, 2, 2, 2, 2, 2, 2, 2, 2, 2, 2, 2, 2, 2, 2, 2, 2, 2, 2, 2, 2, 2, 2, 2, 2, 2, 2, 2, 2, 2, 2, 2, 2, 2, 2, 2, 2, 2, 2, 2, 2, 2, 2, 2, 2, 2, 2, 2, 2, 2, 2, 2, 2, 2, 2, 2, 2, 2, 2, 2, 2, 2, 2, 2, 2, 2, 2, 2, 2, 2, 2, 2, 2, 2, 2, 2, 2, 2, 2, 2, 2, 2, 2, 2, 2, 2, 2, 2, 2, 2, 2, 2, 2, 2, 2, 2, 2, 2, 2, 2, 3 ),
 ( 0.000000000000000000, 1.000000000000000000 ),
 ( 0.000000000000000000, 0.008333333333333333218, 0.01666666666666666644, 0.02500000000000000139, 0.03333333333333333287, 0.04166666666666666435, 0.05000000000000000278, 0.05833333333333333426, 0.06666666666666666574, 0.07499999999999999722, 0.08333333333333332871, 0.09166666666666666019, 0.1000000000000000056, 0.1083333333333333370, 0.1166666666666666685, 0.1250000000000000000, 0.1333333333333333315, 0.1416666666666666630, 0.1499999999999999944, 0.1583333333333333259, 0.1666666666666666574, 0.1749999999999999889, 0.1833333333333333204, 0.1916666666666666796, 0.2000000000000000111, 0.2083333333333333426, 0.2166666666666666741, 0.2250000000000000056, 0.2333333333333333370, 0.2416666666666666685, 0.2500000000000000000, 0.2583333333333333592, 0.2666666666666666630, 0.2750000000000000222, 0.2833333333333333259, 0.2916666666666666852, 0.2999999999999999889, 0.3083333333333333481, 0.3166666666666666519, 0.3250000000000000111, 0.3333333333333333148, 0.3416666666666666741, 0.3499999999999999778, 0.3583333333333333370, 0.3666666666666666408, 0.3750000000000000000, 0.3833333333333333592, 0.3916666666666666630, 0.4000000000000000222, 0.4083333333333333259, 0.4166666666666666852, 0.4249999999999999889, 0.4333333333333333481, 0.4416666666666666519, 0.4500000000000000111, 0.4583333333333333148, 0.4666666666666666741, 0.4749999999999999778, 0.4833333333333333370, 0.4916666666666666408, 0.5000000000000000000, 0.5083333333333333037, 0.5166666666666667185, 0.5250000000000000222, 0.5333333333333333259, 0.5416666666666666297, 0.5500000000000000444, 0.5583333333333333481, 0.5666666666666666519, 0.5749999999999999556, 0.5833333333333333703, 0.5916666666666666741, 0.5999999999999999778, 0.6083333333333332815, 0.6166666666666666963, 0.6250000000000000000, 0.6333333333333333037, 0.6416666666666667185, 0.6500000000000000222, 0.6583333333333333259, 0.6666666666666666297, 0.6750000000000000444, 0.6833333333333333481, 0.6916666666666666519, 0.6999999999999999556, 0.7083333333333333703, 0.7166666666666666741, 0.7249999999999999778, 0.7333333333333332815, 0.7416666666666666963, 0.7500000000000000000, 0.7583333333333333037, 0.7666666666666667185, 0.7750000000000000222, 0.7833333333333333259, 0.7916666666666666297, 0.8000000000000000444, 0.8083333333333333481, 0.8166666666666666519, 0.8249999999999999556, 0.8333333333333333703, 0.8416666666666666741, 0.8499999999999999778, 0.8583333333333332815, 0.8666666666666666963, 0.8750000000000000000, 0.8833333333333333037, 0.8916666666666667185, 0.9000000000000000222, 0.9083333333333333259, 0.9166666666666666297, 0.9250000000000000444, 0.9333333333333333481, 0.9416666666666666519, 0.9499999999999999556, 0.9583333333333333703, 0.9666666666666666741, 0.9749999999999999778, 0.9833333333333332815, 0.9916666666666666963, 1.000000000000000000 ),
 .UNSPECIFIED. ) 
 GEOMETRIC_REPRESENTATION_ITEM ( )  RATIONAL_B_SPLINE_SURFACE ( (
 ( 1.000000000000000000, 0.8660254037844387076, 1.000000000000000000, 0.8660254037844387076, 1.000000000000000000, 0.8660254037844387076, 1.000000000000000000, 0.8660254037844387076, 1.000000000000000000, 0.8660254037844387076, 1.000000000000000000, 0.8660254037844387076, 1.000000000000000000, 0.8660254037844387076, 1.000000000000000000, 0.8660254037844387076, 1.000000000000000000, 0.8660254037844387076, 1.000000000000000000, 0.8660254037844387076, 1.000000000000000000, 0.8660254037844387076, 1.000000000000000000, 0.8660254037844387076, 1.000000000000000000, 0.8660254037844387076, 1.000000000000000000, 0.8660254037844387076, 1.000000000000000000, 0.8660254037844387076, 1.000000000000000000, 0.8660254037844387076, 1.000000000000000000, 0.8660254037844387076, 1.000000000000000000, 0.8660254037844387076, 1.000000000000000000, 0.8660254037844387076, 1.000000000000000000, 0.8660254037844387076, 1.000000000000000000, 0.8660254037844387076, 1.000000000000000000, 0.8660254037844387076, 1.000000000000000000, 0.8660254037844387076, 1.000000000000000000, 0.8660254037844387076, 1.000000000000000000, 0.8660254037844387076, 1.000000000000000000, 0.8660254037844387076, 1.000000000000000000, 0.8660254037844387076, 1.000000000000000000, 0.8660254037844387076, 1.000000000000000000, 0.8660254037844387076, 1.000000000000000000, 0.8660254037844387076, 1.000000000000000000, 0.8660254037844387076, 1.000000000000000000, 0.8660254037844387076, 1.000000000000000000, 0.8660254037844387076, 1.000000000000000000, 0.8660254037844387076, 1.000000000000000000, 0.8660254037844387076, 1.000000000000000000, 0.8660254037844387076, 1.000000000000000000, 0.8660254037844387076, 1.000000000000000000, 0.8660254037844387076, 1.000000000000000000, 0.8660254037844387076, 1.000000000000000000, 0.8660254037844387076, 1.000000000000000000, 0.8660254037844387076, 1.000000000000000000, 0.8660254037844387076, 1.000000000000000000, 0.8660254037844387076, 1.000000000000000000, 0.8660254037844387076, 1.000000000000000000, 0.8660254037844387076, 1.000000000000000000, 0.8660254037844387076, 1.000000000000000000, 0.8660254037844387076, 1.000000000000000000, 0.8660254037844387076, 1.000000000000000000, 0.8660254037844387076, 1.000000000000000000, 0.8660254037844387076, 1.000000000000000000, 0.8660254037844387076, 1.000000000000000000, 0.8660254037844387076, 1.000000000000000000, 0.8660254037844387076, 1.000000000000000000, 0.8660254037844387076, 1.000000000000000000, 0.8660254037844387076, 1.000000000000000000, 0.8660254037844387076, 1.000000000000000000, 0.8660254037844387076, 1.000000000000000000, 0.8660254037844387076, 1.000000000000000000, 0.8660254037844387076, 1.000000000000000000, 0.8660254037844387076, 1.000000000000000000, 0.8660254037844387076, 1.000000000000000000, 0.8660254037844387076, 1.000000000000000000, 0.8660254037844387076, 1.000000000000000000, 0.8660254037844387076, 1.000000000000000000, 0.8660254037844387076, 1.000000000000000000, 0.8660254037844387076, 1.000000000000000000, 0.8660254037844387076, 1.000000000000000000, 0.8660254037844387076, 1.000000000000000000, 0.8660254037844387076, 1.000000000000000000, 0.8660254037844387076, 1.000000000000000000, 0.8660254037844387076, 1.000000000000000000, 0.8660254037844387076, 1.000000000000000000, 0.8660254037844387076, 1.000000000000000000, 0.8660254037844387076, 1.000000000000000000, 0.8660254037844387076, 1.000000000000000000, 0.8660254037844387076, 1.000000000000000000, 0.8660254037844387076, 1.000000000000000000, 0.8660254037844387076, 1.000000000000000000, 0.8660254037844387076, 1.000000000000000000, 0.8660254037844387076, 1.000000000000000000, 0.8660254037844387076, 1.000000000000000000, 0.8660254037844387076, 1.000000000000000000, 0.8660254037844387076, 1.000000000000000000, 0.8660254037844387076, 1.000000000000000000, 0.8660254037844387076, 1.000000000000000000, 0.8660254037844387076, 1.000000000000000000, 0.8660254037844387076, 1.000000000000000000, 0.8660254037844387076, 1.000000000000000000, 0.8660254037844387076, 1.000000000000000000, 0.8660254037844387076, 1.000000000000000000, 0.8660254037844387076, 1.000000000000000000, 0.8660254037844387076, 1.000000000000000000, 0.8660254037844387076, 1.000000000000000000, 0.8660254037844387076, 1.000000000000000000, 0.8660254037844387076, 1.000000000000000000, 0.8660254037844387076, 1.000000000000000000, 0.8660254037844387076, 1.000000000000000000, 0.8660254037844387076, 1.000000000000000000, 0.8660254037844387076, 1.000000000000000000, 0.8660254037844387076, 1.000000000000000000, 0.8660254037844387076, 1.000000000000000000, 0.8660254037844387076, 1.000000000000000000, 0.8660254037844387076, 1.000000000000000000, 0.8660254037844387076, 1.000000000000000000, 0.8660254037844387076, 1.000000000000000000, 0.8660254037844387076, 1.000000000000000000, 0.8660254037844387076, 1.000000000000000000, 0.8660254037844387076, 1.000000000000000000, 0.8660254037844387076, 1.000000000000000000, 0.8660254037844387076, 1.000000000000000000, 0.8660254037844387076, 1.000000000000000000, 0.8660254037844387076, 1.000000000000000000, 0.8660254037844387076, 1.000000000000000000, 0.8660254037844387076, 1.000000000000000000, 0.8660254037844387076, 1.000000000000000000, 0.8660254037844387076, 1.000000000000000000, 0.8660254037844387076, 1.000000000000000000, 0.8660254037844387076, 1.000000000000000000, 0.8660254037844387076, 1.000000000000000000, 0.8660254037844387076, 1.000000000000000000),
 ( 1.000000000000000000, 0.8660254037844387076, 1.000000000000000000, 0.8660254037844387076, 1.000000000000000000, 0.8660254037844387076, 1.000000000000000000, 0.8660254037844387076, 1.000000000000000000, 0.8660254037844387076, 1.000000000000000000, 0.8660254037844387076, 1.000000000000000000, 0.8660254037844387076, 1.000000000000000000, 0.8660254037844387076, 1.000000000000000000, 0.8660254037844387076, 1.000000000000000000, 0.8660254037844387076, 1.000000000000000000, 0.8660254037844387076, 1.000000000000000000, 0.8660254037844387076, 1.000000000000000000, 0.8660254037844387076, 1.000000000000000000, 0.8660254037844387076, 1.000000000000000000, 0.8660254037844387076, 1.000000000000000000, 0.8660254037844387076, 1.000000000000000000, 0.8660254037844387076, 1.000000000000000000, 0.8660254037844387076, 1.000000000000000000, 0.8660254037844387076, 1.000000000000000000, 0.8660254037844387076, 1.000000000000000000, 0.8660254037844387076, 1.000000000000000000, 0.8660254037844387076, 1.000000000000000000, 0.8660254037844387076, 1.000000000000000000, 0.8660254037844387076, 1.000000000000000000, 0.8660254037844387076, 1.000000000000000000, 0.8660254037844387076, 1.000000000000000000, 0.8660254037844387076, 1.000000000000000000, 0.8660254037844387076, 1.000000000000000000, 0.8660254037844387076, 1.000000000000000000, 0.8660254037844387076, 1.000000000000000000, 0.8660254037844387076, 1.000000000000000000, 0.8660254037844387076, 1.000000000000000000, 0.8660254037844387076, 1.000000000000000000, 0.8660254037844387076, 1.000000000000000000, 0.8660254037844387076, 1.000000000000000000, 0.8660254037844387076, 1.000000000000000000, 0.8660254037844387076, 1.000000000000000000, 0.8660254037844387076, 1.000000000000000000, 0.8660254037844387076, 1.000000000000000000, 0.8660254037844387076, 1.000000000000000000, 0.8660254037844387076, 1.000000000000000000, 0.8660254037844387076, 1.000000000000000000, 0.8660254037844387076, 1.000000000000000000, 0.8660254037844387076, 1.000000000000000000, 0.8660254037844387076, 1.000000000000000000, 0.8660254037844387076, 1.000000000000000000, 0.8660254037844387076, 1.000000000000000000, 0.8660254037844387076, 1.000000000000000000, 0.8660254037844387076, 1.000000000000000000, 0.8660254037844387076, 1.000000000000000000, 0.8660254037844387076, 1.000000000000000000, 0.8660254037844387076, 1.000000000000000000, 0.8660254037844387076, 1.000000000000000000, 0.8660254037844387076, 1.000000000000000000, 0.8660254037844387076, 1.000000000000000000, 0.8660254037844387076, 1.000000000000000000, 0.8660254037844387076, 1.000000000000000000, 0.8660254037844387076, 1.000000000000000000, 0.8660254037844387076, 1.000000000000000000, 0.8660254037844387076, 1.000000000000000000, 0.8660254037844387076, 1.000000000000000000, 0.8660254037844387076, 1.000000000000000000, 0.8660254037844387076, 1.000000000000000000, 0.8660254037844387076, 1.000000000000000000, 0.8660254037844387076, 1.000000000000000000, 0.8660254037844387076, 1.000000000000000000, 0.8660254037844387076, 1.000000000000000000, 0.8660254037844387076, 1.000000000000000000, 0.8660254037844387076, 1.000000000000000000, 0.8660254037844387076, 1.000000000000000000, 0.8660254037844387076, 1.000000000000000000, 0.8660254037844387076, 1.000000000000000000, 0.8660254037844387076, 1.000000000000000000, 0.8660254037844387076, 1.000000000000000000, 0.8660254037844387076, 1.000000000000000000, 0.8660254037844387076, 1.000000000000000000, 0.8660254037844387076, 1.000000000000000000, 0.8660254037844387076, 1.000000000000000000, 0.8660254037844387076, 1.000000000000000000, 0.8660254037844387076, 1.000000000000000000, 0.8660254037844387076, 1.000000000000000000, 0.8660254037844387076, 1.000000000000000000, 0.8660254037844387076, 1.000000000000000000, 0.8660254037844387076, 1.000000000000000000, 0.8660254037844387076, 1.000000000000000000, 0.8660254037844387076, 1.000000000000000000, 0.8660254037844387076, 1.000000000000000000, 0.8660254037844387076, 1.000000000000000000, 0.8660254037844387076, 1.000000000000000000, 0.8660254037844387076, 1.000000000000000000, 0.8660254037844387076, 1.000000000000000000, 0.8660254037844387076, 1.000000000000000000, 0.8660254037844387076, 1.000000000000000000, 0.8660254037844387076, 1.000000000000000000, 0.8660254037844387076, 1.000000000000000000, 0.8660254037844387076, 1.000000000000000000, 0.8660254037844387076, 1.000000000000000000, 0.8660254037844387076, 1.000000000000000000, 0.8660254037844387076, 1.000000000000000000, 0.8660254037844387076, 1.000000000000000000, 0.8660254037844387076, 1.000000000000000000, 0.8660254037844387076, 1.000000000000000000, 0.8660254037844387076, 1.000000000000000000, 0.8660254037844387076, 1.000000000000000000, 0.8660254037844387076, 1.000000000000000000, 0.8660254037844387076, 1.000000000000000000, 0.8660254037844387076, 1.000000000000000000, 0.8660254037844387076, 1.000000000000000000, 0.8660254037844387076, 1.000000000000000000, 0.8660254037844387076, 1.000000000000000000, 0.8660254037844387076, 1.000000000000000000, 0.8660254037844387076, 1.000000000000000000, 0.8660254037844387076, 1.000000000000000000, 0.8660254037844387076, 1.000000000000000000, 0.8660254037844387076, 1.000000000000000000, 0.8660254037844387076, 1.000000000000000000, 0.8660254037844387076, 1.000000000000000000, 0.8660254037844387076, 1.000000000000000000, 0.8660254037844387076, 1.000000000000000000, 0.8660254037844387076, 1.000000000000000000) ) ) 
 REPRESENTATION_ITEM ( '' )  SURFACE ( )  );
#111292=CARTESIAN_POINT ( 'NONE',  ( -5.506019780925599960, 5.596313630600862510, 0.7216878364870257245 ) ) ;
#111297=CARTESIAN_POINT ( 'NONE',  ( -5.123001941117347080, 7.070197912760590064, 1.599625672291263179 ) ) ;
#111317=CARTESIAN_POINT ( 'NONE',  ( -7.117104292530948229, 7.267986194233038155, -0.7998128361456362523 ) ) ;
#111319=CARTESIAN_POINT ( 'NONE',  ( -5.652823702255029836, 5.559658838911111900, -0.7998128361456362523 ) ) ;
#111324=ADVANCED_FACE ( 'NONE', ( #151662 ), #44309, .T. ) ;
#111344=CARTESIAN_POINT ( 'NONE',  ( -5.094831863685302942, 9.165997284266655498, 0.7998128361456291469 ) ) ;
#111370=CARTESIAN_POINT ( 'NONE',  ( 5.840530312436913007, 10.03597880781023299, 0.000000000000000000 ) ) ;
#111372=CARTESIAN_POINT ( 'NONE',  ( 5.332099551924443404, 9.442809587212341427, 0.000000000000000000 ) ) ;
#111386=CARTESIAN_POINT ( 'NONE',  ( 5.220047253295719614, 7.706380104734268599, 1.202949228536150938 ) ) ;
#111389=CARTESIAN_POINT ( 'NONE',  ( 6.699137298928145690, 8.909022496873262753, 1.443375672974065660 ) ) ;
#111394=CARTESIAN_POINT ( 'NONE',  ( -5.635349125135588721, 6.603604063193491136, 1.199719254218452935 ) ) ;
#111396=VERTEX_POINT ( 'NONE', #42185 ) ;
#111401=CARTESIAN_POINT ( 'NONE',  ( -4.773879485343255347, 8.583626809626847987, 0.000000000000000000 ) ) ;
#111419=CARTESIAN_POINT ( 'NONE',  ( 6.912678218121202534, 9.158153569265168770, 1.599625672291268286 ) ) ;
#111439=CARTESIAN_POINT ( 'NONE',  ( -7.910256278930404505, 8.193330178365746619, -0.7998128361456362523 ) ) ;
#111441=CARTESIAN_POINT ( 'NONE',  ( -3.752568318859959007, 7.355240624044412812, 0.6449737300090957470 ) ) ;
#111442=CARTESIAN_POINT ( 'NONE',  ( 5.397027666691686321, 8.454226823519094935, 1.199719254218451159 ) ) ;
#111444=CARTESIAN_POINT ( 'NONE',  ( -5.258916259484140099, 7.686978671390940043, 1.214082833407425621 ) ) ;
#111450=CARTESIAN_POINT ( 'NONE',  ( 4.179656494762836516, 8.098292687190454586, -0.7998128361456362523 ) ) ;
#111458=CARTESIAN_POINT ( 'NONE',  ( 3.933273961740298752, 5.682181936820735579, 1.443375672974058777 ) ) ;
#111462=CARTESIAN_POINT ( 'NONE',  ( 5.072158865288233898, 7.971250205261355859, 1.082531754730549078 ) ) ;
#111473=CARTESIAN_POINT ( 'NONE',  ( -5.478903473698260029, 6.525047153136981137, -1.082531754730549967 ) ) ;
#111501=ORIENTED_EDGE ( 'NONE', *, *, #27143, .T. ) ;
#111505=CARTESIAN_POINT ( 'NONE',  ( 6.229045230835819069, 6.231917288922055320, -0.7998128361456481317 ) ) ;
#111517=CARTESIAN_POINT ( 'NONE',  ( -3.984117037569407938, 5.741498858621315371, 1.599625672291270506 ) ) ;
#111520=CARTESIAN_POINT ( 'NONE',  ( 3.892599500454941630, 6.595097612955829192, 1.082531754730549078 ) ) ;
#111537=CARTESIAN_POINT ( 'NONE',  ( -3.662110889467009578, 7.286563447771212232, 0.7216878364870338292 ) ) ;
#111544=CARTESIAN_POINT ( 'NONE',  ( -4.715984300600573498, 7.775727532590477331, -0.9995835380776016965 ) ) ;
#111564=CARTESIAN_POINT ( 'NONE',  ( 5.575758015699216585, 5.849789923344298259, -0.7899890411014517388 ) ) ;
#111573=CARTESIAN_POINT ( 'NONE',  ( -6.831329296439251131, 9.063246493969506545, -1.599625672291271394 ) ) ;
#111574=CARTESIAN_POINT ( 'NONE',  ( -4.936046011350697427, 8.098431898006973384, 1.075429046246343612 ) ) ;
#111580=CARTESIAN_POINT ( 'NONE',  ( 0.000000000000000000, 8.499999999999996447, 0.000000000000000000 ) ) ;
#111582=CARTESIAN_POINT ( 'NONE',  ( -5.340986169140711226, 5.195848383611072485, 0.000000000000000000 ) ) ;
#111585=CARTESIAN_POINT ( 'NONE',  ( -5.842637852846353397, 5.781108681267656202, 0.7998128361456281477 ) ) ;
#111594=CARTESIAN_POINT ( 'NONE',  ( -3.031872956992967882, 6.300826765685804354, -0.7659957782561641615 ) ) ;
#111600=CARTESIAN_POINT ( 'NONE',  ( 4.603875680292229156, 7.528882839386387360, 1.199719254218452047 ) ) ;
#111623=CARTESIAN_POINT ( 'NONE',  ( 6.690022453700429139, 6.769724048930809701, 0.7998128361456331437 ) ) ;
#111624=CARTESIAN_POINT ( 'NONE',  ( 3.953084306836263995, 6.769626237021087789, 1.199719254218452047 ) ) ;
#111626=CARTESIAN_POINT ( 'NONE',  ( 3.878514461961128479, 6.682628084666728085, -1.199719254218448494 ) ) ;
#111639=CARTESIAN_POINT ( 'NONE',  ( 4.636584873806110174, 8.438537862545894441, 0.4145994950837776916 ) ) ;
#111640=CARTESIAN_POINT ( 'NONE',  ( -6.902509602688830626, 7.225551755991315162, -0.7216878364870338292 ) ) ;
#111660=CARTESIAN_POINT ( 'NONE',  ( 0.1054570145121072472, 2.614151819895196738, -2.076146791065091701 ) ) ;
#111669=CARTESIAN_POINT ( 'NONE',  ( 6.201928923608456046, 6.200281597156833691, 0.7998128361456352531 ) ) ;
#111677=FACE_OUTER_BOUND ( 'NONE', #116739, .T. ) ;
#111687=CARTESIAN_POINT ( 'NONE',  ( -5.745623237141265882, 9.925253886631958622, 0.7998128361456291469 ) ) ;
#111694=CARTESIAN_POINT ( 'NONE',  ( -7.013428937081412684, 5.939655416065874327, 2.436399677959149468 ) ) ;
#111699=CARTESIAN_POINT ( 'NONE',  ( 5.559725510055676168, 8.644040974110419384, 1.199719254218451159 ) ) ;
#111704=CARTESIAN_POINT ( 'NONE',  ( 4.227110032410640095, 8.153655147779589996, 0.7998128361456271485 ) ) ;
#111735=CARTESIAN_POINT ( 'NONE',  ( -5.119085517611572378, 8.129960982925583224, 1.199719254218452935 ) ) ;
#111737=CARTESIAN_POINT ( 'NONE',  ( 5.224688093219824303, 7.188831756880171397, -1.599625672291283607 ) ) ;
#111739=DIRECTION ( 'NONE',  ( -1.224646799147353207E-16, 1.000000000000000000, 0.000000000000000000 ) ) ;
#111741=CARTESIAN_POINT ( 'NONE',  ( -5.803772275101700906, 8.928762199997411386, -1.199719254218452047 ) ) ;
#111744=CARTESIAN_POINT ( 'NONE',  ( 5.840530312436913007, 10.03597880781023299, 0.000000000000000000 ) ) ;
#111745=PLANE ( 'NONE',  #64990 ) ;
#111749=CARTESIAN_POINT ( 'NONE',  ( -0.4134159855572216435, 2.995616482383578028, -2.020255554130489184 ) ) ;
#111767=CARTESIAN_POINT ( 'NONE',  ( 5.058600711674583472, 8.915801573680086634, 0.000000000000000000 ) ) ;
#111772=EDGE_LOOP ( 'NONE', ( #91656, #83332, #65239, #71627 ) ) ;
#111774=EDGE_CURVE ( 'NONE', #29321, #128826, #141217, .T. ) ;
#111783=CARTESIAN_POINT ( 'NONE',  ( -4.828112100242303306, 4.805421336470338645, -0.7216878364870338292 ) ) ;
#111787=CARTESIAN_POINT ( 'NONE',  ( 5.598591087800349086, 5.496387455380669529, -0.7998128361456481317 ) ) ;
#111802=ORIENTED_EDGE ( 'NONE', *, *, #11046, .T. ) ;
#111803=CARTESIAN_POINT ( 'NONE',  ( 6.391719147208887897, 6.567463349398139805, 2.438448605600926467 ) ) ;
#111843=CARTESIAN_POINT ( 'NONE',  ( -3.960390268523300339, 7.634556056670224855, 1.214306433183764966E-14 ) ) ;
#111849=CARTESIAN_POINT ( 'NONE',  ( -5.855142236255304944, 7.924361590421551860, -1.599625672291271394 ) ) ;
#111858=CARTESIAN_POINT ( 'NONE',  ( -5.652823702255029836, 5.559658838911111900, -0.7998128361456362523 ) ) ;
#111860=CARTESIAN_POINT ( 'NONE',  ( 5.770588788983777917, 7.358121641400980018, 1.301467365913897112 ) ) ;
#111865=CARTESIAN_POINT ( 'NONE',  ( 4.206772801990143584, 8.129928378955675328, 0.7998128361456271485 ) ) ;
#111872=CARTESIAN_POINT ( 'NONE',  ( -5.178288325776719603, 5.006034233019745372, 0.000000000000000000 ) ) ;
#111877=CARTESIAN_POINT ( 'NONE',  ( -6.445975688654487001, 6.485002823043819475, -0.7998128361456362523 ) ) ;
#111881=CARTESIAN_POINT ( 'NONE',  ( 5.682275777458841048, 8.683053269460405232, 1.082531754730547524 ) ) ;
#111883=CARTESIAN_POINT ( 'NONE',  ( -5.261973015435229328, 9.153069261400824885, 0.000000000000000000 ) ) ;
#111890=CARTESIAN_POINT ( 'NONE',  ( 4.746236293235721604, 7.694970221153795364, 1.199719254218451159 ) ) ;
#111896=CARTESIAN_POINT ( 'NONE',  ( 5.367048706163316751, 7.354919138647580290, -1.599625672291281386 ) ) ;
#111897=EDGE_CURVE ( 'NONE', #209619, #84144, #194679, .T. ) ;
#111899=CARTESIAN_POINT ( 'NONE',  ( -4.042674711113225960, 3.868317915292367015, -2.500000000000000444 ) ) ;
#111922=CARTESIAN_POINT ( 'NONE',  ( 4.601545839464173504, 8.365386937211251706, 0.1680730238927778675 ) ) ;
#111929=CARTESIAN_POINT ( 'NONE',  ( 5.668190738965027897, 8.770583741171307679, -1.199719254218452047 ) ) ;
#111934=CARTESIAN_POINT ( 'NONE',  ( -4.699286343732877569, 8.265425651823845143, 0.5948934201362279239 ) ) ;
#111941=CARTESIAN_POINT ( 'NONE',  ( -5.126391479298592735, 5.153413945369351268, 0.000000000000000000 ) ) ;
#111951=CARTESIAN_POINT ( 'NONE',  ( -4.950662367645459305, 5.804802846121667415, -1.199719254218453823 ) ) ;
#111953=CARTESIAN_POINT ( 'NONE',  ( 6.933015448541703485, 9.181880338089085214, 1.599625672291268286 ) ) ;
#111956=FACE_OUTER_BOUND ( 'NONE', #61888, .T. ) ;
#111962=CARTESIAN_POINT ( 'NONE',  ( 5.554000203453580475, 6.508696987897830688, -1.199719254218452047 ) ) ;
#111965=CARTESIAN_POINT ( 'NONE',  ( 6.007671464186837618, 6.181573927739029806, 0.7216878364870328300 ) ) ;
#111968=VERTEX_POINT ( 'NONE', #33366 ) ;
#111972=VECTOR ( 'NONE', #151798, 1000.000000000000000 ) ;
#111982=CARTESIAN_POINT ( 'NONE',  ( -5.646044625448194410, 5.551749915969804938, 0.000000000000000000 ) ) ;
#111983=CARTESIAN_POINT ( 'NONE',  ( 5.727393547130178675, 5.646656991265468939, 0.000000000000000000 ) ) ;
#111987=AXIS2_PLACEMENT_3D ( 'NONE', #205270, #156557, #203135 ) ;
#111994=CARTESIAN_POINT ( 'NONE',  ( -7.422162748838431412, 7.623887726591770608, -0.7998128361456362523 ) ) ;
#111995=CARTESIAN_POINT ( 'NONE',  ( 5.318541398310776103, 9.426991741329731056, -0.7998128361456481317 ) ) ;
#111997=CARTESIAN_POINT ( 'NONE',  ( 6.658462837642789012, 9.821938173008357253, 1.082531754730549078 ) ) ;
#111999=VERTEX_POINT ( 'NONE', #178569 ) ;
#112002=FACE_OUTER_BOUND ( 'NONE', #51325, .T. ) ;
#112008=CARTESIAN_POINT ( 'NONE',  ( -5.962047440371475382, 7.122956488241998230, -1.095284208787988822 ) ) ;
#112016=CARTESIAN_POINT ( 'NONE',  ( -6.420668264523499147, 9.648474187656182366, 1.199719254218452935 ) ) ;
#112032=CARTESIAN_POINT ( 'NONE',  ( 4.667750024854814050, 8.667735138964429709, -0.7998128361456381397 ) ) ;
#112034=EDGE_CURVE ( 'NONE', #138713, #105777, #8037, .T. ) ;
#112067=CARTESIAN_POINT ( 'NONE',  ( 3.040771591214902259, 6.769593633051179005, -0.7998128361456362523 ) ) ;
#112074=EDGE_CURVE ( 'NONE', #47959, #26714, #30324, .T. ) ;
#112082=EDGE_CURVE ( 'NONE', #135468, #99737, #125740, .T. ) ;
#112083=CARTESIAN_POINT ( 'NONE',  ( -9.336326716892651589, -1.000000000000000888, 2.500000000000000444 ) ) ;
#112097=ORIENTED_EDGE ( 'NONE', *, *, #169486, .F. ) ;
#112098=CARTESIAN_POINT ( 'NONE',  ( -6.168033539574333979, 6.160736982450306876, 0.7998128361456281477 ) ) ;
#112100=CARTESIAN_POINT ( 'NONE',  ( 5.167065940139554669, 9.042344340222555843, -0.7216878364870458196 ) ) ;
#112105=CARTESIAN_POINT ( 'NONE',  ( -6.317173229324657413, 6.334733287159020954, 0.000000000000000000 ) ) ;
#112111=CARTESIAN_POINT ( 'NONE',  ( -3.122120512896910505, 6.864500708346841229, 0.7998128361456352531 ) ) ;
#112116=CARTESIAN_POINT ( 'NONE',  ( -6.459533842268148973, 6.500820668926428958, 0.000000000000000000 ) ) ;
#112125=CARTESIAN_POINT ( 'NONE',  ( -4.176793841461789114, 7.030620694084159794, -1.199719254218455378 ) ) ;
#112130=CARTESIAN_POINT ( 'NONE',  ( -5.424670859243583720, 8.382514198209223721, 1.082531754730550855 ) ) ;
#112131=CARTESIAN_POINT ( 'NONE',  ( -5.763624699140868834, 9.738329559057408602, -0.7216878364870338292 ) ) ;
#112132=CARTESIAN_POINT ( 'NONE',  ( 5.905458427204159477, 9.047396044116986502, 1.199719254218452047 ) ) ;
#112133=CARTESIAN_POINT ( 'NONE',  ( -7.065734331377342414, 8.272386803808890576, -1.199719254218452047 ) ) ;
#112148=B_SPLINE_CURVE_WITH_KNOTS ( 'NONE', 3,
 ( #185335, #34817, #33762, #52154, #169093, #166979, #67299, #17489 ),
 .UNSPECIFIED., .F., .F.,
 ( 4, 2, 2, 4 ),
 ( 0.000000000000000000, 0.0006775471553183762393, 0.001016320732977563437, 0.001355094310636750744 ),
 .UNSPECIFIED. ) ;
#112171=CARTESIAN_POINT ( 'NONE',  ( 4.893454165248502186, 8.027304163657891678, -0.9628252682179049282 ) ) ;
#112185=CARTESIAN_POINT ( 'NONE',  ( 4.864343252252968597, 8.897093904262280972, 0.000000000000000000 ) ) ;
#112188=CARTESIAN_POINT ( 'NONE',  ( -6.140917232347002042, 6.129101290685087911, -0.7998128361456362523 ) ) ;
#112192=CARTESIAN_POINT ( 'NONE',  ( -7.743115126736118015, 8.206258200713163475, 0.7216878364870317197 ) ) ;
#112202=CARTESIAN_POINT ( 'NONE',  ( 7.506374323821472849, 8.786466794993730289, -1.199719254218452047 ) ) ;
#112203=CARTESIAN_POINT ( 'NONE',  ( 4.993145711582793744, 9.047363440147082159, -0.7998128361456481317 ) ) ;
#112207=CARTESIAN_POINT ( 'NONE',  ( -4.832429956831352236, 4.840456299650983674, 0.2774298518010898662 ) ) ;
#112216=CARTESIAN_POINT ( 'NONE',  ( 5.203297092594585393, 9.292540051327542017, 0.7998128361456341429 ) ) ;
#112230=CARTESIAN_POINT ( 'NONE',  ( -5.858531774880906262, 6.967946837850073294, 1.082531754730549078 ) ) ;
#112231=CARTESIAN_POINT ( 'NONE',  ( -5.562588163356775972, 9.711712967216715953, 0.7998128361456291469 ) ) ;
#112242=CARTESIAN_POINT ( 'NONE',  ( -7.065207446497166366, 9.336104335703744539, 0.000000000000000000 ) ) ;
#112243=CARTESIAN_POINT ( 'NONE',  ( 7.686546744304875389, 7.932335721302671949, 0.7998128361456291469 ) ) ;
#112246=CARTESIAN_POINT ( 'NONE',  ( 4.380693030546916944, 6.204170850428461392, 1.443375672974058777 ) ) ;
#112259=CARTESIAN_POINT ( 'NONE',  ( -6.143440778383317813, 6.339971461045375456, 7.509178883279419847E-06 ) ) ;
#112262=CARTESIAN_POINT ( 'NONE',  ( 5.037736595929563244, 8.035053907629919223, -1.199719254218452047 ) ) ;
#112264=CARTESIAN_POINT ( 'NONE',  ( -3.806807270387036368, 7.663301925418665839, 0.000000000000000000 ) ) ;
#112276=CARTESIAN_POINT ( 'NONE',  ( 6.753369913382843315, 8.011924666102361314, -1.082531754730548412 ) ) ;
#112279=CARTESIAN_POINT ( 'NONE',  ( -5.094831863685302942, 9.165997284266655498, 0.7998128361456291469 ) ) ;
#112280=CARTESIAN_POINT ( 'NONE',  ( 6.391743074199808916, 6.421731439513382433, -0.7998128361456481317 ) ) ;
#112289=CARTESIAN_POINT ( 'NONE',  ( -4.014095998097799267, 6.840806543492835345, -1.199719254218450271 ) ) ;
#112292=CARTESIAN_POINT ( 'NONE',  ( -0.4000000000000114575, 2.999999999999999112, 2.023857702507764422 ) ) ;
#112318=CARTESIAN_POINT ( 'NONE',  ( 4.502716413514295191, 6.346531463890372926, -1.443375672974068769 ) ) ;
#112324=CARTESIAN_POINT ( 'NONE',  ( 4.041739190205284160, 7.729463131965888856, 0.000000000000000000 ) ) ;
#112331=VECTOR ( 'NONE', #147866, 1000.000000000000114 ) ;
#112332=EDGE_CURVE ( 'NONE', #137516, #95128, #68758, .T. ) ;
#112339=CARTESIAN_POINT ( 'NONE',  ( -6.967964602780620353, 7.093989889524320525, 0.000000000000000000 ) ) ;
#112341=CARTESIAN_POINT ( 'NONE',  ( -7.598418745816086783, 7.829519723065708092, 0.000000000000000000 ) ) ;
#112347=CARTESIAN_POINT ( 'NONE',  ( 6.933015448541703485, 9.181880338089085214, 1.599625672291268286 ) ) ;
#112352=CARTESIAN_POINT ( 'NONE',  ( -6.473091995881817162, 6.516638514809040217, 0.7998128361456281477 ) ) ;
#112358=CARTESIAN_POINT ( 'NONE',  ( -5.370438244788932280, 6.398504386076097283, 1.082531754730549078 ) ) ;
#112361=CARTESIAN_POINT ( 'NONE',  ( -6.473091995881817162, 6.516638514809040217, 0.7998128361456281477 ) ) ;
#112381=CARTESIAN_POINT ( 'NONE',  ( -4.055297343818976330, 5.824542549245813383, 1.443375672974065660 ) ) ;
#112383=CARTESIAN_POINT ( 'NONE',  ( -4.980641328173854632, 6.904110530993182948, 1.599625672291263179 ) ) ;
#112384=VERTEX_POINT ( 'NONE', #53898 ) ;
#112400=CIRCLE ( 'NONE', #115775, 0.07999999999999998779 ) ;
#112409=CARTESIAN_POINT ( 'NONE',  ( -6.363572996767778100, 8.517530811019446091, -1.599625672291271394 ) ) ;
#112420=AXIS2_PLACEMENT_3D ( 'NONE', #192646, #26952, #44299 ) ;
#112434=CARTESIAN_POINT ( 'NONE',  ( 6.318982112420993502, 9.529840343536603697, -1.199719254218452047 ) ) ;
#112435=CARTESIAN_POINT ( 'NONE',  ( 4.518610335104485287, 8.493738834255713854, 0.000000000000000000 ) ) ;
#112447=CARTESIAN_POINT ( 'NONE',  ( 4.816695983655697511, 8.110494931179941247, 0.8576603160085185529 ) ) ;
#112449=CARTESIAN_POINT ( 'NONE',  ( 7.200788982633824276, 7.573544365927161515, 0.000000000000000000 ) ) ;
#112453=AXIS2_PLACEMENT_3D ( 'NONE', #155572, #7155, #208556 ) ;
#112455=CARTESIAN_POINT ( 'NONE',  ( -4.553559489343377287, 6.405848385690952718, -1.599625672291271394 ) ) ;
#112460=ADVANCED_FACE ( 'NONE', ( #84852 ), #16258, .T. ) ;
#112462=CARTESIAN_POINT ( 'NONE',  ( -6.468648687051513413, 7.679749902049126220, 1.082531754730549078 ) ) ;
#112465=CARTESIAN_POINT ( 'NONE',  ( -5.800535780310947409, 5.989883198674579745, 0.3271122460986007896 ) ) ;
#112472=CARTESIAN_POINT ( 'NONE',  ( -4.309512724297390740, 6.121127159803966933, 1.599625672291270506 ) ) ;
#112482=CARTESIAN_POINT ( 'NONE',  ( 5.643937085038755797, 9.806620042512378177, -0.7998128361456481317 ) ) ;
#112502=CARTESIAN_POINT ( 'NONE',  ( 6.855582950365507244, 8.027210192628430718, -1.199719254218452047 ) ) ;
#112503=CARTESIAN_POINT ( 'NONE',  ( 0.000000000000000000, 0.08000000000000020983, 0.000000000000000000 ) ) ;
#112504=CARTESIAN_POINT ( 'NONE',  ( -5.615968211774352348, 7.384814024763004525, 1.238619054342107839 ) ) ;
#112510=CARTESIAN_POINT ( 'NONE',  ( 3.718679271898170491, 7.560485927181699317, 0.7998128361456271485 ) ) ;
#112516=CARTESIAN_POINT ( 'NONE',  ( 3.445180431648323882, 6.073108699348104267, 1.082531754730549078 ) ) ;
#112520=CARTESIAN_POINT ( 'NONE',  ( 6.753369913382843315, 8.011924666102361314, -1.082531754730548412 ) ) ;
#112532=CARTESIAN_POINT ( 'NONE',  ( -5.641601317062248988, 6.714861303728305586, -1.082531754730549967 ) ) ;
#112565=VERTEX_POINT ( 'NONE', #53103 ) ;
#112569=CARTESIAN_POINT ( 'NONE',  ( 6.042093733545556233, 7.078139439671806699, -1.199719254218452047 ) ) ;
#112571=CARTESIAN_POINT ( 'NONE',  ( 6.062430963966053632, 7.101866208495718702, -1.199719254218452047 ) ) ;
#112582=CARTESIAN_POINT ( 'NONE',  ( -4.228163802615396705, 6.026220084508304708, -1.599625672291271394 ) ) ;
#112586=CARTESIAN_POINT ( 'NONE',  ( 4.367134876933267407, 8.109091433148536865, 0.000000000000000000 ) ) ;
#112602=CARTESIAN_POINT ( 'NONE',  ( -6.970300371201519241, 7.304640985922785212, 0.7216878364870317197 ) ) ;
#112604=CARTESIAN_POINT ( 'NONE',  ( -4.990809943606281607, 6.915973915664348937, -1.443375672974066548 ) ) ;
#112608=FACE_OUTER_BOUND ( 'NONE', #107849, .T. ) ;
#112616=EDGE_CURVE ( 'NONE', #184155, #198714, #153329, .T. ) ;
#112621=ORIENTED_EDGE ( 'NONE', *, *, #24605, .F. ) ;
#112643=CARTESIAN_POINT ( 'NONE',  ( -5.435611771797328906, 7.629049766310559200, 1.344574814272103236 ) ) ;
#112649=DIRECTION ( 'NONE',  ( -0.000000000000000000, 1.000000000000000000, -0.000000000000000000 ) ) ;
#112651=CARTESIAN_POINT ( 'NONE',  ( -4.655245641445871385, 6.524482229810530498, 1.599625672291263179 ) ) ;
#112654=CARTESIAN_POINT ( 'NONE',  ( -4.305596300791617814, 7.180890229968955651, 1.199719254218452935 ) ) ;
#112665=CARTESIAN_POINT ( 'NONE',  ( 5.357406976055401948, 6.279338222599979424, 1.199719254218452935 ) ) ;
#112688=CARTESIAN_POINT ( 'NONE',  ( 5.987861119090863049, 7.014868056141362551, 1.199719254218452047 ) ) ;
#112689=CARTESIAN_POINT ( 'NONE',  ( 4.278479993564246797, 7.149254538203735798, 1.199719254218452047 ) ) ;
#112691=CARTESIAN_POINT ( 'NONE',  ( 3.607351389687783794, 6.366271167014519783, 1.199719254218451159 ) ) ;
#112704=CARTESIAN_POINT ( 'NONE',  ( 4.817101577040221905, 8.228953320636518853, 0.8951067572735508238 ) ) ;
#112705=CARTESIAN_POINT ( 'NONE',  ( -6.604230223188181093, 6.877559146573883453, 0.7216878364870317197 ) ) ;
#112706=CARTESIAN_POINT ( 'NONE',  ( -3.172739462086278550, 6.087116567132428990, 0.9300064228868381022 ) ) ;
#112728=CARTESIAN_POINT ( 'NONE',  ( -0.1950010711912115446, 2.645508648321929002, -2.067621631602482690 ) ) ;
#112735=CARTESIAN_POINT ( 'NONE',  ( 4.044074958626150185, 7.940114228364351767, 0.7998128361456271485 ) ) ;
#112737=CARTESIAN_POINT ( 'NONE',  ( 4.248501033035879004, 6.049946853332221153, -1.599625672291273171 ) ) ;
#112754=CARTESIAN_POINT ( 'NONE',  ( -8.120407659942227241, 8.438506789546210030, 0.7998128361456341429 ) ) ;
#112765=CARTESIAN_POINT ( 'NONE',  ( 6.879836604291781121, 6.991173891287354003, -0.7998128361456341429 ) ) ;
#112772=CARTESIAN_POINT ( 'NONE',  ( 6.561219994370630637, 6.619454513046008515, 0.000000000000000000 ) ) ;
#112783=CARTESIAN_POINT ( 'NONE',  ( 4.716601407767927689, 8.224641112169805979, 0.6639617910879731522 ) ) ;
#112794=CARTESIAN_POINT ( 'NONE',  ( -6.147147853355845015, 6.992553514990425434, 0.9364138244793998034 ) ) ;
#112802=CARTESIAN_POINT ( 'NONE',  ( -5.010620288702242853, 8.003418215864698482, -1.199719254218453823 ) ) ;
#112804=CARTESIAN_POINT ( 'NONE',  ( 6.710359684120930091, 6.793450817754725257, 0.7998128361456352531 ) ) ;
#112809=CARTESIAN_POINT ( 'NONE',  ( -6.749980374757255319, 8.968339418673846097, 1.599625672291269396 ) ) ;
#112816=CARTESIAN_POINT ( 'NONE',  ( -6.586110727467836767, 6.776993156853382771, -0.3129968654442937814 ) ) ;
#112826=CARTESIAN_POINT ( 'NONE',  ( 4.028659262336944380, 3.858644544030801704, 2.500000000000000000 ) ) ;
#112828=ORIENTED_EDGE ( 'NONE', *, *, #156704, .T. ) ;
#112832=CARTESIAN_POINT ( 'NONE',  ( 4.746763178560241769, 8.551991118380046331, 0.7216878364870328300 ) ) ;
#112835=CARTESIAN_POINT ( 'NONE',  ( -8.086512275908061653, 8.398962174839683215, 0.000000000000000000 ) ) ;
#112846=CARTESIAN_POINT ( 'NONE',  ( -3.839356663422469840, 7.492693387012709927, -0.03537628172997089177 ) ) ;
#112847=CARTESIAN_POINT ( 'NONE',  ( -4.882344714696960075, 5.829061934302122161, 1.082531754730549078 ) ) ;
#112851=CARTESIAN_POINT ( 'NONE',  ( 5.734172623936983904, 5.654565914206774124, 0.7998128361456352531 ) ) ;
#112865=ORIENTED_EDGE ( 'NONE', *, *, #143867, .F. ) ;
#112866=CARTESIAN_POINT ( 'NONE',  ( 4.495112795250098436, 8.049017979306480441, 2.444655174081866278 ) ) ;
#112869=CARTESIAN_POINT ( 'NONE',  ( 7.987161891782087686, 8.490979426600148372, -0.7216878364870317197 ) ) ;
#112896=CARTESIAN_POINT ( 'NONE',  ( 3.119784744920330422, 6.653849612466795627, 0.7216878364870257245 ) ) ;
#112903=CARTESIAN_POINT ( 'NONE',  ( -4.163660309340779797, 7.871692890607882021, 0.005041904348490143691 ) ) ;
#112906=CARTESIAN_POINT ( 'NONE',  ( -5.763624699140894592, 5.896852701852039580, -0.7216878364870338292 ) ) ;
#112911=ORIENTED_EDGE ( 'NONE', *, *, #151435, .T. ) ;
#112912=CARTESIAN_POINT ( 'NONE',  ( -4.990283058281743678, 7.979691447040783814, -1.199719254218453823 ) ) ;
#112921=CARTESIAN_POINT ( 'NONE',  ( -5.143339171537843590, 7.093924681584509173, 1.599625672291263179 ) ) ;
#112923=CARTESIAN_POINT ( 'NONE',  ( 6.430738266435902517, 6.882057634903050669, 0.7203813067775278745 ) ) ;
#112928=CARTESIAN_POINT ( 'NONE',  ( 4.694866332082116678, 8.699370830729650450, 0.7998128361456341429 ) ) ;
#112933=ORIENTED_EDGE ( 'NONE', *, *, #61052, .T. ) ;
#112934=CIRCLE ( 'NONE', #178566, 0.8300000000000008482 ) ;
#112936=DIRECTION ( 'NONE',  ( -1.000000000000000000, 2.090028284309406390E-15, 0.000000000000000000 ) ) ;
#112937=CARTESIAN_POINT ( 'NONE',  ( -5.327428015527048366, 5.180030537728460338, -0.7998128361456362523 ) ) ;
#112941=CARTESIAN_POINT ( 'NONE',  ( -5.798046968499580345, 6.793418213784815585, 1.199719254218452935 ) ) ;
#112945=CARTESIAN_POINT ( 'NONE',  ( 7.322812364712459221, 7.715904978352238430, 0.000000000000000000 ) ) ;
#112948=CARTESIAN_POINT ( 'NONE',  ( -6.739811759324831897, 7.996106819701333634, -1.082531754730549967 ) ) ;
#112954=CARTESIAN_POINT ( 'NONE',  ( 4.044074958626150185, 7.940114228364351767, 0.7998128361456271485 ) ) ;
#112955=ORIENTED_EDGE ( 'NONE', *, *, #177202, .F. ) ;
#112990=CARTESIAN_POINT ( 'NONE',  ( 7.075376061485196821, 9.347967719856493218, 1.599625672291268286 ) ) ;
#112995=CARTESIAN_POINT ( 'NONE',  ( -6.259328228163411723, 6.916251825828671151, -0.7980491773402348388 ) ) ;
#113003=CARTESIAN_POINT ( 'NONE',  ( -3.919715807682309094, 6.626733304721049933, 1.082531754730549967 ) ) ;
#113015=CARTESIAN_POINT ( 'NONE',  ( -6.563028877466991595, 9.814561569423593923, 1.199719254218452935 ) ) ;
#113022=ORIENTED_EDGE ( 'NONE', *, *, #188735, .T. ) ;
#113027=CARTESIAN_POINT ( 'NONE',  ( 3.867818961648523235, 7.734482231890414283, 1.040834085586084257E-14 ) ) ;
#113031=CARTESIAN_POINT ( 'NONE',  ( 4.977251789548238214, 7.860525283564661514, -1.082531754730548412 ) ) ;
#113039=CARTESIAN_POINT ( 'NONE',  ( 7.065207446497155708, 9.336104335703744539, 0.000000000000000000 ) ) ;
#113045=CARTESIAN_POINT ( 'NONE',  ( -5.144392941742557568, 4.966489618313220333, -0.7998128361456362523 ) ) ;
#113046=CARTESIAN_POINT ( 'NONE',  ( 4.203910148689107729, 7.062256385849379647, -1.199719254218448494 ) ) ;
#113057=CARTESIAN_POINT ( 'NONE',  ( -6.587282531393266360, 8.778525268082516320, 1.599625672291269396 ) ) ;
#113058=CARTESIAN_POINT ( 'NONE',  ( 6.530187263637528439, 7.647581891445782709, -1.199719254218452047 ) ) ;
#113065=CARTESIAN_POINT ( 'NONE',  ( 4.415115299905642665, 5.179997933758551554, -1.199719254218450271 ) ) ;
#113072=CARTESIAN_POINT ( 'NONE',  ( -6.419454189569741231, 6.887487763818779918, 0.7628848663763813098 ) ) ;
#113080=CARTESIAN_POINT ( 'NONE',  ( -5.139949632912262700, 5.169231791251960750, 0.7216878364870257245 ) ) ;
#113095=CARTESIAN_POINT ( 'NONE',  ( 5.830888582329017744, 8.960397891762626799, -1.199719254218452047 ) ) ;
#113128=CARTESIAN_POINT ( 'NONE',  ( 3.393283585170187688, 7.180857625999046867, 0.7998128361456271485 ) ) ;
#113129=CARTESIAN_POINT ( 'NONE',  ( -4.990809943606294929, 4.995235487061662205, -0.7216878364870338292 ) ) ;
#113161=CARTESIAN_POINT ( 'NONE',  ( -4.294900800479008574, 8.232744377192641849, 0.000000000000000000 ) ) ;
#113163=CARTESIAN_POINT ( 'NONE',  ( 5.343321937117211817, 9.247976336696488886, 0.000000000000000000 ) ) ;
#113168=CARTESIAN_POINT ( 'NONE',  ( -5.468734858265826837, 7.473552982767158070, 1.599625672291263179 ) ) ;
#113174=CARTESIAN_POINT ( 'NONE',  ( -5.008811405605897882, 4.808311159487113073, 0.7998128361456281477 ) ) ;
#113179=CARTESIAN_POINT ( 'NONE',  ( -5.424143973919053785, 8.485862515284315677, 1.199719254218454489 ) ) ;
#113190=CARTESIAN_POINT ( 'NONE',  ( -4.390861645979385663, 6.216034235099629157, -1.599625672291271394 ) ) ;
#113194=CARTESIAN_POINT ( 'NONE',  ( -4.800995793014949165, 8.615262501910491366, 0.7216878364870267237 ) ) ;
#113195=CARTESIAN_POINT ( 'NONE',  ( -6.089020385868862739, 8.197219431637373432, -1.443375672974066548 ) ) ;
#113196=CARTESIAN_POINT ( 'NONE',  ( 7.038618024149998043, 8.240751112043669835, -1.199719254218452047 ) ) ;
#113197=CARTESIAN_POINT ( 'NONE',  ( -5.932574734431526942, 9.079031735882207244, 1.199719254218454489 ) ) ;
#113216=CARTESIAN_POINT ( 'NONE',  ( -1.862912430430173627, 2.484159785402544784, -2.477813002740275827 ) ) ;
#113237=CARTESIAN_POINT ( 'NONE',  ( 5.170590401584001405, 7.751911629329717002, -1.182414590771277085 ) ) ;
#113252=CARTESIAN_POINT ( 'NONE',  ( 6.723917837734620484, 6.809268663637336516, 0.000000000000000000 ) ) ;
#113255=CARTESIAN_POINT ( 'NONE',  ( -5.306037014901836990, 7.283738832175834510, 1.599625672291263179 ) ) ;
#113259=CARTESIAN_POINT ( 'NONE',  ( -6.522881301506166629, 9.663759714182251770, 1.082531754730549967 ) ) ;
#113265=B_SPLINE_CURVE_WITH_KNOTS ( 'NONE', 3,
 ( #54255, #106252, #172276, #5460 ),
 .UNSPECIFIED., .F., .F.,
 ( 4, 4 ),
 ( 0.8646637866085976620, 1.000000000000000000 ),
 .UNSPECIFIED. ) ;
#113270=CARTESIAN_POINT ( 'NONE',  ( 4.050854035433010480, 7.948023151305657841, 0.000000000000000000 ) ) ;
#113272=CARTESIAN_POINT ( 'NONE',  ( 8.018721507839716267, 8.319872945426633137, -0.7998128361456341429 ) ) ;
#113280=CARTESIAN_POINT ( 'NONE',  ( 5.273195401072370281, 5.116759154198018855, -0.7998128361456481317 ) ) ;
#113286=CARTESIAN_POINT ( 'NONE',  ( 7.388267364804250725, 7.584343111885245570, -0.7998128361456341429 ) ) ;
#113299=CARTESIAN_POINT ( 'NONE',  ( -5.072158865288277418, 7.010880990960010273, 1.443375672974058777 ) ) ;
#113300=CARTESIAN_POINT ( 'NONE',  ( 5.614485009834906393, 6.683225611963085733, -1.082531754730548412 ) ) ;
#113313=CARTESIAN_POINT ( 'NONE',  ( -5.804299160426224624, 9.785783097223662352, -0.7216878364870338292 ) ) ;
#113314=CARTESIAN_POINT ( 'NONE',  ( 1.833030277982334422, 2.531131934864056632, -2.500000000000000444 ) ) ;
#113317=CARTESIAN_POINT ( 'NONE',  ( 5.858531774436539052, 6.007577623030311287, 0.000000000000000000 ) ) ;
#113334=CARTESIAN_POINT ( 'NONE',  ( 4.064412189046650248, 7.963840997188264659, 0.7998128361456271485 ) ) ;
#113336=CARTESIAN_POINT ( 'NONE',  ( -5.652823702255029836, 5.559658838911111900, -0.7998128361456362523 ) ) ;
#113345=CARTESIAN_POINT ( 'NONE',  ( 4.690609020473775814, 8.361801240329816309, 0.7176157125430505657 ) ) ;
#113349=CARTESIAN_POINT ( 'NONE',  ( 7.363486825997814123, 7.763358516518489516, 0.000000000000000000 ) ) ;
#113351=CARTESIAN_POINT ( 'NONE',  ( -7.119966945832006289, 8.335658187339330283, 1.199719254218452047 ) ) ;
#113352=CARTESIAN_POINT ( 'NONE',  ( 4.206772801990143584, 8.129928378955675328, 0.7998128361456271485 ) ) ;
#113361=CARTESIAN_POINT ( 'NONE',  ( -4.423703259808839938, 8.383013913077441259, 0.7998128361456352531 ) ) ;
#113373=DIRECTION ( 'NONE',  ( -1.000000000000000000, 0.000000000000000000, 0.000000000000000000 ) ) ;
#113379=VERTEX_POINT ( 'NONE', #171606 ) ;
#113387=CARTESIAN_POINT ( 'NONE',  ( 3.594320121398666856, 7.207474218358159490, -1.734723475976807094E-15 ) ) ;
#113393=CARTESIAN_POINT ( 'NONE',  ( 6.197485614778188712, 6.403023770095574108, -0.7216878364870458196 ) ) ;
#113408=CARTESIAN_POINT ( 'NONE',  ( -6.981522756394290319, 7.109807735406931783, 0.7998128361456341429 ) ) ;
#113410=CARTESIAN_POINT ( 'NONE',  ( -7.262327558775498737, 8.501745569106741840, 1.199719254218452047 ) ) ;
#113416=CARTESIAN_POINT ( 'NONE',  ( 5.826972158823246595, 10.02016096192762085, -0.7998128361456481317 ) ) ;
#113422=CARTESIAN_POINT ( 'NONE',  ( -4.586401103172829785, 8.572828063668767484, 0.7998128361456281477 ) ) ;
#113428=CARTESIAN_POINT ( 'NONE',  ( -5.329763783947941036, 5.390681634126922361, 0.000000000000000000 ) ) ;
#113431=CARTESIAN_POINT ( 'NONE',  ( -4.111865726694519552, 8.019203457777400956, 0.000000000000000000 ) ) ;
#113452=CARTESIAN_POINT ( 'NONE',  ( -5.935437387732586778, 10.14670372898850381, -0.7998128361456362523 ) ) ;
#113453=CARTESIAN_POINT ( 'NONE',  ( 3.237364818613055473, 6.998952398349030268, -1.734723475976807094E-15 ) ) ;
#113454=CARTESIAN_POINT ( 'NONE',  ( -4.294900800479008574, 8.232744377192641849, 0.000000000000000000 ) ) ;
#113455=EDGE_LOOP ( 'NONE', ( #179397, #206601, #146458 ) ) ;
#113479=CARTESIAN_POINT ( 'NONE',  ( -7.781453819600577582, 8.043060642480948985, 0.000000000000000000 ) ) ;
#113504=CARTESIAN_POINT ( 'NONE',  ( 7.862802741282558294, 8.137967717776607657, 0.000000000000000000 ) ) ;
#113505=CARTESIAN_POINT ( 'NONE',  ( 5.494797395288433250, 9.632623737803665875, 0.000000000000000000 ) ) ;
#113518=CARTESIAN_POINT ( 'NONE',  ( 5.975194856099406593, 7.098212677808693805, 1.080521340106417982 ) ) ;
#113520=CARTESIAN_POINT ( 'NONE',  ( 6.482206841109512396, 9.616306177052839743, -1.082531754730548412 ) ) ;
#113523=B_SPLINE_CURVE_WITH_KNOTS ( 'NONE', 3,
 ( #153358, #56922, #38541, #189052, #171733, #172820, #123095, #120936 ),
 .UNSPECIFIED., .F., .F.,
 ( 4, 2, 2, 4 ),
 ( 3.127317220692749988E-18, 0.003096353334791363508, 0.004644530002187043094, 0.006192706669582721812 ),
 .UNSPECIFIED. ) ;
#113527=CARTESIAN_POINT ( 'NONE',  ( -4.749098946536820520, 8.762642214260091933, 0.7998128361456281477 ) ) ;
#113530=TOROIDAL_SURFACE ( 'NONE', #92767, 0.8299999999999999600, 0.08000000000000000167 ) ;
#113533=CARTESIAN_POINT ( 'NONE',  ( -7.580417283372126391, 8.016444050121833698, 0.7216878364870317197 ) ) ;
#113536=CARTESIAN_POINT ( 'NONE',  ( -4.005587769924587427, 7.671888287421506192, 0.1631757730154441144 ) ) ;
#113543=CARTESIAN_POINT ( 'NONE',  ( -5.093022980588950865, 5.970890227889075419, -1.199719254218453823 ) ) ;
#113553=CARTESIAN_POINT ( 'NONE',  ( 4.706615602599436343, 5.520081620234675412, 1.199719254218452935 ) ) ;
#113574=CARTESIAN_POINT ( 'NONE',  ( -6.050681693448748177, 10.28115541899069463, 0.7998128361456291469 ) ) ;
#113577=CARTESIAN_POINT ( 'NONE',  ( 7.028976294042106332, 7.165170195996068969, 0.000000000000000000 ) ) ;
#113579=CARTESIAN_POINT ( 'NONE',  ( -5.171754443046126859, 7.767122556988016235, 1.178735681042131667 ) ) ;
#113585=CARTESIAN_POINT ( 'NONE',  ( 5.204350862799327793, 7.165104988056252289, -1.599625672291281386 ) ) ;
#113591=CARTESIAN_POINT ( 'NONE',  ( 2.929970594329034395, 6.432399770110250437, -0.7216878364870338292 ) ) ;
#113594=CARTESIAN_POINT ( 'NONE',  ( 6.916067756746836714, 8.201738816693689316, -1.082531754730548412 ) ) ;
#113604=CARTESIAN_POINT ( 'NONE',  ( -5.804299160426242388, 6.904675454319632699, -1.082531754730549967 ) ) ;
#113640=CARTESIAN_POINT ( 'NONE',  ( 3.881377115262159894, 7.750300077773022878, 0.7998128361456271485 ) ) ;
#113642=CARTESIAN_POINT ( 'NONE',  ( 5.899733120602060232, 6.912052057904395141, -1.199719254218452047 ) ) ;
#113655=CARTESIAN_POINT ( 'NONE',  ( -5.144392941742557568, 4.966489618313220333, -0.7998128361456362523 ) ) ;
#113658=CARTESIAN_POINT ( 'NONE',  ( 5.031484404002879884, 6.963427452793765404, 1.443375672974065660 ) ) ;
#113671=CARTESIAN_POINT ( 'NONE',  ( -6.292392690518214593, 7.474117906093608710, -1.082531754730549967 ) ) ;
#113673=CARTESIAN_POINT ( 'NONE',  ( -6.156811154381562012, 6.355570232966157640, 0.7216878364870257245 ) ) ;
#113681=CARTESIAN_POINT ( 'NONE',  ( -5.571360081631161698, 7.090533140868425122, -1.217465838365646258 ) ) ;
#113703=CARTESIAN_POINT ( 'NONE',  ( -3.644109427023046521, 7.473487774827342278, 0.000000000000000000 ) ) ;
#113713=CARTESIAN_POINT ( 'NONE',  ( -6.074935347375019390, 9.245119117649618801, 1.199719254218452047 ) ) ;
#113714=CARTESIAN_POINT ( 'NONE',  ( -4.587973201513257493, 8.494803767824503637, 0.1163994284540965235 ) ) ;
#113719=CARTESIAN_POINT ( 'NONE',  ( -6.061904078641520144, 10.08632216847484031, 0.7216878364870267237 ) ) ;
#113722=CARTESIAN_POINT ( 'NONE',  ( -5.652823702255029836, 5.559658838911111900, -0.7998128361456362523 ) ) ;
#113733=CARTESIAN_POINT ( 'NONE',  ( 6.249382461256315580, 6.255644057745969988, -0.7998128361456481317 ) ) ;
#113759=CARTESIAN_POINT ( 'NONE',  ( 4.681308178468477799, 8.683552984847038303, 0.000000000000000000 ) ) ;
#113760=CARTESIAN_POINT ( 'NONE',  ( 3.874598038455354665, 7.742391154831717692, -0.7998128361456362523 ) ) ;
#113762=CARTESIAN_POINT ( 'NONE',  ( 3.067887898442204442, 6.801229324816399746, 0.7998128361456271485 ) ) ;
#113765=DIRECTION ( 'NONE',  ( 0.000000000000000000, 1.000000000000000000, 0.000000000000000000 ) ) ;
#113773=CARTESIAN_POINT ( 'NONE',  ( 4.597876849858236525, 8.486543085689454813, -0.1053875944492469602 ) ) ;
#113774=CARTESIAN_POINT ( 'NONE',  ( -4.787437638956927977, 7.639075441208117212, -1.082531754730549967 ) ) ;
#113775=CARTESIAN_POINT ( 'NONE',  ( -2.978854731913820775, 6.490225589564778019, 0.1926073594339854922 ) ) ;
#113801=CARTESIAN_POINT ( 'NONE',  ( 5.285699784481295183, 7.260012063351913625, 1.599625672291268286 ) ) ;
#113803=CARTESIAN_POINT ( 'NONE',  ( 3.074666975249065626, 6.809138247757705820, 0.000000000000000000 ) ) ;
#113824=CARTESIAN_POINT ( 'NONE',  ( -7.930593509350902792, 8.217056947189661287, -0.7998128361456362523 ) ) ;
#113826=ORIENTED_EDGE ( 'NONE', *, *, #176689, .F. ) ;
#113838=CARTESIAN_POINT ( 'NONE',  ( 5.234329823327693809, 8.264412672927770487, 1.199719254218451159 ) ) ;
#113842=CARTESIAN_POINT ( 'NONE',  ( 6.737475991348287785, 6.825086509519945999, -0.7998128361456481317 ) ) ;
#113852=CARTESIAN_POINT ( 'NONE',  ( -1.890105089649204206, 8.991484090553308661, 0.7750000000000013545 ) ) ;
#113853=ADVANCED_FACE ( 'NONE', ( #95733 ), #115216, .T. ) ;
#113854=CARTESIAN_POINT ( 'NONE',  ( 4.664027441776592120, 8.287593892024585074, -0.5126927951675692707 ) ) ;
#113862=CARTESIAN_POINT ( 'NONE',  ( 4.095971805104268171, 7.792734516014752977, 0.7216878364870203955 ) ) ;
#113868=CARTESIAN_POINT ( 'NONE',  ( -6.001249869575842943, 7.094842513680024609, 1.067311936143347406 ) ) ;
#113876=CARTESIAN_POINT ( 'NONE',  ( -6.631873415740034083, 7.766215735565355160, 1.199719254218452047 ) ) ;
#113878=CARTESIAN_POINT ( 'NONE',  ( 5.794130544993763898, 7.853181283949808744, 1.599625672291269396 ) ) ;
#113880=CARTESIAN_POINT ( 'NONE',  ( 3.791513125430877373, 7.352524219418101303, -0.3677586026353037996 ) ) ;
#113882=CARTESIAN_POINT ( 'NONE',  ( -6.668631453075260396, 8.873432343378178544, -1.599625672291271394 ) ) ;
#113887=CARTESIAN_POINT ( 'NONE',  ( -4.370663978927099791, 5.060324124126027279, 7.500000000000000000 ) ) ;
#113890=CARTESIAN_POINT ( 'NONE',  ( -6.555587544261016753, 6.796970737185429989, -0.4399619850315484859 ) ) ;
#113907=CARTESIAN_POINT ( 'NONE',  ( 6.590672070018850803, 7.822110515511036866, -1.082531754730548412 ) ) ;
#113922=CARTESIAN_POINT ( 'NONE',  ( -4.990809943606281607, 6.915973915664348937, -1.443375672974066548 ) ) ;
#113924=CARTESIAN_POINT ( 'NONE',  ( 5.037736595929563244, 8.035053907629919223, -1.199719254218452047 ) ) ;
#113965=DIRECTION ( 'NONE',  ( -0.6507913734559640506, -0.7592566023653003482, 0.000000000000000000 ) ) ;
#113966=CARTESIAN_POINT ( 'NONE',  ( 4.095971805104288599, 5.871996087412059140, 1.443375672974058777 ) ) ;
#113974=CARTESIAN_POINT ( 'NONE',  ( -4.163738354385607465, 7.871795561280641174, 0.001129208541240749085 ) ) ;
#113977=CARTESIAN_POINT ( 'NONE',  ( -5.655159470231558849, 6.730679149092498648, 1.082531754730549078 ) ) ;
#113982=ORIENTED_EDGE ( 'NONE', *, *, #152126, .F. ) ;
#113983=CARTESIAN_POINT ( 'NONE',  ( -4.936050443827081580, 7.916420063510339666, 1.199719254218452935 ) ) ;
#113988=EDGE_LOOP ( 'NONE', ( #143624, #30677 ) ) ;
#113989=ORIENTED_EDGE ( 'NONE', *, *, #45431, .F. ) ;
#113990=VERTEX_POINT ( 'NONE', #149792 ) ;
#113993=CARTESIAN_POINT ( 'NONE',  ( -6.168033539574333979, 6.160736982450306876, 0.7998128361456281477 ) ) ;
#113996=CARTESIAN_POINT ( 'NONE',  ( 5.997720278586790243, 7.186234674792547850, 1.197368251494409286 ) ) ;
#113999=CARTESIAN_POINT ( 'NONE',  ( 2.975845599428874610, 6.509329181731200009, 0.4525212045368381952 ) ) ;
#114001=CARTESIAN_POINT ( 'NONE',  ( 7.028976294042106332, 7.165170195996068969, 0.000000000000000000 ) ) ;
#114010=CARTESIAN_POINT ( 'NONE',  ( -5.815521545619021460, 5.749472989502435460, -0.7998128361456362523 ) ) ;
#114014=CARTESIAN_POINT ( 'NONE',  ( -7.449279056065764237, 7.655523418356991350, 0.7998128361456341429 ) ) ;
#114018=CARTESIAN_POINT ( 'NONE',  ( 6.658462837642799670, 7.901199744405670522, 1.082531754730549967 ) ) ;
#114020=CARTESIAN_POINT ( 'NONE',  ( -5.926322542504860458, 9.928143709648733051, -0.7216878364870338292 ) ) ;
#114027=CARTESIAN_POINT ( 'NONE',  ( 6.391743074199808916, 6.421731439513382433, -0.7998128361456481317 ) ) ;
#114031=CARTESIAN_POINT ( 'NONE',  ( -4.936355671280336921, 4.883780760425392664, 0.5269810592589857512 ) ) ;
#114058=CARTESIAN_POINT ( 'NONE',  ( 4.664027441776592120, 8.287593892024585074, -0.5126927951675692707 ) ) ;
#114067=CARTESIAN_POINT ( 'NONE',  ( 7.614839552730775729, 8.913009562054615031, 1.199719254218452047 ) ) ;
#114072=CARTESIAN_POINT ( 'NONE',  ( -5.056216892478136771, 7.878110338051091510, -1.109312559570382550 ) ) ;
#114080=CARTESIAN_POINT ( 'NONE',  ( -5.628043163004235794, 5.738674243025936761, 0.7216878364870257245 ) ) ;
#114091=CARTESIAN_POINT ( 'NONE',  ( -5.029148636026397945, 4.832037928311032182, 0.7998128361456281477 ) ) ;
#114093=CARTESIAN_POINT ( 'NONE',  ( 5.826972158823246595, 10.02016096192762085, -0.7998128361456481317 ) ) ;
#114096=ORIENTED_EDGE ( 'NONE', *, *, #23441, .F. ) ;
#114102=CARTESIAN_POINT ( 'NONE',  ( 4.854701522145073334, 7.821512988214679218, -1.199719254218450271 ) ) ;
#114105=CARTESIAN_POINT ( 'NONE',  ( 7.471952054462756010, 7.889901283060952508, 0.7216878364870267237 ) ) ;
#114119=CARTESIAN_POINT ( 'NONE',  ( -6.134138155540168391, 6.121192367743780949, 0.000000000000000000 ) ) ;
#114120=CARTESIAN_POINT ( 'NONE',  ( 4.228163802615382494, 6.026220084508304708, -1.599625672291269396 ) ) ;
#114130=CARTESIAN_POINT ( 'NONE',  ( -7.045397100956844127, 8.248660034984974132, -1.199719254218452047 ) ) ;
#114131=CARTESIAN_POINT ( 'NONE',  ( 7.015418140428412386, 7.149352350113456822, 0.7998128361456331437 ) ) ;
#114133=CARTESIAN_POINT ( 'NONE',  ( -4.613268803136618246, 8.378775596900176481, 0.2107346534404584415 ) ) ;
#114137=CARTESIAN_POINT ( 'NONE',  ( 3.528865121306874464, 7.339036084825155015, -0.7998128361456362523 ) ) ;
#114144=CARTESIAN_POINT ( 'NONE',  ( -5.873358954868365345, 7.276917811852929852, 1.275545277584020365 ) ) ;
#114153=CARTESIAN_POINT ( 'NONE',  ( -4.136646265500970365, 5.919449624541475607, -1.443375672974066548 ) ) ;
#114168=VERTEX_POINT ( 'NONE', #189738 ) ;
#114191=EDGE_LOOP ( 'NONE', ( #126780, #211041, #135081, #111501 ) ) ;
#114198=EDGE_CURVE ( 'NONE', #65494, #189704, #63500, .T. ) ;
#114201=CARTESIAN_POINT ( 'NONE',  ( 3.390420931869152721, 6.113185632892752075, -1.199719254218452047 ) ) ;
#114202=CARTESIAN_POINT ( 'NONE',  ( -3.851925040058345573, 5.587274861525073355, -1.443375672974078761 ) ) ;
#114230=CARTESIAN_POINT ( 'NONE',  ( -4.956387674247580755, 7.940146832334256111, 1.199719254218452935 ) ) ;
#114232=CARTESIAN_POINT ( 'NONE',  ( 5.302647476276220573, 8.240153584747313076, -1.082531754730548412 ) ) ;
#114237=CARTESIAN_POINT ( 'NONE',  ( -7.279802135894939852, 7.457800344824362604, -0.7998128361456362523 ) ) ;
#114246=CARTESIAN_POINT ( 'NONE',  ( -6.784929528996132220, 6.880448970109080520, 0.000000000000000000 ) ) ;
#114259=CARTESIAN_POINT ( 'NONE',  ( -6.069210040772897052, 7.109775131437022999, -1.199719254218453823 ) ) ;
#114262=CARTESIAN_POINT ( 'NONE',  ( -5.966997003790217136, 9.975597247814986801, -0.7216878364870338292 ) ) ;
#114265=CARTESIAN_POINT ( 'NONE',  ( -5.261973015435229328, 9.153069261400824885, 0.000000000000000000 ) ) ;
#114266=CARTESIAN_POINT ( 'NONE',  ( 7.713663051532233972, 7.963971413067895355, -0.7998128361456341429 ) ) ;
#114267=CARTESIAN_POINT ( 'NONE',  ( -6.688968683495758683, 8.897159112202094988, -1.599625672291271394 ) ) ;
#114274=ORIENTED_EDGE ( 'NONE', *, *, #134227, .T. ) ;
#114286=CARTESIAN_POINT ( 'NONE',  ( -1.835699054053199664, 2.512084418327853008, -2.498041437723068636 ) ) ;
#114302=TOROIDAL_SURFACE ( 'NONE', #86545, 0.8300000000000010703, 0.08000000000000000167 ) ;
#114304=CARTESIAN_POINT ( 'NONE',  ( 6.176125489850557315, 6.957122458884915872, -0.8945188991977878201 ) ) ;
#114317=CARTESIAN_POINT ( 'NONE',  ( 7.147083253059300922, 8.367293879104554577, 1.199719254218452935 ) ) ;
#114320=CARTESIAN_POINT ( 'NONE',  ( -3.955946960137363799, 7.837298230127379917, 0.7998128361456352531 ) ) ;
#114335=CARTESIAN_POINT ( 'NONE',  ( 4.980641328173811999, 6.904110530993182948, 1.599625672291269396 ) ) ;
#114337=CARTESIAN_POINT ( 'NONE',  ( 7.679767667498067496, 7.924426798361372093, 0.000000000000000000 ) ) ;
#114341=CARTESIAN_POINT ( 'NONE',  ( -4.733481511527885210, 4.890303307122107590, -0.5491554243041256722 ) ) ;
#114343=CARTESIAN_POINT ( 'NONE',  ( -6.170369307550858551, 8.292126506933035657, 1.443375672974058777 ) ) ;
#114350=CARTESIAN_POINT ( 'NONE',  ( 5.515134625708930649, 9.656350506627580543, 0.000000000000000000 ) ) ;
#114364=CARTESIAN_POINT ( 'NONE',  ( -4.963693636378939011, 8.805076652501815815, 0.7216878364870267237 ) ) ;
#114365=CARTESIAN_POINT ( 'NONE',  ( 6.048345925472191631, 6.229027465905275562, 0.7216878364870328300 ) ) ;
#114373=ORIENTED_EDGE ( 'NONE', *, *, #392, .F. ) ;
#114375=CARTESIAN_POINT ( 'NONE',  ( -7.119440060951841787, 7.478637290631501067, 0.000000000000000000 ) ) ;
#114376=CARTESIAN_POINT ( 'NONE',  ( 8.188198428010544205, 8.517596018959260107, 0.000000000000000000 ) ) ;
#114380=CARTESIAN_POINT ( 'NONE',  ( 5.736508391913541338, 6.825586224388162648, -1.082531754730548412 ) ) ;
#114385=DIRECTION ( 'NONE',  ( 0.6507913734559641616, -0.7592566023653004592, 0.000000000000000000 ) ) ;
#114397=CARTESIAN_POINT ( 'NONE',  ( -4.492547798081878874, 6.334668079219206049, 1.599625672291263179 ) ) ;
#114408=CARTESIAN_POINT ( 'NONE',  ( 3.542423274920540432, 7.354853930707762721, -1.734723475976807094E-15 ) ) ;
#114410=CARTESIAN_POINT ( 'NONE',  ( -6.282224075085783177, 8.422623735723785643, 1.599625672291269396 ) ) ;
#114411=CARTESIAN_POINT ( 'NONE',  ( 5.342795052237045539, 8.390955439988655229, -1.199719254218450271 ) ) ;
#114419=CARTESIAN_POINT ( 'NONE',  ( -6.394605727500880299, 7.489403432619674561, -1.199719254218452047 ) ) ;
#114447=CIRCLE ( 'NONE', #111050, 0.8299999999999999600 ) ;
#114448=CARTESIAN_POINT ( 'NONE',  ( 4.746763178560254204, 6.631252689777363152, 1.443375672974065660 ) ) ;
#114454=CARTESIAN_POINT ( 'NONE',  ( 3.865483193227626124, 7.523831135491951372, -0.7216878364870338292 ) ) ;
#114466=CARTESIAN_POINT ( 'NONE',  ( -5.094831863685302942, 9.165997284266655498, 0.7998128361456291469 ) ) ;
#114468=CARTESIAN_POINT ( 'NONE',  ( -7.449279056065764237, 7.655523418356991350, 0.7998128361456341429 ) ) ;
#114477=CARTESIAN_POINT ( 'NONE',  ( 6.688968683495743583, 8.897159112202094988, -1.599625672291283607 ) ) ;
#114482=CARTESIAN_POINT ( 'NONE',  ( 4.960800185296459830, 8.075801985472857325, -1.085925974634168290 ) ) ;
#114483=CARTESIAN_POINT ( 'NONE',  ( -6.668631453075260396, 8.873432343378178544, -1.599625672291271394 ) ) ;
#114489=CARTESIAN_POINT ( 'NONE',  ( -4.828112100242279325, 8.646898193675708555, -0.7216878364870338292 ) ) ;
#114493=CARTESIAN_POINT ( 'NONE',  ( -5.936491157937300756, 8.019268665717216749, 1.599625672291263179 ) ) ;
#114512=DIRECTION ( 'NONE',  ( 0.7592566023653016805, -0.6507913734559627184, 0.000000000000000000 ) ) ;
#114515=CARTESIAN_POINT ( 'NONE',  ( -3.594320120954326292, 6.247105003538398371, 1.082531754730549967 ) ) ;
#114517=CARTESIAN_POINT ( 'NONE',  ( 3.400062661977048428, 7.188766548940353829, -1.734723475976807094E-15 ) ) ;
#114518=CARTESIAN_POINT ( 'NONE',  ( -6.414942957921379474, 7.513130201443591005, -1.199719254218452047 ) ) ;
#114526=CARTESIAN_POINT ( 'NONE',  ( 5.900277318768097246, 7.249539301847896411, -1.301905728482563251 ) ) ;
#114528=ORIENTED_EDGE ( 'NONE', *, *, #10408, .F. ) ;
#114542=CARTESIAN_POINT ( 'NONE',  ( -6.851666526859749418, 9.086973262793417661, -1.599625672291271394 ) ) ;
#114568=CARTESIAN_POINT ( 'NONE',  ( 3.400062661977048428, 7.188766548940353829, -1.734723475976807094E-15 ) ) ;
#114584=CARTESIAN_POINT ( 'NONE',  ( 6.780486220610169035, 9.003929572168926754, -1.443375672974078761 ) ) ;
#114591=CARTESIAN_POINT ( 'NONE',  ( -4.288121723672178476, 8.224835454251337552, -0.7998128361456362523 ) ) ;
#114596=CARTESIAN_POINT ( 'NONE',  ( -5.587368702163209910, 9.532697562583475559, 0.000000000000000000 ) ) ;
#114600=CARTESIAN_POINT ( 'NONE',  ( -4.001049302594738677, 7.679299581788098017, 0.07148048886325740481 ) ) ;
#114605=CARTESIAN_POINT ( 'NONE',  ( -5.255720823952942489, 6.160704378480398979, -1.199719254218453823 ) ) ;
#114615=CARTESIAN_POINT ( 'NONE',  ( 3.725458348705031231, 7.568394850123006279, -1.734723475976807094E-15 ) ) ;
#114635=ORIENTED_EDGE ( 'NONE', *, *, #167055, .F. ) ;
#114637=CARTESIAN_POINT ( 'NONE',  ( -7.761116589180078407, 8.019333873657032541, 0.000000000000000000 ) ) ;
#114647=CARTESIAN_POINT ( 'NONE',  ( 3.881377115262159894, 7.750300077773022878, 0.7998128361456271485 ) ) ;
#114654=CARTESIAN_POINT ( 'NONE',  ( 3.879041347285658414, 6.579279767591636130, -1.082531754730548412 ) ) ;
#114657=CARTESIAN_POINT ( 'NONE',  ( 6.455090533882185788, 8.624301270986276080, -1.443375672974078761 ) ) ;
#114668=CARTESIAN_POINT ( 'NONE',  ( -5.804299160426229953, 8.825413882922319431, -1.082531754730549967 ) ) ;
#114701=CARTESIAN_POINT ( 'NONE',  ( 4.667750024854814050, 8.667735138964429709, -0.7998128361456381397 ) ) ;
#114703=CARTESIAN_POINT ( 'NONE',  ( 4.213551878797002992, 8.137837301896977849, 0.000000000000000000 ) ) ;
#114716=CARTESIAN_POINT ( 'NONE',  ( -3.311934663488232733, 7.085950550703385531, -0.7998128361456481317 ) ) ;
#114719=CARTESIAN_POINT ( 'NONE',  ( 6.021229617800532452, 6.197391773621639288, 0.000000000000000000 ) ) ;
#114730=CARTESIAN_POINT ( 'NONE',  ( -6.536439455564198475, 8.719208346281938304, 1.443375672974064550 ) ) ;
#114732=CARTESIAN_POINT ( 'NONE',  ( -4.014622883422322985, 7.697827440719083647, -0.7216878364870458196 ) ) ;
#114760=CARTESIAN_POINT ( 'NONE',  ( -3.546339698426324460, 6.295090860542775779, -1.199719254218450271 ) ) ;
#114761=EDGE_CURVE ( 'NONE', #196200, #50747, #75748, .T. ) ;
#114769=CARTESIAN_POINT ( 'NONE',  ( -8.072954122294394352, 8.383144328957069291, -0.7998128361456362523 ) ) ;
#114770=CARTESIAN_POINT ( 'NONE',  ( -5.543378919943204863, 7.538303290789565736, -1.349654061105177050 ) ) ;
#114788=CARTESIAN_POINT ( 'NONE',  ( 6.496291879603339758, 7.608037276739255006, 1.199719254218452935 ) ) ;
#114794=CARTESIAN_POINT ( 'NONE',  ( 0.3999999999999758193, 3.000000000029069636, -2.023857702507768419 ) ) ;
#114811=CARTESIAN_POINT ( 'NONE',  ( 7.354371980770088690, 7.544798497178720531, 0.000000000000000000 ) ) ;
#114812=CARTESIAN_POINT ( 'NONE',  ( 5.845500506147374153, 6.848780674373954547, 1.199719254218453823 ) ) ;
#114814=CARTESIAN_POINT ( 'NONE',  ( 5.578253857379852576, 5.472660686556754861, -0.7998128361456481317 ) ) ;
#114825=CARTESIAN_POINT ( 'NONE',  ( 5.559975706299111309, 7.414571502401146930, -1.245397951563255834 ) ) ;
#114826=CARTESIAN_POINT ( 'NONE',  ( -6.305950843687521790, 7.489935751457798219, 1.082531754730548412 ) ) ;
#114827=CARTESIAN_POINT ( 'NONE',  ( 4.502716413514295191, 6.346531463890372926, -1.443375672974068769 ) ) ;
#114852=CARTESIAN_POINT ( 'NONE',  ( 4.179656494762836516, 8.098292687190454586, -0.7998128361456362523 ) ) ;
#114854=CARTESIAN_POINT ( 'NONE',  ( 2.925527285498711549, 6.635141943048991742, 0.7998128361456281477 ) ) ;
#114872=CARTESIAN_POINT ( 'NONE',  ( -7.795011973214244883, 8.058878488363559356, 0.7998128361456341429 ) ) ;
#114884=CARTESIAN_POINT ( 'NONE',  ( 4.694866332082116678, 8.699370830729650450, 0.7998128361456341429 ) ) ;
#114888=CARTESIAN_POINT ( 'NONE',  ( -6.470902446588409518, 6.777469385738574381, 0.2989120342885512871 ) ) ;
#114889=CARTESIAN_POINT ( 'NONE',  ( 7.035755370848908896, 7.173079118937375931, 0.7998128361456352531 ) ) ;
#114902=CARTESIAN_POINT ( 'NONE',  ( 4.759808938472720463, 8.174556087920027636, -0.7576060450402433144 ) ) ;
#114911=CARTESIAN_POINT ( 'NONE',  ( 3.231779075379137556, 6.036511184309971689, -2.420000000000002149 ) ) ;
#114923=CARTESIAN_POINT ( 'NONE',  ( -7.119966945832006289, 8.335658187339330283, 1.199719254218452047 ) ) ;
#114925=CARTESIAN_POINT ( 'NONE',  ( 6.333594036239346359, 7.418223126147930557, 1.199719254218453823 ) ) ;
#114933=CARTESIAN_POINT ( 'NONE',  ( 2.300394833791450377, 2.756885564284757617, -2.500000000000000444 ) ) ;
#114936=CARTESIAN_POINT ( 'NONE',  ( -0.1010051578917390280, 3.387064998577566488, -1.997555336163420181 ) ) ;
#114952=CARTESIAN_POINT ( 'NONE',  ( 5.072158865288233898, 7.971250205261355859, 1.082531754730549078 ) ) ;
#114957=ORIENTED_EDGE ( 'NONE', *, *, #130852, .F. ) ;
#114967=CARTESIAN_POINT ( 'NONE',  ( -5.153507786970276783, 6.145418851954329575, -1.082531754730549967 ) ) ;
#114969=CARTESIAN_POINT ( 'NONE',  ( 5.200434439293556643, 8.224868058221247225, -1.199719254218452047 ) ) ;
#114974=CARTESIAN_POINT ( 'NONE',  ( -2.993318053567081360, 6.714231172462041819, 0.000000000000000000 ) ) ;
#114986=CARTESIAN_POINT ( 'NONE',  ( -2.796816994357229635, 2.968434822912338067, 2.452793345967703598 ) ) ;
#114988=CARTESIAN_POINT ( 'NONE',  ( -6.102578539482539810, 6.292298848917299736, 0.000000000000000000 ) ) ;
#115003=ORIENTED_EDGE ( 'NONE', *, *, #23766, .F. ) ;
#115013=DIRECTION ( 'NONE',  ( -0.7771862570881746812, 0.6292706268317899143, 0.000000000000000000 ) ) ;
#115023=CARTESIAN_POINT ( 'NONE',  ( 3.553118775233146120, 6.302999783484076524, -1.199719254218453823 ) ) ;
#115029=CARTESIAN_POINT ( 'NONE',  ( -6.116136693096208887, 6.308116694799912771, 0.7216878364870257245 ) ) ;
#115030=FACE_BOUND ( 'NONE', #84987, .T. ) ;
#115035=CARTESIAN_POINT ( 'NONE',  ( -6.774234028683526532, 7.932303117332766718, 1.199719254218452047 ) ) ;
#115042=ORIENTED_EDGE ( 'NONE', *, *, #31289, .F. ) ;
#115045=CARTESIAN_POINT ( 'NONE',  ( -6.038177310039794854, 8.137902509836795417, -1.599625672291271394 ) ) ;
#115047=CARTESIAN_POINT ( 'NONE',  ( 5.853046489161108035, 7.294594176516559614, 1.271900669079442325 ) ) ;
#115052=CARTESIAN_POINT ( 'NONE',  ( 7.517069824134078537, 7.734612647770044092, 0.000000000000000000 ) ) ;
#115058=VERTEX_POINT ( 'NONE', #91239 ) ;
#115060=CARTESIAN_POINT ( 'NONE',  ( -4.950662367645459305, 5.804802846121667415, -1.199719254218453823 ) ) ;
#115066=CARTESIAN_POINT ( 'NONE',  ( -5.424143973919053785, 8.485862515284315677, 1.199719254218454489 ) ) ;
#115070=CARTESIAN_POINT ( 'NONE',  ( 6.251718229232841928, 8.387033582228703210, -1.443375672974078761 ) ) ;
#115072=CARTESIAN_POINT ( 'NONE',  ( -5.424670858799220063, 9.342883411992149334, 0.000000000000000000 ) ) ;
#115078=CARTESIAN_POINT ( 'NONE',  ( 6.215487077222150880, 6.216099443039444949, 0.000000000000000000 ) ) ;
#115121=CARTESIAN_POINT ( 'NONE',  ( -6.114219544286552122, 7.015314154546907766, -0.9703045268592332961 ) ) ;
#115139=CARTESIAN_POINT ( 'NONE',  ( -8.072954122294394352, 8.383144328957069291, -0.7998128361456362523 ) ) ;
#115153=CARTESIAN_POINT ( 'NONE',  ( 6.229045230835819069, 6.231917288922055320, -0.7998128361456481317 ) ) ;
#115156=CARTESIAN_POINT ( 'NONE',  ( 5.926322542504858681, 8.007405281046052536, -1.443375672974078761 ) ) ;
#115159=EDGE_CURVE ( 'NONE', #85209, #184855, #76316, .T. ) ;
#115170=CARTESIAN_POINT ( 'NONE',  ( -6.784929528996132220, 6.880448970109080520, 0.000000000000000000 ) ) ;
#115171=CARTESIAN_POINT ( 'NONE',  ( 5.564695703766185275, 5.456842840674144490, 0.000000000000000000 ) ) ;
#115179=ORIENTED_EDGE ( 'NONE', *, *, #160804, .T. ) ;
#115181=CARTESIAN_POINT ( 'NONE',  ( -5.725286006720766707, 9.901527117808042178, 0.7998128361456291469 ) ) ;
#115182=CARTESIAN_POINT ( 'NONE',  ( 5.397027666691686321, 8.454226823519094935, 1.199719254218451159 ) ) ;
#115184=CARTESIAN_POINT ( 'NONE',  ( -4.596923820214036560, 8.483565078729160547, 0.2266403168418751335 ) ) ;
#115188=CARTESIAN_POINT ( 'NONE',  ( 5.727393547130178675, 5.646656991265468939, 0.000000000000000000 ) ) ;
#115192=CARTESIAN_POINT ( 'NONE',  ( -0.2713731142545342534, 2.604673336870401812, 1.982545097633750197 ) ) ;
#115196=CARTESIAN_POINT ( 'NONE',  ( -6.081163491871431681, 7.123212080692602477, 1.153528356629534013 ) ) ;
#115204=CARTESIAN_POINT ( 'NONE',  ( -3.133342898089680695, 6.669667457830990465, 0.7216878364870338292 ) ) ;
#115216=CYLINDRICAL_SURFACE ( 'NONE', #1313, 0.08000000000000041800 ) ;
#115218=CARTESIAN_POINT ( 'NONE',  ( -7.015401035077363900, 6.062865449010540253, 2.437084766375293476 ) ) ;
#115236=VECTOR ( 'NONE', #12272, 1000.000000000000227 ) ;
#115254=CARTESIAN_POINT ( 'NONE',  ( 5.225741863424510747, 5.061396693608882558, 0.7998128361456352531 ) ) ;
#115275=( BOUNDED_SURFACE ( )  B_SPLINE_SURFACE ( 1, 2, ( 
 ( #23805, #73633, #124611, #190569, #139732, #203605, #205756, #56324, #121405, #187377, #57386, #41160, #107269, #173289, #8625, #140810, #54884, #152383, #137220, #83095, #3961, #51693, #136144, #19163, #149174, #203240, #198963, #20226, #17019, #18085, #70029, #185925, #85237, #36486, #167563, #135085, #121038, #50607, #202162, #116732, #187005, #102563, #182731, #134034, #132960, #100423, #53820, #201099, #52739, #184859, #168623, #34350, #751, #119950, #86311, #101493, #66817, #37561, #151325, #103641, #166494, #35415, #169693, #5027, #21281, #118873, #1830, #87387, #67889, #84173, #150262, #2893, #200042, #117815, #183805, #153454, #68966, #38636, #71102, #104715, #139353, #106894, #189150, #206457, #207528, #124246, #171835, #88464, #55953, #22352, #204297, #57022, #155590, #123189, #73246, #72174, #90607, #191263, #26645, #122106, #190204, #175058, #92746, #188071, #172920, #23428, #154524, #138282, #6104, #24496, #39700, #7175, #105809, #140446, #158790, #41864, #10387, #126372, #107973, #208578, #75407, #40789, #109039, #156666, #76462, #9334, #142571, #174002, #205383, #58084, #25573, #8258, #91684, #74342, #89539, #157737, #141520, #59147, #125305, #60211, #42929, #192331, #43990, #170763, #46940, #197420, #45873, #164929, #130384, #81547, #62108, #14394, #115182, #198476, #82604, #114131, #195309, #49062, #113058, #79417, #29611, #146585, #210470, #161751, #95696, #258, #13342, #99936, #98876, #50121, #179064, #212602, #80485, #31748, #32802, #163886, #211532, #128267, #145534, #194229, #63167, #96766, #30683, #162817, #64240, #111995, #129333, #196374, #83666, #48014, #180123, #15461, #97821, #147630, #148689, #116242, #177997, #213648, #65274, #131420, #181177, #16521, #66329, #132474, #182231, #33855, #165998, #17583, #19734, #87949, #149757, #3467, #85813, #150832, #18664, #21841, #187572, #102067, #52249, #201666, #170256, #104209, #35986, #118376, #51185, #2394, #151892, #22921, #200602, #69536, #103136, #135643, #53313, #154023, #137783, #1334, #185433, #4524, #67395, #119445, #54389 ),
 ( #136713, #133536, #117308, #37053, #169194, #199543, #121600, #186506, #183304, #5590, #34911, #100983, #167072, #84744, #20787, #71669, #203802, #68473, #86882, #55448, #39197, #134601, #152949, #184364, #168132, #70599, #202738, #120527, #38137, #105289, #171325, #58653, #10945, #108535, #77019, #44554, #42430, #126941, #208085, #107471, #27206, #173497, #143148, #142071, #209143, #174565, #73834, #190766, #26141, #25073, #92254, #189708, #138851, #122683, #74906, #158300, #155091, #159348, #91175, #191831, #205957, #157234, #6677, #123747, #109614, #204868, #8829, #110670, #89036, #57590, #125872, #192898, #141014, #41361, #188646, #176670, #72754, #56523, #60782, #207022, #93313, #124807, #40277, #106387, #9891, #172410, #23998, #75968, #59712, #43494, #90101, #156166, #7747, #175619, #139930, #78094, #61851, #16266, #148441, #111737, #147379, #94377, #128018, #146328, #13082, #15211, #79162, #177743, #193972, #178817, #28282, #45620, #29358, #32545, #95452, #132216, #131182, #82350, #211284, #30430, #46686, #63984, #65027, #196126, #161502, #160417, #145278, #12022, #62907, #129077, #195048, #112804, #96516, #144221, #162565, #14137, #115988, #80230, #212343, #47764, #130137, #113878, #114925, #9, #210215, #179873, #97573, #31498, #163630, #213406, #81302, #98620, #197172, #48808, #180924, #164681, #66074, #198225, #49861, #35729, #51998, #183051, #50929, #54128, #5329, #134344, #84485, #19472, #202475, #136457, #68214, #87685, #118124, #117054, #70340, #55193, #100736, #186239, #150575, #184109, #21580, #120265, #71410, #102877, #153759, #33607, #168935, #2137, #86620, #101805, #99677, #137522, #149496, #185168, #181976, #34666, #20538, #37874, #167874, #201410, #85549, #151639, #203539, #1079, #152688, #67144, #165747, #53049, #133278, #200349, #83414, #166815, #4270, #3206, #69275, #135389, #119182, #199286, #17333, #103951, #18409, #169993, #36792, #75703, #41093, #206758, #187314, #139666, #25871, #109346, #207820, #154828, #57323, #121339, #72485, #6413, #125605, #138586, #10683, #9626, #175356 ) ),
 .UNSPECIFIED., .F., .F., .T. ) 
 B_SPLINE_SURFACE_WITH_KNOTS ( ( 2, 2 ),
 ( 3, 2, 2, 2, 2, 2, 2, 2, 2, 2, 2, 2, 2, 2, 2, 2, 2, 2, 2, 2, 2, 2, 2, 2, 2, 2, 2, 2, 2, 2, 2, 2, 2, 2, 2, 2, 2, 2, 2, 2, 2, 2, 2, 2, 2, 2, 2, 2, 2, 2, 2, 2, 2, 2, 2, 2, 2, 2, 2, 2, 2, 2, 2, 2, 2, 2, 2, 2, 2, 2, 2, 2, 2, 2, 2, 2, 2, 2, 2, 2, 2, 2, 2, 2, 2, 2, 2, 2, 2, 2, 2, 2, 2, 2, 2, 2, 2, 2, 2, 2, 2, 2, 2, 2, 2, 2, 2, 2, 2, 2, 2, 2, 2, 2, 2, 2, 2, 2, 2, 2, 3 ),
 ( 0.000000000000000000, 1.000000000000000000 ),
 ( 0.000000000000000000, 0.008333333333333333218, 0.01666666666666666644, 0.02500000000000000139, 0.03333333333333333287, 0.04166666666666666435, 0.05000000000000000278, 0.05833333333333333426, 0.06666666666666666574, 0.07499999999999999722, 0.08333333333333332871, 0.09166666666666666019, 0.1000000000000000056, 0.1083333333333333370, 0.1166666666666666685, 0.1250000000000000000, 0.1333333333333333315, 0.1416666666666666630, 0.1499999999999999944, 0.1583333333333333259, 0.1666666666666666574, 0.1749999999999999889, 0.1833333333333333204, 0.1916666666666666796, 0.2000000000000000111, 0.2083333333333333426, 0.2166666666666666741, 0.2250000000000000056, 0.2333333333333333370, 0.2416666666666666685, 0.2500000000000000000, 0.2583333333333333592, 0.2666666666666666630, 0.2750000000000000222, 0.2833333333333333259, 0.2916666666666666852, 0.2999999999999999889, 0.3083333333333333481, 0.3166666666666666519, 0.3250000000000000111, 0.3333333333333333148, 0.3416666666666666741, 0.3499999999999999778, 0.3583333333333333370, 0.3666666666666666408, 0.3750000000000000000, 0.3833333333333333592, 0.3916666666666666630, 0.4000000000000000222, 0.4083333333333333259, 0.4166666666666666852, 0.4249999999999999889, 0.4333333333333333481, 0.4416666666666666519, 0.4500000000000000111, 0.4583333333333333148, 0.4666666666666666741, 0.4749999999999999778, 0.4833333333333333370, 0.4916666666666666408, 0.5000000000000000000, 0.5083333333333333037, 0.5166666666666667185, 0.5250000000000000222, 0.5333333333333333259, 0.5416666666666666297, 0.5500000000000000444, 0.5583333333333333481, 0.5666666666666666519, 0.5749999999999999556, 0.5833333333333333703, 0.5916666666666666741, 0.5999999999999999778, 0.6083333333333332815, 0.6166666666666666963, 0.6250000000000000000, 0.6333333333333333037, 0.6416666666666667185, 0.6500000000000000222, 0.6583333333333333259, 0.6666666666666666297, 0.6750000000000000444, 0.6833333333333333481, 0.6916666666666666519, 0.6999999999999999556, 0.7083333333333333703, 0.7166666666666666741, 0.7249999999999999778, 0.7333333333333332815, 0.7416666666666666963, 0.7500000000000000000, 0.7583333333333333037, 0.7666666666666667185, 0.7750000000000000222, 0.7833333333333333259, 0.7916666666666666297, 0.8000000000000000444, 0.8083333333333333481, 0.8166666666666666519, 0.8249999999999999556, 0.8333333333333333703, 0.8416666666666666741, 0.8499999999999999778, 0.8583333333333332815, 0.8666666666666666963, 0.8750000000000000000, 0.8833333333333333037, 0.8916666666666667185, 0.9000000000000000222, 0.9083333333333333259, 0.9166666666666666297, 0.9250000000000000444, 0.9333333333333333481, 0.9416666666666666519, 0.9499999999999999556, 0.9583333333333333703, 0.9666666666666666741, 0.9749999999999999778, 0.9833333333333332815, 0.9916666666666666963, 1.000000000000000000 ),
 .UNSPECIFIED. ) 
 GEOMETRIC_REPRESENTATION_ITEM ( )  RATIONAL_B_SPLINE_SURFACE ( (
 ( 1.000000000000000000, 0.8660254037844387076, 1.000000000000000000, 0.8660254037844387076, 1.000000000000000000, 0.8660254037844387076, 1.000000000000000000, 0.8660254037844387076, 1.000000000000000000, 0.8660254037844387076, 1.000000000000000000, 0.8660254037844387076, 1.000000000000000000, 0.8660254037844387076, 1.000000000000000000, 0.8660254037844387076, 1.000000000000000000, 0.8660254037844387076, 1.000000000000000000, 0.8660254037844387076, 1.000000000000000000, 0.8660254037844387076, 1.000000000000000000, 0.8660254037844387076, 1.000000000000000000, 0.8660254037844387076, 1.000000000000000000, 0.8660254037844387076, 1.000000000000000000, 0.8660254037844387076, 1.000000000000000000, 0.8660254037844387076, 1.000000000000000000, 0.8660254037844387076, 1.000000000000000000, 0.8660254037844387076, 1.000000000000000000, 0.8660254037844387076, 1.000000000000000000, 0.8660254037844387076, 1.000000000000000000, 0.8660254037844387076, 1.000000000000000000, 0.8660254037844387076, 1.000000000000000000, 0.8660254037844387076, 1.000000000000000000, 0.8660254037844387076, 1.000000000000000000, 0.8660254037844387076, 1.000000000000000000, 0.8660254037844387076, 1.000000000000000000, 0.8660254037844387076, 1.000000000000000000, 0.8660254037844387076, 1.000000000000000000, 0.8660254037844387076, 1.000000000000000000, 0.8660254037844387076, 1.000000000000000000, 0.8660254037844387076, 1.000000000000000000, 0.8660254037844387076, 1.000000000000000000, 0.8660254037844387076, 1.000000000000000000, 0.8660254037844387076, 1.000000000000000000, 0.8660254037844387076, 1.000000000000000000, 0.8660254037844387076, 1.000000000000000000, 0.8660254037844387076, 1.000000000000000000, 0.8660254037844387076, 1.000000000000000000, 0.8660254037844387076, 1.000000000000000000, 0.8660254037844387076, 1.000000000000000000, 0.8660254037844387076, 1.000000000000000000, 0.8660254037844387076, 1.000000000000000000, 0.8660254037844387076, 1.000000000000000000, 0.8660254037844387076, 1.000000000000000000, 0.8660254037844387076, 1.000000000000000000, 0.8660254037844387076, 1.000000000000000000, 0.8660254037844387076, 1.000000000000000000, 0.8660254037844387076, 1.000000000000000000, 0.8660254037844387076, 1.000000000000000000, 0.8660254037844387076, 1.000000000000000000, 0.8660254037844387076, 1.000000000000000000, 0.8660254037844387076, 1.000000000000000000, 0.8660254037844387076, 1.000000000000000000, 0.8660254037844387076, 1.000000000000000000, 0.8660254037844387076, 1.000000000000000000, 0.8660254037844387076, 1.000000000000000000, 0.8660254037844387076, 1.000000000000000000, 0.8660254037844387076, 1.000000000000000000, 0.8660254037844387076, 1.000000000000000000, 0.8660254037844387076, 1.000000000000000000, 0.8660254037844387076, 1.000000000000000000, 0.8660254037844387076, 1.000000000000000000, 0.8660254037844387076, 1.000000000000000000, 0.8660254037844387076, 1.000000000000000000, 0.8660254037844387076, 1.000000000000000000, 0.8660254037844387076, 1.000000000000000000, 0.8660254037844387076, 1.000000000000000000, 0.8660254037844387076, 1.000000000000000000, 0.8660254037844387076, 1.000000000000000000, 0.8660254037844387076, 1.000000000000000000, 0.8660254037844387076, 1.000000000000000000, 0.8660254037844387076, 1.000000000000000000, 0.8660254037844387076, 1.000000000000000000, 0.8660254037844387076, 1.000000000000000000, 0.8660254037844387076, 1.000000000000000000, 0.8660254037844387076, 1.000000000000000000, 0.8660254037844387076, 1.000000000000000000, 0.8660254037844387076, 1.000000000000000000, 0.8660254037844387076, 1.000000000000000000, 0.8660254037844387076, 1.000000000000000000, 0.8660254037844387076, 1.000000000000000000, 0.8660254037844387076, 1.000000000000000000, 0.8660254037844387076, 1.000000000000000000, 0.8660254037844387076, 1.000000000000000000, 0.8660254037844387076, 1.000000000000000000, 0.8660254037844387076, 1.000000000000000000, 0.8660254037844387076, 1.000000000000000000, 0.8660254037844387076, 1.000000000000000000, 0.8660254037844387076, 1.000000000000000000, 0.8660254037844387076, 1.000000000000000000, 0.8660254037844387076, 1.000000000000000000, 0.8660254037844387076, 1.000000000000000000, 0.8660254037844387076, 1.000000000000000000, 0.8660254037844387076, 1.000000000000000000, 0.8660254037844387076, 1.000000000000000000, 0.8660254037844387076, 1.000000000000000000, 0.8660254037844387076, 1.000000000000000000, 0.8660254037844387076, 1.000000000000000000, 0.8660254037844387076, 1.000000000000000000, 0.8660254037844387076, 1.000000000000000000, 0.8660254037844387076, 1.000000000000000000, 0.8660254037844387076, 1.000000000000000000, 0.8660254037844387076, 1.000000000000000000, 0.8660254037844387076, 1.000000000000000000, 0.8660254037844387076, 1.000000000000000000, 0.8660254037844387076, 1.000000000000000000, 0.8660254037844387076, 1.000000000000000000, 0.8660254037844387076, 1.000000000000000000, 0.8660254037844387076, 1.000000000000000000, 0.8660254037844387076, 1.000000000000000000, 0.8660254037844387076, 1.000000000000000000, 0.8660254037844387076, 1.000000000000000000, 0.8660254037844387076, 1.000000000000000000, 0.8660254037844387076, 1.000000000000000000, 0.8660254037844387076, 1.000000000000000000, 0.8660254037844387076, 1.000000000000000000, 0.8660254037844387076, 1.000000000000000000, 0.8660254037844387076, 1.000000000000000000, 0.8660254037844387076, 1.000000000000000000, 0.8660254037844387076, 1.000000000000000000),
 ( 1.000000000000000000, 0.8660254037844387076, 1.000000000000000000, 0.8660254037844387076, 1.000000000000000000, 0.8660254037844387076, 1.000000000000000000, 0.8660254037844387076, 1.000000000000000000, 0.8660254037844387076, 1.000000000000000000, 0.8660254037844387076, 1.000000000000000000, 0.8660254037844387076, 1.000000000000000000, 0.8660254037844387076, 1.000000000000000000, 0.8660254037844387076, 1.000000000000000000, 0.8660254037844387076, 1.000000000000000000, 0.8660254037844387076, 1.000000000000000000, 0.8660254037844387076, 1.000000000000000000, 0.8660254037844387076, 1.000000000000000000, 0.8660254037844387076, 1.000000000000000000, 0.8660254037844387076, 1.000000000000000000, 0.8660254037844387076, 1.000000000000000000, 0.8660254037844387076, 1.000000000000000000, 0.8660254037844387076, 1.000000000000000000, 0.8660254037844387076, 1.000000000000000000, 0.8660254037844387076, 1.000000000000000000, 0.8660254037844387076, 1.000000000000000000, 0.8660254037844387076, 1.000000000000000000, 0.8660254037844387076, 1.000000000000000000, 0.8660254037844387076, 1.000000000000000000, 0.8660254037844387076, 1.000000000000000000, 0.8660254037844387076, 1.000000000000000000, 0.8660254037844387076, 1.000000000000000000, 0.8660254037844387076, 1.000000000000000000, 0.8660254037844387076, 1.000000000000000000, 0.8660254037844387076, 1.000000000000000000, 0.8660254037844387076, 1.000000000000000000, 0.8660254037844387076, 1.000000000000000000, 0.8660254037844387076, 1.000000000000000000, 0.8660254037844387076, 1.000000000000000000, 0.8660254037844387076, 1.000000000000000000, 0.8660254037844387076, 1.000000000000000000, 0.8660254037844387076, 1.000000000000000000, 0.8660254037844387076, 1.000000000000000000, 0.8660254037844387076, 1.000000000000000000, 0.8660254037844387076, 1.000000000000000000, 0.8660254037844387076, 1.000000000000000000, 0.8660254037844387076, 1.000000000000000000, 0.8660254037844387076, 1.000000000000000000, 0.8660254037844387076, 1.000000000000000000, 0.8660254037844387076, 1.000000000000000000, 0.8660254037844387076, 1.000000000000000000, 0.8660254037844387076, 1.000000000000000000, 0.8660254037844387076, 1.000000000000000000, 0.8660254037844387076, 1.000000000000000000, 0.8660254037844387076, 1.000000000000000000, 0.8660254037844387076, 1.000000000000000000, 0.8660254037844387076, 1.000000000000000000, 0.8660254037844387076, 1.000000000000000000, 0.8660254037844387076, 1.000000000000000000, 0.8660254037844387076, 1.000000000000000000, 0.8660254037844387076, 1.000000000000000000, 0.8660254037844387076, 1.000000000000000000, 0.8660254037844387076, 1.000000000000000000, 0.8660254037844387076, 1.000000000000000000, 0.8660254037844387076, 1.000000000000000000, 0.8660254037844387076, 1.000000000000000000, 0.8660254037844387076, 1.000000000000000000, 0.8660254037844387076, 1.000000000000000000, 0.8660254037844387076, 1.000000000000000000, 0.8660254037844387076, 1.000000000000000000, 0.8660254037844387076, 1.000000000000000000, 0.8660254037844387076, 1.000000000000000000, 0.8660254037844387076, 1.000000000000000000, 0.8660254037844387076, 1.000000000000000000, 0.8660254037844387076, 1.000000000000000000, 0.8660254037844387076, 1.000000000000000000, 0.8660254037844387076, 1.000000000000000000, 0.8660254037844387076, 1.000000000000000000, 0.8660254037844387076, 1.000000000000000000, 0.8660254037844387076, 1.000000000000000000, 0.8660254037844387076, 1.000000000000000000, 0.8660254037844387076, 1.000000000000000000, 0.8660254037844387076, 1.000000000000000000, 0.8660254037844387076, 1.000000000000000000, 0.8660254037844387076, 1.000000000000000000, 0.8660254037844387076, 1.000000000000000000, 0.8660254037844387076, 1.000000000000000000, 0.8660254037844387076, 1.000000000000000000, 0.8660254037844387076, 1.000000000000000000, 0.8660254037844387076, 1.000000000000000000, 0.8660254037844387076, 1.000000000000000000, 0.8660254037844387076, 1.000000000000000000, 0.8660254037844387076, 1.000000000000000000, 0.8660254037844387076, 1.000000000000000000, 0.8660254037844387076, 1.000000000000000000, 0.8660254037844387076, 1.000000000000000000, 0.8660254037844387076, 1.000000000000000000, 0.8660254037844387076, 1.000000000000000000, 0.8660254037844387076, 1.000000000000000000, 0.8660254037844387076, 1.000000000000000000, 0.8660254037844387076, 1.000000000000000000, 0.8660254037844387076, 1.000000000000000000, 0.8660254037844387076, 1.000000000000000000, 0.8660254037844387076, 1.000000000000000000, 0.8660254037844387076, 1.000000000000000000, 0.8660254037844387076, 1.000000000000000000, 0.8660254037844387076, 1.000000000000000000, 0.8660254037844387076, 1.000000000000000000, 0.8660254037844387076, 1.000000000000000000, 0.8660254037844387076, 1.000000000000000000, 0.8660254037844387076, 1.000000000000000000, 0.8660254037844387076, 1.000000000000000000, 0.8660254037844387076, 1.000000000000000000, 0.8660254037844387076, 1.000000000000000000, 0.8660254037844387076, 1.000000000000000000, 0.8660254037844387076, 1.000000000000000000, 0.8660254037844387076, 1.000000000000000000, 0.8660254037844387076, 1.000000000000000000, 0.8660254037844387076, 1.000000000000000000, 0.8660254037844387076, 1.000000000000000000, 0.8660254037844387076, 1.000000000000000000, 0.8660254037844387076, 1.000000000000000000, 0.8660254037844387076, 1.000000000000000000, 0.8660254037844387076, 1.000000000000000000, 0.8660254037844387076, 1.000000000000000000) ) ) 
 REPRESENTATION_ITEM ( '' )  SURFACE ( )  );
#115282=EDGE_CURVE ( 'NONE', #139590, #93819, #125512, .T. ) ;
#115283=ORIENTED_EDGE ( 'NONE', *, *, #133829, .F. ) ;
#115284=CARTESIAN_POINT ( 'NONE',  ( -5.818384198920079520, 6.817144982608731141, 1.199719254218452935 ) ) ;
#115286=CARTESIAN_POINT ( 'NONE',  ( 5.844973620822830895, 8.872867420051733234, 1.082531754730549967 ) ) ;
#115291=CARTESIAN_POINT ( 'NONE',  ( -6.903036488013351679, 8.082572653217566128, -1.199719254218452047 ) ) ;
#115301=CARTESIAN_POINT ( 'NONE',  ( -6.936931872047518155, 8.122117267924091166, 1.199719254218452047 ) ) ;
#115313=CARTESIAN_POINT ( 'NONE',  ( -5.204350862799341115, 7.165104988056252289, -1.599625672291271394 ) ) ;
#115318=CARTESIAN_POINT ( 'NONE',  ( -5.302647476720585118, 9.200522799567075083, 0.000000000000000000 ) ) ;
#115320=CARTESIAN_POINT ( 'NONE',  ( -7.743115126736118015, 8.206258200713163475, 0.7216878364870317197 ) ) ;
#115321=CARTESIAN_POINT ( 'NONE',  ( 7.014364370223726830, 9.276787413384745662, -1.599625672291269396 ) ) ;
#115322=CARTESIAN_POINT ( 'NONE',  ( -4.136646265500970365, 5.919449624541475607, -1.443375672974066548 ) ) ;
#115337=CARTESIAN_POINT ( 'NONE',  ( -0.4592128676388293473, 2.866047475813795486, 1.947548603248408616 ) ) ;
#115341=CARTESIAN_POINT ( 'NONE',  ( 6.270956187569860063, 6.991113019333711875, 0.9580997929081371822 ) ) ;
#115348=CARTESIAN_POINT ( 'NONE',  ( 5.574911853349990842, 7.504993371562844295, -1.384166627116256709 ) ) ;
#115360=CARTESIAN_POINT ( 'NONE',  ( 6.403672513108120690, 6.804938187689173468, -0.5019199613840990004 ) ) ;
#115365=AXIS2_PLACEMENT_3D ( 'NONE', #168513, #114512, #180508 ) ;
#115375=CARTESIAN_POINT ( 'NONE',  ( 6.851666526859736983, 9.086973262793417661, -1.599625672291269396 ) ) ;
#115378=CARTESIAN_POINT ( 'NONE',  ( -4.145761110728687804, 8.058748072483927771, -0.7998128361456481317 ) ) ;
#115391=AXIS2_PLACEMENT_3D ( 'NONE', #140242, #206263, #9140 ) ;
#115393=CARTESIAN_POINT ( 'NONE',  ( 5.086243903782109221, 5.962981304947771122, -1.199719254218452047 ) ) ;
#115395=CARTESIAN_POINT ( 'NONE',  ( 7.693325821111733021, 7.940244644243982464, -0.7998128361456341429 ) ) ;
#115401=CARTESIAN_POINT ( 'NONE',  ( -7.092323753280154186, 7.447001598347859463, 0.7216878364870317197 ) ) ;
#115407=CARTESIAN_POINT ( 'NONE',  ( 5.989670002187236442, 10.20997511251894529, -0.7998128361456481317 ) ) ;
#115412=CARTESIAN_POINT ( 'NONE',  ( 1.848071122224584251, 8.944961669792201420, 0.7750000000000004663 ) ) ;
#115419=CARTESIAN_POINT ( 'NONE',  ( -7.295696057929500711, 7.684269287105433222, 0.7216878364870317197 ) ) ;
#115420=CARTESIAN_POINT ( 'NONE',  ( 4.258669648468278446, 7.022179452304728287, 1.082531754730549078 ) ) ;
#115429=CARTESIAN_POINT ( 'NONE',  ( -4.821859908315634158, 5.654533310236863564, 1.199719254218452935 ) ) ;
#115430=CARTESIAN_POINT ( 'NONE',  ( -7.132998214565509087, 7.494455136514109661, 0.7216878364870317197 ) ) ;
#115435=CARTESIAN_POINT ( 'NONE',  ( 3.729901657090938460, 7.365652676665848553, 0.7216878364870257245 ) ) ;
#115451=CARTESIAN_POINT ( 'NONE',  ( -4.685165750215470659, 7.704147214923535714, 1.047329974316240753 ) ) ;
#115455=CARTESIAN_POINT ( 'NONE',  ( -4.034433228518296666, 6.864533312316751790, -1.199719254218450271 ) ) ;
#115466=CARTESIAN_POINT ( 'NONE',  ( 2.878073747850912412, 6.579779482459851003, -0.7998128361456362523 ) ) ;
#115469=CARTESIAN_POINT ( 'NONE',  ( 5.879395890181562834, 6.888325289080478697, -1.199719254218452047 ) ) ;
#115476=CARTESIAN_POINT ( 'NONE',  ( -5.906512197408906317, 6.919960980845699439, -1.199719254218453823 ) ) ;
#115501=CARTESIAN_POINT ( 'NONE',  ( 3.879041347285658414, 6.579279767591636130, -1.082531754730548412 ) ) ;
#115507=CARTESIAN_POINT ( 'NONE',  ( 5.356880090730863131, 7.343055753976412525, 1.443375672974064550 ) ) ;
#115519=CARTESIAN_POINT ( 'NONE',  ( -4.633854640820660009, 8.628190524257904670, -0.7998128361456362523 ) ) ;
#115521=CARTESIAN_POINT ( 'NONE',  ( -5.749539660647037032, 8.865490816466966351, 1.199719254218454489 ) ) ;
#115529=CARTESIAN_POINT ( 'NONE',  ( 7.550965208168244125, 7.774157262476569130, -0.7998128361456341429 ) ) ;
#115535=CARTESIAN_POINT ( 'NONE',  ( -6.343235766347277149, 8.493804042195527870, -1.599625672291271394 ) ) ;
#115541=CARTESIAN_POINT ( 'NONE',  ( -5.858531774880906262, 6.967946837850073294, 1.082531754730549078 ) ) ;
#115544=CARTESIAN_POINT ( 'NONE',  ( -5.101610940492132151, 9.173906207207963348, -0.7998128361456362523 ) ) ;
#115563=CARTESIAN_POINT ( 'NONE',  ( -4.841670253855968831, 4.821239182352949904, 0.000000000000000000 ) ) ;
#115564=ORIENTED_EDGE ( 'NONE', *, *, #180702, .F. ) ;
#115565=CARTESIAN_POINT ( 'NONE',  ( -6.688968683495758683, 8.897159112202094988, -1.599625672291271394 ) ) ;
#115566=CARTESIAN_POINT ( 'NONE',  ( 5.032011289327418702, 5.899709921417326974, 1.199719254218452935 ) ) ;
#115567=CARTESIAN_POINT ( 'NONE',  ( -6.317173229324657413, 6.334733287159020954, 0.000000000000000000 ) ) ;
#115586=DIRECTION ( 'NONE',  ( -1.000000000000000000, 0.000000000000000000, 0.000000000000000000 ) ) ;
#115617=CARTESIAN_POINT ( 'NONE',  ( 3.386504508363381571, 7.172948703057747011, -0.7998128361456362523 ) ) ;
#115629=CARTESIAN_POINT ( 'NONE',  ( 4.784634885068531851, 8.146353749921887655, 0.8039021629790907841 ) ) ;
#115631=CARTESIAN_POINT ( 'NONE',  ( 4.913904330310220558, 4.697586238308844919, 0.000000000000000000 ) ) ;
#115636=CARTESIAN_POINT ( 'NONE',  ( -5.098748287191073203, 8.106234214101666780, 1.199719254218452935 ) ) ;
#115643=CARTESIAN_POINT ( 'NONE',  ( -7.146556367734805626, 9.431011410480991231, 1.443375672974064550 ) ) ;
#115647=CARTESIAN_POINT ( 'NONE',  ( -4.916039773278787273, 4.881957280557857715, 0.5603013081572870702 ) ) ;
#115651=EDGE_CURVE ( 'NONE', #162782, #96449, #150081, .T. ) ;
#115652=CARTESIAN_POINT ( 'NONE',  ( 5.777182853198898904, 6.873039762554409293, -1.082531754730548412 ) ) ;
#115655=CARTESIAN_POINT ( 'NONE',  ( -3.772911886352873445, 7.623757310712140800, 0.7998128361456352531 ) ) ;
#115666=CARTESIAN_POINT ( 'NONE',  ( 4.167152111353856547, 5.955039778036558040, 1.599625672291262513 ) ) ;
#115683=CARTESIAN_POINT ( 'NONE',  ( -5.599738924909661186, 5.745725798494749625, 0.2540040342395213369 ) ) ;
#115687=CARTESIAN_POINT ( 'NONE',  ( 6.051950339013592028, 7.082009231019537943, 1.085686599464001478 ) ) ;
#115698=CARTESIAN_POINT ( 'NONE',  ( 7.530627977747744062, 7.750430493652658015, -0.7998128361456341429 ) ) ;
#115706=CARTESIAN_POINT ( 'NONE',  ( 4.421367491832270957, 6.251624388594711590, 1.443375672974058777 ) ) ;
#115709=CARTESIAN_POINT ( 'NONE',  ( 5.533136088152891929, 9.469426179571447832, -0.7216878364870458196 ) ) ;
#115721=CARTESIAN_POINT ( 'NONE',  ( -6.943184063974178422, 8.233374508458908281, -1.082531754730549967 ) ) ;
#115755=CARTESIAN_POINT ( 'NONE',  ( 4.854701522145073334, 7.821512988214679218, -1.199719254218450271 ) ) ;
#115757=CARTESIAN_POINT ( 'NONE',  ( 6.737475991348287785, 6.825086509519945999, -0.7998128361456481317 ) ) ;
#115765=CARTESIAN_POINT ( 'NONE',  ( -2.836231403021655773, 6.427000396871998866, 0.000000000000000000 ) ) ;
#115770=CARTESIAN_POINT ( 'NONE',  ( -3.902768115887413014, 5.646591783325653147, -1.599625672291283607 ) ) ;
#115773=CARTESIAN_POINT ( 'NONE',  ( 3.865483193227626124, 7.523831135491951372, -0.7216878364870338292 ) ) ;
#115775=AXIS2_PLACEMENT_3D ( 'NONE', #148442, #111739, #131185 ) ;
#115782=CARTESIAN_POINT ( 'NONE',  ( -4.309512724297390740, 6.121127159803966933, 1.599625672291270506 ) ) ;
#115789=CARTESIAN_POINT ( 'NONE',  ( -7.919371124158132602, 8.411890197705517380, -0.7216878364870338292 ) ) ;
#115791=CARTESIAN_POINT ( 'NONE',  ( -6.143253000767895600, 6.339752387083549934, 0.000000000000000000 ) ) ;
#115809=CARTESIAN_POINT ( 'NONE',  ( -5.307090785106547415, 5.156303768904543894, -0.7998128361456362523 ) ) ;
#115810=ORIENTED_EDGE ( 'NONE', *, *, #107334, .F. ) ;
#115821=CARTESIAN_POINT ( 'NONE',  ( -5.503684012504701961, 5.385662534202396934, 0.000000000000000000 ) ) ;
#115833=CARTESIAN_POINT ( 'NONE',  ( -4.684263184503158151, 8.377143357790286515, -0.6327197186303500365 ) ) ;
#115850=CARTESIAN_POINT ( 'NONE',  ( 5.631432701629774051, 7.663367133358481631, 1.599625672291269396 ) ) ;
#115855=CARTESIAN_POINT ( 'NONE',  ( -0.1054627972275519465, 3.385846599571567417, -2.076146368081344118 ) ) ;
#115874=CARTESIAN_POINT ( 'NONE',  ( 6.180537922983273091, 8.303989891604203422, -1.599625672291281386 ) ) ;
#115875=CARTESIAN_POINT ( 'NONE',  ( 4.389807875774629942, 8.343469298370917997, 0.7998128361456271485 ) ) ;
#115877=CARTESIAN_POINT ( 'NONE',  ( 3.705121118284530279, 7.544668081299086282, -1.734723475976807094E-15 ) ) ;
#115881=CARTESIAN_POINT ( 'NONE',  ( -4.448483798615272100, 8.203998508444197313, 0.000000000000000000 ) ) ;
#115889=CARTESIAN_POINT ( 'NONE',  ( 5.488371254093075358, 7.473176909139983337, -1.250075884424824757 ) ) ;
#115890=CARTESIAN_POINT ( 'NONE',  ( -4.434925645001610128, 8.188180662561590495, 0.7216878364870338292 ) ) ;
#115891=CARTESIAN_POINT ( 'NONE',  ( 5.397554552016228691, 5.469770863539975991, 0.7216878364870328300 ) ) ;
#115915=CARTESIAN_POINT ( 'NONE',  ( 6.378184920586140727, 6.405913593630768510, 0.000000000000000000 ) ) ;
#115917=CARTESIAN_POINT ( 'NONE',  ( 4.085803189671889157, 5.860132702740892263, -1.599625672291273171 ) ) ;
#115920=EDGE_CURVE ( 'NONE', #103686, #212524, #8283, .T. ) ;
#115935=B_SPLINE_CURVE_WITH_KNOTS ( 'NONE', 3,
 ( #143001, #208999, #111594, #94237 ),
 .UNSPECIFIED., .F., .F.,
 ( 4, 4 ),
 ( 0.000000000000000000, 0.0001936595853974351948 ),
 .UNSPECIFIED. ) ;
#115945=DIRECTION ( 'NONE',  ( 0.000000000000000000, 0.000000000000000000, -1.000000000000000000 ) ) ;
#115946=CARTESIAN_POINT ( 'NONE',  ( 4.844006021832467646, 8.873367135438366304, 0.000000000000000000 ) ) ;
#115950=CARTESIAN_POINT ( 'NONE',  ( -6.197060558222979409, 6.958367536249086882, 0.8797177744420351386 ) ) ;
#115951=CARTESIAN_POINT ( 'NONE',  ( 5.525830126021535449, 8.604496359403894346, -1.199719254218452047 ) ) ;
#115962=CARTESIAN_POINT ( 'NONE',  ( 4.871809496981259535, 8.050285353323946680, -0.9368363805376724862 ) ) ;
#115968=EDGE_CURVE ( 'NONE', #192662, #212849, #32593, .T. ) ;
#115986=CARTESIAN_POINT ( 'NONE',  ( -7.117104292530948229, 7.267986194233038155, -0.7998128361456362523 ) ) ;
#115988=CARTESIAN_POINT ( 'NONE',  ( 5.200434439293556643, 8.224868058221247225, -1.199719254218452047 ) ) ;
#115989=CARTESIAN_POINT ( 'NONE',  ( -5.303674958368855386, 4.754885796981216828, 2.500000000000000444 ) ) ;
#115991=CARTESIAN_POINT ( 'NONE',  ( -4.556949027968976829, 5.449433633119473264, 1.082531754730549078 ) ) ;
#115994=ORIENTED_EDGE ( 'NONE', *, *, #17058, .T. ) ;
#115996=CARTESIAN_POINT ( 'NONE',  ( -7.065207446497166366, 9.336104335703744539, 0.000000000000000000 ) ) ;
#116000=CARTESIAN_POINT ( 'NONE',  ( -6.335246490290919574, 6.944623119882351148, -0.8941629942194727620 ) ) ;
#116018=CARTESIAN_POINT ( 'NONE',  ( 5.180624094197585627, 8.097792972322238825, -1.082531754730548412 ) ) ;
#116030=CARTESIAN_POINT ( 'NONE',  ( -5.655159470675923394, 5.770309935309573923, 0.000000000000000000 ) ) ;
#116032=CARTESIAN_POINT ( 'NONE',  ( 6.737475991348287785, 6.825086509519945999, -0.7998128361456481317 ) ) ;
#116037=CARTESIAN_POINT ( 'NONE',  ( -6.064239847062411926, 10.29697326487330500, 0.000000000000000000 ) ) ;
#116078=CARTESIAN_POINT ( 'NONE',  ( 5.401997860402196316, 5.267028690082820930, 0.000000000000000000 ) ) ;
#116083=CARTESIAN_POINT ( 'NONE',  ( -5.058600711230246461, 7.955432358860325515, 1.082531754730549967 ) ) ;
#116090=CARTESIAN_POINT ( 'NONE',  ( -7.099629715411508890, 8.311931418515415615, 1.199719254218452047 ) ) ;
#116096=CARTESIAN_POINT ( 'NONE',  ( 4.779848517908583894, 4.883929213520019630, -0.7538207499340529028 ) ) ;
#116098=CARTESIAN_POINT ( 'NONE',  ( -6.791708605802965870, 6.888357893050385705, -0.7998128361456362523 ) ) ;
#116099=CARTESIAN_POINT ( 'NONE',  ( -6.966220764712148572, 6.002124920821316323, 2.500000000000000444 ) ) ;
#116101=CARTESIAN_POINT ( 'NONE',  ( 4.941988244637107286, 8.095350367992509177, 1.064974588601754757 ) ) ;
#116106=CARTESIAN_POINT ( 'NONE',  ( 6.587282531393223728, 8.778525268082516320, 1.599625672291268286 ) ) ;
#116116=CARTESIAN_POINT ( 'NONE',  ( -5.978219388983010418, 5.939287140093762574, -0.7998128361456362523 ) ) ;
#116119=VECTOR ( 'NONE', #72470, 1000.000000000000000 ) ;
#116122=CARTESIAN_POINT ( 'NONE',  ( -6.286140498591554326, 7.362860665558790707, 1.199719254218452047 ) ) ;
#116127=CARTESIAN_POINT ( 'NONE',  ( 5.655159470231527763, 9.611786791996525636, -0.7216878364870458196 ) ) ;
#116129=CARTESIAN_POINT ( 'NONE',  ( -6.360183458142173230, 9.473945563590925545, 1.082531754730549967 ) ) ;
#116135=CARTESIAN_POINT ( 'NONE',  ( 4.993145711582793744, 9.047363440147082159, -0.7998128361456481317 ) ) ;
#116136=ORIENTED_EDGE ( 'NONE', *, *, #33908, .T. ) ;
#116151=CARTESIAN_POINT ( 'NONE',  ( 6.272253174914359519, 6.990222103910356921, -0.9563742486745248073 ) ) ;
#116167=CARTESIAN_POINT ( 'NONE',  ( 4.644395130292630292, 8.311692339142366492, -0.4369040224408097250 ) ) ;
#116180=CARTESIAN_POINT ( 'NONE',  ( -5.717536675473545493, 7.305230138711669596, -1.214019596050613492 ) ) ;
#116188=DIRECTION ( 'NONE',  ( 0.000000000000000000, 1.000000000000000000, 0.000000000000000000 ) ) ;
#116196=DIRECTION ( 'NONE',  ( 1.000000000000000000, 0.000000000000000000, 0.000000000000000000 ) ) ;
#116200=CARTESIAN_POINT ( 'NONE',  ( -6.330731382938325602, 6.350551133041632212, 0.7998128361456281477 ) ) ;
#116202=CARTESIAN_POINT ( 'NONE',  ( 8.025500584646550806, 8.327781868367935658, 0.000000000000000000 ) ) ;
#116214=VERTEX_POINT ( 'NONE', #175421 ) ;
#116215=CARTESIAN_POINT ( 'NONE',  ( 6.638652492546827766, 7.774124658506663010, 1.199719254218452047 ) ) ;
#116217=CARTESIAN_POINT ( 'NONE',  ( 5.492461626867537916, 9.421972641405202964, -0.7216878364870458196 ) ) ;
#116230=CARTESIAN_POINT ( 'NONE',  ( -6.283277845290492714, 6.295188672452495915, -0.7998128361456362523 ) ) ;
#116231=CARTESIAN_POINT ( 'NONE',  ( 5.890091390494168522, 5.836471141856793388, 0.000000000000000000 ) ) ;
#116241=CARTESIAN_POINT ( 'NONE',  ( -3.006876207180748217, 6.730049018344652190, -0.7998128361456481317 ) ) ;
#116242=CARTESIAN_POINT ( 'NONE',  ( 6.505933609711257226, 8.683618192786854095, -1.599625672291281386 ) ) ;
#116250=CARTESIAN_POINT ( 'NONE',  ( 3.217027588192558074, 6.975225629525113824, -1.734723475976807094E-15 ) ) ;
#116252=CARTESIAN_POINT ( 'NONE',  ( -0.4525991836887841013, 2.827044806229560336, 1.949989785391225361 ) ) ;
#116256=CARTESIAN_POINT ( 'NONE',  ( -6.279577920751266973, 6.982973266031838655, 0.9645283542769074181 ) ) ;
#116264=CARTESIAN_POINT ( 'NONE',  ( -3.472296738431328134, 7.065113604896248845, 0.000000000000000000 ) ) ;
#116271=CARTESIAN_POINT ( 'NONE',  ( -3.614985261929179128, 3.508924507031892848, 2.500000000000000000 ) ) ;
#116286=CARTESIAN_POINT ( 'NONE',  ( -6.337068562759858636, 6.936200024879327408, -0.9492287992594623525 ) ) ;
#116294=CARTESIAN_POINT ( 'NONE',  ( 3.888156192069020634, 7.758209000714329839, 1.040834085586084257E-14 ) ) ;
#116312=CARTESIAN_POINT ( 'NONE',  ( 0.2032326336602353622, 3.360045134790890842, 2.069225858299823084 ) ) ;
#116314=CARTESIAN_POINT ( 'NONE',  ( 4.420840606507738357, 7.315341919971147355, 1.199719254218451159 ) ) ;
#116315=CARTESIAN_POINT ( 'NONE',  ( -5.167065940583949413, 5.200867483535597913, 0.000000000000000000 ) ) ;
#116329=DIRECTION ( 'NONE',  ( 0.6095094443605824086, -2.582722057095079198E-12, -0.7927788072566358535 ) ) ;
#116340=EDGE_LOOP ( 'NONE', ( #183171, #158142, #109566, #61805 ) ) ;
#116341=CARTESIAN_POINT ( 'NONE',  ( -4.959250327548641479, 9.007818825440551791, -0.7998128361456362523 ) ) ;
#116353=( BOUNDED_CURVE ( )  B_SPLINE_CURVE ( 2, ( #124191, #103586, #87332, #186952, #72123 ),
 .UNSPECIFIED., .F., .T. ) 
 B_SPLINE_CURVE_WITH_KNOTS ( ( 3, 2, 3 ),
 ( 0.5000000000000000000, 0.5083333333333333037, 0.5121012724118086945 ),
 .UNSPECIFIED. ) 
 CURVE ( )  GEOMETRIC_REPRESENTATION_ITEM ( )  RATIONAL_B_SPLINE_CURVE ( ( 1.000000000000000000, 0.8660254037844387076, 1.000000000000000000, 0.9394230260075716599, 0.9336261354299888460 ) ) 
 REPRESENTATION_ITEM ( '' )  );
#116356=CARTESIAN_POINT ( 'NONE',  ( -7.259464905474441565, 7.434073576000447048, -0.7998128361456362523 ) ) ;
#116363=CARTESIAN_POINT ( 'NONE',  ( 4.686278372178935392, 5.496354851410763409, 1.199719254218452047 ) ) ;
#116369=CARTESIAN_POINT ( 'NONE',  ( -10.17567228521070710, -0.02076350362892331880, 2.419999999999999485 ) ) ;
#116370=CARTESIAN_POINT ( 'NONE',  ( -5.529746549527323474, 7.544733289238903851, -1.599625672291271394 ) ) ;
#116373=CARTESIAN_POINT ( 'NONE',  ( -7.132998214565509087, 7.494455136514109661, 0.7216878364870317197 ) ) ;
#116375=CARTESIAN_POINT ( 'NONE',  ( -6.197485614778184271, 9.284131412999601096, 1.082531754730549967 ) ) ;
#116376=CARTESIAN_POINT ( 'NONE',  ( 6.688968683495743583, 8.897159112202094988, -1.599625672291283607 ) ) ;
#116377=CARTESIAN_POINT ( 'NONE',  ( -6.474900878978163021, 9.711745571186627402, -1.199719254218452047 ) ) ;
#116379=VERTEX_POINT ( 'NONE', #45422 ) ;
#116395=CARTESIAN_POINT ( 'NONE',  ( -1.833030277982346634, 2.531131934864056632, -2.499999999999998668 ) ) ;
#116396=CARTESIAN_POINT ( 'NONE',  ( 6.582202237817778467, 6.781708767774706104, 0.2773405359152263383 ) ) ;
#116403=CARTESIAN_POINT ( 'NONE',  ( 5.900277318768097246, 7.249539301847896411, -1.301905728482563251 ) ) ;
#116416=CARTESIAN_POINT ( 'NONE',  ( 6.151318917739748038, 6.974181327834800825, -0.9227930848511676221 ) ) ;
#116427=CARTESIAN_POINT ( 'NONE',  ( -2.428612866367529932E-14, 2.999999999999999112, 7.500000000000000000 ) ) ;
#116429=CARTESIAN_POINT ( 'NONE',  ( 5.989670002187236442, 10.20997511251894529, -0.7998128361456481317 ) ) ;
#116432=CARTESIAN_POINT ( 'NONE',  ( -5.004894982100124068, 5.868074229652107121, 1.199719254218452935 ) ) ;
#116445=CARTESIAN_POINT ( 'NONE',  ( 3.400062661977048428, 7.188766548940353829, -1.734723475976807094E-15 ) ) ;
#116447=CARTESIAN_POINT ( 'NONE',  ( 6.261886844665240481, 8.398896966899865646, 1.599625672291268286 ) ) ;
#116454=CARTESIAN_POINT ( 'NONE',  ( -6.739811759324831897, 7.996106819701333634, -1.082531754730549967 ) ) ;
#116460=CARTESIAN_POINT ( 'NONE',  ( 7.472478939787284169, 8.746922180287201698, 1.199719254218452935 ) ) ;
#116463=CIRCLE ( 'NONE', #16183, 0.7499999999999997780 ) ;
#116473=EDGE_CURVE ( 'NONE', #111396, #183890, #92089, .T. ) ;
#116476=CARTESIAN_POINT ( 'NONE',  ( -5.804299160426237059, 7.865044668620976509, -1.443375672974066548 ) ) ;
#116477=CARTESIAN_POINT ( 'NONE',  ( 5.451787166470912993, 6.493411461371761284, -1.082531754730548412 ) ) ;
#116483=DIRECTION ( 'NONE',  ( 0.000000000000000000, 0.000000000000000000, -1.000000000000000000 ) ) ;
#116488=CARTESIAN_POINT ( 'NONE',  ( -4.390861645979385663, 6.216034235099629157, -1.599625672291271394 ) ) ;
#116489=CARTESIAN_POINT ( 'NONE',  ( -6.048345925472225382, 8.149765894507963182, 1.443375672974058777 ) ) ;
#116490=CARTESIAN_POINT ( 'NONE',  ( 7.876360894896227371, 8.153785563659219804, -0.7998128361456341429 ) ) ;
#116493=CARTESIAN_POINT ( 'NONE',  ( 5.085717018457579286, 6.066329622022862189, -1.082531754730548412 ) ) ;
#116507=CARTESIAN_POINT ( 'NONE',  ( 2.957086901556340575, 6.464035461875470290, 0.7216878364870257245 ) ) ;
#116510=CARTESIAN_POINT ( 'NONE',  ( -3.630551273409382329, 7.457669928944732796, 0.7998128361456352531 ) ) ;
#116521=CARTESIAN_POINT ( 'NONE',  ( 3.230585741806197841, 6.991043475407723307, 0.7998128361456271485 ) ) ;
#116560=CARTESIAN_POINT ( 'NONE',  ( 4.407809338218622308, 8.156544971314787063, 0.000000000000000000 ) ) ;
#116565=CARTESIAN_POINT ( 'NONE',  ( 5.600926855776875435, 7.627776979863398310, -1.443375672974078761 ) ) ;
#116579=CARTESIAN_POINT ( 'NONE',  ( -5.271087860662956537, 9.371629280740593870, 0.000000000000000000 ) ) ;
#116591=CARTESIAN_POINT ( 'NONE',  ( 7.472478939787284169, 8.746922180287201698, 1.199719254218452935 ) ) ;
#116597=CARTESIAN_POINT ( 'NONE',  ( -7.747558435566414659, 8.003516027774422170, -0.7998128361456362523 ) ) ;
#116603=CARTESIAN_POINT ( 'NONE',  ( -6.346625304972878467, 7.537389289624049304, 1.082531754730548412 ) ) ;
#116607=CARTESIAN_POINT ( 'NONE',  ( -5.611095471209320174, 7.639640364534566075, 1.599625672291263179 ) ) ;
#116622=DIRECTION ( 'NONE',  ( -0.000000000000000000, -1.000000000000000000, -0.000000000000000000 ) ) ;
#116628=CARTESIAN_POINT ( 'NONE',  ( -4.855228407469635243, 4.837057028235559386, 0.7216878364870257245 ) ) ;
#116630=CARTESIAN_POINT ( 'NONE',  ( -4.462041952228957165, 5.338708711422782471, -1.082531754730549967 ) ) ;
#116631=CARTESIAN_POINT ( 'NONE',  ( 3.562760505341037831, 7.378580699531681830, -1.734723475976807094E-15 ) ) ;
#116632=CARTESIAN_POINT ( 'NONE',  ( -5.306037014901836990, 7.283738832175834510, 1.599625672291263179 ) ) ;
#116639=EDGE_LOOP ( 'NONE', ( #159214, #190978, #63895, #158155 ) ) ;
#116645=ORIENTED_EDGE ( 'NONE', *, *, #149694, .F. ) ;
#116651=CARTESIAN_POINT ( 'NONE',  ( 4.529832720741620022, 7.338536369956936589, -1.082531754730548412 ) ) ;
#116682=CARTESIAN_POINT ( 'NONE',  ( 3.576318658954677598, 7.394398545414291313, 0.7998128361456281477 ) ) ;
#116695=CARTESIAN_POINT ( 'NONE',  ( 4.649081266440608928, 8.305916344280937835, -0.4560373724170601606 ) ) ;
#116697=CARTESIAN_POINT ( 'NONE',  ( 7.865138509703455405, 8.348618814175074121, -0.7216878364870317197 ) ) ;
#116703=CARTESIAN_POINT ( 'NONE',  ( -5.088052786878465739, 9.158088361325352977, 0.000000000000000000 ) ) ;
#116706=ORIENTED_EDGE ( 'NONE', *, *, #105660, .T. ) ;
#116709=CARTESIAN_POINT ( 'NONE',  ( -7.417719440008134768, 7.826629899530511025, 0.7216878364870317197 ) ) ;
#116711=CARTESIAN_POINT ( 'NONE',  ( -4.933139366528609848, 7.815959757607085834, 1.092252181328734473 ) ) ;
#116712=AXIS2_PLACEMENT_3D ( 'NONE', #141476, #116188, #131371 ) ;
#116717=CARTESIAN_POINT ( 'NONE',  ( 5.397554552016212703, 8.350878506444006533, 1.082531754730547524 ) ) ;
#116720=CARTESIAN_POINT ( 'NONE',  ( -5.957882158562513908, 5.915560371269843465, -0.7998128361456362523 ) ) ;
#116732=CARTESIAN_POINT ( 'NONE',  ( 4.390861645979372341, 6.216034235099629157, -1.599625672291269396 ) ) ;
#116733=CARTESIAN_POINT ( 'NONE',  ( 3.953084306836263995, 6.769626237021087789, 1.199719254218452047 ) ) ;
#116739=EDGE_LOOP ( 'NONE', ( #183521, #143227, #198080, #172941, #112911 ) ) ;
#116752=DIRECTION ( 'NONE',  ( 0.000000000000000000, 0.000000000000000000, 1.000000000000000000 ) ) ;
#116758=CARTESIAN_POINT ( 'NONE',  ( 6.749980374757213575, 8.968339418673846097, 1.599625672291268286 ) ) ;
#116760=B_SPLINE_CURVE_WITH_KNOTS ( 'NONE', 3,
 ( #178738, #177670, #140934, #79082, #145201, #141999, #211207, #128992, #43413, #99600 ),
 .UNSPECIFIED., .F., .F.,
 ( 4, 3, 3, 4 ),
 ( 4.570397642887432356E-18, 3.125189670681054644E-05, 5.835922535859565738E-05, 8.547800541132622365E-05 ),
 .UNSPECIFIED. ) ;
#116767=CARTESIAN_POINT ( 'NONE',  ( 5.830888582329017744, 8.960397891762626799, -1.199719254218452047 ) ) ;
#116769=CIRCLE ( 'NONE', #120199, 2.000000000000000000 ) ;
#116774=CARTESIAN_POINT ( 'NONE',  ( 5.289089323106923146, 6.303597310780433283, -1.082531754730548412 ) ) ;
#116777=CARTESIAN_POINT ( 'NONE',  ( 5.722950238744187956, 9.690876021928001904, 0.7216878364870317197 ) ) ;
#116789=CARTESIAN_POINT ( 'NONE',  ( 6.176125489850557315, 6.957122458884915872, -0.8945188991977878201 ) ) ;
#116790=CARTESIAN_POINT ( 'NONE',  ( -5.912764389335557702, 8.951956649983198844, 1.082531754730550855 ) ) ;
#116807=ORIENTED_EDGE ( 'NONE', *, *, #10571, .F. ) ;
#116823=CARTESIAN_POINT ( 'NONE',  ( 7.126746022638799971, 8.343567110280638133, 1.199719254218452047 ) ) ;
#116825=CARTESIAN_POINT ( 'NONE',  ( 4.199993725183334803, 8.122019456014369254, -0.7998128361456362523 ) ) ;
#116840=CARTESIAN_POINT ( 'NONE',  ( -4.984557751679625781, 5.844347460828191565, 1.199719254218452935 ) ) ;
#116842=CARTESIAN_POINT ( 'NONE',  ( 4.529832720297257254, 8.298905583739861314, 0.000000000000000000 ) ) ;
#116850=CARTESIAN_POINT ( 'NONE',  ( -5.320648938720212051, 5.172121614787156929, 0.000000000000000000 ) ) ;
#116856=CARTESIAN_POINT ( 'NONE',  ( -6.943184063974178422, 8.233374508458908281, -1.082531754730549967 ) ) ;
#116858=CARTESIAN_POINT ( 'NONE',  ( -5.397554552016258889, 7.390509292142662723, 1.443375672974058777 ) ) ;
#116868=DIRECTION ( 'NONE',  ( 0.000000000000000000, -1.000000000000000000, 0.000000000000000000 ) ) ;
#116886=CARTESIAN_POINT ( 'NONE',  ( -4.167152111353897403, 5.955039778036558040, 1.599625672291270506 ) ) ;
#116898=CARTESIAN_POINT ( 'NONE',  ( -4.728114892278019177, 8.325812319508695936, -0.7463954279460782715 ) ) ;
#116916=CARTESIAN_POINT ( 'NONE',  ( 6.200875153403774043, 8.327716660428123419, -1.599625672291283607 ) ) ;
#116928=ADVANCED_FACE ( 'NONE', ( #206216, #76225, #59977, #160685 ), #144479, .T. ) ;
#116938=CARTESIAN_POINT ( 'NONE',  ( 7.367930134383754215, 7.560616343061329125, -0.7998128361456341429 ) ) ;
#116939=CARTESIAN_POINT ( 'NONE',  ( 4.064412189046650248, 7.963840997188264659, 0.7998128361456271485 ) ) ;
#116941=CARTESIAN_POINT ( 'NONE',  ( 3.854260808034858155, 7.718664386007802136, -0.7998128361456362523 ) ) ;
#116952=LINE ( 'NONE', #102780, #195408 ) ;
#116956=CARTESIAN_POINT ( 'NONE',  ( 4.616554244727909762, 8.463227371007752353, -0.2998622348379786362 ) ) ;
#116957=CARTESIAN_POINT ( 'NONE',  ( -5.926322542504872892, 8.007405281046052536, -1.443375672974066548 ) ) ;
#116958=CARTESIAN_POINT ( 'NONE',  ( 5.289089323106923146, 6.303597310780433283, -1.082531754730548412 ) ) ;
#116983=CARTESIAN_POINT ( 'NONE',  ( 4.694866332082116678, 8.699370830729650450, 0.7998128361456341429 ) ) ;
#117011=CARTESIAN_POINT ( 'NONE',  ( -2.837146587356454752, 6.532031128549641075, -0.3849993420583495141 ) ) ;
#117012=CARTESIAN_POINT ( 'NONE',  ( 5.993586425693011144, 9.150212042353954800, -1.199719254218452047 ) ) ;
#117018=CARTESIAN_POINT ( 'NONE',  ( -6.370507937826336509, 6.842553425211714391, 0.6026486057824770315 ) ) ;
#117019=CARTESIAN_POINT ( 'NONE',  ( 7.537407054554579489, 7.758339416593960536, 0.000000000000000000 ) ) ;
#117052=CARTESIAN_POINT ( 'NONE',  ( -6.444921918449773024, 8.612437886315108315, 1.599625672291269396 ) ) ;
#117054=CARTESIAN_POINT ( 'NONE',  ( 5.176180785367283654, 9.260904359562321275, -0.7998128361456481317 ) ) ;
#117062=FACE_OUTER_BOUND ( 'NONE', #70118, .T. ) ;
#117075=CARTESIAN_POINT ( 'NONE',  ( 6.424584688029230328, 8.588711117491191871, 1.599625672291268286 ) ) ;
#117084=CARTESIAN_POINT ( 'NONE',  ( 4.913904330310220558, 4.697586238308844919, 0.000000000000000000 ) ) ;
#117087=EDGE_LOOP ( 'NONE', ( #53197, #157230, #20530, #95479 ) ) ;
#117096=CARTESIAN_POINT ( 'NONE',  ( -4.014622883422329203, 6.737458226417744278, -1.082531754730546636 ) ) ;
#117098=CARTESIAN_POINT ( 'NONE',  ( 5.525830126021535449, 8.604496359403894346, -1.199719254218452047 ) ) ;
#117104=CARTESIAN_POINT ( 'NONE',  ( -5.029148636026397945, 4.832037928311032182, 0.7998128361456281477 ) ) ;
#117126=CARTESIAN_POINT ( 'NONE',  ( -5.823017895876262173, 7.308274721394978357, -1.333157625313810879 ) ) ;
#117140=EDGE_CURVE ( 'NONE', #51039, #95128, #140194, .T. ) ;
#117144=CARTESIAN_POINT ( 'NONE',  ( 3.255366281057017197, 6.812028071292901998, -0.7216878364870338292 ) ) ;
#117150=CARTESIAN_POINT ( 'NONE',  ( 4.577813143269636065, 5.369812084349879555, -1.199719254218450271 ) ) ;
#117152=CARTESIAN_POINT ( 'NONE',  ( -4.163329363839114450, 7.870638172372564689, 0.03594691204382176319 ) ) ;
#117153=CARTESIAN_POINT ( 'NONE',  ( -6.283277845290492714, 6.295188672452495915, -0.7998128361456362523 ) ) ;
#117157=CARTESIAN_POINT ( 'NONE',  ( -5.383996397958228819, 8.335060660042973524, 1.082531754730550855 ) ) ;
#117163=CARTESIAN_POINT ( 'NONE',  ( -5.912237504011027767, 9.055304967058290799, 1.199719254218454489 ) ) ;
#117168=ORIENTED_EDGE ( 'NONE', *, *, #99878, .T. ) ;
#117169=CARTESIAN_POINT ( 'NONE',  ( 4.732378691258949388, 4.890468360863969188, -0.8126286185507647364 ) ) ;
#117172=CARTESIAN_POINT ( 'NONE',  ( -6.629010762438975135, 6.698543742459062145, -0.7998128361456362523 ) ) ;
#117174=CARTESIAN_POINT ( 'NONE',  ( 4.641000714467984345, 8.433135692799648808, 0.4354600853693716411 ) ) ;
#117180=CARTESIAN_POINT ( 'NONE',  ( 5.508355548902068577, 9.648441583686274470, 0.7998128361456331437 ) ) ;
#117186=CARTESIAN_POINT ( 'NONE',  ( -5.004894982100124068, 5.868074229652107121, 1.199719254218452935 ) ) ;
#117188=AXIS2_PLACEMENT_3D ( 'NONE', #102539, #118851, #39678 ) ;
#117191=CARTESIAN_POINT ( 'NONE',  ( -6.771371375382467583, 6.864631124226471037, -0.7998128361456362523 ) ) ;
#117196=CARTESIAN_POINT ( 'NONE',  ( 6.143253000323500856, 10.18122924377050609, -0.7216878364870458196 ) ) ;
#117198=CARTESIAN_POINT ( 'NONE',  ( -6.061904078641520144, 10.08632216847484031, 0.7216878364870267237 ) ) ;
#117200=EDGE_CURVE ( 'NONE', #198620, #41470, #153813, .T. ) ;
#117205=CARTESIAN_POINT ( 'NONE',  ( 6.866278450678116485, 6.975356045404744521, 0.000000000000000000 ) ) ;
#117218=CARTESIAN_POINT ( 'NONE',  ( 5.595231165798738360, 7.497995327707586810, -1.335214257040851615 ) ) ;
#117231=ORIENTED_EDGE ( 'NONE', *, *, #202906, .T. ) ;
#117240=CARTESIAN_POINT ( 'NONE',  ( 5.982890925380405456, 10.20206618957764100, 0.000000000000000000 ) ) ;
#117241=ORIENTED_EDGE ( 'NONE', *, *, #40298, .F. ) ;
#117245=CARTESIAN_POINT ( 'NONE',  ( -6.300768610526733760, 6.888587422923714954, -0.7334343799849201151 ) ) ;
#117265=CARTESIAN_POINT ( 'NONE',  ( -4.468294144155606773, 7.370704380560280100, 1.199719254218452935 ) ) ;
#117279=CARTESIAN_POINT ( 'NONE',  ( 5.855142236255289845, 7.924361590421551860, -1.599625672291281386 ) ) ;
#117280=CARTESIAN_POINT ( 'NONE',  ( 2.925527285498711549, 6.635141943048991742, 0.7998128361456281477 ) ) ;
#117282=CARTESIAN_POINT ( 'NONE',  ( 5.356880090730857802, 8.303424968277756335, 1.082531754730548412 ) ) ;
#117297=CARTESIAN_POINT ( 'NONE',  ( -4.960304097753355457, 6.880383762169266504, 1.599625672291263179 ) ) ;
#117298=CARTESIAN_POINT ( 'NONE',  ( 5.448397627845284141, 7.449826213943242514, 1.599625672291268286 ) ) ;
#117307=CARTESIAN_POINT ( 'NONE',  ( -7.587723245503481095, 8.881373870289390737, 1.199719254218452047 ) ) ;
#117308=CARTESIAN_POINT ( 'NONE',  ( 4.435452530326143616, 5.203724702582467998, -1.199719254218452047 ) ) ;
#117310=CARTESIAN_POINT ( 'NONE',  ( -3.855102659574312973, 8.506872032339167333, -2.500000000000000888 ) ) ;
#117316=CARTESIAN_POINT ( 'NONE',  ( 3.705121118284530279, 7.544668081299086282, -1.734723475976807094E-15 ) ) ;
#117318=CARTESIAN_POINT ( 'NONE',  ( 5.550083779947807550, 7.568460058062819407, -1.599625672291283607 ) ) ;
#117323=CARTESIAN_POINT ( 'NONE',  ( -6.611092229237963025, 6.760716375176868631, -0.1380881291089108287 ) ) ;
#117334=CARTESIAN_POINT ( 'NONE',  ( -7.944151662964566540, 8.232874793072271657, 0.000000000000000000 ) ) ;
#117339=CARTESIAN_POINT ( 'NONE',  ( -1.792484642137049056, 2.460830816602578075, 2.500000000000000000 ) ) ;
#117356=CARTESIAN_POINT ( 'NONE',  ( -6.645558177068566330, 6.717849059526919575, 0.1763403335921341630 ) ) ;
#117386=CARTESIAN_POINT ( 'NONE',  ( 0.3866926556112008639, 2.897682894409560284, 2.027578619373314073 ) ) ;
#117388=CARTESIAN_POINT ( 'NONE',  ( 4.258142763143749399, 7.125527769379820242, 1.199719254218451159 ) ) ;
#117389=CARTESIAN_POINT ( 'NONE',  ( -3.336715202739028552, 6.906935146588564223, 0.7216878364870338292 ) ) ;
#117414=CARTESIAN_POINT ( 'NONE',  ( -5.875479466675803231, 7.948088359245467416, -1.599625672291271394 ) ) ;
#117417=CIRCLE ( 'NONE', #199922, 0.08000000000000041800 ) ;
#117421=CARTESIAN_POINT ( 'NONE',  ( -2.810282979782591006, 6.500690253046801814, 0.000000000000000000 ) ) ;
#117428=CARTESIAN_POINT ( 'NONE',  ( -5.752402313948099533, 9.933162809573264695, -0.7998128361456362523 ) ) ;
#117436=CARTESIAN_POINT ( 'NONE',  ( 3.770049233051776749, 6.556085317605844232, 1.199719254218451159 ) ) ;
#117441=CARTESIAN_POINT ( 'NONE',  ( 3.947104627881618200, 8.980740528188865923, 0.7749999999999996891 ) ) ;
#117442=CARTESIAN_POINT ( 'NONE',  ( -4.936050443827081580, 7.916420063510339666, 1.199719254218452935 ) ) ;
#117445=CARTESIAN_POINT ( 'NONE',  ( -7.621091744657483069, 8.063897588288083895, 0.7216878364870317197 ) ) ;
#117449=CARTESIAN_POINT ( 'NONE',  ( -6.414416072596837104, 9.537216947121368804, -1.082531754730549967 ) ) ;
#117450=CARTESIAN_POINT ( 'NONE',  ( 4.923019175093585886, 5.876515471431535076, -1.082531754730548412 ) ) ;
#117451=CARTESIAN_POINT ( 'NONE',  ( -3.973948422136970748, 6.690004688251493192, -1.082531754730546636 ) ) ;
#117469=CARTESIAN_POINT ( 'NONE',  ( 6.512538272292041519, 6.827515365185738538, -0.5364851146780359459 ) ) ;
#117490=CARTESIAN_POINT ( 'NONE',  ( 6.423677080210483226, 6.791898735554919853, -0.4454198846488600649 ) ) ;
#117504=CARTESIAN_POINT ( 'NONE',  ( 6.556249800660121529, 9.806652646482286073, 1.199719254218452047 ) ) ;
#117507=CARTESIAN_POINT ( 'NONE',  ( -5.981082042284069367, 7.006959133200059142, 1.199719254218452935 ) ) ;
#117511=CARTESIAN_POINT ( 'NONE',  ( -8.041394506236766659, 8.554250810130591631, -0.7216878364870338292 ) ) ;
#117519=CARTESIAN_POINT ( 'NONE',  ( 5.037736595929563244, 8.035053907629919223, -1.199719254218452047 ) ) ;
#117521=CARTESIAN_POINT ( 'NONE',  ( 6.831329296439236032, 9.063246493969506545, -1.599625672291267398 ) ) ;
#117522=CARTESIAN_POINT ( 'NONE',  ( 6.966220764712121927, 6.002124920821316323, 2.500000000000000444 ) ) ;
#117526=CARTESIAN_POINT ( 'NONE',  ( -7.078765599666485997, 7.431183752465250869, 0.000000000000000000 ) ) ;
#117527=ORIENTED_EDGE ( 'NONE', *, *, #51328, .F. ) ;
#117532=CARTESIAN_POINT ( 'NONE',  ( 6.770317605177710085, 8.992066187497757213, 1.599625672291268286 ) ) ;
#117542=CARTESIAN_POINT ( 'NONE',  ( 5.514321724087592358, 5.998106097858366681, 0.7610078497430600164 ) ) ;
#117546=CARTESIAN_POINT ( 'NONE',  ( -6.834718835064852449, 8.106831741398025315, 1.082531754730549078 ) ) ;
#117547=CARTESIAN_POINT ( 'NONE',  ( 5.180624094197585627, 8.097792972322238825, -1.082531754730548412 ) ) ;
#117549=DIRECTION ( 'NONE',  ( -1.000000000000000000, 0.000000000000000000, 0.000000000000000000 ) ) ;
#117552=VERTEX_POINT ( 'NONE', #17599 ) ;
#117557=CARTESIAN_POINT ( 'NONE',  ( -4.176793841461789114, 7.030620694084159794, -1.199719254218455378 ) ) ;
#117558=CARTESIAN_POINT ( 'NONE',  ( -2.810282979782591006, 6.500690253046801814, 0.000000000000000000 ) ) ;
#117561=CARTESIAN_POINT ( 'NONE',  ( 4.868786560638885597, 7.733982516503781213, 1.082531754730548412 ) ) ;
#117567=CARTESIAN_POINT ( 'NONE',  ( 0.000000000000000000, 8.980740528189222971, 0.000000000000000000 ) ) ;
#117573=CARTESIAN_POINT ( 'NONE',  ( -5.076314662610137418, 7.858265529090583179, 1.124058833742283436 ) ) ;
#117579=CARTESIAN_POINT ( 'NONE',  ( 3.553645660557675612, 6.199651466408984568, -1.082531754730549967 ) ) ;
#117583=CARTESIAN_POINT ( 'NONE',  ( -5.224688093219839402, 7.188831756880171397, -1.599625672291271394 ) ) ;
#117596=CARTESIAN_POINT ( 'NONE',  ( 5.252858170651868441, 5.093032385374103299, -0.7998128361456481317 ) ) ;
#117605=FACE_OUTER_BOUND ( 'NONE', #201402, .T. ) ;
#117636=CARTESIAN_POINT ( 'NONE',  ( 5.017926250833595780, 7.907978821730911712, -1.082531754730548412 ) ) ;
#117642=CARTESIAN_POINT ( 'NONE',  ( 6.685579144870162693, 6.972466221869550118, -0.7216878364870458196 ) ) ;
#117666=CARTESIAN_POINT ( 'NONE',  ( -3.492107083971660586, 6.231819477012331632, 1.199719254218452935 ) ) ;
#117668=CARTESIAN_POINT ( 'NONE',  ( 5.533136087708556694, 5.627949321847663278, 0.000000000000000000 ) ) ;
#117674=CARTESIAN_POINT ( 'NONE',  ( -7.045397100956844127, 8.248660034984974132, -1.199719254218452047 ) ) ;
#117682=CARTESIAN_POINT ( 'NONE',  ( -5.397554552016258889, 7.390509292142662723, 1.443375672974058777 ) ) ;
#117685=CARTESIAN_POINT ( 'NONE',  ( -7.273023059088104425, 7.449891421883056530, 0.000000000000000000 ) ) ;
#117705=CARTESIAN_POINT ( 'NONE',  ( -4.177320726786328819, 5.966903162707725805, -1.443375672974066548 ) ) ;
#117707=CARTESIAN_POINT ( 'NONE',  ( -4.299344108864961989, 6.109263775132799168, -1.443375672974066548 ) ) ;
#117708=CARTESIAN_POINT ( 'NONE',  ( 5.110497557708379546, 4.926945003606695295, -0.7998128361456481317 ) ) ;
#117709=CARTESIAN_POINT ( 'NONE',  ( -5.276058054373441664, 6.184431147304315424, -1.199719254218453823 ) ) ;
#117710=CARTESIAN_POINT ( 'NONE',  ( -6.466312919074983512, 6.508729591867735031, -0.7998128361456362523 ) ) ;
#117735=CARTESIAN_POINT ( 'NONE',  ( -8.093291352714894415, 8.406871097780989288, -0.7998128361456362523 ) ) ;
#117757=CARTESIAN_POINT ( 'NONE',  ( 2.998579151156815392, 6.400053006662376198, -0.4921665831622086817 ) ) ;
#117762=ORIENTED_EDGE ( 'NONE', *, *, #142352, .F. ) ;
#117765=CARTESIAN_POINT ( 'NONE',  ( 4.947799714344386146, 4.737130853015369958, -0.7998128361456481317 ) ) ;
#117778=CARTESIAN_POINT ( 'NONE',  ( 4.666668778386947380, 8.284408874816399759, 0.5204741841226891985 ) ) ;
#117781=CARTESIAN_POINT ( 'NONE',  ( 6.048345925472166762, 10.07050432311064903, 0.7216878364870317197 ) ) ;
#117788=CARTESIAN_POINT ( 'NONE',  ( -6.622231685632140596, 6.690634819517756959, 0.000000000000000000 ) ) ;
#117794=CARTESIAN_POINT ( 'NONE',  ( -4.485769045089750939, 8.247486273217061736, 0.1636802980241918171 ) ) ;
#117799=CARTESIAN_POINT ( 'NONE',  ( 5.804299160426222848, 7.865044668620976509, -1.443375672974078761 ) ) ;
#117802=CARTESIAN_POINT ( 'NONE',  ( -4.553559489343377287, 6.405848385690952718, -1.599625672291271394 ) ) ;
#117815=CARTESIAN_POINT ( 'NONE',  ( 5.903649544107831382, 5.852288987739402870, -0.7998128361456481317 ) ) ;
#117816=CARTESIAN_POINT ( 'NONE',  ( 5.408776937209000657, 5.274937613024121674, 0.7998128361456352531 ) ) ;
#117817=EDGE_LOOP ( 'NONE', ( #10386, #15358, #7743 ) ) ;
#117839=CARTESIAN_POINT ( 'NONE',  ( 7.828907357248368726, 8.098423103070084395, 0.7998128361456281477 ) ) ;
#117847=CARTESIAN_POINT ( 'NONE',  ( 6.717138760927786834, 6.801359740696030443, -0.7998128361456481317 ) ) ;
#117851=CARTESIAN_POINT ( 'NONE',  ( 3.594320121398666856, 7.207474218358159490, -1.734723475976807094E-15 ) ) ;
#117855=CARTESIAN_POINT ( 'NONE',  ( 6.319508997745523438, 9.426492026461511742, -1.082531754730548412 ) ) ;
#117867=CARTESIAN_POINT ( 'NONE',  ( 6.330867959801246059, 6.852818249511213544, -0.6651261847785728820 ) ) ;
#117868=CARTESIAN_POINT ( 'NONE',  ( -5.750066545971566079, 8.762142499391876171, 1.082531754730550855 ) ) ;
#117889=VECTOR ( 'NONE', #2969, 1000.000000000000000 ) ;
#117901=CARTESIAN_POINT ( 'NONE',  ( 7.693325821111733021, 7.940244644243982464, -0.7998128361456341429 ) ) ;
#117903=CARTESIAN_POINT ( 'NONE',  ( 7.198453214212898743, 7.362893269528701268, 0.7998128361456291469 ) ) ;
#117911=SURFACE_STYLE_FILL_AREA ( #182834 ) ;
#117917=CARTESIAN_POINT ( 'NONE',  ( -4.716257332707368910, 6.595662536282280719, -1.599625672291271394 ) ) ;
#117919=CARTESIAN_POINT ( 'NONE',  ( 5.356880090730850696, 9.263794182579101033, 0.7216878364870317197 ) ) ;
#117928=CARTESIAN_POINT ( 'NONE',  ( -3.526002468005825286, 6.271364091718859335, -1.199719254218450271 ) ) ;
#117934=CARTESIAN_POINT ( 'NONE',  ( -6.400857919427531684, 9.521399101757175742, 1.082531754730549967 ) ) ;
#117935=ORIENTED_EDGE ( 'NONE', *, *, #112074, .T. ) ;
#117936=CARTESIAN_POINT ( 'NONE',  ( -6.129694847154222970, 7.284303755502281597, -1.082531754730549967 ) ) ;
#117959=CARTESIAN_POINT ( 'NONE',  ( -3.318713740295064163, 7.093859473644694269, 0.000000000000000000 ) ) ;
#117969=CARTESIAN_POINT ( 'NONE',  ( 0.000000000000000000, 0.000000000000000000, 0.000000000000000000 ) ) ;
#117970=CARTESIAN_POINT ( 'NONE',  ( 2.750651594100012254, 2.940524554645664868, -2.453100423511232808 ) ) ;
#117971=CARTESIAN_POINT ( 'NONE',  ( -5.594533863947632746, 7.496198557292433229, -1.347124935377568722 ) ) ;
#117974=ORIENTED_EDGE ( 'NONE', *, *, #135323, .T. ) ;
#117989=CARTESIAN_POINT ( 'NONE',  ( 5.200434439293556643, 8.224868058221247225, -1.199719254218452047 ) ) ;
#118012=CARTESIAN_POINT ( 'NONE',  ( 6.638652492546827766, 7.774124658506663010, 1.199719254218452047 ) ) ;
#118013=CARTESIAN_POINT ( 'NONE',  ( 6.398522151006641678, 6.429640362454684954, 0.000000000000000000 ) ) ;
#118015=CARTESIAN_POINT ( 'NONE',  ( 4.746236293235721604, 7.694970221153795364, 1.199719254218451159 ) ) ;
#118019=CARTESIAN_POINT ( 'NONE',  ( -5.345849613874695372, 4.689682906365682413, -2.440353602067509176 ) ) ;
#118028=CARTESIAN_POINT ( 'NONE',  ( 4.605689926069578277, 8.476745573306274650, -0.2140288463435610078 ) ) ;
#118030=CARTESIAN_POINT ( 'NONE',  ( -6.427974226210522168, 6.671927150099951298, 0.000000000000000000 ) ) ;
#118031=CARTESIAN_POINT ( 'NONE',  ( 5.560252395380222090, 5.659585014131299552, 0.7216878364870328300 ) ) ;
#118053=CARTESIAN_POINT ( 'NONE',  ( -3.296040741453672318, 6.859481608422314025, 0.7216878364870338292 ) ) ;
#118058=CARTESIAN_POINT ( 'NONE',  ( 4.532168488718122390, 8.509556680138327778, 0.7998128361456271485 ) ) ;
#118076=CARTESIAN_POINT ( 'NONE',  ( -4.333496373511149358, 7.757669579117222547, -0.6939643617286651578 ) ) ;
#118086=CARTESIAN_POINT ( 'NONE',  ( 7.191674137406095291, 7.354984346587396082, 0.000000000000000000 ) ) ;
#118091=CARTESIAN_POINT ( 'NONE',  ( -5.130090819275266334, 7.806487709571898748, 1.156910012491520590 ) ) ;
#118092=CARTESIAN_POINT ( 'NONE',  ( 5.338878628731272613, 9.450718510153643948, -0.7998128361456481317 ) ) ;
#118102=CARTESIAN_POINT ( 'NONE',  ( 1.807185592549606312, 2.518115318451403795, 2.499999999999998668 ) ) ;
#118118=CARTESIAN_POINT ( 'NONE',  ( 4.923019175537949543, 4.916146257648610352, 0.000000000000000000 ) ) ;
#118122=CARTESIAN_POINT ( 'NONE',  ( -7.456058132872594335, 7.663432341298296535, 0.000000000000000000 ) ) ;
#118124=CARTESIAN_POINT ( 'NONE',  ( 5.688527969385528849, 8.794310509995222347, -1.199719254218452047 ) ) ;
#118133=DIRECTION ( 'NONE',  ( 0.7592566023652995710, -0.6507913734559650498, 0.000000000000000000 ) ) ;
#118146=CARTESIAN_POINT ( 'NONE',  ( 6.373214726875630731, 9.593111727067046957, 1.199719254218452047 ) ) ;
#118156=CARTESIAN_POINT ( 'NONE',  ( 2.905190055078214595, 6.611415174225076186, 0.7998128361456271485 ) ) ;
#118168=CARTESIAN_POINT ( 'NONE',  ( -5.316205630334255972, 8.255971431148344308, -1.082531754730549967 ) ) ;
#118171=CARTESIAN_POINT ( 'NONE',  ( 5.875479466675786355, 7.948088359245467416, -1.599625672291283607 ) ) ;
#118176=CARTESIAN_POINT ( 'NONE',  ( -7.587723245503481095, 8.881373870289390737, 1.199719254218452047 ) ) ;
#118188=CARTESIAN_POINT ( 'NONE',  ( -0.4461645575834740640, 3.167858595401910282, -1.950569735685831807 ) ) ;
#118215=CARTESIAN_POINT ( 'NONE',  ( 5.587368702607580673, 5.691220705896524734, -0.7216878364870458196 ) ) ;
#118220=CARTESIAN_POINT ( 'NONE',  ( 5.388439706788500594, 5.251210844200210559, 0.7998128361456352531 ) ) ;
#118223=CARTESIAN_POINT ( 'NONE',  ( -4.125423880308188629, 8.035021303660014880, -0.7998128361456481317 ) ) ;
#118227=CARTESIAN_POINT ( 'NONE',  ( -5.980555156959541208, 7.110307450275150210, 1.082531754730549078 ) ) ;
#118228=ADVANCED_FACE ( 'NONE', ( #42442 ), #53437, .T. ) ;
#118234=CARTESIAN_POINT ( 'NONE',  ( -7.096767062110449942, 7.244259425409119046, -0.7998128361456362523 ) ) ;
#118241=CARTESIAN_POINT ( 'NONE',  ( 3.570880328030153539, 7.341005539872356600, 0.2896471194287209006 ) ) ;
#118244=CARTESIAN_POINT ( 'NONE',  ( -5.336015975430226099, 8.383046517047350932, -1.199719254218453823 ) ) ;
#118246=CARTESIAN_POINT ( 'NONE',  ( 4.597299534708283453, 8.487268731053720927, 0.09294953129799360392 ) ) ;
#118250=LINE ( 'NONE', #128, #212419 ) ;
#118252=CARTESIAN_POINT ( 'NONE',  ( 5.671053392266061977, 9.838255734277600695, 0.7998128361456331437 ) ) ;
#118257=CARTESIAN_POINT ( 'NONE',  ( -5.387385936583832802, 7.378645907471495846, -1.599625672291271394 ) ) ;
#118261=CARTESIAN_POINT ( 'NONE',  ( -4.911796789900812144, 8.952456364851418158, 0.7998128361456291469 ) ) ;
#118266=CARTESIAN_POINT ( 'NONE',  ( -8.068510813464099485, 8.585886501895810596, 0.7216878364870317197 ) ) ;
#118272=CARTESIAN_POINT ( 'NONE',  ( 6.692885107001518286, 7.837396042037102717, -1.199719254218452047 ) ) ;
#118285=CARTESIAN_POINT ( 'NONE',  ( -0.3999999999999003797, 3.087878369845980853, -2.023857702507796397 ) ) ;
#118286=CARTESIAN_POINT ( 'NONE',  ( 6.562153376633583335, 6.794832157118596783, -0.3727171428496069971 ) ) ;
#118293=PLANE ( 'NONE',  #140182 ) ;
#118309=CARTESIAN_POINT ( 'NONE',  ( -4.610264723183647995, 8.173666352459294515, -0.5982188967808210744 ) ) ;
#118310=ORIENTED_EDGE ( 'NONE', *, *, #112082, .T. ) ;
#118314=CARTESIAN_POINT ( 'NONE',  ( -6.419454189569741231, 6.887487763818779918, 0.7628848663763813098 ) ) ;
#118327=B_SPLINE_CURVE_WITH_KNOTS ( 'NONE', 3,
 ( #187423, #4377, #101916, #85660 ),
 .UNSPECIFIED., .F., .F.,
 ( 4, 4 ),
 ( 0.0006956056399114353287, 0.0009226328642097691209 ),
 .UNSPECIFIED. ) ;
#118333=CARTESIAN_POINT ( 'NONE',  ( -4.197131071882288289, 7.054347462908075350, -1.199719254218455378 ) ) ;
#118339=VECTOR ( 'NONE', #189782, 1000.000000000000000 ) ;
#118349=CARTESIAN_POINT ( 'NONE',  ( 4.830447868218803897, 8.857549289555754157, -0.7998128361456481317 ) ) ;
#118350=CARTESIAN_POINT ( 'NONE',  ( 3.627688620108284745, 6.389997935838436227, 1.199719254218452047 ) ) ;
#118352=CARTESIAN_POINT ( 'NONE',  ( 4.841670253411575864, 8.662716039039905169, -0.7216878364870458196 ) ) ;
#118365=CARTESIAN_POINT ( 'NONE',  ( -6.622231685632140596, 6.690634819517756959, 0.000000000000000000 ) ) ;
#118366=ADVANCED_FACE ( 'NONE', ( #92268 ), #146857, .T. ) ;
#118367=CARTESIAN_POINT ( 'NONE',  ( 6.229045230835819069, 6.231917288922055320, -0.7998128361456481317 ) ) ;
#118375=CARTESIAN_POINT ( 'NONE',  ( -5.178288325776719603, 5.006034233019745372, 0.000000000000000000 ) ) ;
#118376=CARTESIAN_POINT ( 'NONE',  ( 5.833751235630055376, 10.02806988486892514, 0.7998128361456331437 ) ) ;
#118384=CARTESIAN_POINT ( 'NONE',  ( 4.227110032410640095, 8.153655147779589996, 0.7998128361456271485 ) ) ;
#118390=CARTESIAN_POINT ( 'NONE',  ( -5.569768141569340969, 7.516503378918355516, 1.348759926630802131 ) ) ;
#118397=CARTESIAN_POINT ( 'NONE',  ( 2.886471042457359637, 6.589576326167374098, -0.3044456787500351980 ) ) ;
#118402=CARTESIAN_POINT ( 'NONE',  ( -5.908321080505254841, 10.11506803722328129, 0.7998128361456291469 ) ) ;
#118410=B_SPLINE_CURVE_WITH_KNOTS ( 'NONE', 3,
 ( #138219, #58018, #88394, #91619, #125241, #55884, #154461, #9267, #56956, #6039 ),
 .UNSPECIFIED., .F., .F.,
 ( 4, 3, 3, 4 ),
 ( 0.000000000000000000, 3.125302649357442460E-05, 8.414501133366901735E-05, 0.0001371975721651944632 ),
 .UNSPECIFIED. ) ;
#118413=CARTESIAN_POINT ( 'NONE',  ( 3.119784744920330422, 6.653849612466795627, 0.7216878364870257245 ) ) ;
#118434=CARTESIAN_POINT ( 'NONE',  ( 6.235824307642648279, 6.239826211863360506, 0.000000000000000000 ) ) ;
#118453=CARTESIAN_POINT ( 'NONE',  ( -0.2822871844487425119, 3.300644403538278038, 1.982554686319321302 ) ) ;
#118456=CARTESIAN_POINT ( 'NONE',  ( 5.876533236880477240, 5.820653295974182129, 0.7998128361456352531 ) ) ;
#118457=CARTESIAN_POINT ( 'NONE',  ( -4.014622883422322985, 7.697827440719083647, -0.7216878364870458196 ) ) ;
#118480=ORIENTED_EDGE ( 'NONE', *, *, #191207, .F. ) ;
#118481=CARTESIAN_POINT ( 'NONE',  ( -6.363572996767778100, 8.517530811019446091, -1.599625672291271394 ) ) ;
#118489=CARTESIAN_POINT ( 'NONE',  ( -3.902768115887413014, 5.646591783325653147, -1.599625672291283607 ) ) ;
#118492=CARTESIAN_POINT ( 'NONE',  ( 2.970157261343746580, 6.585292010301047938, 0.4235207732182846851 ) ) ;
#118497=CARTESIAN_POINT ( 'NONE',  ( -7.273023059088104425, 7.449891421883056530, 0.000000000000000000 ) ) ;
#118504=CARTESIAN_POINT ( 'NONE',  ( 4.740510986633625024, 5.559626234941203116, -1.199719254218450271 ) ) ;
#118508=CARTESIAN_POINT ( 'NONE',  ( -4.450819567036169211, 8.414649604842665553, -0.7998128361456362523 ) ) ;
#118511=CARTESIAN_POINT ( 'NONE',  ( -5.953438850176548947, 9.959779401932374654, 0.000000000000000000 ) ) ;
#118515=CARTESIAN_POINT ( 'NONE',  ( 5.370438244344566847, 5.438135171256338829, 0.000000000000000000 ) ) ;
#118516=CARTESIAN_POINT ( 'NONE',  ( -5.465345319640241506, 5.548860092434608760, 0.7216878364870257245 ) ) ;
#118534=CARTESIAN_POINT ( 'NONE',  ( 6.328358748234019338, 6.951510624437585939, -0.8854765018257749754 ) ) ;
#118555=CARTESIAN_POINT ( 'NONE',  ( 6.119462805442048570, 6.996221746119736018, -0.9567421715909133484 ) ) ;
#118569=CARTESIAN_POINT ( 'NONE',  ( 6.393551957296131683, 9.616838495890963401, 1.199719254218452047 ) ) ;
#118572=CARTESIAN_POINT ( 'NONE',  ( -4.620296487206990932, 8.612372678375294299, 0.000000000000000000 ) ) ;
#118582=CARTESIAN_POINT ( 'NONE',  ( 6.412080304620304538, 6.445458208337293549, -0.7998128361456481317 ) ) ;
#118589=CYLINDRICAL_SURFACE ( 'NONE', #29910, 0.4000000000000001332 ) ;
#118590=CARTESIAN_POINT ( 'NONE',  ( -5.261973015435229328, 9.153069261400824885, 0.000000000000000000 ) ) ;
#118595=CARTESIAN_POINT ( 'NONE',  ( 3.512971199272317602, 6.152197928242737923, -1.082531754730549967 ) ) ;
#118602=CARTESIAN_POINT ( 'NONE',  ( 1.855128211190495202, 8.960462962215050453, 0.7750000000000004663 ) ) ;
#118606=ORIENTED_EDGE ( 'NONE', *, *, #167207, .F. ) ;
#118609=CARTESIAN_POINT ( 'NONE',  ( -6.780486220610195680, 7.083191143566240910, -0.7216878364870338292 ) ) ;
#118611=CARTESIAN_POINT ( 'NONE',  ( 5.641601317062233001, 7.675230518029648508, -1.443375672974078761 ) ) ;
#118613=FACE_OUTER_BOUND ( 'NONE', #177859, .T. ) ;
#118617=EDGE_LOOP ( 'NONE', ( #97503, #95022, #191894, #42905 ) ) ;
#118622=CARTESIAN_POINT ( 'NONE',  ( -5.659602779061863487, 5.567567761852417085, 0.7998128361456281477 ) ) ;
#118623=CARTESIAN_POINT ( 'NONE',  ( -4.496464221587651799, 5.274905009054215554, 1.199719254218452935 ) ) ;
#118626=CARTESIAN_POINT ( 'NONE',  ( 5.004368096775565711, 8.852530189631227842, -0.7216878364870458196 ) ) ;
#118629=B_SPLINE_CURVE_WITH_KNOTS ( 'NONE', 3,
 ( #149195, #165440, #82051, #34369, #198982, #83114 ),
 .UNSPECIFIED., .F., .F.,
 ( 4, 2, 4 ),
 ( 0.000000000000000000, 0.002406312826513422667, 0.004812625653026847070 ),
 .UNSPECIFIED. ) ;
#118640=CARTESIAN_POINT ( 'NONE',  ( -4.752344554418619360, 8.202642464201909789, 0.7248784622895955154 ) ) ;
#118645=CARTESIAN_POINT ( 'NONE',  ( 4.421367491832282504, 5.291255174293369556, 1.082531754730549078 ) ) ;
#118648=CARTESIAN_POINT ( 'NONE',  ( -5.631432701629818460, 7.663367133358481631, 1.599625672291263179 ) ) ;
#118662=CARTESIAN_POINT ( 'NONE',  ( 5.564695703766185275, 5.456842840674144490, 0.000000000000000000 ) ) ;
#118669=DIRECTION ( 'NONE',  ( 0.7592566023653005702, -0.6507913734559639396, 0.000000000000000000 ) ) ;
#118696=CARTESIAN_POINT ( 'NONE',  ( 5.478903473698239601, 7.485416367438324059, -1.443375672974078761 ) ) ;
#118701=CARTESIAN_POINT ( 'NONE',  ( 4.678972410047582464, 8.472901888448573615, -0.7216878364870357165 ) ) ;
#118713=CARTESIAN_POINT ( 'NONE',  ( -5.596483547390937119, 9.751257581923240991, 0.000000000000000000 ) ) ;
#118725=CARTESIAN_POINT ( 'NONE',  ( 3.377389663135653031, 6.954388683717978026, -0.7216878364870338292 ) ) ;
#118732=CARTESIAN_POINT ( 'NONE',  ( -7.598418745816086783, 7.829519723065708092, 0.000000000000000000 ) ) ;
#118737=CARTESIAN_POINT ( 'NONE',  ( -5.587368702607575344, 8.572328348800551723, 1.082531754730550855 ) ) ;
#118740=CARTESIAN_POINT ( 'NONE',  ( -7.422162748838431412, 7.623887726591770608, -0.7998128361456362523 ) ) ;
#118759=CARTESIAN_POINT ( 'NONE',  ( -5.180624094197616714, 5.216685329418210948, 0.7216878364870257245 ) ) ;
#118760=VERTEX_POINT ( 'NONE', #29371 ) ;
#118761=CARTESIAN_POINT ( 'NONE',  ( -3.973948422136968084, 7.650373902552835226, -0.7216878364870458196 ) ) ;
#118763=CARTESIAN_POINT ( 'NONE',  ( 5.061990249855835344, 6.999017606288844284, -1.599625672291273171 ) ) ;
#118764=CARTESIAN_POINT ( 'NONE',  ( -6.140917232347002042, 6.129101290685087911, -0.7998128361456362523 ) ) ;
#118765=CARTESIAN_POINT ( 'NONE',  ( -7.618755976236585958, 7.853246491889623648, 0.000000000000000000 ) ) ;
#118781=CARTESIAN_POINT ( 'NONE',  ( 4.796824973295459316, 8.251456047330133714, 0.8599625132450954279 ) ) ;
#118802=EDGE_CURVE ( 'NONE', #56229, #45216, #208570, .T. ) ;
#118819=CARTESIAN_POINT ( 'NONE',  ( 4.167152111353856547, 5.955039778036558040, 1.599625672291262513 ) ) ;
#118833=CARTESIAN_POINT ( 'NONE',  ( 4.635702676548680401, 8.322458603728597026, -0.3981331281527732968 ) ) ;
#118836=CARTESIAN_POINT ( 'NONE',  ( 3.542423274920540432, 7.354853930707762721, -1.734723475976807094E-15 ) ) ;
#118846=CARTESIAN_POINT ( 'NONE',  ( -5.912237504011027767, 9.055304967058290799, 1.199719254218454489 ) ) ;
#118851=DIRECTION ( 'NONE',  ( 0.000000000000000000, 1.000000000000000000, 0.000000000000000000 ) ) ;
#118858=CARTESIAN_POINT ( 'NONE',  ( 5.058600711674583472, 8.915801573680086634, 0.000000000000000000 ) ) ;
#118862=CARTESIAN_POINT ( 'NONE',  ( -4.776215253764153346, 8.794277906025310898, -0.7998128361456362523 ) ) ;
#118869=VERTEX_POINT ( 'NONE', #88785 ) ;
#118873=CARTESIAN_POINT ( 'NONE',  ( 3.691562964670865199, 7.528850235416478576, -0.7998128361456362523 ) ) ;
#118874=CARTESIAN_POINT ( 'NONE',  ( 6.710359684120930091, 6.793450817754725257, 0.7998128361456352531 ) ) ;
#118887=ORIENTED_EDGE ( 'NONE', *, *, #68041, .F. ) ;
#118895=CARTESIAN_POINT ( 'NONE',  ( -5.587017333170084754, 5.816630895727369577, 0.4567169512200538461 ) ) ;
#118896=CARTESIAN_POINT ( 'NONE',  ( 5.253852870291571442, 7.792406146126436006, -1.285611862062207011 ) ) ;
#118900=CARTESIAN_POINT ( 'NONE',  ( 3.791513125430877373, 7.352524219418101303, -0.3677586026353037996 ) ) ;
#118904=CARTESIAN_POINT ( 'NONE',  ( 3.061108821635398769, 6.793320401875094561, -0.7998128361456362523 ) ) ;
#118910=CARTESIAN_POINT ( 'NONE',  ( 5.332099551924443404, 9.442809587212341427, 0.000000000000000000 ) ) ;
#118917=CARTESIAN_POINT ( 'NONE',  ( 4.245111494854632461, 7.966730820723463502, 0.000000000000000000 ) ) ;
#118921=CARTESIAN_POINT ( 'NONE',  ( 3.553118775233146120, 6.302999783484076524, -1.199719254218453823 ) ) ;
#118933=CARTESIAN_POINT ( 'NONE',  ( 6.373787108001086388, 6.824503602047865769, -0.5760177672454840359 ) ) ;
#118934=CARTESIAN_POINT ( 'NONE',  ( -5.478903473698247595, 8.445785581739666981, -1.082531754730549967 ) ) ;
#118941=CARTESIAN_POINT ( 'NONE',  ( -5.561176828107109671, 5.894252131381872317, 0.6462735908731042089 ) ) ;
#118967=CARTESIAN_POINT ( 'NONE',  ( 5.494797395288433250, 9.632623737803665875, 0.000000000000000000 ) ) ;
#118969=CARTESIAN_POINT ( 'NONE',  ( 7.225569521440261767, 7.394528961293920233, -0.7998128361456341429 ) ) ;
#118982=CARTESIAN_POINT ( 'NONE',  ( -5.635349125135588721, 6.603604063193491136, 1.199719254218452935 ) ) ;
#118984=CARTESIAN_POINT ( 'NONE',  ( 6.875393295461478260, 8.154285278527437342, -1.082531754730548412 ) ) ;
#118994=CARTESIAN_POINT ( 'NONE',  ( -5.157951095356222204, 4.982307464195829816, 0.000000000000000000 ) ) ;
#118998=CARTESIAN_POINT ( 'NONE',  ( -3.469446951953614189E-15, 8.999999999999998224, -2.420000000000000373 ) ) ;
#119002=CARTESIAN_POINT ( 'NONE',  ( -5.804299160426224624, 9.785783097223662352, -0.7216878364870338292 ) ) ;
#119004=CARTESIAN_POINT ( 'NONE',  ( -5.885648082108231982, 7.959951743916638733, 1.443375672974058777 ) ) ;
#119026=CARTESIAN_POINT ( 'NONE',  ( -5.438755897737433287, 6.374245297895642537, -1.199719254218453823 ) ) ;
#119035=CARTESIAN_POINT ( 'NONE',  ( -4.638114411034067963, 8.432649648999159808, -0.4721908680582111995 ) ) ;
#119058=CARTESIAN_POINT ( 'NONE',  ( -1.806654366501805775, 0.000000000000000000, 2.500000000000000444 ) ) ;
#119059=CARTESIAN_POINT ( 'NONE',  ( 1.858560999665780145, 8.965769984707671725, -0.7749999999999996891 ) ) ;
#119069=CARTESIAN_POINT ( 'NONE',  ( 5.761288931164342486, 5.686201605971993978, -0.7998128361456481317 ) ) ;
#119077=CARTESIAN_POINT ( 'NONE',  ( 6.086684617892325733, 6.065829907154645539, -0.7998128361456481317 ) ) ;
#119079=CARTESIAN_POINT ( 'NONE',  ( 5.662465432362883355, 6.635239754958710989, 1.199719254218451159 ) ) ;
#119081=( BOUNDED_CURVE ( )  B_SPLINE_CURVE ( 2, ( #23032, #40393, #106497, #92364, #5703, #172524, #58760 ),
 .UNSPECIFIED., .F., .T. ) 
 B_SPLINE_CURVE_WITH_KNOTS ( ( 3, 2, 2, 3 ),
 ( 0.4750000000000001998, 0.4833333333333335036, 0.4916666666666666963, 0.5000000000000000000 ),
 .UNSPECIFIED. ) 
 CURVE ( )  GEOMETRIC_REPRESENTATION_ITEM ( )  RATIONAL_B_SPLINE_CURVE ( ( 0.9999999999999964473, 0.8660254037844422603, 1.000000000000000000, 0.8660254037844387076, 1.000000000000000000, 0.8660254037844387076, 1.000000000000000000 ) ) 
 REPRESENTATION_ITEM ( '' )  );
#119093=CARTESIAN_POINT ( 'NONE',  ( 5.061762083669725243, 7.855803969722688684, -1.119403510469544782 ) ) ;
#119095=CARTESIAN_POINT ( 'NONE',  ( -6.305950843687521790, 7.489935751457798219, 1.082531754730548412 ) ) ;
#119096=CARTESIAN_POINT ( 'NONE',  ( 5.899206235721897507, 6.055031161196562373, 0.000000000000000000 ) ) ;
#119113=CARTESIAN_POINT ( 'NONE',  ( -5.655159470231558849, 6.730679149092498648, 1.082531754730549078 ) ) ;
#119119=CARTESIAN_POINT ( 'NONE',  ( 5.020262018810099924, 9.078999131912302900, 0.7998128361456331437 ) ) ;
#119147=CARTESIAN_POINT ( 'NONE',  ( 5.833751235630055376, 10.02806988486892514, 0.7998128361456331437 ) ) ;
#119175=CARTESIAN_POINT ( 'NONE',  ( 5.072158865288245444, 5.090142562357324429, 0.7216878364870338292 ) ) ;
#119182=CARTESIAN_POINT ( 'NONE',  ( 7.862802741282558294, 8.137967717776607657, 0.000000000000000000 ) ) ;
#119190=ORIENTED_EDGE ( 'NONE', *, *, #162356, .F. ) ;
#119205=CARTESIAN_POINT ( 'NONE',  ( 5.332099551924443404, 9.442809587212341427, 0.000000000000000000 ) ) ;
#119208=ADVANCED_FACE ( 'NONE', ( #106139 ), #25885, .T. ) ;
#119217=CARTESIAN_POINT ( 'NONE',  ( 7.024532985656136930, 8.328281583754568729, 1.082531754730549967 ) ) ;
#119230=CARTESIAN_POINT ( 'NONE',  ( -5.885648082108231982, 7.959951743916638733, 1.443375672974058777 ) ) ;
#119233=CARTESIAN_POINT ( 'NONE',  ( 7.849244587668864348, 8.122149871893999062, 0.7998128361456291469 ) ) ;
#119238=CARTESIAN_POINT ( 'NONE',  ( -3.467853430045390706, 7.267855778353407459, 0.7998128361456352531 ) ) ;
#119239=CARTESIAN_POINT ( 'NONE',  ( -5.398914348987512213, 6.259949555863199677, 2.500000000000001332 ) ) ;
#119240=CARTESIAN_POINT ( 'NONE',  ( 3.973272364828547509, 7.311925558592853314, -0.9262215144194854144 ) ) ;
#119248=ORIENTED_EDGE ( 'NONE', *, *, #151435, .F. ) ;
#119251=CARTESIAN_POINT ( 'NONE',  ( 7.065207446497155708, 9.336104335703744539, 0.000000000000000000 ) ) ;
#119253=FACE_OUTER_BOUND ( 'NONE', #45202, .T. ) ;
#119283=CARTESIAN_POINT ( 'NONE',  ( -4.620296487206990932, 8.612372678375294299, 0.000000000000000000 ) ) ;
#119287=CARTESIAN_POINT ( 'NONE',  ( -4.664887371553763096, 7.600063145858131364, -1.199719254218453823 ) ) ;
#119288=CARTESIAN_POINT ( 'NONE',  ( -5.601453741101424022, 6.564059448486966986, -1.199719254218453823 ) ) ;
#119290=ORIENTED_EDGE ( 'NONE', *, *, #194283, .F. ) ;
#119291=CARTESIAN_POINT ( 'NONE',  ( -6.441532379824190357, 6.687744995982559892, 0.7216878364870257245 ) ) ;
#119297=CARTESIAN_POINT ( 'NONE',  ( -5.399890319992785237, 9.521898816625391504, 0.7998128361456291469 ) ) ;
#119303=CARTESIAN_POINT ( 'NONE',  ( 4.760479229700392168, 4.886233537081844602, -0.7782378322892316014 ) ) ;
#119304=CARTESIAN_POINT ( 'NONE',  ( -1.883777847254928028, 2.479999999999988880, 2.461990205983016100 ) ) ;
#119305=CARTESIAN_POINT ( 'NONE',  ( -6.252245114557387851, 7.323316050852266557, -1.199719254218453823 ) ) ;
#119307=CARTESIAN_POINT ( 'NONE',  ( 4.978670620768666844, 8.057607364700732688, 1.103355461389814662 ) ) ;
#119312=CARTESIAN_POINT ( 'NONE',  ( 5.494797395288433250, 9.632623737803665875, 0.000000000000000000 ) ) ;
#119326=CARTESIAN_POINT ( 'NONE',  ( -6.912678218121246942, 9.158153569265168770, 1.599625672291269396 ) ) ;
#119329=CARTESIAN_POINT ( 'NONE',  ( 3.947104627881218963, 8.980740528189222971, -0.7749999999999996891 ) ) ;
#119339=CARTESIAN_POINT ( 'NONE',  ( 6.204791576909545192, 7.267953590263130259, -1.199719254218452047 ) ) ;
#119352=CARTESIAN_POINT ( 'NONE',  ( -0.2646952133101811433, 3.312294480054168933, -2.056620194547992053 ) ) ;
#119353=CARTESIAN_POINT ( 'NONE',  ( 5.396826230253299883, 7.665096674459883630, -1.326205021280580265 ) ) ;
#119376=CARTESIAN_POINT ( 'NONE',  ( -4.543700865150305468, 8.221430542475131276, -0.3925545784149546691 ) ) ;
#119382=CARTESIAN_POINT ( 'NONE',  ( -6.292453103784333202, 6.974073686386621951, 0.9489479220791104952 ) ) ;
#119400=CARTESIAN_POINT ( 'NONE',  ( -5.143339171537843590, 7.093924681584509173, 1.599625672291263179 ) ) ;
#119411=ORIENTED_EDGE ( 'NONE', *, *, #115651, .T. ) ;
#119418=FACE_OUTER_BOUND ( 'NONE', #190510, .T. ) ;
#119426=CARTESIAN_POINT ( 'NONE',  ( 5.750066545971570520, 5.881034856487848295, -0.7216878364870458196 ) ) ;
#119430=CARTESIAN_POINT ( 'NONE',  ( 5.356880090730862243, 7.343055753976412525, 1.443375672974064550 ) ) ;
#119434=CARTESIAN_POINT ( 'NONE',  ( -5.936491157937300756, 8.019268665717216749, 1.599625672291263179 ) ) ;
#119436=CARTESIAN_POINT ( 'NONE',  ( 6.042093733545556233, 7.078139439671806699, -1.199719254218452047 ) ) ;
#119444=CARTESIAN_POINT ( 'NONE',  ( -5.015590482412729756, 4.816220082428420923, 0.000000000000000000 ) ) ;
#119445=CARTESIAN_POINT ( 'NONE',  ( 8.154303043976348420, 8.478051404252736845, 0.7998128361456281477 ) ) ;
#119453=CARTESIAN_POINT ( 'NONE',  ( 7.713663051532233972, 7.963971413067895355, -0.7998128361456341429 ) ) ;
#119458=CARTESIAN_POINT ( 'NONE',  ( -5.638125304375204649, 7.460809226315815224, 1.342380602066863160 ) ) ;
#119468=CARTESIAN_POINT ( 'NONE',  ( -5.438229012412911345, 5.517224400669388018, -0.7216878364870338292 ) ) ;
#119479=CARTESIAN_POINT ( 'NONE',  ( 5.072158865288243668, 6.050511776658669127, 1.082531754730549078 ) ) ;
#119483=CARTESIAN_POINT ( 'NONE',  ( -4.990283058281743678, 7.979691447040783814, -1.199719254218453823 ) ) ;
#119485=ORIENTED_EDGE ( 'NONE', *, *, #23022, .F. ) ;
#119493=CARTESIAN_POINT ( 'NONE',  ( 4.121797130385867369, 7.239738145266779945, 1.078207043259531872 ) ) ;
#119495=CARTESIAN_POINT ( 'NONE',  ( 5.408776937209000657, 5.274937613024121674, 0.7998128361456352531 ) ) ;
#119499=CARTESIAN_POINT ( 'NONE',  ( 6.073126464278658432, 6.050012061272033392, 0.000000000000000000 ) ) ;
#119521=CARTESIAN_POINT ( 'NONE',  ( 5.662465432362883355, 6.635239754958710989, 1.199719254218451159 ) ) ;
#119522=CARTESIAN_POINT ( 'NONE',  ( -5.804299160426249493, 5.944306240018289778, -0.7216878364870338292 ) ) ;
#119547=CARTESIAN_POINT ( 'NONE',  ( -7.618755976236585958, 7.853246491889623648, 0.000000000000000000 ) ) ;
#119553=CARTESIAN_POINT ( 'NONE',  ( -2.959422669532919326, 6.674686557755516780, 0.7998128361456352531 ) ) ;
#119561=CARTESIAN_POINT ( 'NONE',  ( -5.088052786878465739, 9.158088361325352977, 0.000000000000000000 ) ) ;
#119563=CARTESIAN_POINT ( 'NONE',  ( 4.960800185296459830, 8.075801985472857325, -1.085925974634168290 ) ) ;
#119571=ADVANCED_FACE ( 'NONE', ( #207835 ), #60523, .F. ) ;
#119574=CARTESIAN_POINT ( 'NONE',  ( -5.803772275101700906, 8.928762199997411386, -1.199719254218452047 ) ) ;
#119579=CARTESIAN_POINT ( 'NONE',  ( -3.471769853551161411, 6.208092708188416076, 1.199719254218452935 ) ) ;
#119582=CARTESIAN_POINT ( 'NONE',  ( -7.607533590599451223, 9.008448956188397361, 1.082531754730549078 ) ) ;
#119583=CARTESIAN_POINT ( 'NONE',  ( 5.194182247366878613, 6.192872389083746043, 1.082531754730549078 ) ) ;
#119585=CARTESIAN_POINT ( 'NONE',  ( -5.004368096775595021, 5.971422546727199077, 1.082531754730549078 ) ) ;
#119590=CARTESIAN_POINT ( 'NONE',  ( -3.786470039966538970, 7.639575156594750283, 0.000000000000000000 ) ) ;
#119603=CARTESIAN_POINT ( 'NONE',  ( -1.833504494307588661, 2.521637134586328877, -2.499652564413211042 ) ) ;
#119604=CARTESIAN_POINT ( 'NONE',  ( 6.592372495380235620, 6.775069446727209233, 0.2122460957004346782 ) ) ;
#119607=CARTESIAN_POINT ( 'NONE',  ( 3.125598124496329360E-16, 2.519999999999999130, 2.000000000000000000 ) ) ;
#119613=CARTESIAN_POINT ( 'NONE',  ( 5.203297092594585393, 9.292540051327542017, 0.7998128361456341429 ) ) ;
#119624=CARTESIAN_POINT ( 'NONE',  ( 6.174897528274166270, 6.957956273452501783, 0.8961316764096085574 ) ) ;
#119642=CARTESIAN_POINT ( 'NONE',  ( -6.805266759416629618, 6.904175738932996964, 0.000000000000000000 ) ) ;
#119653=CARTESIAN_POINT ( 'NONE',  ( 4.712340909201580885, 7.655425606447271214, -1.199719254218452047 ) ) ;
#119659=FACE_OUTER_BOUND ( 'NONE', #154331, .T. ) ;
#119660=CARTESIAN_POINT ( 'NONE',  ( -7.390603132780795725, 8.755363422066633206, -1.082531754730549967 ) ) ;
#119664=CARTESIAN_POINT ( 'NONE',  ( 4.001064729364292916, 6.721640380016713934, -1.082531754730548412 ) ) ;
#119679=CARTESIAN_POINT ( 'NONE',  ( -7.268579750702160780, 8.613002809641560731, -1.082531754730549967 ) ) ;
#119680=CARTESIAN_POINT ( 'NONE',  ( 6.875393295905841917, 7.193916064744513506, 0.000000000000000000 ) ) ;
#119688=CARTESIAN_POINT ( 'NONE',  ( -5.000000000000013323, 8.499999999999996447, 0.7750000000000004663 ) ) ;
#119691=ORIENTED_EDGE ( 'NONE', *, *, #148050, .F. ) ;
#119692=CARTESIAN_POINT ( 'NONE',  ( -5.147255595043616516, 6.034161611419515125, 1.199719254218452935 ) ) ;
#119693=CARTESIAN_POINT ( 'NONE',  ( -4.146814880933400005, 5.931313009212638931, 1.599625672291270506 ) ) ;
#119696=CARTESIAN_POINT ( 'NONE',  ( 5.329763783503544516, 9.232158490813878515, -0.7216878364870458196 ) ) ;
#119701=CARTESIAN_POINT ( 'NONE',  ( -5.634755928360857702, 5.776502004022960435, -0.2774256996143938947 ) ) ;
#119704=CARTESIAN_POINT ( 'NONE',  ( -5.431221679128885427, 7.631776636990481144, 1.349246548148795632 ) ) ;
#119708=VECTOR ( 'NONE', #180086, 1000.000000000000000 ) ;
#119709=CARTESIAN_POINT ( 'NONE',  ( -4.907053429147543611, 8.030730943182621928, 0.9696864716568325271 ) ) ;
#119717=CARTESIAN_POINT ( 'NONE',  ( -4.132202957115018727, 8.042930226601317401, 0.000000000000000000 ) ) ;
#119731=CARTESIAN_POINT ( 'NONE',  ( 5.499767588998890844, 6.445425604367387429, 1.199719254218451159 ) ) ;
#119766=CARTESIAN_POINT ( 'NONE',  ( 5.641601317062233001, 7.675230518029648508, -1.443375672974078761 ) ) ;
#119771=CARTESIAN_POINT ( 'NONE',  ( 5.180624093753221970, 9.058162186105164437, 0.000000000000000000 ) ) ;
#119785=CARTESIAN_POINT ( 'NONE',  ( -7.456058132872594335, 7.663432341298296535, 0.000000000000000000 ) ) ;
#119798=CARTESIAN_POINT ( 'NONE',  ( 3.838366886000300404, 6.531826229425389485, -1.082531754730548412 ) ) ;
#119804=CARTESIAN_POINT ( 'NONE',  ( -3.709037541790315640, 6.484905011134099340, -1.199719254218450271 ) ) ;
#119809=CARTESIAN_POINT ( 'NONE',  ( -5.614485009834902840, 9.564333254867113610, 0.7216878364870267237 ) ) ;
#119812=CARTESIAN_POINT ( 'NONE',  ( -6.400331034103001748, 9.624747418832267698, 1.199719254218452935 ) ) ;
#119817=CARTESIAN_POINT ( 'NONE',  ( -4.659162064951642535, 5.464719159645540003, 1.199719254218452935 ) ) ;
#119834=CARTESIAN_POINT ( 'NONE',  ( -3.363831509966360489, 6.938570838353784076, -0.7216878364870458196 ) ) ;
#119836=CARTESIAN_POINT ( 'NONE',  ( -4.868786560638931782, 6.773613302202437403, 1.443375672974058777 ) ) ;
#119837=CARTESIAN_POINT ( 'NONE',  ( 4.980641328173811999, 6.904110530993182948, 1.599625672291269396 ) ) ;
#119839=CARTESIAN_POINT ( 'NONE',  ( -4.145761110728687804, 8.058748072483927771, -0.7998128361456481317 ) ) ;
#119840=CARTESIAN_POINT ( 'NONE',  ( -7.279802135894939852, 7.457800344824362604, -0.7998128361456362523 ) ) ;
#119848=ORIENTED_EDGE ( 'NONE', *, *, #182569, .F. ) ;
#119889=CARTESIAN_POINT ( 'NONE',  ( -4.994822026498660250, 4.892179926465111350, 0.1397116456474693513 ) ) ;
#119899=CARTESIAN_POINT ( 'NONE',  ( 4.441177836928239309, 7.339068688795062911, 1.199719254218452047 ) ) ;
#119915=CARTESIAN_POINT ( 'NONE',  ( 6.201928923608456046, 6.200281597156833691, 0.7998128361456352531 ) ) ;
#119921=CARTESIAN_POINT ( 'NONE',  ( -7.259464905474441565, 7.434073576000447048, -0.7998128361456362523 ) ) ;
#119925=EDGE_LOOP ( 'NONE', ( #80712, #86307, #129156, #75459, #43259, #107429, #188065 ) ) ;
#119932=CARTESIAN_POINT ( 'NONE',  ( 5.858531774436539052, 6.007577623030311287, 0.000000000000000000 ) ) ;
#119936=CARTESIAN_POINT ( 'NONE',  ( 5.045042558060919724, 8.899983727797476263, -0.7216878364870458196 ) ) ;
#119939=CARTESIAN_POINT ( 'NONE',  ( -4.261005416444848315, 8.193199762486115034, 0.7998128361456352531 ) ) ;
#119950=CARTESIAN_POINT ( 'NONE',  ( 3.528865121306874464, 7.339036084825155015, -0.7998128361456362523 ) ) ;
#119951=CARTESIAN_POINT ( 'NONE',  ( 5.037736595929563244, 8.035053907629919223, -1.199719254218452047 ) ) ;
#119971=CARTESIAN_POINT ( 'NONE',  ( 5.845834525830363226, 7.300097092180095615, -1.274846751706928849 ) ) ;
#119982=CARTESIAN_POINT ( 'NONE',  ( 3.074666975249065626, 6.809138247757705820, 0.000000000000000000 ) ) ;
#119986=CARTESIAN_POINT ( 'NONE',  ( 6.017840079619279692, 8.114175741012878973, -1.599625672291281386 ) ) ;
#119991=CARTESIAN_POINT ( 'NONE',  ( 5.451787166470912993, 6.493411461371761284, -1.082531754730548412 ) ) ;
#119994=CARTESIAN_POINT ( 'NONE',  ( 2.878073747850912412, 6.579779482459851003, -0.7998128361456362523 ) ) ;
#120006=CARTESIAN_POINT ( 'NONE',  ( 6.484283628081795037, 6.752753718119230975, 0.1579380340677779548 ) ) ;
#120007=CARTESIAN_POINT ( 'NONE',  ( -5.157951095356222204, 4.982307464195829816, 0.000000000000000000 ) ) ;
#120023=LINE ( 'NONE', #37633, #117889 ) ;
#120042=CARTESIAN_POINT ( 'NONE',  ( 7.191674137406095291, 7.354984346587396082, 0.000000000000000000 ) ) ;
#120044=CARTESIAN_POINT ( 'NONE',  ( 7.309781096423290769, 8.557108029695882578, 1.199719254218452935 ) ) ;
#120050=AXIS2_PLACEMENT_3D ( 'NONE', #76290, #145611, #44889 ) ;
#120052=SURFACE_SIDE_STYLE ('',( #117911 ) ) ;
#120059=CARTESIAN_POINT ( 'NONE',  ( -5.957882158562513908, 5.915560371269843465, -0.7998128361456362523 ) ) ;
#120061=CARTESIAN_POINT ( 'NONE',  ( 5.194182247366861738, 9.073980031987776584, 0.7216878364870317197 ) ) ;
#120071=CARTESIAN_POINT ( 'NONE',  ( -4.659162064951642535, 5.464719159645540003, 1.199719254218452935 ) ) ;
#120074=CARTESIAN_POINT ( 'NONE',  ( -4.177320726786328819, 5.966903162707725805, -1.443375672974066548 ) ) ;
#120078=CARTESIAN_POINT ( 'NONE',  ( -3.984117037569407938, 5.741498858621315371, 1.599625672291270506 ) ) ;
#120079=ORIENTED_EDGE ( 'NONE', *, *, #78821, .T. ) ;
#120080=CARTESIAN_POINT ( 'NONE',  ( -5.153507786970267013, 8.066157280557016307, -1.082531754730549967 ) ) ;
#120089=CARTESIAN_POINT ( 'NONE',  ( 0.3999999999999758193, 3.000000000000047518, 2.023857702507768419 ) ) ;
#120102=CARTESIAN_POINT ( 'NONE',  ( -4.522526758610270647, 7.433975764090723359, -1.199719254218453823 ) ) ;
#120105=CARTESIAN_POINT ( 'NONE',  ( -3.654804927335652209, 6.421633627603656080, 1.199719254218452935 ) ) ;
#120113=CARTESIAN_POINT ( 'NONE',  ( -6.555587544261016753, 6.796970737185429989, -0.4399619850315484859 ) ) ;
#120116=ORIENTED_EDGE ( 'NONE', *, *, #208162, .F. ) ;
#120147=CARTESIAN_POINT ( 'NONE',  ( 4.115782150200256950, 6.959440387612411349, 1.199719254218452047 ) ) ;
#120149=CARTESIAN_POINT ( 'NONE',  ( 4.098537063712264228, 7.253343185014818673, 1.055677455976588686 ) ) ;
#120156=CARTESIAN_POINT ( 'NONE',  ( 5.363132282657546490, 8.414682208812571673, -1.199719254218452047 ) ) ;
#120158=CARTESIAN_POINT ( 'NONE',  ( 5.123001941117305336, 7.070197912760590064, 1.599625672291268286 ) ) ;
#120170=CARTESIAN_POINT ( 'NONE',  ( 6.435429789636040177, 6.784273175954743884, -0.4071148367965071735 ) ) ;
#120172=CARTESIAN_POINT ( 'NONE',  ( -4.936577328707246082, 8.773440960218172435, 0.000000000000000000 ) ) ;
#120173=CARTESIAN_POINT ( 'NONE',  ( 5.397554552016212703, 8.350878506444006533, 1.082531754730547524 ) ) ;
#120182=CARTESIAN_POINT ( 'NONE',  ( -5.171509248969888617, 4.998125310078441075, 0.7998128361456281477 ) ) ;
#120192=CARTESIAN_POINT ( 'NONE',  ( -3.797692425159308716, 7.444741906078900406, 0.000000000000000000 ) ) ;
#120197=CARTESIAN_POINT ( 'NONE',  ( 6.475954649182838807, 7.584310507915338562, 1.199719254218452047 ) ) ;
#120199=AXIS2_PLACEMENT_3D ( 'NONE', #83449, #168968, #20571 ) ;
#120215=CARTESIAN_POINT ( 'NONE',  ( -2.352382916832147064, 2.704376054464897816, -2.456006149337788269 ) ) ;
#120228=CARTESIAN_POINT ( 'NONE',  ( 7.828907357248368726, 8.098423103070084395, 0.7998128361456281477 ) ) ;
#120248=CARTESIAN_POINT ( 'NONE',  ( -3.147653791585731220, 8.920000000000001705, -2.419999999999998597 ) ) ;
#120254=ORIENTED_EDGE ( 'NONE', *, *, #193063, .F. ) ;
#120255=CARTESIAN_POINT ( 'NONE',  ( 3.268924434670684498, 6.827845917175511481, -1.734723475976807094E-15 ) ) ;
#120265=CARTESIAN_POINT ( 'NONE',  ( 7.388267364804250725, 7.584343111885245570, -0.7998128361456341429 ) ) ;
#120268=CARTESIAN_POINT ( 'NONE',  ( -3.960390268967665328, 6.674186842887300131, 1.082531754730549967 ) ) ;
#120299=CARTESIAN_POINT ( 'NONE',  ( 6.943184063974162434, 9.193743722760251202, -1.443375672974064550 ) ) ;
#120310=CARTESIAN_POINT ( 'NONE',  ( -5.804299160426242388, 6.904675454319632699, -1.082531754730549967 ) ) ;
#120313=CARTESIAN_POINT ( 'NONE',  ( 6.688968683495743583, 8.897159112202094988, -1.599625672291283607 ) ) ;
#120318=CARTESIAN_POINT ( 'NONE',  ( -5.981082042284069367, 7.006959133200059142, 1.199719254218452935 ) ) ;
#120330=CARTESIAN_POINT ( 'NONE',  ( -6.189608320745405123, 5.317548586107503361, 2.438128985384274472 ) ) ;
#120334=PLANE ( 'NONE',  #159766 ) ;
#120348=ORIENTED_EDGE ( 'NONE', *, *, #46978, .T. ) ;
#120359=ADVANCED_FACE ( 'NONE', ( #17629 ), #194540, .T. ) ;
#120360=CARTESIAN_POINT ( 'NONE',  ( 4.746763178560261309, 5.670883475476017566, 1.082531754730549078 ) ) ;
#120364=CARTESIAN_POINT ( 'NONE',  ( -6.954406449166956605, 7.078172043641714595, -0.7998128361456362523 ) ) ;
#120368=CARTESIAN_POINT ( 'NONE',  ( -5.798046968499580345, 6.793418213784815585, 1.199719254218452935 ) ) ;
#120369=CARTESIAN_POINT ( 'NONE',  ( -4.980641328173854632, 6.904110530993182948, 1.599625672291263401 ) ) ;
#120373=CARTESIAN_POINT ( 'NONE',  ( -6.753369912938502750, 7.051555451282599307, 0.000000000000000000 ) ) ;
#120378=ORIENTED_EDGE ( 'NONE', *, *, #179894, .F. ) ;
#120379=CARTESIAN_POINT ( 'NONE',  ( -8.100070429521727178, 8.414780020722290033, 0.7998128361456341429 ) ) ;
#120387=CARTESIAN_POINT ( 'NONE',  ( -7.608060475923978494, 8.905100639113307182, 1.199719254218452047 ) ) ;
#120389=CARTESIAN_POINT ( 'NONE',  ( 4.812217717264355876, 8.234349973070900219, 0.8868998539744571419 ) ) ;
#120394=CARTESIAN_POINT ( 'NONE',  ( 4.934241560730721510, 4.721313007132757811, 0.000000000000000000 ) ) ;
#120404=CARTESIAN_POINT ( 'NONE',  ( -7.587723245503481095, 8.881373870289390737, 1.199719254218452047 ) ) ;
#120408=CARTESIAN_POINT ( 'NONE',  ( 3.931903513251288285, 8.991426765939651844, -0.7749999999999996891 ) ) ;
#120418=CARTESIAN_POINT ( 'NONE',  ( 7.856023664475727308, 8.130058794835305136, -0.7998128361456341429 ) ) ;
#120433=CARTESIAN_POINT ( 'NONE',  ( 6.142241479726070708, 7.081583759122534794, -1.089790755372788800 ) ) ;
#120446=ORIENTED_EDGE ( 'NONE', *, *, #38054, .F. ) ;
#120455=EDGE_CURVE ( 'NONE', #211530, #105777, #162063, .T. ) ;
#120463=CARTESIAN_POINT ( 'NONE',  ( -6.126043159632901691, 7.090966632250176538, 1.117993467579528222 ) ) ;
#120483=CARTESIAN_POINT ( 'NONE',  ( -3.657667580636712934, 7.489305620709952649, -0.7998128361456481317 ) ) ;
#120502=CARTESIAN_POINT ( 'NONE',  ( -5.425723655374722121, 6.121007837424875753, 1.095972955597510401 ) ) ;
#120504=CARTESIAN_POINT ( 'NONE',  ( 7.648208051440442468, 8.095533279534887328, 0.000000000000000000 ) ) ;
#120516=CARTESIAN_POINT ( 'NONE',  ( 4.369470645354133431, 8.319742529546998000, 0.7998128361456271485 ) ) ;
#120526=CARTESIAN_POINT ( 'NONE',  ( -5.517242166118370150, 5.401480380085008193, 0.7998128361456281477 ) ) ;
#120527=CARTESIAN_POINT ( 'NONE',  ( 4.248501033035879004, 6.049946853332221153, -1.599625672291273171 ) ) ;
#120533=CARTESIAN_POINT ( 'NONE',  ( 3.006787879153326681, 6.373552747333731006, -0.4818892653130519843 ) ) ;
#120536=CARTESIAN_POINT ( 'NONE',  ( 5.664274315459256748, 9.830346811336296398, -0.7998128361456481317 ) ) ;
#120541=CARTESIAN_POINT ( 'NONE',  ( -4.651396499164954790, 8.416516698401213858, 0.5247324002638984464 ) ) ;
#120551=CARTESIAN_POINT ( 'NONE',  ( -5.004368096775595021, 5.971422546727199077, 1.082531754730549078 ) ) ;
#120561=CARTESIAN_POINT ( 'NONE',  ( 3.879041347285658414, 6.579279767591636130, -1.082531754730548412 ) ) ;
#120566=CARTESIAN_POINT ( 'NONE',  ( -6.934069218746458318, 7.054445274817795486, -0.7998128361456362523 ) ) ;
#120584=CARTESIAN_POINT ( 'NONE',  ( -4.896959554461132846, 4.880740138633571590, -0.5902973598261325172 ) ) ;
#120607=CARTESIAN_POINT ( 'NONE',  ( -4.448483799059637533, 7.243629294661272588, 1.082531754730549967 ) ) ;
#120619=CARTESIAN_POINT ( 'NONE',  ( 4.207966135563078858, 7.175396087857926375, 7.500000000000000000 ) ) ;
#120631=CARTESIAN_POINT ( 'NONE',  ( -6.903036488013351679, 8.082572653217566128, -1.199719254218452047 ) ) ;
#120637=CARTESIAN_POINT ( 'NONE',  ( -2.972980823146582186, 6.690504403638126263, 0.000000000000000000 ) ) ;
#120644=CARTESIAN_POINT ( 'NONE',  ( -3.142457743317409680, 6.888227477170756785, 0.7998128361456352531 ) ) ;
#120650=CARTESIAN_POINT ( 'NONE',  ( 2.878073747850912412, 6.579779482459851003, -0.7998128361456362523 ) ) ;
#120656=CARTESIAN_POINT ( 'NONE',  ( -6.343235766347277149, 8.493804042195527870, -1.599625672291271394 ) ) ;
#120659=CARTESIAN_POINT ( 'NONE',  ( -3.311934663488232733, 7.085950550703385531, -0.7998128361456481317 ) ) ;
#120663=CARTESIAN_POINT ( 'NONE',  ( -6.522881301506166629, 9.663759714182251770, 1.082531754730549967 ) ) ;
#120664=CARTESIAN_POINT ( 'NONE',  ( 4.163762572728282763, 6.911454530608037494, -1.082531754730548412 ) ) ;
#120665=CARTESIAN_POINT ( 'NONE',  ( -4.136646265500958819, 7.840188053144158786, -0.7216878364870458196 ) ) ;
#120670=CARTESIAN_POINT ( 'NONE',  ( -4.125423880308188629, 8.035021303660013103, -0.7998128361456481317 ) ) ;
#120673=CARTESIAN_POINT ( 'NONE',  ( 4.927462483923885195, 4.713404084191450849, -0.7998128361456481317 ) ) ;
#120674=VERTEX_POINT ( 'NONE', #104253 ) ;
#120679=CARTESIAN_POINT ( 'NONE',  ( 4.529305835417093640, 7.441884687032027657, -1.199719254218450271 ) ) ;
#120684=CARTESIAN_POINT ( 'NONE',  ( 1.863054968392299671, 2.484104531656126102, 2.477705830955055699 ) ) ;
#120685=CARTESIAN_POINT ( 'NONE',  ( 4.831949485534527966, 8.212610664285437068, 0.9193987405316924599 ) ) ;
#120691=VERTEX_POINT ( 'NONE', #187615 ) ;
#120693=B_SPLINE_CURVE_WITH_KNOTS ( 'NONE', 3,
 ( #196236, #53176, #71533, #88894, #73688, #119304, #69398 ),
 .UNSPECIFIED., .F., .F.,
 ( 4, 3, 4 ),
 ( 0.000000000000000000, 3.004831683896754227E-05, 4.142468191938748892E-05 ),
 .UNSPECIFIED. ) ;
#120695=CARTESIAN_POINT ( 'NONE',  ( 6.200875153403774043, 8.327716660428123419, -1.599625672291283607 ) ) ;
#120705=CARTESIAN_POINT ( 'NONE',  ( 5.355423173304108886, 7.585870477640591858, 1.239999553246450725 ) ) ;
#120711=( BOUNDED_CURVE ( )  B_SPLINE_CURVE ( 2, ( #71966, #40581, #39494, #154320, #186801 ),
 .UNSPECIFIED., .F., .T. ) 
 B_SPLINE_CURVE_WITH_KNOTS ( ( 3, 2, 3 ),
 ( 0.2625000001274112038, 0.2666666666666666075, 0.2749999999999999112 ),
 .UNSPECIFIED. ) 
 CURVE ( )  GEOMETRIC_REPRESENTATION_ITEM ( )  RATIONAL_B_SPLINE_CURVE ( ( 0.9330127018922194093, 0.9330127039406028722, 1.000000000000000000, 0.8660254037844404840, 0.9999999999999982236 ) ) 
 REPRESENTATION_ITEM ( '' )  );
#120721=CARTESIAN_POINT ( 'NONE',  ( 4.147109113946162218, 7.227559249243857842, -0.9911899289537524638 ) ) ;
#120724=CARTESIAN_POINT ( 'NONE',  ( -4.769436176957319695, 8.786368983084006601, 0.7998128361456281477 ) ) ;
#120737=CARTESIAN_POINT ( 'NONE',  ( 6.062430963966053632, 7.101866208495718702, -1.199719254218452047 ) ) ;
#120739=CARTESIAN_POINT ( 'NONE',  ( 8.167861197590044142, 8.493869250135347215, 0.000000000000000000 ) ) ;
#120749=CARTESIAN_POINT ( 'NONE',  ( 3.729901657090948230, 6.405283462364505631, 1.082531754730549078 ) ) ;
#120756=CARTESIAN_POINT ( 'NONE',  ( 1.913245249192530695, 8.998828458478531189, 0.7750000000000004663 ) ) ;
#120763=CARTESIAN_POINT ( 'NONE',  ( -6.292392690518202159, 9.394856334696294553, -1.082531754730549967 ) ) ;
#120764=CARTESIAN_POINT ( 'NONE',  ( 5.383996398402570271, 9.295429874862735531, 0.000000000000000000 ) ) ;
#120773=CARTESIAN_POINT ( 'NONE',  ( -5.041653019435350380, 6.975290837464928728, -1.599625672291271394 ) ) ;
#120774=CARTESIAN_POINT ( 'NONE',  ( -3.298376509874564988, 7.070132704820777825, 0.000000000000000000 ) ) ;
#120776=CARTESIAN_POINT ( 'NONE',  ( 6.834718834620487016, 7.146462526578263308, 0.000000000000000000 ) ) ;
#120783=FACE_OUTER_BOUND ( 'NONE', #188642, .T. ) ;
#120785=CARTESIAN_POINT ( 'NONE',  ( -4.694778114904050170, 8.360933773907422761, 0.7116201367730221605 ) ) ;
#120789=CARTESIAN_POINT ( 'NONE',  ( -4.767604096130494185, 8.184890741402179870, -0.7573865900243268445 ) ) ;
#120793=CARTESIAN_POINT ( 'NONE',  ( 4.909461021924244051, 6.821066840368686712, 1.443375672974065660 ) ) ;
#120798=CARTESIAN_POINT ( 'NONE',  ( -4.294900800479008574, 8.232744377192641849, 0.000000000000000000 ) ) ;
#120810=CARTESIAN_POINT ( 'NONE',  ( 4.044074958626150185, 7.940114228364351767, 0.7998128361456271485 ) ) ;
#120850=CARTESIAN_POINT ( 'NONE',  ( 5.560252395380206991, 7.580323442733986283, 1.443375672974065660 ) ) ;
#120855=CARTESIAN_POINT ( 'NONE',  ( 4.543390873910894356, 8.314723429622471684, 0.7216878364870317197 ) ) ;
#120857=CARTESIAN_POINT ( 'NONE',  ( -3.931903513251300275, 8.991426765939651844, 0.7749999999999996891 ) ) ;
#120869=CARTESIAN_POINT ( 'NONE',  ( -6.933015448541747006, 9.181880338089085214, 1.599625672291269396 ) ) ;
#120882=CARTESIAN_POINT ( 'NONE',  ( 5.844973620822844218, 5.991759777147701804, 0.7216878364870328300 ) ) ;
#120888=CARTESIAN_POINT ( 'NONE',  ( -4.085803189671902480, 5.860132702740892263, -1.599625672291271394 ) ) ;
#120893=CARTESIAN_POINT ( 'NONE',  ( -5.641601317062239218, 8.635599732330991429, -1.082531754730549967 ) ) ;
#120896=CARTESIAN_POINT ( 'NONE',  ( -6.936931872047518155, 8.122117267924091166, 1.199719254218452047 ) ) ;
#120901=CARTESIAN_POINT ( 'NONE',  ( -3.634467696915153034, 6.397906858779740524, 1.199719254218452935 ) ) ;
#120904=CYLINDRICAL_SURFACE ( 'NONE', #98087, 3.100000000000000089 ) ;
#120910=CARTESIAN_POINT ( 'NONE',  ( -3.526002468005825286, 6.271364091718859335, -1.199719254218450271 ) ) ;
#120915=CARTESIAN_POINT ( 'NONE',  ( -5.506019780925599960, 5.596313630600862510, 0.7216878364870257245 ) ) ;
#120917=CARTESIAN_POINT ( 'NONE',  ( -5.465345319640241506, 5.548860092434608760, 0.7216878364870257245 ) ) ;
#120919=CARTESIAN_POINT ( 'NONE',  ( 6.249382461256315580, 6.255644057745969988, -0.7998128361456481317 ) ) ;
#120920=CARTESIAN_POINT ( 'NONE',  ( -4.294900800479008574, 8.232744377192641849, 0.000000000000000000 ) ) ;
#120921=CARTESIAN_POINT ( 'NONE',  ( -6.363572996767778100, 8.517530811019446091, -1.599625672291271394 ) ) ;
#120922=CARTESIAN_POINT ( 'NONE',  ( -6.533654225826463602, 6.808800017212038647, -0.5559908469023568944 ) ) ;
#120936=CARTESIAN_POINT ( 'NONE',  ( 1.886825320689233809, 2.480000000000016858, 2.459652456995882641 ) ) ;
#120970=FACE_OUTER_BOUND ( 'NONE', #116340, .T. ) ;
#120972=CARTESIAN_POINT ( 'NONE',  ( -1.860351378971601966, 8.967085675740335660, -0.7749999999999996891 ) ) ;
#120975=CARTESIAN_POINT ( 'NONE',  ( 6.387350227230087718, 6.552219065276430499, -2.500000000000000444 ) ) ;
#120983=CARTESIAN_POINT ( 'NONE',  ( 4.603875680292229156, 7.528882839386387360, 1.199719254218452047 ) ) ;
#121000=CARTESIAN_POINT ( 'NONE',  ( 5.337069745634900997, 6.255611453776062980, 1.199719254218452047 ) ) ;
#121006=CARTESIAN_POINT ( 'NONE',  ( -5.641074431737709283, 8.738948049406083385, -1.199719254218452047 ) ) ;
#121011=CARTESIAN_POINT ( 'NONE',  ( 5.910428620914669473, 5.860197910680708944, 0.000000000000000000 ) ) ;
#121018=CARTESIAN_POINT ( 'NONE',  ( -4.831252850731225124, 7.910156596299903420, 0.9996086013765632661 ) ) ;
#121024=CARTESIAN_POINT ( 'NONE',  ( 6.156811154381533591, 9.236677875870187293, -1.082531754730548412 ) ) ;
#121026=CARTESIAN_POINT ( 'NONE',  ( -4.841670253855968831, 4.821239182352949904, 0.000000000000000000 ) ) ;
#121027=CARTESIAN_POINT ( 'NONE',  ( -4.773352600463090845, 7.726605912919016106, 1.199719254218452935 ) ) ;
#121038=CARTESIAN_POINT ( 'NONE',  ( 5.401997860402196316, 5.267028690082820930, 0.000000000000000000 ) ) ;
#121039=CARTESIAN_POINT ( 'NONE',  ( 4.875038752565570732, 7.845239757038595663, -1.199719254218452047 ) ) ;
#121065=CARTESIAN_POINT ( 'NONE',  ( 3.898851692381625877, 6.706354853490643642, -1.199719254218452047 ) ) ;
#121069=CARTESIAN_POINT ( 'NONE',  ( 7.666209513884374438, 7.908608952478760834, 0.7998128361456281477 ) ) ;
#121075=CARTESIAN_POINT ( 'NONE',  ( 7.024532985656141371, 7.367912369453226695, 0.7216878364870328300 ) ) ;
#121077=CARTESIAN_POINT ( 'NONE',  ( -6.466312919074983512, 6.508729591867735031, -0.7998128361456362523 ) ) ;
#121079=CARTESIAN_POINT ( 'NONE',  ( 4.146814880933355596, 5.931313009212638931, 1.599625672291261402 ) ) ;
#121090=CARTESIAN_POINT ( 'NONE',  ( 6.132331002353889282, 6.987295666328819266, -0.9434213173033257904 ) ) ;
#121091=CARTESIAN_POINT ( 'NONE',  ( -4.821859908315634158, 5.654533310236863564, 1.199719254218452935 ) ) ;
#121105=B_SPLINE_CURVE_WITH_KNOTS ( 'NONE', 3,
 ( #169716, #115687, #2918, #83119, #185953, #17040, #197935, #99392, #68991, #37585 ),
 .UNSPECIFIED., .F., .F.,
 ( 4, 2, 2, 2, 4 ),
 ( 0.002464548724426622421, 0.002919784301308119001, 0.003375019878189615581, 0.003830255455071112161, 0.004285491031952610476 ),
 .UNSPECIFIED. ) ;
#121108=CARTESIAN_POINT ( 'NONE',  ( 4.580108180932601414, 8.499999999999996447, -0.1719113009628105149 ) ) ;
#121127=CARTESIAN_POINT ( 'NONE',  ( 7.503511670520385479, 7.718794801887437274, 0.7998128361456281477 ) ) ;
#121130=CARTESIAN_POINT ( 'NONE',  ( 7.038618024149998043, 8.240751112043669835, -1.199719254218452047 ) ) ;
#121143=CARTESIAN_POINT ( 'NONE',  ( -4.014095998097799267, 6.840806543492835345, -1.199719254218450271 ) ) ;
#121145=CARTESIAN_POINT ( 'NONE',  ( 6.821160681006793070, 7.130644680695653825, 0.7216878364870328300 ) ) ;
#121154=CARTESIAN_POINT ( 'NONE',  ( -3.637330350216213759, 7.465578851886037093, -0.7998128361456481317 ) ) ;
#121160=CARTESIAN_POINT ( 'NONE',  ( -4.146814880933400005, 5.931313009212638931, 1.599625672291270506 ) ) ;
#121161=ORIENTED_EDGE ( 'NONE', *, *, #213932, .F. ) ;
#121168=CARTESIAN_POINT ( 'NONE',  ( -2.974142338115852269, 6.685868392857900133, 0.1038623869373533903 ) ) ;
#121183=EDGE_LOOP ( 'NONE', ( #135157, #29014, #115003, #154029 ) ) ;
#121184=CARTESIAN_POINT ( 'NONE',  ( -4.457598643843001973, 8.422558527783969851, 0.000000000000000000 ) ) ;
#121186=CARTESIAN_POINT ( 'NONE',  ( -4.085803189671902480, 5.860132702740892263, -1.599625672291271394 ) ) ;
#121195=CARTESIAN_POINT ( 'NONE',  ( -6.600870636098118638, 6.767368133241304484, -0.2259646751960984468 ) ) ;
#121207=LINE ( 'NONE', #88634, #111137 ) ;
#121210=CARTESIAN_POINT ( 'NONE',  ( 3.620328817674754340, 3.489345133411980715, 2.447831560964480513 ) ) ;
#121216=CARTESIAN_POINT ( 'NONE',  ( 0.000000000000000000, 8.999999999999998224, 0.000000000000000000 ) ) ;
#121228=CARTESIAN_POINT ( 'NONE',  ( 5.571474780572990504, 5.464751763615448787, 0.7998128361456352531 ) ) ;
#121236=CARTESIAN_POINT ( 'NONE',  ( 5.176180785367283654, 9.260904359562321275, -0.7998128361456481317 ) ) ;
#121238=CARTESIAN_POINT ( 'NONE',  ( 7.028976294042106332, 7.165170195996068969, 0.000000000000000000 ) ) ;
#121251=CARTESIAN_POINT ( 'NONE',  ( 6.132331002353889282, 6.987295666328819266, -0.9434213173033257904 ) ) ;
#121253=CARTESIAN_POINT ( 'NONE',  ( 5.614485009834906393, 6.683225611963085733, -1.082531754730548412 ) ) ;
#121259=CARTESIAN_POINT ( 'NONE',  ( -3.122120512896910505, 6.864500708346841229, 0.7998128361456352531 ) ) ;
#121265=ADVANCED_FACE ( 'NONE', ( #159391 ), #96664, .T. ) ;
#121269=CARTESIAN_POINT ( 'NONE',  ( -5.600926855776894975, 6.667407765562058053, -1.082531754730549967 ) ) ;
#121273=CARTESIAN_POINT ( 'NONE',  ( 7.367930134383754215, 7.560616343061329125, -0.7998128361456341429 ) ) ;
#121279=CARTESIAN_POINT ( 'NONE',  ( 6.966220764712143243, 6.002124920821316323, -2.420000000000000373 ) ) ;
#121289=CARTESIAN_POINT ( 'NONE',  ( -1.886825320689270225, 2.480000000000016858, -2.459652456995881753 ) ) ;
#121329=CARTESIAN_POINT ( 'NONE',  ( 4.407809338218622308, 8.156544971314787063, 0.000000000000000000 ) ) ;
#121331=CARTESIAN_POINT ( 'NONE',  ( 5.722950238744211937, 5.849399164722627553, 0.7216878364870328300 ) ) ;
#121339=CARTESIAN_POINT ( 'NONE',  ( 5.989670002187236442, 10.20997511251894529, -0.7998128361456481317 ) ) ;
#121343=CARTESIAN_POINT ( 'NONE',  ( -4.285785955695645910, 7.053815144069948140, 1.082531754730549967 ) ) ;
#121347=CARTESIAN_POINT ( 'NONE',  ( 4.686350348575522240, 8.284075936624162750, 0.5876776440279610769 ) ) ;
#121363=CARTESIAN_POINT ( 'NONE',  ( 5.969332771766739931, 10.18624834369502885, -0.7998128361456481317 ) ) ;
#121373=CARTESIAN_POINT ( 'NONE',  ( 7.675324359112103423, 8.127168971818530707, 0.7216878364870267237 ) ) ;
#121387=CARTESIAN_POINT ( 'NONE',  ( -6.617788377246204945, 6.893376992974917350, -0.7216878364870338292 ) ) ;
#121390=CARTESIAN_POINT ( 'NONE',  ( 6.526270840131753737, 8.707344961610770540, -1.599625672291283607 ) ) ;
#121395=CARTESIAN_POINT ( 'NONE',  ( -3.969505113751027547, 7.853116076009993840, 1.214306433183764966E-14 ) ) ;
#121405=CARTESIAN_POINT ( 'NONE',  ( 3.444653546323793947, 6.176457016423196222, 1.199719254218451159 ) ) ;
#121436=CARTESIAN_POINT ( 'NONE',  ( -2.820451594992841482, 6.512553637458760036, 0.000000000000000000 ) ) ;
#121437=CARTESIAN_POINT ( 'NONE',  ( 4.584065335196260804, 6.441438539186039591, 1.443375672974065660 ) ) ;
#121441=CARTESIAN_POINT ( 'NONE',  ( -7.306918443122272677, 7.489436036589583345, 0.7998128361456341429 ) ) ;
#121445=CARTESIAN_POINT ( 'NONE',  ( -5.773793314573309132, 7.829454515125894964, 1.599625672291263179 ) ) ;
#121446=CARTESIAN_POINT ( 'NONE',  ( -4.630991987519598396, 7.560518531151607213, 1.199719254218452935 ) ) ;
#121450=CARTESIAN_POINT ( 'NONE',  ( -5.926322542504860458, 9.928143709648733051, -0.7216878364870338292 ) ) ;
#121456=CARTESIAN_POINT ( 'NONE',  ( -7.370792787684826486, 8.628288336167626582, -1.199719254218452047 ) ) ;
#121465=CARTESIAN_POINT ( 'NONE',  ( -5.433785704026946384, 9.561443431331920095, 0.000000000000000000 ) ) ;
#121467=CARTESIAN_POINT ( 'NONE',  ( 5.010605496441194795, 7.906410611435644498, -1.080668833775387139 ) ) ;
#121472=CARTESIAN_POINT ( 'NONE',  ( 3.953084306836263995, 6.769626237021087789, 1.199719254218452047 ) ) ;
#121482=CARTESIAN_POINT ( 'NONE',  ( -5.589704470584107909, 9.743348658981940247, -0.7998128361456362523 ) ) ;
#121494=CARTESIAN_POINT ( 'NONE',  ( 5.096939404094710468, 4.911127157724081371, 0.000000000000000000 ) ) ;
#121508=CARTESIAN_POINT ( 'NONE',  ( 6.604949037901548969, 6.766875157141204689, 0.08182522243922914218 ) ) ;
#121538=CARTESIAN_POINT ( 'NONE',  ( -6.612840081267999714, 6.759580388257274919, -0.1161152146933758927 ) ) ;
#121555=CARTESIAN_POINT ( 'NONE',  ( -7.279802135894939852, 7.457800344824362604, -0.7998128361456362523 ) ) ;
#121567=DIRECTION ( 'NONE',  ( -0.7592566023652995710, -0.6507913734559650498, 0.000000000000000000 ) ) ;
#121572=CARTESIAN_POINT ( 'NONE',  ( 3.237364818613055473, 6.998952398349030268, -1.734723475976807094E-15 ) ) ;
#121574=CARTESIAN_POINT ( 'NONE',  ( 6.658462837642791676, 8.861568958707010779, 1.443375672974063439 ) ) ;
#121588=CARTESIAN_POINT ( 'NONE',  ( 6.690022453700429139, 6.769724048930809701, 0.7998128361456331437 ) ) ;
#121598=CARTESIAN_POINT ( 'NONE',  ( -5.978219388983010418, 5.939287140093762574, -0.7998128361456362523 ) ) ;
#121600=CARTESIAN_POINT ( 'NONE',  ( 2.911969131885072670, 6.619324097166378706, 0.000000000000000000 ) ) ;
#121604=CARTESIAN_POINT ( 'NONE',  ( -7.096767062110449942, 7.244259425409119046, -0.7998128361456362523 ) ) ;
#121608=CARTESIAN_POINT ( 'NONE',  ( 7.062871678076271920, 7.204714810702593120, -0.7998128361456341429 ) ) ;
#121615=CARTESIAN_POINT ( 'NONE',  ( -5.370252646843524325, 7.685795487962019834, 1.333085116894404232 ) ) ;
#121625=CARTESIAN_POINT ( 'NONE',  ( -3.946832114909637479, 7.618738210787614484, 0.7216878364870338292 ) ) ;
#121634=CARTESIAN_POINT ( 'NONE',  ( 3.282482588284323821, 6.843663763058119187, 0.7216878364870257245 ) ) ;
#121637=CARTESIAN_POINT ( 'NONE',  ( 5.024051501469349645, 4.898199347683565463, -0.07077548676925468629 ) ) ;
#121639=CARTESIAN_POINT ( 'NONE',  ( -6.454563648557663846, 9.688018802362710957, -1.199719254218452047 ) ) ;
#121643=EDGE_CURVE ( 'NONE', #80483, #22839, #192367, .T. ) ;
#121653=CARTESIAN_POINT ( 'NONE',  ( 3.736153849017632922, 6.516540702899320081, -1.199719254218453823 ) ) ;
#121669=EDGE_LOOP ( 'NONE', ( #103200, #78588, #119848 ) ) ;
#121681=CARTESIAN_POINT ( 'NONE',  ( -4.312902262922974295, 8.045820050136510915, 0.7216878364870338292 ) ) ;
#121694=VERTEX_POINT ( 'NONE', #163605 ) ;
#121707=CARTESIAN_POINT ( 'NONE',  ( -6.474900878978163021, 9.711745571186627402, -1.199719254218452047 ) ) ;
#121710=B_SPLINE_CURVE_WITH_KNOTS ( 'NONE', 3,
 ( #173863, #105664, #11319, #140304, #108905, #126237 ),
 .UNSPECIFIED., .F., .F.,
 ( 4, 2, 4 ),
 ( 0.000000000000000000, 0.002406312826513442183, 0.004812625653026884366 ),
 .UNSPECIFIED. ) ;
#121714=CARTESIAN_POINT ( 'NONE',  ( -4.285259070371116863, 7.157163461145040095, 1.199719254218452935 ) ) ;
#121721=CARTESIAN_POINT ( 'NONE',  ( -5.490125858891038213, 5.369844688319787451, -0.7998128361456362523 ) ) ;
#121727=CARTESIAN_POINT ( 'NONE',  ( 3.528865121306874464, 7.339036084825155015, -0.7998128361456362523 ) ) ;
#121732=CARTESIAN_POINT ( 'NONE',  ( -5.250750630242457362, 9.347902511916677426, 0.000000000000000000 ) ) ;
#121736=CARTESIAN_POINT ( 'NONE',  ( -4.984557751679625781, 5.844347460828191565, 1.199719254218452935 ) ) ;
#121739=CARTESIAN_POINT ( 'NONE',  ( 4.231553341240931410, 7.950912974840878888, -0.7216878364870107365 ) ) ;
#121740=CARTESIAN_POINT ( 'NONE',  ( 4.217995187182920880, 6.974725914138481642, 1.082531754730549078 ) ) ;
#121741=CARTESIAN_POINT ( 'NONE',  ( -6.089020385868876062, 6.276481003034692030, -0.7216878364870338292 ) ) ;
#121747=CARTESIAN_POINT ( 'NONE',  ( 3.607351389687783794, 6.366271167014519783, 1.199719254218451159 ) ) ;
#121759=CARTESIAN_POINT ( 'NONE',  ( 5.403926048761924505, 7.658933883257522446, 1.327442161737320436 ) ) ;
#121765=ORIENTED_EDGE ( 'NONE', *, *, #48284, .F. ) ;
#121768=CARTESIAN_POINT ( 'NONE',  ( 5.905458427204159477, 9.047396044116986502, 1.199719254218452047 ) ) ;
#121780=CARTESIAN_POINT ( 'NONE',  ( 6.348661983278831578, 6.841051910588018536, 0.6299351563821649069 ) ) ;
#121795=CARTESIAN_POINT ( 'NONE',  ( -8.106849506328558164, 8.422688943663599659, 0.000000000000000000 ) ) ;
#121800=CARTESIAN_POINT ( 'NONE',  ( -7.065207446497166366, 9.336104335703744539, 0.000000000000000000 ) ) ;
#121809=CARTESIAN_POINT ( 'NONE',  ( 6.235824307642648279, 6.239826211863360506, 0.000000000000000000 ) ) ;
#121816=CARTESIAN_POINT ( 'NONE',  ( -6.414416072596837104, 9.537216947121368804, -1.082531754730549967 ) ) ;
#121820=CARTESIAN_POINT ( 'NONE',  ( 5.207740400980577888, 5.248321020665011716, 0.000000000000000000 ) ) ;
#121833=CARTESIAN_POINT ( 'NONE',  ( -2.972980823146582186, 6.690504403638126263, 0.000000000000000000 ) ) ;
#121834=CARTESIAN_POINT ( 'NONE',  ( 5.506019780925567986, 8.477421273504887722, -1.082531754730548412 ) ) ;
#121845=CARTESIAN_POINT ( 'NONE',  ( -4.437261413422502798, 8.398831758960053406, 0.000000000000000000 ) ) ;
#121846=CARTESIAN_POINT ( 'NONE',  ( -4.442231607132987925, 5.211633625523774960, -1.199719254218453823 ) ) ;
#121848=CARTESIAN_POINT ( 'NONE',  ( 7.173672674962134899, 7.541908673643526129, -0.7216878364870317197 ) ) ;
#121860=CARTESIAN_POINT ( 'NONE',  ( -4.934256961717153445, 8.002024883745839645, -1.000413331142641526 ) ) ;
#121864=CARTESIAN_POINT ( 'NONE',  ( 4.828112100242277549, 6.726159765073026264, -1.443375672974068769 ) ) ;
#121868=CARTESIAN_POINT ( 'NONE',  ( -6.967964602780620353, 7.093989889524320525, 0.000000000000000000 ) ) ;
#121882=CARTESIAN_POINT ( 'NONE',  ( 6.039231080244466199, 6.010467446565510130, 0.7998128361456352531 ) ) ;
#121921=CARTESIAN_POINT ( 'NONE',  ( 6.916067756746836714, 8.201738816693689316, -1.082531754730548412 ) ) ;
#121926=CARTESIAN_POINT ( 'NONE',  ( 6.333067150914808430, 8.481940657524365434, 1.443375672974063439 ) ) ;
#121941=CARTESIAN_POINT ( 'NONE',  ( -5.420227550413282636, 9.545625585449309725, 0.7998128361456291469 ) ) ;
#121950=CARTESIAN_POINT ( 'NONE',  ( -3.546339698426324460, 6.295090860542775779, -1.199719254218450271 ) ) ;
#121952=CARTESIAN_POINT ( 'NONE',  ( 3.675669042636310557, 6.342012078834061484, -1.082531754730549967 ) ) ;
#121958=CARTESIAN_POINT ( 'NONE',  ( -2.830620210203090181, 6.524417021870718258, 0.000000000000000000 ) ) ;
#121963=CARTESIAN_POINT ( 'NONE',  ( -6.617788377246193399, 8.814115421577600529, -1.443375672974066548 ) ) ;
#121967=CARTESIAN_POINT ( 'NONE',  ( -7.370792787684826486, 8.628288336167626582, -1.199719254218452047 ) ) ;
#121974=CARTESIAN_POINT ( 'NONE',  ( -5.255720823952942489, 6.160704378480398979, -1.199719254218453823 ) ) ;
#121988=CARTESIAN_POINT ( 'NONE',  ( -4.123088112331656951, 6.864000993478624579, 1.082531754730549967 ) ) ;
#121990=CARTESIAN_POINT ( 'NONE',  ( -5.329763783503577379, 6.351050847909847086, 1.082531754730549078 ) ) ;
#121992=CARTESIAN_POINT ( 'NONE',  ( 3.739016502318667445, 7.584212696005614873, 0.7998128361456271485 ) ) ;
#121993=CARTESIAN_POINT ( 'NONE',  ( -6.303615075710993665, 6.318915441276411471, -0.7998128361456362523 ) ) ;
#121994=CARTESIAN_POINT ( 'NONE',  ( -5.108390017298964914, 9.181815130149269422, 0.000000000000000000 ) ) ;
#122013=CARTESIAN_POINT ( 'NONE',  ( 5.203297092594585393, 9.292540051327542017, 0.7998128361456341429 ) ) ;
#122018=CARTESIAN_POINT ( 'NONE',  ( -5.458264003855187951, 7.602368174425947700, -1.382272695577278387 ) ) ;
#122037=CARTESIAN_POINT ( 'NONE',  ( 4.857564175446106525, 8.889184981320973122, 0.7998128361456331437 ) ) ;
#122044=CARTESIAN_POINT ( 'NONE',  ( 4.450244736157840109, 7.987476157872942295, -2.500000000000000444 ) ) ;
#122052=CARTESIAN_POINT ( 'NONE',  ( 6.561219994370630637, 6.619454513046008515, 0.000000000000000000 ) ) ;
#122066=CARTESIAN_POINT ( 'NONE',  ( 6.343551558972070126, 6.506286488053498296, 2.500000000000000000 ) ) ;
#122067=AXIS2_PLACEMENT_3D ( 'NONE', #26393, #3984, #122126 ) ;
#122070=CARTESIAN_POINT ( 'NONE',  ( 4.553559489343365740, 6.405848385690952718, -1.599625672291269396 ) ) ;
#122077=CARTESIAN_POINT ( 'NONE',  ( -7.937372586157736443, 8.224965870130965584, 0.7998128361456341429 ) ) ;
#122082=CARTESIAN_POINT ( 'NONE',  ( 4.199993725183334803, 8.122019456014369254, -0.7998128361456362523 ) ) ;
#122092=CARTESIAN_POINT ( 'NONE',  ( 5.994113311017540191, 9.046863725278862844, -1.082531754730548412 ) ) ;
#122093=CARTESIAN_POINT ( 'NONE',  ( -4.828112100242303306, 4.805421336470338645, -0.7216878364870338292 ) ) ;
#122094=CARTESIAN_POINT ( 'NONE',  ( -6.448838341955544173, 7.552674816150118708, 1.199719254218452047 ) ) ;
#122106=CARTESIAN_POINT ( 'NONE',  ( 5.204350862799327793, 7.165104988056252289, -1.599625672291281386 ) ) ;
#122107=CARTESIAN_POINT ( 'NONE',  ( 4.549643065837591038, 7.465611455855944101, -1.199719254218452047 ) ) ;
#122110=CARTESIAN_POINT ( 'NONE',  ( 6.068156270568149324, 9.237210194708310951, 1.199719254218452047 ) ) ;
#122126=DIRECTION ( 'NONE',  ( 0.000000000000000000, 0.000000000000000000, 1.000000000000000000 ) ) ;
#122129=CARTESIAN_POINT ( 'NONE',  ( 5.717785742877111055, 7.006476535625807855, -2.500000000000000000 ) ) ;
#122130=CARTESIAN_POINT ( 'NONE',  ( 5.734172623936983904, 5.654565914206774124, 0.7998128361456352531 ) ) ;
#122134=CARTESIAN_POINT ( 'NONE',  ( 4.760848217054122422, 5.583353003765119560, -1.199719254218452047 ) ) ;
#122138=CARTESIAN_POINT ( 'NONE',  ( 4.934241560730721510, 4.721313007132757811, 0.000000000000000000 ) ) ;
#122142=CARTESIAN_POINT ( 'NONE',  ( 5.397554552016216256, 7.390509292142662723, 1.443375672974065660 ) ) ;
#122144=CARTESIAN_POINT ( 'NONE',  ( -4.620296487206990932, 8.612372678375294299, 0.000000000000000000 ) ) ;
#122146=CARTESIAN_POINT ( 'NONE',  ( 3.230585741806197841, 6.991043475407723307, 0.7998128361456271485 ) ) ;
#122159=CARTESIAN_POINT ( 'NONE',  ( -7.485510208520816278, 8.866088343763324886, 1.082531754730549078 ) ) ;
#122164=ORIENTED_EDGE ( 'NONE', *, *, #197691, .T. ) ;
#122170=CARTESIAN_POINT ( 'NONE',  ( 0.4770138163741251547, 3.005786281947454786, -1.942556692846756361 ) ) ;
#122198=CARTESIAN_POINT ( 'NONE',  ( 5.671053392266061977, 9.838255734277600695, 0.7998128361456331437 ) ) ;
#122200=CARTESIAN_POINT ( 'NONE',  ( 6.444921918449731280, 8.612437886315108315, 1.599625672291268286 ) ) ;
#122214=CARTESIAN_POINT ( 'NONE',  ( -6.180537922983287302, 8.303989891604203422, -1.599625672291271394 ) ) ;
#122216=CARTESIAN_POINT ( 'NONE',  ( 5.763624699140868834, 7.817591130454727200, -1.443375672974078761 ) ) ;
#122227=CARTESIAN_POINT ( 'NONE',  ( -4.984557751679625781, 5.844347460828191565, 1.199719254218452935 ) ) ;
#122235=CARTESIAN_POINT ( 'NONE',  ( -3.959863383643135393, 6.777535159962392086, 1.199719254218452935 ) ) ;
#122258=CARTESIAN_POINT ( 'NONE',  ( -6.330731382938325602, 6.350551133041632212, 0.7998128361456281477 ) ) ;
#122270=CYLINDRICAL_SURFACE ( 'NONE', #111231, 1.250000000000000000 ) ;
#122271=CARTESIAN_POINT ( 'NONE',  ( -4.983945206004156248, 6.510271170337021296, -1.264942728826349949 ) ) ;
#122281=CARTESIAN_POINT ( 'NONE',  ( -3.096514578442687515, 6.188910745953249304, -0.7944190528704382359 ) ) ;
#122284=CARTESIAN_POINT ( 'NONE',  ( -4.308458954092677651, 8.248562223075252220, -0.7998128361456362523 ) ) ;
#122285=CARTESIAN_POINT ( 'NONE',  ( 6.966220764712121927, 6.002124920821316323, 2.500000000000000444 ) ) ;
#122294=EDGE_CURVE ( 'NONE', #40830, #197229, #73449, .T. ) ;
#122305=CARTESIAN_POINT ( 'NONE',  ( 6.073126464278658432, 6.050012061272033392, 0.000000000000000000 ) ) ;
#122314=CARTESIAN_POINT ( 'NONE',  ( 6.363572996767764778, 8.517530811019446091, -1.599625672291283607 ) ) ;
#122316=CARTESIAN_POINT ( 'NONE',  ( 6.703580607314123085, 6.785541894813420072, 0.000000000000000000 ) ) ;
#122329=CARTESIAN_POINT ( 'NONE',  ( 6.365646016822680942, 6.829858545691475769, 0.5939985411197836740 ) ) ;
#122331=CARTESIAN_POINT ( 'NONE',  ( 4.584065335196252811, 8.362176967788721882, 0.7216878364870328300 ) ) ;
#122339=CARTESIAN_POINT ( 'NONE',  ( -4.228163802615396705, 6.026220084508304708, -1.599625672291271394 ) ) ;
#122340=CARTESIAN_POINT ( 'NONE',  ( 3.611473365557979598, 7.348452737196720541, -0.2779858853791586926 ) ) ;
#122350=CARTESIAN_POINT ( 'NONE',  ( -4.624739795592936353, 7.449261290616792763, -1.082531754730549967 ) ) ;
#122353=CARTESIAN_POINT ( 'NONE',  ( 7.289443866002793371, 8.533381260871966134, 1.199719254218452047 ) ) ;
#122373=CARTESIAN_POINT ( 'NONE',  ( 7.028976294042106332, 7.165170195996068969, 0.000000000000000000 ) ) ;
#122390=VERTEX_POINT ( 'NONE', #39559 ) ;
#122392=CARTESIAN_POINT ( 'NONE',  ( 3.231779075379113131, 6.036511184309971689, 0.9899555337401855226 ) ) ;
#122393=CARTESIAN_POINT ( 'NONE',  ( -3.001735798205259265, 6.389591682482198109, -0.7455002297410243672 ) ) ;
#122410=CARTESIAN_POINT ( 'NONE',  ( 4.746763178560261309, 5.670883475476017566, 1.082531754730549078 ) ) ;
#122423=CARTESIAN_POINT ( 'NONE',  ( -5.641601317062259646, 5.754492089426966217, -0.7216878364870338292 ) ) ;
#122454=CARTESIAN_POINT ( 'NONE',  ( 4.634908411025333130, 6.500755460986618495, 1.599625672291268286 ) ) ;
#122468=CARTESIAN_POINT ( 'NONE',  ( -5.966997003790232235, 7.094489604910957148, -1.082531754730549967 ) ) ;
#122470=CARTESIAN_POINT ( 'NONE',  ( 6.013923656113508542, 9.173938811177871244, -1.199719254218452047 ) ) ;
#122485=ORIENTED_EDGE ( 'NONE', *, *, #85855, .F. ) ;
#122519=CARTESIAN_POINT ( 'NONE',  ( -7.282664789195997912, 8.525472337930658284, 1.199719254218452047 ) ) ;
#122522=CARTESIAN_POINT ( 'NONE',  ( -6.017840079619296567, 8.114175741012878973, -1.599625672291271394 ) ) ;
#122523=CARTESIAN_POINT ( 'NONE',  ( -4.132202957115018727, 8.042930226601317401, 0.000000000000000000 ) ) ;
#122527=CARTESIAN_POINT ( 'NONE',  ( -6.414416072596845986, 8.576847732820027659, -1.443375672974066548 ) ) ;
#122529=CARTESIAN_POINT ( 'NONE',  ( 6.604230223188150894, 9.758666789477915771, -1.082531754730548412 ) ) ;
#122535=CARTESIAN_POINT ( 'NONE',  ( -4.625266680917477835, 5.425174544939014964, -1.199719254218453823 ) ) ;
#122542=CARTESIAN_POINT ( 'NONE',  ( -5.908321080505254841, 10.11506803722328129, 0.7998128361456291469 ) ) ;
#122544=CARTESIAN_POINT ( 'NONE',  ( 4.653539691347775786, 8.417882268172059312, -0.4891605808478947104 ) ) ;
#122549=CARTESIAN_POINT ( 'NONE',  ( 5.571474780572990504, 5.464751763615448787, 0.7998128361456352531 ) ) ;
#122550=ADVANCED_FACE ( 'NONE', ( #126233, #89397 ), #40648, .F. ) ;
#122559=CARTESIAN_POINT ( 'NONE',  ( -6.454563648557663846, 9.688018802362710957, -1.199719254218452047 ) ) ;
#122572=CARTESIAN_POINT ( 'NONE',  ( 7.828907357248368726, 8.098423103070084395, 0.7998128361456281477 ) ) ;
#122587=CARTESIAN_POINT ( 'NONE',  ( 5.669760509565840323, 7.437725440679550992, 1.325564871123290356 ) ) ;
#122606=CARTESIAN_POINT ( 'NONE',  ( 0.000000000000000000, 5.939655416065874327, 0.000000000000000000 ) ) ;
#122614=CARTESIAN_POINT ( 'NONE',  ( -6.454776619733716636, 6.787828609132271929, -0.3692292702514640146 ) ) ;
#122624=LINE ( 'NONE', #152890, #20508 ) ;
#122630=CARTESIAN_POINT ( 'NONE',  ( 3.582479189645107809, 7.343285104996937207, -0.3223619143407419063 ) ) ;
#122634=CARTESIAN_POINT ( 'NONE',  ( -6.119526231721793330, 8.232809585132461194, 1.599625672291263179 ) ) ;
#122650=CARTESIAN_POINT ( 'NONE',  ( 6.249382461256315580, 6.255644057745969988, -0.7998128361456481317 ) ) ;
#122662=CARTESIAN_POINT ( 'NONE',  ( 5.324837791525375508, 7.612559486139466536, 1.234112182050936646 ) ) ;
#122681=CARTESIAN_POINT ( 'NONE',  ( -5.829079699232685208, 5.765290835385048496, 0.000000000000000000 ) ) ;
#122683=CARTESIAN_POINT ( 'NONE',  ( 3.549202351727371862, 7.362762853649070571, -0.7998128361456362523 ) ) ;
#122686=CARTESIAN_POINT ( 'NONE',  ( -4.586401103172829785, 8.572828063668767484, 0.7998128361456281477 ) ) ;
#122690=CARTESIAN_POINT ( 'NONE',  ( 7.038618024149998043, 8.240751112043669835, -1.199719254218452047 ) ) ;
#122696=CARTESIAN_POINT ( 'NONE',  ( -4.594589183792981757, 8.486487934283967860, 0.2047448450237729367 ) ) ;
#122705=CARTESIAN_POINT ( 'NONE',  ( -5.492461626867567226, 6.540864998501174199, 1.082531754730549078 ) ) ;
#122716=CARTESIAN_POINT ( 'NONE',  ( 5.099275172515607579, 5.121778254122544283, -0.7216878364870458196 ) ) ;
#122719=CARTESIAN_POINT ( 'NONE',  ( -5.752402313948099533, 9.933162809573264695, -0.7998128361456362523 ) ) ;
#122737=CARTESIAN_POINT ( 'NONE',  ( 6.561219994370630637, 6.619454513046008515, 0.000000000000000000 ) ) ;
#122763=CARTESIAN_POINT ( 'NONE',  ( -4.665414256878301025, 6.536345614481700927, -1.443375672974066548 ) ) ;
#122785=CARTESIAN_POINT ( 'NONE',  ( -7.014364370223741929, 9.276787413384745662, -1.599625672291271394 ) ) ;
#122787=CARTESIAN_POINT ( 'NONE',  ( -2.844178363816758814, 6.540234867753325076, -0.7998128361456481317 ) ) ;
#122792=CARTESIAN_POINT ( 'NONE',  ( -4.930325137224961907, 5.781076077297750970, -1.199719254218453823 ) ) ;
#122796=DIRECTION ( 'NONE',  ( 0.000000000000000000, 0.000000000000000000, -1.000000000000000000 ) ) ;
#122801=CARTESIAN_POINT ( 'NONE',  ( -4.492547798081878874, 6.334668079219206049, 1.599625672291263179 ) ) ;
#122803=CARTESIAN_POINT ( 'NONE',  ( 6.435676556713933572, 6.878741676577107889, -0.7109887800627444632 ) ) ;
#122807=CARTESIAN_POINT ( 'NONE',  ( 3.881377115262159894, 7.750300077773022878, 0.7998128361456271485 ) ) ;
#122812=CARTESIAN_POINT ( 'NONE',  ( -6.099189001301292379, 8.209082816308541197, 1.599625672291263179 ) ) ;
#122817=CARTESIAN_POINT ( 'NONE',  ( -4.553559489343377287, 6.405848385690952718, -1.599625672291271394 ) ) ;
#122822=CARTESIAN_POINT ( 'NONE',  ( 5.275531169048895741, 7.248148678680751189, -1.443375672974078761 ) ) ;
#122823=CARTESIAN_POINT ( 'NONE',  ( -4.787437638956927977, 7.639075441208117212, -1.082531754730549967 ) ) ;
#122831=CARTESIAN_POINT ( 'NONE',  ( 5.578253857379852576, 5.472660686556754861, -0.7998128361456481317 ) ) ;
#122838=DIRECTION ( 'NONE',  ( 0.000000000000000000, 0.000000000000000000, 1.000000000000000000 ) ) ;
#122843=CARTESIAN_POINT ( 'NONE',  ( 5.869365784521903606, 7.282179437329668659, 1.264975801879052453 ) ) ;
#122854=CARTESIAN_POINT ( 'NONE',  ( 4.538947565524982686, 8.517465603079630299, 0.000000000000000000 ) ) ;
#122864=CARTESIAN_POINT ( 'NONE',  ( 5.606371582794006159, 7.377293116531995487, 1.238817421570908905 ) ) ;
#122876=EDGE_CURVE ( 'NONE', #75032, #53161, #43567, .T. ) ;
#122883=CARTESIAN_POINT ( 'NONE',  ( -7.618755976236585958, 7.853246491889623648, 0.000000000000000000 ) ) ;
#122895=CARTESIAN_POINT ( 'NONE',  ( 7.038618024149998043, 8.240751112043669835, -1.199719254218452047 ) ) ;
#122901=CARTESIAN_POINT ( 'NONE',  ( -6.983858524370814003, 9.241197259889665006, 1.443375672974064550 ) ) ;
#122902=ORIENTED_EDGE ( 'NONE', *, *, #131609, .T. ) ;
#122903=CARTESIAN_POINT ( 'NONE',  ( 3.984117037569365305, 5.741498858621315371, 1.599625672291261402 ) ) ;
#122906=CARTESIAN_POINT ( 'NONE',  ( 3.065552130021340194, 6.590578228417936835, 0.000000000000000000 ) ) ;
#122919=CARTESIAN_POINT ( 'NONE',  ( -5.008811405605897882, 4.808311159487113073, 0.7998128361456281477 ) ) ;
#122920=CARTESIAN_POINT ( 'NONE',  ( 8.014278199453778839, 8.522615118883788199, 0.000000000000000000 ) ) ;
#122930=ORIENTED_EDGE ( 'NONE', *, *, #143526, .F. ) ;
#122931=CARTESIAN_POINT ( 'NONE',  ( -6.069210040772897052, 7.109775131437022999, -1.199719254218453823 ) ) ;
#122932=CARTESIAN_POINT ( 'NONE',  ( -3.623772196602547346, 7.449761006003425834, 0.000000000000000000 ) ) ;
#122934=CARTESIAN_POINT ( 'NONE',  ( 5.031484404002878996, 7.923796667095108326, 1.082531754730548412 ) ) ;
#122945=CARTESIAN_POINT ( 'NONE',  ( -4.629329830860687167, 8.351765225447314478, -0.3187335059142253346 ) ) ;
#122949=CARTESIAN_POINT ( 'NONE',  ( 5.750066545971570520, 5.881034856487848295, -0.7216878364870458196 ) ) ;
#122951=DIRECTION ( 'NONE',  ( 1.000000000000000000, 0.000000000000000000, 0.000000000000000000 ) ) ;
#122954=CARTESIAN_POINT ( 'NONE',  ( -5.420227550413282636, 9.545625585449309725, 0.7998128361456291469 ) ) ;
#122968=CARTESIAN_POINT ( 'NONE',  ( 6.201928923608456046, 6.200281597156833691, 0.7998128361456352531 ) ) ;
#122982=EDGE_CURVE ( 'NONE', #135497, #129718, #24488, .T. ) ;
#122984=CARTESIAN_POINT ( 'NONE',  ( -6.966220764712169000, 6.002124920821316323, -2.420000000000000373 ) ) ;
#123008=CARTESIAN_POINT ( 'NONE',  ( 5.072158865288222351, 8.931619419562697004, 0.7216878364870317197 ) ) ;
#123015=CARTESIAN_POINT ( 'NONE',  ( 7.648208051440442468, 8.095533279534887328, 0.000000000000000000 ) ) ;
#123042=CARTESIAN_POINT ( 'NONE',  ( -4.411198876399886615, 6.239761003923544713, -1.599625672291271394 ) ) ;
#123044=CARTESIAN_POINT ( 'NONE',  ( 4.543390873910903238, 7.354354215321133204, 1.082531754730548412 ) ) ;
#123050=CARTESIAN_POINT ( 'NONE',  ( -3.318713740295064163, 7.093859473644694269, 0.000000000000000000 ) ) ;
#123054=CARTESIAN_POINT ( 'NONE',  ( -6.943184063974175757, 9.193743722760251202, -1.443375672974066548 ) ) ;
#123057=CARTESIAN_POINT ( 'NONE',  ( -7.923814432544069142, 8.209148024248356990, 0.000000000000000000 ) ) ;
#123062=CARTESIAN_POINT ( 'NONE',  ( -4.122561227007127016, 6.967349310553715647, 1.199719254218452935 ) ) ;
#123074=DIRECTION ( 'NONE',  ( 0.6507913734559658270, -0.7592566023652989049, 0.000000000000000000 ) ) ;
#123075=CARTESIAN_POINT ( 'NONE',  ( -5.641601317062248988, 6.714861303728305586, -1.082531754730549967 ) ) ;
#123077=CARTESIAN_POINT ( 'NONE',  ( -5.275531169048901958, 8.208517892982092334, -1.082531754730549967 ) ) ;
#123078=CARTESIAN_POINT ( 'NONE',  ( 5.761288931164342486, 5.686201605971993978, -0.7998128361456481317 ) ) ;
#123079=CARTESIAN_POINT ( 'NONE',  ( -6.967964602780620353, 7.093989889524320525, 0.000000000000000000 ) ) ;
#123093=VERTEX_POINT ( 'NONE', #37171 ) ;
#123095=CARTESIAN_POINT ( 'NONE',  ( 2.352382916832110649, 2.704376054464898704, 2.456006149337789157 ) ) ;
#123100=CARTESIAN_POINT ( 'NONE',  ( 6.363572996767764778, 8.517530811019446091, -1.599625672291283607 ) ) ;
#123138=CARTESIAN_POINT ( 'NONE',  ( 4.525389411911321602, 8.501647757197021704, -0.7998128361456381397 ) ) ;
#123141=CARTESIAN_POINT ( 'NONE',  ( -5.517242166118370150, 5.401480380085008193, 0.7998128361456281477 ) ) ;
#123156=CARTESIAN_POINT ( 'NONE',  ( 5.713835393516482952, 5.630839145382857680, 0.7998128361456352531 ) ) ;
#123161=CARTESIAN_POINT ( 'NONE',  ( -5.887983850084758330, 10.09134126839936840, 0.7998128361456291469 ) ) ;
#123165=CARTESIAN_POINT ( 'NONE',  ( 4.655245641445829641, 6.524482229810530498, 1.599625672291269396 ) ) ;
#123176=CARTESIAN_POINT ( 'NONE',  ( 6.482206841109512396, 9.616306177052839743, -1.082531754730548412 ) ) ;
#123177=CARTESIAN_POINT ( 'NONE',  ( -4.990809943606294929, 4.995235487061662205, -0.7216878364870338292 ) ) ;
#123178=CARTESIAN_POINT ( 'NONE',  ( -6.445975688654487001, 6.485002823043819475, -0.7998128361456362523 ) ) ;
#123189=CARTESIAN_POINT ( 'NONE',  ( 5.123001941117305336, 7.070197912760590064, 1.599625672291268286 ) ) ;
#123190=CARTESIAN_POINT ( 'NONE',  ( 6.086684617892325733, 6.065829907154645539, -0.7998128361456481317 ) ) ;
#123193=CARTESIAN_POINT ( 'NONE',  ( 5.691390622686558487, 9.861982503101517139, 0.7998128361456341429 ) ) ;
#123198=DIRECTION ( 'NONE',  ( -1.000000000000000000, -3.135042426464105837E-15, 0.000000000000000000 ) ) ;
#123207=CARTESIAN_POINT ( 'NONE',  ( 5.959663945170571075, 7.214374732172471383, -1.219933935757764099 ) ) ;
#123208=VERTEX_POINT ( 'NONE', #33970 ) ;
#123210=CARTESIAN_POINT ( 'NONE',  ( 4.329849954717849947, 6.144853928627882489, 1.599625672291262513 ) ) ;
#123214=CARTESIAN_POINT ( 'NONE',  ( 4.598150373690133463, 5.393538853173795111, -1.199719254218452047 ) ) ;
#123219=CARTESIAN_POINT ( 'NONE',  ( 2.925527285498711549, 6.635141943048991742, 0.7998128361456281477 ) ) ;
#123223=CARTESIAN_POINT ( 'NONE',  ( 5.316205630334249754, 7.295602216847000498, -1.443375672974078761 ) ) ;
#123225=CARTESIAN_POINT ( 'NONE',  ( -4.796552484184649856, 8.818004674849227342, -0.7998128361456362523 ) ) ;
#123227=CARTESIAN_POINT ( 'NONE',  ( 5.228604516725597229, 6.129068686715179126, -1.199719254218450271 ) ) ;
#123237=CARTESIAN_POINT ( 'NONE',  ( -4.496464221587651799, 5.274905009054215554, 1.199719254218452935 ) ) ;
#123242=VERTEX_POINT ( 'NONE', #166109 ) ;
#123246=CARTESIAN_POINT ( 'NONE',  ( -5.608757509019083543, 5.629766575900002401, -2.420000000000000373 ) ) ;
#123247=CARTESIAN_POINT ( 'NONE',  ( 0.3975484427966501366, 2.885820281855256741, -1.961872594692045890 ) ) ;
#123269=CARTESIAN_POINT ( 'NONE',  ( 5.099275172515607579, 5.121778254122544283, -0.7216878364870458196 ) ) ;
#123271=VERTEX_POINT ( 'NONE', #7859 ) ;
#123275=CARTESIAN_POINT ( 'NONE',  ( -5.182812566104885832, 7.844509203380741980, -1.320274515446249408 ) ) ;
#123277=CARTESIAN_POINT ( 'NONE',  ( 3.214691819771663628, 6.764574533126651801, -0.7216878364870338292 ) ) ;
#123288=CARTESIAN_POINT ( 'NONE',  ( -4.288121723672178476, 8.224835454251337552, -0.7998128361456362523 ) ) ;
#123290=CARTESIAN_POINT ( 'NONE',  ( 7.471952054462756010, 7.889901283060952508, 0.7216878364870267237 ) ) ;
#123299=CARTESIAN_POINT ( 'NONE',  ( -3.935609729716867289, 7.813571461303467913, 0.7998128361456352531 ) ) ;
#123307=CARTESIAN_POINT ( 'NONE',  ( -2.810282979782591006, 6.500690253046801814, 0.000000000000000000 ) ) ;
#123329=CARTESIAN_POINT ( 'NONE',  ( -7.119966945832006289, 8.335658187339330283, 1.199719254218452047 ) ) ;
#123354=CARTESIAN_POINT ( 'NONE',  ( -5.981082042284069367, 7.006959133200059142, 1.199719254218452935 ) ) ;
#123356=VERTEX_POINT ( 'NONE', #206063 ) ;
#123362=CARTESIAN_POINT ( 'NONE',  ( 5.980555156959511898, 9.991415093179179863, -0.7216878364870458196 ) ) ;
#123369=CARTESIAN_POINT ( 'NONE',  ( -4.467832636417345071, 7.566084030862750609, 0.9469059386725534599 ) ) ;
#123373=CARTESIAN_POINT ( 'NONE',  ( 4.050854035433010480, 7.948023151305657841, 0.000000000000000000 ) ) ;
#123381=CARTESIAN_POINT ( 'NONE',  ( 4.850785098639300408, 8.881276058379668825, -0.7998128361456481317 ) ) ;
#123383=CARTESIAN_POINT ( 'NONE',  ( 5.182959862174088883, 9.268813282503625572, 0.7998128361456331437 ) ) ;
#123390=ADVANCED_FACE ( 'NONE', ( #91286 ), #56631, .F. ) ;
#123397=CARTESIAN_POINT ( 'NONE',  ( 6.486339200172205999, 6.751434215916642501, 0.1376000389162572446 ) ) ;
#123399=CARTESIAN_POINT ( 'NONE',  ( 4.584065335196261692, 7.401807753487379848, 1.082531754730549078 ) ) ;
#123406=CARTESIAN_POINT ( 'NONE',  ( -4.995253251992230581, 4.792493313604505367, 0.000000000000000000 ) ) ;
#123412=CIRCLE ( 'NONE', #54051, 7.424569270082293393 ) ;
#123418=CARTESIAN_POINT ( 'NONE',  ( -5.763624699140894592, 5.896852701852039580, -0.7216878364870338292 ) ) ;
#123423=CARTESIAN_POINT ( 'NONE',  ( 7.018280793729500644, 8.217024343219755167, -1.199719254218452047 ) ) ;
#123424=CARTESIAN_POINT ( 'NONE',  ( 4.779848517908583894, 4.883929213520019630, -0.7538207499340529028 ) ) ;
#123440=CARTESIAN_POINT ( 'NONE',  ( 6.343235766347262938, 8.493804042195527870, -1.599625672291281386 ) ) ;
#123460=CARTESIAN_POINT ( 'NONE',  ( -4.938913097128142304, 8.984092056616635347, -0.7998128361456362523 ) ) ;
#123464=CARTESIAN_POINT ( 'NONE',  ( -6.492003545397249553, 6.763960095814848472, -0.1687977717132038147 ) ) ;
#123481=CARTESIAN_POINT ( 'NONE',  ( 4.584065335196271462, 5.481069324884694005, 1.082531754730549078 ) ) ;
#123491=CARTESIAN_POINT ( 'NONE',  ( -3.363831509966360489, 6.938570838353784076, -0.7216878364870458196 ) ) ;
#123495=CARTESIAN_POINT ( 'NONE',  ( 5.586571952581918410, 5.815697052094486175, 0.6573761775866425738 ) ) ;
#123501=CARTESIAN_POINT ( 'NONE',  ( -6.414416072596883289, 6.656109304217317835, -0.7216878364870141782 ) ) ;
#123510=ADVANCED_FACE ( 'NONE', ( #26245 ), #155202, .F. ) ;
#123522=CARTESIAN_POINT ( 'NONE',  ( 3.555981428534177091, 7.370671776590375757, 0.7998128361456271485 ) ) ;
#123524=DIRECTION ( 'NONE',  ( -1.000000000000000000, -0.000000000000000000, -0.000000000000000000 ) ) ;
#123533=CARTESIAN_POINT ( 'NONE',  ( -5.302647476720585118, 9.200522799567075083, 0.000000000000000000 ) ) ;
#123535=CARTESIAN_POINT ( 'NONE',  ( 7.713663051532233972, 7.963971413067895355, -0.7998128361456341429 ) ) ;
#123552=CARTESIAN_POINT ( 'NONE',  ( -4.258669648468323743, 6.061810238003387141, 1.443375672974065660 ) ) ;
#123556=CARTESIAN_POINT ( 'NONE',  ( -5.983791420057156252, 7.107340751733106643, 1.079986564815892613 ) ) ;
#123579=FACE_OUTER_BOUND ( 'NONE', #29833, .T. ) ;
#123583=CARTESIAN_POINT ( 'NONE',  ( -6.851666526859749418, 9.086973262793417661, -1.599625672291271394 ) ) ;
#123586=CARTESIAN_POINT ( 'NONE',  ( -4.613517410400161722, 8.604463755433990002, -0.7998128361456362523 ) ) ;
#123591=CARTESIAN_POINT ( 'NONE',  ( -5.926322542504864899, 8.967774495347393682, -1.082531754730549967 ) ) ;
#123592=CARTESIAN_POINT ( 'NONE',  ( 7.973603738168424826, 8.475161580717541554, 0.000000000000000000 ) ) ;
#123598=CARTESIAN_POINT ( 'NONE',  ( -7.910256278930404505, 8.193330178365746619, -0.7998128361456362523 ) ) ;
#123603=ORIENTED_EDGE ( 'NONE', *, *, #59652, .F. ) ;
#123607=CARTESIAN_POINT ( 'NONE',  ( -5.759181390754928742, 9.941071732514568993, 0.000000000000000000 ) ) ;
#123609=CARTESIAN_POINT ( 'NONE',  ( 5.488371254093075358, 7.473176909139983337, -1.250075884424824757 ) ) ;
#123612=CARTESIAN_POINT ( 'NONE',  ( 4.492294583948199360, 8.028511867738709284, 2.499999999999656719 ) ) ;
#123614=CARTESIAN_POINT ( 'NONE',  ( 5.408776937209000657, 5.274937613024121674, 0.7998128361456352531 ) ) ;
#123624=CARTESIAN_POINT ( 'NONE',  ( -7.910256278930404505, 8.193330178365746619, -0.7998128361456362523 ) ) ;
#123637=CARTESIAN_POINT ( 'NONE',  ( 7.666209513884374438, 7.908608952478760834, 0.7998128361456281477 ) ) ;
#123653=CARTESIAN_POINT ( 'NONE',  ( 6.587573780899039555, 6.778200402807202707, -0.2451836268814889253 ) ) ;
#123654=CARTESIAN_POINT ( 'NONE',  ( -4.407809337774280856, 7.196175756495025055, 1.082531754730549967 ) ) ;
#123680=CARTESIAN_POINT ( 'NONE',  ( 4.634908411025333130, 6.500755460986618495, 1.599625672291268286 ) ) ;
#123682=FACE_OUTER_BOUND ( 'NONE', #58238, .T. ) ;
#123699=CARTESIAN_POINT ( 'NONE',  ( -6.954406449166956605, 7.078172043641714595, -0.7998128361456362523 ) ) ;
#123714=CARTESIAN_POINT ( 'NONE',  ( 5.761288931164342486, 5.686201605971993978, -0.7998128361456481317 ) ) ;
#123715=EDGE_CURVE ( 'NONE', #12133, #45181, #119081, .T. ) ;
#123717=CARTESIAN_POINT ( 'NONE',  ( 7.973603738168424826, 8.475161580717541554, 0.000000000000000000 ) ) ;
#123723=CARTESIAN_POINT ( 'NONE',  ( 4.781538967055604772, 8.149846084806789293, 0.7984123896064146964 ) ) ;
#123726=CARTESIAN_POINT ( 'NONE',  ( 5.748548729368831545, 7.266256959964179529, 1.200940202139972435 ) ) ;
#123745=CARTESIAN_POINT ( 'NONE',  ( -6.005335696210345020, 5.970922831858983315, 0.7998128361456281477 ) ) ;
#123747=CARTESIAN_POINT ( 'NONE',  ( 4.736594563127852098, 6.619389305106191834, -1.599625672291273171 ) ) ;
#123750=CARTESIAN_POINT ( 'NONE',  ( -5.692444392891315097, 7.734547439830227411, -1.599625672291271394 ) ) ;
#123753=CARTESIAN_POINT ( 'NONE',  ( 6.363572996767764778, 8.517530811019446091, -1.599625672291283607 ) ) ;
#123759=CARTESIAN_POINT ( 'NONE',  ( -4.638114411034067963, 8.432649648999159808, -0.4721908680582111995 ) ) ;
#123769=CARTESIAN_POINT ( 'NONE',  ( -4.543390873910949423, 6.393985001019784953, 1.443375672974058777 ) ) ;
#123777=CARTESIAN_POINT ( 'NONE',  ( 4.394251184604957672, 8.140727125432173139, -0.7216878364870357165 ) ) ;
#123782=CARTESIAN_POINT ( 'NONE',  ( -7.208094944320834863, 8.438474185576302133, -1.199719254218452047 ) ) ;
#123792=CARTESIAN_POINT ( 'NONE',  ( -4.014622883422336308, 5.777089012116397804, -1.443375672974066548 ) ) ;
#123823=CARTESIAN_POINT ( 'NONE',  ( -5.261973015879593873, 8.192700047617899273, 1.082531754730549967 ) ) ;
#123840=CARTESIAN_POINT ( 'NONE',  ( -4.009193028827814587, 7.297902834095492786, -0.7581239365674132813 ) ) ;
#123847=CARTESIAN_POINT ( 'NONE',  ( -4.624739795592948788, 5.528522862014106920, -1.082531754730549967 ) ) ;
#123852=CARTESIAN_POINT ( 'NONE',  ( -4.767627293860968507, 5.591261926706423857, -1.199719254218453823 ) ) ;
#123860=CARTESIAN_POINT ( 'NONE',  ( -2.844178363816758814, 6.540234867753325076, -0.7998128361456481317 ) ) ;
#123862=CARTESIAN_POINT ( 'NONE',  ( 6.604365638557201379, 6.767254738080503706, -0.09251035838216993545 ) ) ;
#123866=CARTESIAN_POINT ( 'NONE',  ( 5.499767588998890844, 6.445425604367387429, 1.199719254218451159 ) ) ;
#123871=CARTESIAN_POINT ( 'NONE',  ( -6.936931872047518155, 8.122117267924091166, 1.199719254218452047 ) ) ;
#123874=VECTOR ( 'NONE', #103668, 1000.000000000000000 ) ;
#123877=CARTESIAN_POINT ( 'NONE',  ( -3.851398154733808088, 6.650992392901508232, -1.199719254218450271 ) ) ;
#123882=CARTESIAN_POINT ( 'NONE',  ( 5.682275777458851707, 6.762314840857718501, 1.082531754730549078 ) ) ;
#123883=CARTESIAN_POINT ( 'NONE',  ( -4.570507181138272479, 7.385989907086349504, 1.082531754730549967 ) ) ;
#123886=CARTESIAN_POINT ( 'NONE',  ( -5.984998465789844069, 5.947196063035064206, 0.7998128361456282587 ) ) ;
#123889=CARTESIAN_POINT ( 'NONE',  ( 3.040771591214902259, 6.769593633051179005, -0.7998128361456362523 ) ) ;
#123893=DIRECTION ( 'NONE',  ( 0.7592566023653005702, 0.6507913734559640506, 0.000000000000000000 ) ) ;
#123896=DIRECTION ( 'NONE',  ( -0.7592566023653003482, 0.6507913734559641616, 0.000000000000000000 ) ) ;
#123900=CARTESIAN_POINT ( 'NONE',  ( 5.307274686206796765, 7.744096871513173497, 1.304404211447189876 ) ) ;
#123911=CARTESIAN_POINT ( 'NONE',  ( 6.119526231721748033, 8.232809585132461194, 1.599625672291269396 ) ) ;
#123922=CARTESIAN_POINT ( 'NONE',  ( 6.353009478083933459, 6.838182937092724956, 0.6209923359970755952 ) ) ;
#123929=CARTESIAN_POINT ( 'NONE',  ( 7.018280793729500644, 8.217024343219755167, -1.199719254218452047 ) ) ;
#123933=CARTESIAN_POINT ( 'NONE',  ( -4.767604096130494185, 8.184890741402179870, -0.7573865900243268445 ) ) ;
#123939=CARTESIAN_POINT ( 'NONE',  ( -5.772739544368596043, 9.956889578397179363, -0.7998128361456362523 ) ) ;
#123951=CARTESIAN_POINT ( 'NONE',  ( 7.147083253059300922, 8.367293879104554577, 1.199719254218452935 ) ) ;
#123960=CARTESIAN_POINT ( 'NONE',  ( 5.076602173674213070, 4.887400388900169368, 0.000000000000000000 ) ) ;
#123962=CARTESIAN_POINT ( 'NONE',  ( 5.533136087708556694, 5.627949321847663278, 0.000000000000000000 ) ) ;
#123971=CARTESIAN_POINT ( 'NONE',  ( -3.719872605471121751, 6.605953636083950364, 2.499999999999999556 ) ) ;
#123977=CARTESIAN_POINT ( 'NONE',  ( -6.861835142292179057, 9.098836647464588978, 1.443375672974064550 ) ) ;
#123978=CARTESIAN_POINT ( 'NONE',  ( 6.617788377246179188, 8.814115421577600529, -1.443375672974078761 ) ) ;
#123990=CARTESIAN_POINT ( 'NONE',  ( -3.935609729716867289, 7.813571461303467913, 0.7998128361456352531 ) ) ;
#123991=CARTESIAN_POINT ( 'NONE',  ( -5.822300622425855110, 5.757381912443740646, 0.7998128361456281477 ) ) ;
#123992=CARTESIAN_POINT ( 'NONE',  ( 7.526184668917440312, 8.913541880892736913, -1.082531754730548412 ) ) ;
#123994=EDGE_LOOP ( 'NONE', ( #74460, #196379, #76317, #99441, #95446 ) ) ;
#123999=DIRECTION ( 'NONE',  ( -0.5620411653108546846, 0.8271092603133013421, 3.252606517456488690E-14 ) ) ;
#124004=CARTESIAN_POINT ( 'NONE',  ( -5.432786300537782331, 7.535064667520821047, -1.248352293942560642 ) ) ;
#124007=CARTESIAN_POINT ( 'NONE',  ( 3.906157654512984134, 7.571284673658201569, -0.7216878364870338292 ) ) ;
#124012=CARTESIAN_POINT ( 'NONE',  ( -6.903036488013351679, 8.082572653217566128, -1.199719254218452047 ) ) ;
#124020=CARTESIAN_POINT ( 'NONE',  ( -5.398914348987532641, 6.259949555863199677, -2.420000000000000373 ) ) ;
#124027=CARTESIAN_POINT ( 'NONE',  ( 4.366607992053101128, 7.252070536440704096, -1.199719254218448494 ) ) ;
#124065=CARTESIAN_POINT ( 'NONE',  ( 5.994113311017540191, 9.046863725278862844, -1.082531754730548412 ) ) ;
#124069=CARTESIAN_POINT ( 'NONE',  ( 0.000000000000000000, 9.999999999999998224, 0.000000000000000000 ) ) ;
#124070=CARTESIAN_POINT ( 'NONE',  ( 5.655159470231527763, 9.611786791996525636, -0.7216878364870458196 ) ) ;
#124096=CARTESIAN_POINT ( 'NONE',  ( -4.679499295372141709, 5.488445928469455559, 1.199719254218452935 ) ) ;
#124098=CARTESIAN_POINT ( 'NONE',  ( 4.868786560638885597, 7.733982516503781213, 1.082531754730548412 ) ) ;
#124105=CARTESIAN_POINT ( 'NONE',  ( -4.034433228518296666, 6.864533312316751790, -1.199719254218450271 ) ) ;
#124110=CARTESIAN_POINT ( 'NONE',  ( -7.431277594066160397, 7.842447745931541370, -0.7216878364870338292 ) ) ;
#124117=CARTESIAN_POINT ( 'NONE',  ( -4.821859908315634158, 5.654533310236863564, 1.199719254218452935 ) ) ;
#124127=CARTESIAN_POINT ( 'NONE',  ( -2.810282979782591006, 6.500690253046801814, 0.000000000000000000 ) ) ;
#124130=CARTESIAN_POINT ( 'NONE',  ( -5.234856708652269042, 7.200695141551334721, 1.443375672974058777 ) ) ;
#124132=CARTESIAN_POINT ( 'NONE',  ( -6.007671464186866928, 8.102312356341712984, 1.443375672974058777 ) ) ;
#124133=CARTESIAN_POINT ( 'NONE',  ( 6.561219994370630637, 6.619454513046008515, 0.000000000000000000 ) ) ;
#124134=CARTESIAN_POINT ( 'NONE',  ( -4.471156797456668386, 8.438376373666578445, -0.7998128361456362523 ) ) ;
#124154=CARTESIAN_POINT ( 'NONE',  ( 7.713663051532233972, 7.963971413067895355, -0.7998128361456341429 ) ) ;
#124161=AXIS2_PLACEMENT_3D ( 'NONE', #122984, #156464, #91475 ) ;
#124190=CARTESIAN_POINT ( 'NONE',  ( 3.725458348705031231, 7.568394850123006279, -1.734723475976807094E-15 ) ) ;
#124191=CARTESIAN_POINT ( 'NONE',  ( 6.387299765813869712, 6.624473612970537495, 0.000000000000000000 ) ) ;
#124193=CARTESIAN_POINT ( 'NONE',  ( -3.492107083971660586, 6.231819477012331632, 1.199719254218452935 ) ) ;
#124196=CARTESIAN_POINT ( 'NONE',  ( -5.546694241322218666, 8.524874810634301525, 1.082531754730550855 ) ) ;
#124208=CARTESIAN_POINT ( 'NONE',  ( 3.464990776744291345, 6.200183785247111778, 1.199719254218452047 ) ) ;
#124209=CARTESIAN_POINT ( 'NONE',  ( 6.879836604291781121, 6.991173891287354003, -0.7998128361456341429 ) ) ;
#124220=EDGE_LOOP ( 'NONE', ( #114373, #48117, #2917, #140337 ) ) ;
#124221=CARTESIAN_POINT ( 'NONE',  ( 3.576318658954677598, 7.394398545414291313, 0.7998128361456281477 ) ) ;
#124223=ORIENTED_EDGE ( 'NONE', *, *, #193855, .T. ) ;
#124229=DIRECTION ( 'NONE',  ( 0.000000000000000000, 0.000000000000000000, -1.000000000000000000 ) ) ;
#124232=CARTESIAN_POINT ( 'NONE',  ( 7.187230829020129441, 8.518095734345896730, 1.082531754730549967 ) ) ;
#124233=CARTESIAN_POINT ( 'NONE',  ( -5.506019780925599960, 5.596313630600862510, 0.7216878364870257245 ) ) ;
#124234=CARTESIAN_POINT ( 'NONE',  ( -6.505933609711270549, 8.683618192786854095, -1.599625672291271394 ) ) ;
#124244=CARTESIAN_POINT ( 'NONE',  ( 6.505933609711257226, 8.683618192786854095, -1.599625672291281386 ) ) ;
#124246=CARTESIAN_POINT ( 'NONE',  ( 6.066347387471824781, 6.042103138330730872, -0.7998128361456481317 ) ) ;
#124247=CARTESIAN_POINT ( 'NONE',  ( 5.677832469072920496, 9.846164657218904992, 0.000000000000000000 ) ) ;
#124250=CARTESIAN_POINT ( 'NONE',  ( 7.472478939787284169, 8.746922180287201698, 1.199719254218452935 ) ) ;
#124265=EDGE_LOOP ( 'NONE', ( #171186, #79075, #8644, #214288, #44876 ) ) ;
#124266=AXIS2_PLACEMENT_3D ( 'NONE', #51959, #202432, #83365 ) ;
#124269=CARTESIAN_POINT ( 'NONE',  ( 5.910428620914669473, 5.860197910680708944, 0.000000000000000000 ) ) ;
#124273=CARTESIAN_POINT ( 'NONE',  ( 5.899733120602060232, 6.912052057904395141, -1.199719254218452047 ) ) ;
#124278=CARTESIAN_POINT ( 'NONE',  ( 3.061108821635398769, 6.793320401875094561, -0.7998128361456362523 ) ) ;
#124282=CARTESIAN_POINT ( 'NONE',  ( 6.726253606155519371, 7.019919760035800316, -0.7216878364870458196 ) ) ;
#124285=CARTESIAN_POINT ( 'NONE',  ( -4.118644803501354978, 8.027112380718707030, 0.7998128361456352531 ) ) ;
#124286=CARTESIAN_POINT ( 'NONE',  ( 4.095444919779759552, 6.935713618788495793, 1.199719254218451159 ) ) ;
#124296=CARTESIAN_POINT ( 'NONE',  ( -5.334207092333882017, 5.187939460669764635, 0.7998128361456281477 ) ) ;
#124330=CARTESIAN_POINT ( 'NONE',  ( 7.842465510862060896, 8.114240948952696542, 0.000000000000000000 ) ) ;
#124331=CARTESIAN_POINT ( 'NONE',  ( 4.299344108864946890, 6.109263775132799168, -1.443375672974068769 ) ) ;
#124344=CARTESIAN_POINT ( 'NONE',  ( -5.960744811863571968, 6.983232364376142698, 1.199719254218452935 ) ) ;
#124346=CARTESIAN_POINT ( 'NONE',  ( 5.655159470231527763, 9.611786791996525636, -0.7216878364870458196 ) ) ;
#124356=CARTESIAN_POINT ( 'NONE',  ( -4.447956913735107598, 7.346977611736363656, 1.199719254218452935 ) ) ;
#124357=( GEOMETRIC_REPRESENTATION_CONTEXT ( 3 ) GLOBAL_UNCERTAINTY_ASSIGNED_CONTEXT ( ( #177282 ) ) GLOBAL_UNIT_ASSIGNED_CONTEXT ( ( #210372, #133438, #83575 ) ) REPRESENTATION_CONTEXT ( 'NONE', 'WORKASPACE' ) );
#124363=CARTESIAN_POINT ( 'NONE',  ( -3.024877669624710386, 6.543124691288523920, 0.000000000000000000 ) ) ;
#124367=CARTESIAN_POINT ( 'NONE',  ( -5.483346782084204563, 5.361935765378481378, 0.000000000000000000 ) ) ;
#124376=ADVANCED_FACE ( 'NONE', ( #169342 ), #103843, .T. ) ;
#124388=CARTESIAN_POINT ( 'NONE',  ( -5.444481204339554736, 8.509589284108232121, 1.199719254218454489 ) ) ;
#124398=B_SPLINE_CURVE_WITH_KNOTS ( 'NONE', 3,
 ( #139042, #24182, #152079, #88141 ),
 .UNSPECIFIED., .F., .F.,
 ( 4, 4 ),
 ( 0.5002441414044666024, 0.5750605836579747443 ),
 .UNSPECIFIED. ) ;
#124415=CARTESIAN_POINT ( 'NONE',  ( -4.294900800479008574, 8.232744377192641849, 0.000000000000000000 ) ) ;
#124442=CARTESIAN_POINT ( 'NONE',  ( 6.550524494058025837, 7.671308660269694712, -1.199719254218452047 ) ) ;
#124445=CARTESIAN_POINT ( 'NONE',  ( 6.261886844665240481, 8.398896966899865646, 1.599625672291268286 ) ) ;
#124457=CARTESIAN_POINT ( 'NONE',  ( 6.426609430950597890, 6.789993649951097332, 0.4362094596595481599 ) ) ;
#124459=CARTESIAN_POINT ( 'NONE',  ( 6.373741612200174878, 6.608655767087927124, 0.7216878364870328300 ) ) ;
#124467=CARTESIAN_POINT ( 'NONE',  ( -4.930325137224961907, 5.781076077297750970, -1.199719254218453823 ) ) ;
#124469=ORIENTED_EDGE ( 'NONE', *, *, #82621, .F. ) ;
#124477=CARTESIAN_POINT ( 'NONE',  ( -5.709392084686210289, 8.714688961225625974, 1.082531754730550855 ) ) ;
#124496=CARTESIAN_POINT ( 'NONE',  ( 5.993586425693011144, 9.150212042353954800, -1.199719254218452047 ) ) ;
#124514=CARTESIAN_POINT ( 'NONE',  ( -6.424584688029276514, 8.588711117491191871, 1.599625672291269396 ) ) ;
#124519=CARTESIAN_POINT ( 'NONE',  ( -6.490830876026181251, 6.764709549658621590, 0.1777360701797660314 ) ) ;
#124528=CARTESIAN_POINT ( 'NONE',  ( -5.000000000000013323, 8.499999999999996447, 0.7750000000000004663 ) ) ;
#124538=CARTESIAN_POINT ( 'NONE',  ( 4.733205024946604667, 8.536173272497439513, 0.000000000000000000 ) ) ;
#124539=EDGE_LOOP ( 'NONE', ( #102798, #185950, #78308, #106305 ) ) ;
#124549=CARTESIAN_POINT ( 'NONE',  ( -3.350273356352693188, 6.922752992471175482, 0.000000000000000000 ) ) ;
#124554=CARTESIAN_POINT ( 'NONE',  ( 4.699688308863886554, 8.280832412640696916, 0.6266364797024156497 ) ) ;
#124569=CARTESIAN_POINT ( 'NONE',  ( 3.147653791585693028, 8.920000000000001705, 2.419999999999999485 ) ) ;
#124579=CARTESIAN_POINT ( 'NONE',  ( 5.740951700743842423, 5.662474837148078421, -0.7998128361456481317 ) ) ;
#124590=CARTESIAN_POINT ( 'NONE',  ( -5.316205630334251531, 9.216340645449683677, -0.7216878364870338292 ) ) ;
#124594=CARTESIAN_POINT ( 'NONE',  ( 5.221298554594243413, 5.264138866547622975, -0.7216878364870458196 ) ) ;
#124611=CARTESIAN_POINT ( 'NONE',  ( 4.415115299905642665, 5.179997933758551554, -1.199719254218450271 ) ) ;
#124613=CARTESIAN_POINT ( 'NONE',  ( 3.947104627881618200, 8.980740528188865923, 0.7749999999999996891 ) ) ;
#124635=B_SPLINE_CURVE_WITH_KNOTS ( 'NONE', 3,
 ( #131822, #146990, #197831, #48420, #133949, #213008, #100339, #66732, #49464, #180526 ),
 .UNSPECIFIED., .F., .F.,
 ( 4, 3, 3, 4 ),
 ( 1.970267125075963426E-17, 3.125277950706723017E-05, 6.250528927673665086E-05, 0.0001035880062255934710 ),
 .UNSPECIFIED. ) ;
#124644=CARTESIAN_POINT ( 'NONE',  ( -5.447343857640614573, 9.577261277214532242, -0.7998128361456362523 ) ) ;
#124647=CARTESIAN_POINT ( 'NONE',  ( -4.450819567036169211, 8.414649604842665553, -0.7998128361456362523 ) ) ;
#124648=CARTESIAN_POINT ( 'NONE',  ( -5.818384198920079520, 6.817144982608731141, 1.199719254218452935 ) ) ;
#124649=CARTESIAN_POINT ( 'NONE',  ( -4.624015273241393942, 8.365221982611680929, 0.3117065211258822077 ) ) ;
#124650=ORIENTED_EDGE ( 'NONE', *, *, #25859, .T. ) ;
#124652=CARTESIAN_POINT ( 'NONE',  ( -5.709392084686210289, 8.714688961225625974, 1.082531754730550855 ) ) ;
#124655=CARTESIAN_POINT ( 'NONE',  ( -4.167152111353897403, 5.955039778036558040, 1.599625672291270506 ) ) ;
#124658=CARTESIAN_POINT ( 'NONE',  ( -4.679499295372141709, 5.488445928469455559, 1.199719254218452935 ) ) ;
#124666=CARTESIAN_POINT ( 'NONE',  ( -7.553827861469316396, 8.841829255582865699, -1.199719254218452047 ) ) ;
#124668=CARTESIAN_POINT ( 'NONE',  ( 4.915098833515745724, 8.004322973991836676, -0.9888141558981374812 ) ) ;
#124672=CARTESIAN_POINT ( 'NONE',  ( 7.075376061485196821, 9.347967719856493218, 1.599625672291268286 ) ) ;
#124693=CARTESIAN_POINT ( 'NONE',  ( 7.693325821111733021, 7.940244644243982464, -0.7998128361456341429 ) ) ;
#124707=CARTESIAN_POINT ( 'NONE',  ( -3.719872605471121751, 6.605953636083950364, 2.499999999999999556 ) ) ;
#124708=CARTESIAN_POINT ( 'NONE',  ( 6.576141308597898139, 6.785670920958930985, -0.3094590540993913952 ) ) ;
#124709=CARTESIAN_POINT ( 'NONE',  ( -5.953438849732214599, 6.118302544208584770, 0.7216878364870257245 ) ) ;
#124739=CARTESIAN_POINT ( 'NONE',  ( 3.203469434578891661, 6.959407783642502565, -0.7998128361456362523 ) ) ;
#124758=CARTESIAN_POINT ( 'NONE',  ( -6.143779885648060102, 7.196773283791382703, 1.199719254218452047 ) ) ;
#124769=ORIENTED_EDGE ( 'NONE', *, *, #177718, .F. ) ;
#124773=CARTESIAN_POINT ( 'NONE',  ( 3.953084306836263995, 6.769626237021087789, 1.199719254218452047 ) ) ;
#124782=CARTESIAN_POINT ( 'NONE',  ( 4.811213433158714636, 8.116601557201025940, 0.8487219550047861993 ) ) ;
#124784=CARTESIAN_POINT ( 'NONE',  ( 4.954704567260191261, 7.963257648925383236, 1.029694947009308859 ) ) ;
#124785=CARTESIAN_POINT ( 'NONE',  ( 5.129297441109695654, 7.908270138404875027, 1.225875489271853302 ) ) ;
#124805=CARTESIAN_POINT ( 'NONE',  ( -5.991777542596674166, 5.955104985976372944, 0.000000000000000000 ) ) ;
#124807=CARTESIAN_POINT ( 'NONE',  ( 4.980641328173811999, 6.904110530993182948, 1.599625672291269396 ) ) ;
#124809=CARTESIAN_POINT ( 'NONE',  ( -6.180537922983287302, 8.303989891604203422, -1.599625672291271394 ) ) ;
#124815=CARTESIAN_POINT ( 'NONE',  ( -4.882431421883429046, 8.154724402237897962, -1.012048471081774093 ) ) ;
#124823=DIRECTION ( 'NONE',  ( -0.2636425362803287986, 0.9646204502620061572, 0.000000000000000000 ) ) ;
#124830=CARTESIAN_POINT ( 'NONE',  ( 6.075462232699553766, 6.260663157670496304, -0.7216878364870458196 ) ) ;
#124834=CARTESIAN_POINT ( 'NONE',  ( -5.088052786878465739, 9.158088361325352977, 0.000000000000000000 ) ) ;
#124849=CARTESIAN_POINT ( 'NONE',  ( 5.896870467300973750, 5.844380064798101237, 0.7998128361456352531 ) ) ;
#124852=B_SPLINE_CURVE_WITH_KNOTS ( 'NONE', 3,
 ( #88695, #54050, #21507, #5256, #71332, #163026, #160887, #14609, #159812, #111131 ),
 .UNSPECIFIED., .F., .F.,
 ( 4, 2, 2, 2, 4 ),
 ( 0.000000000000000000, 0.0003432858056828389979, 0.0006865716113656779957, 0.001029857417048516939, 0.001373143222731355991 ),
 .UNSPECIFIED. ) ;
#124878=CARTESIAN_POINT ( 'NONE',  ( -6.048345925472225382, 8.149765894507963182, 1.443375672974058777 ) ) ;
#124904=CARTESIAN_POINT ( 'NONE',  ( -6.583366107887490770, 9.838288338247510367, 1.199719254218452935 ) ) ;
#124909=CARTESIAN_POINT ( 'NONE',  ( -3.800028193580205382, 7.655393002477360653, -0.7998128361456481317 ) ) ;
#124919=CARTESIAN_POINT ( 'NONE',  ( -4.085803189671902480, 5.860132702740892263, -1.599625672291271394 ) ) ;
#124921=CARTESIAN_POINT ( 'NONE',  ( 5.862225131719664972, 7.287605523280396902, -1.268052015211480033 ) ) ;
#124926=CARTESIAN_POINT ( 'NONE',  ( 6.052789233858158369, 6.026285292448116948, 0.000000000000000000 ) ) ;
#124931=CARTESIAN_POINT ( 'NONE',  ( -7.587723245503481095, 8.881373870289390737, 1.199719254218452047 ) ) ;
#124935=CARTESIAN_POINT ( 'NONE',  ( -4.878955176071358757, 6.785476686873604280, -1.599625672291271394 ) ) ;
#124942=CARTESIAN_POINT ( 'NONE',  ( 4.543390873910894356, 8.314723429622471684, 0.7216878364870317197 ) ) ;
#124943=CARTESIAN_POINT ( 'NONE',  ( -3.797692425159308716, 7.444741906078900406, 0.000000000000000000 ) ) ;
#124949=CARTESIAN_POINT ( 'NONE',  ( 3.379725431556547477, 7.165039780116438273, -1.734723475976807094E-15 ) ) ;
#124957=CARTESIAN_POINT ( 'NONE',  ( 5.285699784481295183, 7.260012063351913625, 1.599625672291268286 ) ) ;
#124979=CARTESIAN_POINT ( 'NONE',  ( 4.594747986498664005, 8.374059380672374431, -0.03693212167796278145 ) ) ;
#124988=CARTESIAN_POINT ( 'NONE',  ( 5.559725510055676168, 8.644040974110419384, 1.199719254218451159 ) ) ;
#124992=CARTESIAN_POINT ( 'NONE',  ( -4.604539980425653489, 8.383423159197839425, -0.07723066608773809794 ) ) ;
#125000=CARTESIAN_POINT ( 'NONE',  ( -5.420227550413282636, 9.545625585449309725, 0.7998128361456291469 ) ) ;
#125013=CARTESIAN_POINT ( 'NONE',  ( 6.550524494058025837, 7.671308660269694712, -1.199719254218452047 ) ) ;
#125015=CIRCLE ( 'NONE', #31545, 0.08000000000000030698 ) ;
#125022=CARTESIAN_POINT ( 'NONE',  ( 5.228604516725597229, 6.129068686715179126, -1.199719254218450271 ) ) ;
#125026=CARTESIAN_POINT ( 'NONE',  ( 6.021229617800532452, 6.197391773621639288, 0.000000000000000000 ) ) ;
#125027=CARTESIAN_POINT ( 'NONE',  ( 0.1019944501368414136, 2.531386338185347640, -1.997494965961774005 ) ) ;
#125035=EDGE_CURVE ( 'NONE', #179985, #170847, #178513, .T. ) ;
#125042=CARTESIAN_POINT ( 'NONE',  ( -4.878955176071358757, 6.785476686873604280, -1.599625672291271394 ) ) ;
#125043=CARTESIAN_POINT ( 'NONE',  ( 6.943184063974162434, 9.193743722760251202, -1.443375672974064550 ) ) ;
#125055=CARTESIAN_POINT ( 'NONE',  ( -6.784929528996132220, 6.880448970109080520, 0.000000000000000000 ) ) ;
#125056=CARTESIAN_POINT ( 'NONE',  ( -3.772911886352873445, 7.623757310712140800, 0.7998128361456352531 ) ) ;
#125058=CARTESIAN_POINT ( 'NONE',  ( 8.136301581532414673, 8.664975731308866003, 0.000000000000000000 ) ) ;
#125061=CARTESIAN_POINT ( 'NONE',  ( -2.974698719455045381, 6.690899969729074748, -0.05384663926280564006 ) ) ;
#125064=DIRECTION ( 'NONE',  ( 0.6507913734559641616, -0.7592566023653004592, 0.000000000000000000 ) ) ;
#125070=CARTESIAN_POINT ( 'NONE',  ( -6.127277117991962285, 7.006264510460848527, -0.9572512136472415278 ) ) ;
#125076=CARTESIAN_POINT ( 'NONE',  ( 5.587368702607580673, 5.691220705896524734, -0.7216878364870458196 ) ) ;
#125080=CARTESIAN_POINT ( 'NONE',  ( -5.433785704026946384, 9.561443431331920095, 0.000000000000000000 ) ) ;
#125093=CARTESIAN_POINT ( 'NONE',  ( 5.006703865196457492, 9.063181286029688977, 0.000000000000000000 ) ) ;
#125127=CARTESIAN_POINT ( 'NONE',  ( 5.668717624289557833, 8.667235424096215723, -1.082531754730548412 ) ) ;
#125132=CARTESIAN_POINT ( 'NONE',  ( 7.471952054462756010, 7.889901283060952508, 0.7216878364870267237 ) ) ;
#125133=B_SPLINE_CURVE_WITH_KNOTS ( 'NONE', 3,
 ( #146044, #147102, #61566, #45334, #163341, #177458, #95156, #12793, #78867, #96224 ),
 .UNSPECIFIED., .F., .F.,
 ( 4, 3, 3, 4 ),
 ( 0.000000000000000000, 0.0001748932287411561373, 0.0003221082053133044300, 0.0004700044474451332398 ),
 .UNSPECIFIED. ) ;
#125157=CARTESIAN_POINT ( 'NONE',  ( -5.276058054373441664, 6.184431147304315424, -1.199719254218453823 ) ) ;
#125159=CARTESIAN_POINT ( 'NONE',  ( 6.346625304528514810, 6.577020074804287297, 0.000000000000000000 ) ) ;
#125164=CARTESIAN_POINT ( 'NONE',  ( -6.303615075710993665, 6.318915441276411471, -0.7998128361456362523 ) ) ;
#125169=CARTESIAN_POINT ( 'NONE',  ( -4.995253251992230581, 4.792493313604505367, 0.000000000000000000 ) ) ;
#125175=CARTESIAN_POINT ( 'NONE',  ( -3.949167883330528372, 7.829389307186077396, 1.214306433183764966E-14 ) ) ;
#125182=EDGE_CURVE ( 'NONE', #127411, #135468, #32727, .T. ) ;
#125185=CARTESIAN_POINT ( 'NONE',  ( -5.971440312176176768, 5.931378217152456500, 0.000000000000000000 ) ) ;
#125188=CARTESIAN_POINT ( 'NONE',  ( -4.340018570150306232, 8.077455741901736985, -0.7216878364870338292 ) ) ;
#125189=CARTESIAN_POINT ( 'NONE',  ( -4.760321331729590710, 8.567808963744235839, 0.7216878364870267237 ) ) ;
#125190=CARTESIAN_POINT ( 'NONE',  ( 4.525389411911321602, 8.501647757197021704, -0.7998128361456381397 ) ) ;
#125191=CARTESIAN_POINT ( 'NONE',  ( -6.317173229324657413, 6.334733287159020954, 0.000000000000000000 ) ) ;
#125210=CARTESIAN_POINT ( 'NONE',  ( 6.003228155800906407, 10.22579295840155744, 0.000000000000000000 ) ) ;
#125217=CARTESIAN_POINT ( 'NONE',  ( -2.974698719455045381, 6.690899969729074748, -0.05384663926280564006 ) ) ;
#125233=CARTESIAN_POINT ( 'NONE',  ( 4.915098833515745724, 8.004322973991836676, -0.9888141558981374812 ) ) ;
#125241=CARTESIAN_POINT ( 'NONE',  ( 5.061565854856461932, 4.907682761174942065, 0.2605415071502180657 ) ) ;
#125249=CARTESIAN_POINT ( 'NONE',  ( 5.742760583840166966, 8.857581893525663830, 1.199719254218452047 ) ) ;
#125252=CARTESIAN_POINT ( 'NONE',  ( -5.164730172163054966, 4.990216387137135889, -0.7998128361456362523 ) ) ;
#125255=CARTESIAN_POINT ( 'NONE',  ( -6.089020385868850305, 10.11795786024005572, -0.7216878364870338292 ) ) ;
#125266=CARTESIAN_POINT ( 'NONE',  ( 5.273195401072370281, 5.116759154198018855, -0.7998128361456481317 ) ) ;
#125267=CARTESIAN_POINT ( 'NONE',  ( 6.540882763950133238, 6.595727744222092959, 0.000000000000000000 ) ) ;
#125279=CARTESIAN_POINT ( 'NONE',  ( 3.739016502318667445, 7.584212696005614873, 0.7998128361456271485 ) ) ;
#125291=CARTESIAN_POINT ( 'NONE',  ( 6.021229618244865023, 10.03886863134542828, -0.7216878364870458196 ) ) ;
#125293=CARTESIAN_POINT ( 'NONE',  ( -6.305950844131887223, 6.529566537674873494, 0.000000000000000000 ) ) ;
#125294=CARTESIAN_POINT ( 'NONE',  ( -5.399890319992785237, 9.521898816625391504, 0.7998128361456291469 ) ) ;
#125305=CARTESIAN_POINT ( 'NONE',  ( 4.681308178468477799, 8.683552984847038303, 0.000000000000000000 ) ) ;
#125306=CARTESIAN_POINT ( 'NONE',  ( 5.338878628731272613, 9.450718510153643948, -0.7998128361456481317 ) ) ;
#125309=CARTESIAN_POINT ( 'NONE',  ( 4.001064729364292916, 6.721640380016713934, -1.082531754730548412 ) ) ;
#125313=FACE_OUTER_BOUND ( 'NONE', #23020, .T. ) ;
#125327=CARTESIAN_POINT ( 'NONE',  ( 5.411639590510088027, 6.342609606130419131, -1.199719254218452047 ) ) ;
#125330=CARTESIAN_POINT ( 'NONE',  ( 4.929271367020211514, 7.908511140569038922, 1.199719254218452047 ) ) ;
#125334=CARTESIAN_POINT ( 'NONE',  ( 7.856023664475727308, 8.130058794835305136, -0.7998128361456341429 ) ) ;
#125339=CARTESIAN_POINT ( 'NONE',  ( 5.180624094197585627, 8.097792972322238825, -1.082531754730548412 ) ) ;
#125341=CARTESIAN_POINT ( 'NONE',  ( -5.981082042284069367, 7.006959133200059142, 1.199719254218452935 ) ) ;
#125342=CARTESIAN_POINT ( 'NONE',  ( 4.203910148689107729, 7.062256385849379647, -1.199719254218448494 ) ) ;
#125352=CARTESIAN_POINT ( 'NONE',  ( -5.984998465789844069, 5.947196063035064206, 0.7998128361456281477 ) ) ;
#125385=CARTESIAN_POINT ( 'NONE',  ( 7.506374323821472849, 8.786466794993730289, -1.199719254218452047 ) ) ;
#125386=CARTESIAN_POINT ( 'NONE',  ( 6.933015448541703485, 9.181880338089085214, 1.599625672291268286 ) ) ;
#125394=( BOUNDED_SURFACE ( )  B_SPLINE_SURFACE ( 1, 2, ( 
 ( #77120, #31591, #143243, #161597, #79264, #129176, #97666, #145381, #14230, #80325, #76063, #142162, #208179, #48903, #117150, #181020, #115023, #100830, #199381, #32640, #98717, #134444, #184206, #67242, #164776, #16366, #182068, #84588, #68313, #131275, #1178, #200447, #52093, #148534, #163724, #118220, #116078, #35829, #33700, #99777, #197263, #183153, #81392, #167972, #19578, #101907, #15304, #82444, #149594, #51028, #147477, #101, #213497, #66167, #65119, #132314, #198319, #165842, #2236, #49959, #17428, #83511, #166915, #133376, #34756, #18509, #150675, #112510, #193687, #178522, #63695, #126647, #161204, #143929, #110387, #14917, #164398, #29069, #12790, #114647, #177455, #62617, #192612, #97283, #128779, #13859, #208858, #78864, #47470, #130895, #129849, #144985, #45331, #64753, #180640, #96221, #194756, #127729, #179587, #113585, #46393, #111450, #30132, #94094, #196889, #27997, #60489, #176392, #162272, #163338, #95152, #61563, #44265, #31209, #79936, #210990, #146041, #212055, #195832, #81011, #147099, #160133, #209924, #213123, #15981, #48527, #142854, #32265, #98332, #11732, #77808, #70066, #148158, #117847, #783, #202197, #214159, #20263, #152418, #66850, #53853, #150295, #1862, #67923, #166528, #86347, #37595, #35448, #134067, #101528, #200076, #136179, #17049, #33320, #135119, #51725, #183839, #131935, #182765, #119986, #18119, #165454, #184893, #169726, #132994, #3997, #198995, #185963, #83128, #167597, #19196, #149208, #85274, #151361, #84207, #103678, #2930, #168658, #69002, #201135, #82066, #50641, #52773, #65785, #116767, #34382, #118910, #99401, #36517, #100455, #102604, #197946, #49573, #115698, #181690, #157766, #59175, #106928, #22387, #187037, #155622, #41895, #91717, #121069, #40820, #25605, #9366, #204328, #21315, #174033, #171867, #75437, #23461, #89573, #54918, #8292, #153489, #125334, #191297, #141549, #207556, #88496, #139384, #172953, #190236, #42965, #109073, #39735, #87422, #74375, #5059, #140477, #71134, #137252, #7207, #104748, #55986, #105840, #72205, #205417, #203272 ),
 ( #122138, #73280, #38669, #108006, #57055, #24532, #170796, #123219, #206489, #154557, #156700, #189183, #138313, #6136, #188105, #90640, #58119, #124278, #76483, #27742, #142594, #141540, #126394, #10411, #140467, #92770, #24521, #208603, #158815, #60234, #57044, #39725, #159876, #123210, #204319, #189171, #93837, #188093, #55977, #23451, #11481, #192354, #77552, #174024, #207548, #59167, #157758, #40811, #7198, #73271, #105831, #172943, #25594, #171856, #176142, #106919, #75429, #8281, #44011, #122130, #90631, #110131, #156691, #89563, #205405, #58110, #190227, #139374, #91707, #9355, #206480, #155613, #124269, #74365, #125327, #41886, #107997, #191288, #42954, #109064, #175080, #26666, #145800, #163090, #79688, #47218, #94898, #14671, #2401, #146854, #210749, #113334, #194503, #179341, #64507, #127472, #162024, #144739, #111195, #18674, #168139, #29886, #13615, #118384, #178276, #63444, #193443, #100993, #129596, #80765, #209668, #211806, #51196, #134607, #130651, #195583, #46149, #68480, #184372, #97038, #30963, #128534, #12540, #117318, #112262, #62372, #212874, #160950, #200611, #28814, #61311, #177199, #199552, #167083, #95970, #183315, #45086, #34920, #84753, #150840, #52258, #35992, #102073, #19740, #143675, #78614, #86890, #87956, #173504, #136719, #107478, #105296, #38143, #187578, #172417, #73841, #151899, #121608, #4531, #205963, #3474, #24006, #156174, #70605, #57595, #154030, #5596, #71677, #170263, #90108, #41367, #39205, #137790, #171332, #203810, #139936, #20794, #37060, #138859, #55455, #22927, #135650, #186512, #123753, #21849, #169201, #89042, #155099, #6683, #72760, #7754, #85820, #204874, #56529, #122690, #188652, #189715, #152955, #103142, #40284, #106393, #69543, #201673, #104216, #53320, #119453, #202744, #185440, #54396, #120536, #29365, #158307, #145286, #26147, #93319, #10953, #174571, #126948, #44562, #175626, #46694, #27213, #111744, #192905, #190773, #95460, #8834, #79170, #144228, #28290, #141020, #159355, #110677, #77026, #143156, #42435, #176677, #161509, #94384, #92261, #209150 ) ),
 .UNSPECIFIED., .F., .F., .T. ) 
 B_SPLINE_SURFACE_WITH_KNOTS ( ( 2, 2 ),
 ( 3, 2, 2, 2, 2, 2, 2, 2, 2, 2, 2, 2, 2, 2, 2, 2, 2, 2, 2, 2, 2, 2, 2, 2, 2, 2, 2, 2, 2, 2, 2, 2, 2, 2, 2, 2, 2, 2, 2, 2, 2, 2, 2, 2, 2, 2, 2, 2, 2, 2, 2, 2, 2, 2, 2, 2, 2, 2, 2, 2, 2, 2, 2, 2, 2, 2, 2, 2, 2, 2, 2, 2, 2, 2, 2, 2, 2, 2, 2, 2, 2, 2, 2, 2, 2, 2, 2, 2, 2, 2, 2, 2, 2, 2, 2, 2, 2, 2, 2, 2, 2, 2, 2, 2, 2, 2, 2, 2, 2, 2, 2, 2, 2, 2, 2, 2, 2, 2, 2, 2, 3 ),
 ( 0.000000000000000000, 1.000000000000000000 ),
 ( 0.000000000000000000, 0.008333333333333333218, 0.01666666666666666644, 0.02500000000000000139, 0.03333333333333333287, 0.04166666666666666435, 0.05000000000000000278, 0.05833333333333333426, 0.06666666666666666574, 0.07499999999999999722, 0.08333333333333332871, 0.09166666666666666019, 0.1000000000000000056, 0.1083333333333333370, 0.1166666666666666685, 0.1250000000000000000, 0.1333333333333333315, 0.1416666666666666630, 0.1499999999999999944, 0.1583333333333333259, 0.1666666666666666574, 0.1749999999999999889, 0.1833333333333333204, 0.1916666666666666796, 0.2000000000000000111, 0.2083333333333333426, 0.2166666666666666741, 0.2250000000000000056, 0.2333333333333333370, 0.2416666666666666685, 0.2500000000000000000, 0.2583333333333333592, 0.2666666666666666630, 0.2750000000000000222, 0.2833333333333333259, 0.2916666666666666852, 0.2999999999999999889, 0.3083333333333333481, 0.3166666666666666519, 0.3250000000000000111, 0.3333333333333333148, 0.3416666666666666741, 0.3499999999999999778, 0.3583333333333333370, 0.3666666666666666408, 0.3750000000000000000, 0.3833333333333333592, 0.3916666666666666630, 0.4000000000000000222, 0.4083333333333333259, 0.4166666666666666852, 0.4249999999999999889, 0.4333333333333333481, 0.4416666666666666519, 0.4500000000000000111, 0.4583333333333333148, 0.4666666666666666741, 0.4749999999999999778, 0.4833333333333333370, 0.4916666666666666408, 0.5000000000000000000, 0.5083333333333333037, 0.5166666666666667185, 0.5250000000000000222, 0.5333333333333333259, 0.5416666666666666297, 0.5500000000000000444, 0.5583333333333333481, 0.5666666666666666519, 0.5749999999999999556, 0.5833333333333333703, 0.5916666666666666741, 0.5999999999999999778, 0.6083333333333332815, 0.6166666666666666963, 0.6250000000000000000, 0.6333333333333333037, 0.6416666666666667185, 0.6500000000000000222, 0.6583333333333333259, 0.6666666666666666297, 0.6750000000000000444, 0.6833333333333333481, 0.6916666666666666519, 0.6999999999999999556, 0.7083333333333333703, 0.7166666666666666741, 0.7249999999999999778, 0.7333333333333332815, 0.7416666666666666963, 0.7500000000000000000, 0.7583333333333333037, 0.7666666666666667185, 0.7750000000000000222, 0.7833333333333333259, 0.7916666666666666297, 0.8000000000000000444, 0.8083333333333333481, 0.8166666666666666519, 0.8249999999999999556, 0.8333333333333333703, 0.8416666666666666741, 0.8499999999999999778, 0.8583333333333332815, 0.8666666666666666963, 0.8750000000000000000, 0.8833333333333333037, 0.8916666666666667185, 0.9000000000000000222, 0.9083333333333333259, 0.9166666666666666297, 0.9250000000000000444, 0.9333333333333333481, 0.9416666666666666519, 0.9499999999999999556, 0.9583333333333333703, 0.9666666666666666741, 0.9749999999999999778, 0.9833333333333332815, 0.9916666666666666963, 1.000000000000000000 ),
 .UNSPECIFIED. ) 
 GEOMETRIC_REPRESENTATION_ITEM ( )  RATIONAL_B_SPLINE_SURFACE ( (
 ( 1.000000000000000000, 0.8660254037844387076, 1.000000000000000000, 0.8660254037844387076, 1.000000000000000000, 0.8660254037844387076, 1.000000000000000000, 0.8660254037844387076, 1.000000000000000000, 0.8660254037844387076, 1.000000000000000000, 0.8660254037844387076, 1.000000000000000000, 0.8660254037844387076, 1.000000000000000000, 0.8660254037844387076, 1.000000000000000000, 0.8660254037844387076, 1.000000000000000000, 0.8660254037844387076, 1.000000000000000000, 0.8660254037844387076, 1.000000000000000000, 0.8660254037844387076, 1.000000000000000000, 0.8660254037844387076, 1.000000000000000000, 0.8660254037844387076, 1.000000000000000000, 0.8660254037844387076, 1.000000000000000000, 0.8660254037844387076, 1.000000000000000000, 0.8660254037844387076, 1.000000000000000000, 0.8660254037844387076, 1.000000000000000000, 0.8660254037844387076, 1.000000000000000000, 0.8660254037844387076, 1.000000000000000000, 0.8660254037844387076, 1.000000000000000000, 0.8660254037844387076, 1.000000000000000000, 0.8660254037844387076, 1.000000000000000000, 0.8660254037844387076, 1.000000000000000000, 0.8660254037844387076, 1.000000000000000000, 0.8660254037844387076, 1.000000000000000000, 0.8660254037844387076, 1.000000000000000000, 0.8660254037844387076, 1.000000000000000000, 0.8660254037844387076, 1.000000000000000000, 0.8660254037844387076, 1.000000000000000000, 0.8660254037844387076, 1.000000000000000000, 0.8660254037844387076, 1.000000000000000000, 0.8660254037844387076, 1.000000000000000000, 0.8660254037844387076, 1.000000000000000000, 0.8660254037844387076, 1.000000000000000000, 0.8660254037844387076, 1.000000000000000000, 0.8660254037844387076, 1.000000000000000000, 0.8660254037844387076, 1.000000000000000000, 0.8660254037844387076, 1.000000000000000000, 0.8660254037844387076, 1.000000000000000000, 0.8660254037844387076, 1.000000000000000000, 0.8660254037844387076, 1.000000000000000000, 0.8660254037844387076, 1.000000000000000000, 0.8660254037844387076, 1.000000000000000000, 0.8660254037844387076, 1.000000000000000000, 0.8660254037844387076, 1.000000000000000000, 0.8660254037844387076, 1.000000000000000000, 0.8660254037844387076, 1.000000000000000000, 0.8660254037844387076, 1.000000000000000000, 0.8660254037844387076, 1.000000000000000000, 0.8660254037844387076, 1.000000000000000000, 0.8660254037844387076, 1.000000000000000000, 0.8660254037844387076, 1.000000000000000000, 0.8660254037844387076, 1.000000000000000000, 0.8660254037844387076, 1.000000000000000000, 0.8660254037844387076, 1.000000000000000000, 0.8660254037844387076, 1.000000000000000000, 0.8660254037844387076, 1.000000000000000000, 0.8660254037844387076, 1.000000000000000000, 0.8660254037844387076, 1.000000000000000000, 0.8660254037844387076, 1.000000000000000000, 0.8660254037844387076, 1.000000000000000000, 0.8660254037844387076, 1.000000000000000000, 0.8660254037844387076, 1.000000000000000000, 0.8660254037844387076, 1.000000000000000000, 0.8660254037844387076, 1.000000000000000000, 0.8660254037844387076, 1.000000000000000000, 0.8660254037844387076, 1.000000000000000000, 0.8660254037844387076, 1.000000000000000000, 0.8660254037844387076, 1.000000000000000000, 0.8660254037844387076, 1.000000000000000000, 0.8660254037844387076, 1.000000000000000000, 0.8660254037844387076, 1.000000000000000000, 0.8660254037844387076, 1.000000000000000000, 0.8660254037844387076, 1.000000000000000000, 0.8660254037844387076, 1.000000000000000000, 0.8660254037844387076, 1.000000000000000000, 0.8660254037844387076, 1.000000000000000000, 0.8660254037844387076, 1.000000000000000000, 0.8660254037844387076, 1.000000000000000000, 0.8660254037844387076, 1.000000000000000000, 0.8660254037844387076, 1.000000000000000000, 0.8660254037844387076, 1.000000000000000000, 0.8660254037844387076, 1.000000000000000000, 0.8660254037844387076, 1.000000000000000000, 0.8660254037844387076, 1.000000000000000000, 0.8660254037844387076, 1.000000000000000000, 0.8660254037844387076, 1.000000000000000000, 0.8660254037844387076, 1.000000000000000000, 0.8660254037844387076, 1.000000000000000000, 0.8660254037844387076, 1.000000000000000000, 0.8660254037844387076, 1.000000000000000000, 0.8660254037844387076, 1.000000000000000000, 0.8660254037844387076, 1.000000000000000000, 0.8660254037844387076, 1.000000000000000000, 0.8660254037844387076, 1.000000000000000000, 0.8660254037844387076, 1.000000000000000000, 0.8660254037844387076, 1.000000000000000000, 0.8660254037844387076, 1.000000000000000000, 0.8660254037844387076, 1.000000000000000000, 0.8660254037844387076, 1.000000000000000000, 0.8660254037844387076, 1.000000000000000000, 0.8660254037844387076, 1.000000000000000000, 0.8660254037844387076, 1.000000000000000000, 0.8660254037844387076, 1.000000000000000000, 0.8660254037844387076, 1.000000000000000000, 0.8660254037844387076, 1.000000000000000000, 0.8660254037844387076, 1.000000000000000000, 0.8660254037844387076, 1.000000000000000000, 0.8660254037844387076, 1.000000000000000000, 0.8660254037844387076, 1.000000000000000000, 0.8660254037844387076, 1.000000000000000000, 0.8660254037844387076, 1.000000000000000000, 0.8660254037844387076, 1.000000000000000000, 0.8660254037844387076, 1.000000000000000000, 0.8660254037844387076, 1.000000000000000000, 0.8660254037844387076, 1.000000000000000000, 0.8660254037844387076, 1.000000000000000000, 0.8660254037844387076, 1.000000000000000000, 0.8660254037844387076, 1.000000000000000000),
 ( 1.000000000000000000, 0.8660254037844387076, 1.000000000000000000, 0.8660254037844387076, 1.000000000000000000, 0.8660254037844387076, 1.000000000000000000, 0.8660254037844387076, 1.000000000000000000, 0.8660254037844387076, 1.000000000000000000, 0.8660254037844387076, 1.000000000000000000, 0.8660254037844387076, 1.000000000000000000, 0.8660254037844387076, 1.000000000000000000, 0.8660254037844387076, 1.000000000000000000, 0.8660254037844387076, 1.000000000000000000, 0.8660254037844387076, 1.000000000000000000, 0.8660254037844387076, 1.000000000000000000, 0.8660254037844387076, 1.000000000000000000, 0.8660254037844387076, 1.000000000000000000, 0.8660254037844387076, 1.000000000000000000, 0.8660254037844387076, 1.000000000000000000, 0.8660254037844387076, 1.000000000000000000, 0.8660254037844387076, 1.000000000000000000, 0.8660254037844387076, 1.000000000000000000, 0.8660254037844387076, 1.000000000000000000, 0.8660254037844387076, 1.000000000000000000, 0.8660254037844387076, 1.000000000000000000, 0.8660254037844387076, 1.000000000000000000, 0.8660254037844387076, 1.000000000000000000, 0.8660254037844387076, 1.000000000000000000, 0.8660254037844387076, 1.000000000000000000, 0.8660254037844387076, 1.000000000000000000, 0.8660254037844387076, 1.000000000000000000, 0.8660254037844387076, 1.000000000000000000, 0.8660254037844387076, 1.000000000000000000, 0.8660254037844387076, 1.000000000000000000, 0.8660254037844387076, 1.000000000000000000, 0.8660254037844387076, 1.000000000000000000, 0.8660254037844387076, 1.000000000000000000, 0.8660254037844387076, 1.000000000000000000, 0.8660254037844387076, 1.000000000000000000, 0.8660254037844387076, 1.000000000000000000, 0.8660254037844387076, 1.000000000000000000, 0.8660254037844387076, 1.000000000000000000, 0.8660254037844387076, 1.000000000000000000, 0.8660254037844387076, 1.000000000000000000, 0.8660254037844387076, 1.000000000000000000, 0.8660254037844387076, 1.000000000000000000, 0.8660254037844387076, 1.000000000000000000, 0.8660254037844387076, 1.000000000000000000, 0.8660254037844387076, 1.000000000000000000, 0.8660254037844387076, 1.000000000000000000, 0.8660254037844387076, 1.000000000000000000, 0.8660254037844387076, 1.000000000000000000, 0.8660254037844387076, 1.000000000000000000, 0.8660254037844387076, 1.000000000000000000, 0.8660254037844387076, 1.000000000000000000, 0.8660254037844387076, 1.000000000000000000, 0.8660254037844387076, 1.000000000000000000, 0.8660254037844387076, 1.000000000000000000, 0.8660254037844387076, 1.000000000000000000, 0.8660254037844387076, 1.000000000000000000, 0.8660254037844387076, 1.000000000000000000, 0.8660254037844387076, 1.000000000000000000, 0.8660254037844387076, 1.000000000000000000, 0.8660254037844387076, 1.000000000000000000, 0.8660254037844387076, 1.000000000000000000, 0.8660254037844387076, 1.000000000000000000, 0.8660254037844387076, 1.000000000000000000, 0.8660254037844387076, 1.000000000000000000, 0.8660254037844387076, 1.000000000000000000, 0.8660254037844387076, 1.000000000000000000, 0.8660254037844387076, 1.000000000000000000, 0.8660254037844387076, 1.000000000000000000, 0.8660254037844387076, 1.000000000000000000, 0.8660254037844387076, 1.000000000000000000, 0.8660254037844387076, 1.000000000000000000, 0.8660254037844387076, 1.000000000000000000, 0.8660254037844387076, 1.000000000000000000, 0.8660254037844387076, 1.000000000000000000, 0.8660254037844387076, 1.000000000000000000, 0.8660254037844387076, 1.000000000000000000, 0.8660254037844387076, 1.000000000000000000, 0.8660254037844387076, 1.000000000000000000, 0.8660254037844387076, 1.000000000000000000, 0.8660254037844387076, 1.000000000000000000, 0.8660254037844387076, 1.000000000000000000, 0.8660254037844387076, 1.000000000000000000, 0.8660254037844387076, 1.000000000000000000, 0.8660254037844387076, 1.000000000000000000, 0.8660254037844387076, 1.000000000000000000, 0.8660254037844387076, 1.000000000000000000, 0.8660254037844387076, 1.000000000000000000, 0.8660254037844387076, 1.000000000000000000, 0.8660254037844387076, 1.000000000000000000, 0.8660254037844387076, 1.000000000000000000, 0.8660254037844387076, 1.000000000000000000, 0.8660254037844387076, 1.000000000000000000, 0.8660254037844387076, 1.000000000000000000, 0.8660254037844387076, 1.000000000000000000, 0.8660254037844387076, 1.000000000000000000, 0.8660254037844387076, 1.000000000000000000, 0.8660254037844387076, 1.000000000000000000, 0.8660254037844387076, 1.000000000000000000, 0.8660254037844387076, 1.000000000000000000, 0.8660254037844387076, 1.000000000000000000, 0.8660254037844387076, 1.000000000000000000, 0.8660254037844387076, 1.000000000000000000, 0.8660254037844387076, 1.000000000000000000, 0.8660254037844387076, 1.000000000000000000, 0.8660254037844387076, 1.000000000000000000, 0.8660254037844387076, 1.000000000000000000, 0.8660254037844387076, 1.000000000000000000, 0.8660254037844387076, 1.000000000000000000, 0.8660254037844387076, 1.000000000000000000, 0.8660254037844387076, 1.000000000000000000, 0.8660254037844387076, 1.000000000000000000, 0.8660254037844387076, 1.000000000000000000, 0.8660254037844387076, 1.000000000000000000, 0.8660254037844387076, 1.000000000000000000, 0.8660254037844387076, 1.000000000000000000, 0.8660254037844387076, 1.000000000000000000, 0.8660254037844387076, 1.000000000000000000, 0.8660254037844387076, 1.000000000000000000, 0.8660254037844387076, 1.000000000000000000) ) ) 
 REPRESENTATION_ITEM ( '' )  SURFACE ( )  );
#125398=CARTESIAN_POINT ( 'NONE',  ( -3.644109427023046521, 7.473487774827342278, 0.000000000000000000 ) ) ;
#125400=CARTESIAN_POINT ( 'NONE',  ( -5.478376588373717659, 8.549133898814758936, -1.199719254218452047 ) ) ;
#125402=CARTESIAN_POINT ( 'NONE',  ( 7.471952054462754234, 8.850270497362297206, 1.082531754730549078 ) ) ;
#125404=CARTESIAN_POINT ( 'NONE',  ( -3.801259017012812436, 7.351524727272684245, -0.7148551115157241176 ) ) ;
#125411=CARTESIAN_POINT ( 'NONE',  ( -5.795184315198522285, 5.725746220678519904, -0.7998128361456362523 ) ) ;
#125418=CARTESIAN_POINT ( 'NONE',  ( -4.665414256878293031, 7.496714828783040296, -1.082531754730549967 ) ) ;
#125422=CARTESIAN_POINT ( 'NONE',  ( -3.610214042988883598, 7.433943160120816351, 0.7998128361456352531 ) ) ;
#125428=B_SPLINE_CURVE_WITH_KNOTS ( 'NONE', 3,
 ( #161479, #25051, #160395, #129052, #9868, #110648 ),
 .UNSPECIFIED., .F., .F.,
 ( 4, 2, 4 ),
 ( 0.002243932016730776184, 0.002555488403984033582, 0.002867044791237291414 ),
 .UNSPECIFIED. ) ;
#125435=EDGE_CURVE ( 'NONE', #13120, #51039, #200597, .T. ) ;
#125449=CARTESIAN_POINT ( 'NONE',  ( -5.094831863685302942, 9.165997284266655498, 0.7998128361456291469 ) ) ;
#125451=CARTESIAN_POINT ( 'NONE',  ( -3.955946960137363799, 7.837298230127379917, 0.7998128361456352531 ) ) ;
#125463=ORIENTED_EDGE ( 'NONE', *, *, #21454, .F. ) ;
#125478=CARTESIAN_POINT ( 'NONE',  ( -6.479871072688648148, 6.524547437750345402, 0.000000000000000000 ) ) ;
#125487=DIRECTION ( 'NONE',  ( -0.000000000000000000, -0.000000000000000000, -1.000000000000000000 ) ) ;
#125502=CARTESIAN_POINT ( 'NONE',  ( 7.849244587668864348, 8.122149871893999062, 0.7998128361456291469 ) ) ;
#125504=CARTESIAN_POINT ( 'NONE',  ( 7.503511670520385479, 7.718794801887437274, 0.7998128361456281477 ) ) ;
#125512=B_SPLINE_CURVE_WITH_KNOTS ( 'NONE', 3,
 ( #179934, #48870, #114986, #180986, #32607, #20599, #120330, #150640 ),
 .UNSPECIFIED., .F., .F.,
 ( 4, 2, 2, 4 ),
 ( 1.563658610346381350E-18, 0.001552951981419670906, 0.003105903962839340511, 0.006211807925678679287 ),
 .UNSPECIFIED. ) ;
#125519=CARTESIAN_POINT ( 'NONE',  ( 6.174897528274166270, 6.957956273452501783, 0.8961316764096085574 ) ) ;
#125521=CARTESIAN_POINT ( 'NONE',  ( 5.370438244788902971, 9.279612028980123384, -0.7216878364870458196 ) ) ;
#125530=CARTESIAN_POINT ( 'NONE',  ( -5.646044625448194410, 5.551749915969804938, 0.000000000000000000 ) ) ;
#125537=CARTESIAN_POINT ( 'NONE',  ( -5.248414861821563804, 9.137251415518218067, 0.7216878364870267237 ) ) ;
#125540=CARTESIAN_POINT ( 'NONE',  ( 6.505933609711257226, 8.683618192786854095, -1.599625672291281386 ) ) ;
#125541=CARTESIAN_POINT ( 'NONE',  ( 5.086602265255201871, 4.915193406792433883, -0.1714109360824608297 ) ) ;
#125545=EDGE_CURVE ( 'NONE', #198714, #175863, #192410, .T. ) ;
#125547=CARTESIAN_POINT ( 'NONE',  ( -2.823841133396259639, 6.516508098929413961, -0.7998128361456481317 ) ) ;
#125556=CARTESIAN_POINT ( 'NONE',  ( 5.481239241674765950, 9.616805891921051952, -0.7998128361456481317 ) ) ;
#125575=CARTESIAN_POINT ( 'NONE',  ( -6.936931872047518155, 8.122117267924091166, 1.199719254218452047 ) ) ;
#125577=CARTESIAN_POINT ( 'NONE',  ( 6.505933609711257226, 8.683618192786854095, -1.599625672291281386 ) ) ;
#125598=CARTESIAN_POINT ( 'NONE',  ( 4.584065335196252811, 8.362176967788721882, 0.7216878364870328300 ) ) ;
#125605=CARTESIAN_POINT ( 'NONE',  ( 6.556249800660121529, 9.806652646482286073, 1.199719254218452047 ) ) ;
#125610=CARTESIAN_POINT ( 'NONE',  ( -4.773879485787619892, 7.623257595843924150, 1.082531754730549967 ) ) ;
#125614=CARTESIAN_POINT ( 'NONE',  ( 2.976681210565074842, 6.504977021307106533, -0.5719620471287272245 ) ) ;
#125636=EDGE_LOOP ( 'NONE', ( #78409, #119485, #65580, #152717, #109854 ) ) ;
#125640=CARTESIAN_POINT ( 'NONE',  ( 4.309512724297349884, 6.121127159803966933, 1.599625672291261402 ) ) ;
#125650=CARTESIAN_POINT ( 'NONE',  ( -6.997416678428844072, 8.296645891989347987, 1.082531754730549078 ) ) ;
#125652=CARTESIAN_POINT ( 'NONE',  ( 5.045042557616584489, 5.058506870073687267, 0.000000000000000000 ) ) ;
#125660=DIRECTION ( 'NONE',  ( -0.000000000000000000, 1.000000000000000000, -0.000000000000000000 ) ) ;
#125669=CARTESIAN_POINT ( 'NONE',  ( -3.851925040058345573, 5.587274861525073355, -1.443375672974078761 ) ) ;
#125703=CARTESIAN_POINT ( 'NONE',  ( -7.605197822622922210, 7.837428646007010613, -0.7998128361456362523 ) ) ;
#125706=CARTESIAN_POINT ( 'NONE',  ( -7.286581212701773502, 7.465709267765667789, 0.7998128361456341429 ) ) ;
#125707=CARTESIAN_POINT ( 'NONE',  ( -6.317173229324657413, 6.334733287159020954, 0.000000000000000000 ) ) ;
#125709=ORIENTED_EDGE ( 'NONE', *, *, #88206, .T. ) ;
#125711=CARTESIAN_POINT ( 'NONE',  ( -7.878696662872776812, 8.364436659539265406, -0.7216878364870338292 ) ) ;
#125712=CARTESIAN_POINT ( 'NONE',  ( 6.007671464186812749, 10.02305078494439883, 0.7216878364870317197 ) ) ;
#125718=CARTESIAN_POINT ( 'NONE',  ( -3.980200614063634568, 6.801261928786307642, 1.199719254218452935 ) ) ;
#125725=DIRECTION ( 'NONE',  ( 0.000000000000000000, 0.000000000000000000, -1.000000000000000000 ) ) ;
#125732=CARTESIAN_POINT ( 'NONE',  ( 5.737035277238070385, 6.722237907313067140, -1.199719254218452047 ) ) ;
#125740=CIRCLE ( 'NONE', #59939, 1.250000000000000888 ) ;
#125756=AXIS2_PLACEMENT_3D ( 'NONE', #36847, #167930, #100787 ) ;
#125757=CARTESIAN_POINT ( 'NONE',  ( 5.879395890181562834, 6.888325289080478697, -1.199719254218452047 ) ) ;
#125758=CARTESIAN_POINT ( 'NONE',  ( 3.627688620108284745, 6.389997935838436227, 1.199719254218452047 ) ) ;
#125773=CARTESIAN_POINT ( 'NONE',  ( 6.509182584184366682, 6.829728176725765820, 0.5468608461018635847 ) ) ;
#125774=CARTESIAN_POINT ( 'NONE',  ( -3.458738584817664385, 7.049295759013638474, 0.7216878364870338292 ) ) ;
#125775=CARTESIAN_POINT ( 'NONE',  ( -3.231779075379149546, 6.036511184309975242, 0.9899555337401846344 ) ) ;
#125803=CARTESIAN_POINT ( 'NONE',  ( 4.553559489343365740, 6.405848385690952718, -1.599625672291269396 ) ) ;
#125813=CARTESIAN_POINT ( 'NONE',  ( 5.996449078994045223, 10.21788403546024782, 0.7998128361456331437 ) ) ;
#125818=EDGE_CURVE ( 'NONE', #93819, #186231, #123412, .T. ) ;
#125823=CARTESIAN_POINT ( 'NONE',  ( -6.038177310039794854, 8.137902509836795417, -1.599625672291271394 ) ) ;
#125833=VECTOR ( 'NONE', #83673, 1000.000000000000000 ) ;
#125838=CARTESIAN_POINT ( 'NONE',  ( 3.901714345682657292, 7.774026846596938434, 0.7998128361456271485 ) ) ;
#125850=CARTESIAN_POINT ( 'NONE',  ( 6.198956711081595294, 6.941498593865138567, 0.8670033951987624610 ) ) ;
#125870=CARTESIAN_POINT ( 'NONE',  ( -4.118644803501354978, 8.027112380718707030, 0.7998128361456352531 ) ) ;
#125872=CARTESIAN_POINT ( 'NONE',  ( 5.357406976055401948, 6.279338222599979424, 1.199719254218452935 ) ) ;
#125873=DIRECTION ( 'NONE',  ( 0.000000000000000000, 0.000000000000000000, 1.000000000000000000 ) ) ;
#125876=CARTESIAN_POINT ( 'NONE',  ( -6.934069218746458318, 7.054445274817795486, -0.7998128361456362523 ) ) ;
#125885=CARTESIAN_POINT ( 'NONE',  ( -5.393601776927423153, 7.665310133586674901, -1.338224700579364379 ) ) ;
#125903=CARTESIAN_POINT ( 'NONE',  ( 5.072158865288233009, 7.010880990960010273, 1.443375672974065660 ) ) ;
#125907=CARTESIAN_POINT ( 'NONE',  ( -6.129167961829681488, 9.308390501180058507, -1.199719254218452047 ) ) ;
#125911=ORIENTED_EDGE ( 'NONE', *, *, #18226, .F. ) ;
#125921=CARTESIAN_POINT ( 'NONE',  ( 4.441177836928239309, 7.339068688795062911, 1.199719254218452047 ) ) ;
#125970=CARTESIAN_POINT ( 'NONE',  ( -5.908321080505254841, 10.11506803722328129, 0.7998128361456291469 ) ) ;
#125975=CARTESIAN_POINT ( 'NONE',  ( -4.960304097753355457, 6.880383762169266504, 1.599625672291263179 ) ) ;
#125982=CARTESIAN_POINT ( 'NONE',  ( -3.630551273409382329, 7.457669928944732796, 0.7998128361456352531 ) ) ;
#125985=CARTESIAN_POINT ( 'NONE',  ( 5.586791213849657822, 7.504901977030062454, -1.335864709735144817 ) ) ;
#125989=CARTESIAN_POINT ( 'NONE',  ( 6.378184920586140727, 6.405913593630768510, 0.000000000000000000 ) ) ;
#125994=CARTESIAN_POINT ( 'NONE',  ( -4.462568837553487100, 5.235360394347691404, -1.199719254218453823 ) ) ;
#125999=CARTESIAN_POINT ( 'NONE',  ( -5.309953438407606363, 6.223975762010839574, 1.199719254218452935 ) ) ;
#126003=CARTESIAN_POINT ( 'NONE',  ( 4.028181036591620412, 7.713645286083276709, -0.7216878364870338292 ) ) ;
#126004=CARTESIAN_POINT ( 'NONE',  ( -4.611181641979265500, 8.393812659035525314, 0.000000000000000000 ) ) ;
#126012=CARTESIAN_POINT ( 'NONE',  ( 5.388439706788500594, 5.251210844200210559, 0.7998128361456352531 ) ) ;
#126016=CARTESIAN_POINT ( 'NONE',  ( -4.489157070319179432, 8.251450656689856444, 5.811111664500048210E-05 ) ) ;
#126020=CARTESIAN_POINT ( 'NONE',  ( 6.201928923608456046, 6.200281597156833691, 0.7998128361456350310 ) ) ;
#126031=CARTESIAN_POINT ( 'NONE',  ( -2.817581654649482292, 6.509205373724840982, -0.4305581727225830102 ) ) ;
#126039=CARTESIAN_POINT ( 'NONE',  ( 4.789099507923308963, 8.141322699134850183, 0.8117711051834965996 ) ) ;
#126048=CARTESIAN_POINT ( 'NONE',  ( 7.015418140428412386, 7.149352350113456822, 0.7998128361456331437 ) ) ;
#126055=CARTESIAN_POINT ( 'NONE',  ( -4.683575932806860465, 8.284415941318199472, -0.5487617172068790516 ) ) ;
#126061=CARTESIAN_POINT ( 'NONE',  ( -5.271087860662956537, 9.371629280740593870, 0.000000000000000000 ) ) ;
#126068=DIRECTION ( 'NONE',  ( 0.6507913734559640506, -0.7592566023653003482, 0.000000000000000000 ) ) ;
#126075=CARTESIAN_POINT ( 'NONE',  ( 5.352436782344940802, 9.466536356036257871, 0.000000000000000000 ) ) ;
#126079=DIRECTION ( 'NONE',  ( -0.6507913734559641616, -0.7592566023653004592, 0.000000000000000000 ) ) ;
#126084=CARTESIAN_POINT ( 'NONE',  ( 4.716257332707354699, 6.595662536282280719, -1.599625672291269396 ) ) ;
#126087=CARTESIAN_POINT ( 'NONE',  ( 5.899206235277530297, 7.015400374979486209, -1.082531754730548412 ) ) ;
#126095=CARTESIAN_POINT ( 'NONE',  ( -6.490830876026181251, 6.764709549658621590, 0.1777360701797660314 ) ) ;
#126103=CARTESIAN_POINT ( 'NONE',  ( -5.171509248969888617, 4.998125310078441075, 0.7998128361456281477 ) ) ;
#126104=CARTESIAN_POINT ( 'NONE',  ( 7.539742822975472158, 7.968990512992423447, -0.7216878364870317197 ) ) ;
#126116=CARTESIAN_POINT ( 'NONE',  ( -5.749539660647037032, 8.865490816466966351, 1.199719254218454489 ) ) ;
#126117=CARTESIAN_POINT ( 'NONE',  ( -5.984998465789844069, 5.947196063035064206, 0.7998128361456281477 ) ) ;
#126119=CARTESIAN_POINT ( 'NONE',  ( 7.648208051440442468, 8.095533279534887328, 0.000000000000000000 ) ) ;
#126130=CARTESIAN_POINT ( 'NONE',  ( -5.018153416333300143, 7.915986710968343054, -1.079799343345327234 ) ) ;
#126134=CARTESIAN_POINT ( 'NONE',  ( 5.614485009834906393, 6.683225611963085733, -1.082531754730548412 ) ) ;
#126139=CARTESIAN_POINT ( 'NONE',  ( -6.607619761813764647, 8.802252036906432764, 1.599625672291269396 ) ) ;
#126155=CARTESIAN_POINT ( 'NONE',  ( 5.397027666691686321, 8.454226823519094935, 1.199719254218451159 ) ) ;
#126190=CARTESIAN_POINT ( 'NONE',  ( 7.539742822975472158, 7.968990512992423447, -0.7216878364870317197 ) ) ;
#126222=CARTESIAN_POINT ( 'NONE',  ( -5.438755897737433287, 6.374245297895642537, -1.199719254218453823 ) ) ;
#126224=CARTESIAN_POINT ( 'NONE',  ( 5.194182247366868843, 8.113610817686430110, 1.082531754730548412 ) ) ;
#126229=CARTESIAN_POINT ( 'NONE',  ( -3.955946960137363799, 7.837298230127379917, 0.7998128361456352531 ) ) ;
#126233=FACE_BOUND ( 'NONE', #154820, .T. ) ;
#126235=CARTESIAN_POINT ( 'NONE',  ( -2.986538976760251263, 6.706322249520737522, -0.7998128361456481317 ) ) ;
#126237=CARTESIAN_POINT ( 'NONE',  ( -3.188928480291423728, 8.980740528189222971, 2.451733079074398969 ) ) ;
#126242=CARTESIAN_POINT ( 'NONE',  ( -3.311934663488232733, 7.085950550703385531, -0.7998128361456481317 ) ) ;
#126253=CARTESIAN_POINT ( 'NONE',  ( -3.637330350216213759, 7.465578851886037093, -0.7998128361456481317 ) ) ;
#126257=CARTESIAN_POINT ( 'NONE',  ( -6.794044374223859428, 7.099008989448849505, 0.000000000000000000 ) ) ;
#126258=CARTESIAN_POINT ( 'NONE',  ( -6.441532379824190357, 6.687744995982559892, 0.7216878364870257245 ) ) ;
#126260=CARTESIAN_POINT ( 'NONE',  ( 6.723917837734620484, 6.809268663637336516, 0.000000000000000000 ) ) ;
#126262=CARTESIAN_POINT ( 'NONE',  ( -5.908321080505254841, 10.11506803722328129, 0.7998128361456291469 ) ) ;
#126270=ORIENTED_EDGE ( 'NONE', *, *, #96537, .F. ) ;
#126280=CARTESIAN_POINT ( 'NONE',  ( 6.176621499477501054, 9.363752961769195693, -1.199719254218452047 ) ) ;
#126297=CARTESIAN_POINT ( 'NONE',  ( 4.613585901703492809, 8.466914752176691650, -0.2784627230535564046 ) ) ;
#126301=TOROIDAL_SURFACE ( 'NONE', #84770, 0.8300000000000010703, 0.08000000000000000167 ) ;
#126311=CARTESIAN_POINT ( 'NONE',  ( 6.821687566331318564, 7.987665577921906568, 1.199719254218452935 ) ) ;
#126314=CARTESIAN_POINT ( 'NONE',  ( -5.191846479390389568, 5.021852078902356631, 0.7998128361456281477 ) ) ;
#126317=CARTESIAN_POINT ( 'NONE',  ( -5.424670858799220063, 9.342883411992149334, 0.000000000000000000 ) ) ;
#126330=CARTESIAN_POINT ( 'NONE',  ( 8.005163354226054295, 8.304055099544019214, 0.000000000000000000 ) ) ;
#126331=CARTESIAN_POINT ( 'NONE',  ( 6.717138760927786834, 6.801359740696030443, -0.7998128361456481317 ) ) ;
#126335=CARTESIAN_POINT ( 'NONE',  ( 0.000000000000000000, 2.999999999999999112, -2.420000000000000373 ) ) ;
#126345=CARTESIAN_POINT ( 'NONE',  ( 7.198453214212898743, 7.362893269528701268, 0.7998128361456291469 ) ) ;
#126359=CARTESIAN_POINT ( 'NONE',  ( -5.153507786970275006, 7.105788066255672497, -1.443375672974066548 ) ) ;
#126360=CARTESIAN_POINT ( 'NONE',  ( -7.937372586157736443, 8.224965870130965584, 0.7998128361456341429 ) ) ;
#126372=CARTESIAN_POINT ( 'NONE',  ( 5.448397627845284141, 7.449826213943242514, 1.599625672291268286 ) ) ;
#126373=CARTESIAN_POINT ( 'NONE',  ( 7.374709211190586089, 7.568525266002632534, 0.000000000000000000 ) ) ;
#126376=CARTESIAN_POINT ( 'NONE',  ( 3.973948422136968084, 5.729635473950147606, -1.443375672974068769 ) ) ;
#126390=ORIENTED_EDGE ( 'NONE', *, *, #81808, .F. ) ;
#126394=CARTESIAN_POINT ( 'NONE',  ( 4.706615602599436343, 5.520081620234675412, 1.199719254218452935 ) ) ;
#126398=CARTESIAN_POINT ( 'NONE',  ( 5.411639590510088027, 6.342609606130419131, -1.199719254218452047 ) ) ;
#126403=DIRECTION ( 'NONE',  ( 0.000000000000000000, 0.000000000000000000, -1.000000000000000000 ) ) ;
#126408=CARTESIAN_POINT ( 'NONE',  ( 6.482206841109512396, 9.616306177052839743, -1.082531754730548412 ) ) ;
#126410=CARTESIAN_POINT ( 'NONE',  ( -7.279802135894939852, 7.457800344824362604, -0.7998128361456362523 ) ) ;
#126411=CARTESIAN_POINT ( 'NONE',  ( 5.391302360089590628, 6.318882837306503575, -1.199719254218452047 ) ) ;
#126421=CARTESIAN_POINT ( 'NONE',  ( -3.610214042988883598, 7.433943160120816351, 0.7998128361456352531 ) ) ;
#126456=CARTESIAN_POINT ( 'NONE',  ( 5.840530312436913007, 10.03597880781023299, 0.000000000000000000 ) ) ;
#126467=CARTESIAN_POINT ( 'NONE',  ( -4.736594563127865420, 6.619389305106191834, -1.599625672291271394 ) ) ;
#126469=CARTESIAN_POINT ( 'NONE',  ( -6.611536185319534908, 7.742488966741438716, 1.199719254218452047 ) ) ;
#126481=CARTESIAN_POINT ( 'NONE',  ( -5.773793314573309132, 7.829454515125894964, 1.599625672291263179 ) ) ;
#126489=CARTESIAN_POINT ( 'NONE',  ( -6.129694847154231852, 6.323934541200937787, -0.7216878364870338292 ) ) ;
#126493=CARTESIAN_POINT ( 'NONE',  ( -5.472651281771599763, 6.413789912602166687, 1.199719254218452935 ) ) ;
#126515=ORIENTED_EDGE ( 'NONE', *, *, #16540, .F. ) ;
#126516=CARTESIAN_POINT ( 'NONE',  ( -5.284646014276622950, 9.387447126623207794, -0.7998128361456362523 ) ) ;
#126519=CARTESIAN_POINT ( 'NONE',  ( -4.685224601974262271, 7.623789914682047808, -1.199719254218453823 ) ) ;
#126544=CARTESIAN_POINT ( 'NONE',  ( -5.433785704026946384, 9.561443431331920095, 0.000000000000000000 ) ) ;
#126572=CARTESIAN_POINT ( 'NONE',  ( 5.318541398310776103, 9.426991741329731056, -0.7998128361456481317 ) ) ;
#126581=CARTESIAN_POINT ( 'NONE',  ( 6.364460139928007187, 6.849615385491503616, 0.6807898044721304442 ) ) ;
#126585=CARTESIAN_POINT ( 'NONE',  ( 5.234661009243278151, 7.693064604033777343, 1.208367059251337361 ) ) ;
#126587=CARTESIAN_POINT ( 'NONE',  ( 5.560252395380198998, 9.501061871336672127, 0.7216878364870317197 ) ) ;
#126593=CARTESIAN_POINT ( 'NONE',  ( -5.041653019435350380, 6.975290837464928728, -1.599625672291271394 ) ) ;
#126599=CARTESIAN_POINT ( 'NONE',  ( -5.383996397958228819, 8.335060660042973524, 1.082531754730550855 ) ) ;
#126603=CARTESIAN_POINT ( 'NONE',  ( 7.503511670520385479, 7.718794801887437274, 0.7998128361456281477 ) ) ;
#126604=CARTESIAN_POINT ( 'NONE',  ( -5.609475307034339053, 6.101878995311609266, -0.7682545557971790506 ) ) ;
#126608=CARTESIAN_POINT ( 'NONE',  ( -3.634467696915153034, 6.397906858779740524, 1.199719254218452935 ) ) ;
#126616=CARTESIAN_POINT ( 'NONE',  ( 3.559858690238754342, 7.375195248579016649, -0.1711817872153587328 ) ) ;
#126618=CARTESIAN_POINT ( 'NONE',  ( 4.598150373690133463, 5.393538853173795111, -1.199719254218452047 ) ) ;
#126631=DIRECTION ( 'NONE',  ( 0.000000000000000000, 0.000000000000000000, -1.000000000000000000 ) ) ;
#126636=CARTESIAN_POINT ( 'NONE',  ( -6.587282531393266360, 8.778525268082516320, 1.599625672291269396 ) ) ;
#126639=CARTESIAN_POINT ( 'NONE',  ( 6.047819040147648373, 9.213483425884394507, 1.199719254218452047 ) ) ;
#126647=CARTESIAN_POINT ( 'NONE',  ( 5.876533236880477240, 5.820653295974182129, 0.7998128361456352531 ) ) ;
#126650=CARTESIAN_POINT ( 'NONE',  ( 4.517520595836055364, 8.499999999998847144, 0.1397284385386432237 ) ) ;
#126660=CARTESIAN_POINT ( 'NONE',  ( 4.719646871332936477, 8.520355426614829142, -0.7216878364870357165 ) ) ;
#126672=CARTESIAN_POINT ( 'NONE',  ( -6.129694847154231852, 6.323934541200937787, -0.7216878364870338292 ) ) ;
#126678=CARTESIAN_POINT ( 'NONE',  ( 2.972033609136344623, 6.549060441754430251, -0.4946758370507741698 ) ) ;
#126705=CARTESIAN_POINT ( 'NONE',  ( 4.390861645979372341, 6.216034235099629157, -1.599625672291269396 ) ) ;
#126710=CARTESIAN_POINT ( 'NONE',  ( 5.554837709854577810, 5.910988393603817670, -0.7721120281754164649 ) ) ;
#126711=EDGE_CURVE ( 'NONE', #157478, #116214, #102594, .T. ) ;
#126718=CARTESIAN_POINT ( 'NONE',  ( -7.132998214565509087, 7.494455136514109661, 0.7216878364870317197 ) ) ;
#126720=CARTESIAN_POINT ( 'NONE',  ( 4.543390873910906791, 6.393985001019784953, 1.443375672974065660 ) ) ;
#126738=CARTESIAN_POINT ( 'NONE',  ( -4.177320726786328819, 5.966903162707725805, -1.443375672974066548 ) ) ;
#126757=ADVANCED_FACE ( 'NONE', ( #43048 ), #10504, .F. ) ;
#126772=CARTESIAN_POINT ( 'NONE',  ( -5.610041701004606196, 9.767075427805856691, -0.7998128361456362523 ) ) ;
#126776=CARTESIAN_POINT ( 'NONE',  ( -4.662743238902972820, 8.402825839448235357, 0.5650157067484343765 ) ) ;
#126780=ORIENTED_EDGE ( 'NONE', *, *, #70214, .T. ) ;
#126782=CARTESIAN_POINT ( 'NONE',  ( -7.065207446052809814, 9.336104335185325453, -1.443375672974066548 ) ) ;
#126786=CARTESIAN_POINT ( 'NONE',  ( -4.625266680917477835, 5.425174544939014964, -1.199719254218453823 ) ) ;
#126790=CARTESIAN_POINT ( 'NONE',  ( -5.004894982100124068, 5.868074229652107121, 1.199719254218452935 ) ) ;
#126798=CARTESIAN_POINT ( 'NONE',  ( -6.084577077482911101, 10.32070003369722144, 0.000000000000000000 ) ) ;
#126803=CARTESIAN_POINT ( 'NONE',  ( 3.576318658954677598, 7.394398545414291313, 0.7998128361456281477 ) ) ;
#126825=CARTESIAN_POINT ( 'NONE',  ( 5.041653019435334393, 6.975290837464928728, -1.599625672291269396 ) ) ;
#126826=CARTESIAN_POINT ( 'NONE',  ( 4.655245641445829641, 6.524482229810530498, 1.599625672291269396 ) ) ;
#126828=CARTESIAN_POINT ( 'NONE',  ( 3.715816618597135523, 6.492813934075403637, -1.199719254218453823 ) ) ;
#126840=CARTESIAN_POINT ( 'NONE',  ( 5.057296774772758852, 7.978757421411086348, 1.172581024337983724 ) ) ;
#126841=CARTESIAN_POINT ( 'NONE',  ( -5.777182852754558340, 5.912670547734647286, 0.000000000000000000 ) ) ;
#126842=CARTESIAN_POINT ( 'NONE',  ( 3.390947817193682656, 6.009837315817661008, -1.082531754730549967 ) ) ;
#126871=CARTESIAN_POINT ( 'NONE',  ( 5.239300017038202917, 5.077214539491492928, 0.000000000000000000 ) ) ;
#126906=CARTESIAN_POINT ( 'NONE',  ( 4.603875680292229156, 7.528882839386387360, 1.199719254218452047 ) ) ;
#126918=CARTESIAN_POINT ( 'NONE',  ( 5.685886686578042415, 7.314606927785019863, 1.221034997698521307 ) ) ;
#126939=CARTESIAN_POINT ( 'NONE',  ( -6.981522756394290319, 7.109807735406931783, 0.7998128361456341429 ) ) ;
#126941=CARTESIAN_POINT ( 'NONE',  ( 5.435893244436359240, 5.306573304789342416, -0.7998128361456481317 ) ) ;
#126945=CARTESIAN_POINT ( 'NONE',  ( -5.752402313948099533, 9.933162809573264695, -0.7998128361456362523 ) ) ;
#126948=CARTESIAN_POINT ( 'NONE',  ( 7.876360894896227371, 8.153785563659219804, -0.7998128361456341429 ) ) ;
#126953=CARTESIAN_POINT ( 'NONE',  ( -5.929989559956849732, 7.234276776666978215, -1.248630897662094563 ) ) ;
#126972=CARTESIAN_POINT ( 'NONE',  ( 4.529832720741620022, 7.338536369956936589, -1.082531754730548412 ) ) ;
#126986=CARTESIAN_POINT ( 'NONE',  ( -3.894504475113999664, 7.459775595827967898, -0.4024148884765280654 ) ) ;
#126991=CARTESIAN_POINT ( 'NONE',  ( 4.549643065837591038, 7.465611455855944101, -1.199719254218452047 ) ) ;
#127040=CARTESIAN_POINT ( 'NONE',  ( -5.004368096775595021, 5.971422546727199077, 1.082531754730549078 ) ) ;
#127047=CARTESIAN_POINT ( 'NONE',  ( -5.635349125135588721, 6.603604063193491136, 1.199719254218452935 ) ) ;
#127056=CARTESIAN_POINT ( 'NONE',  ( -4.308458954092677651, 8.248562223075252220, -0.7998128361456362523 ) ) ;
#127059=CARTESIAN_POINT ( 'NONE',  ( 6.425920342564602983, 6.885296541689900351, -0.7293792964763821107 ) ) ;
#127064=CARTESIAN_POINT ( 'NONE',  ( 6.099189001301251523, 8.209082816308541197, 1.599625672291268286 ) ) ;
#127069=CARTESIAN_POINT ( 'NONE',  ( -5.901542003698421190, 10.10715911428198055, 0.000000000000000000 ) ) ;
#127076=CARTESIAN_POINT ( 'NONE',  ( -6.120580001926503755, 6.105374521861167914, -0.7998128361456362523 ) ) ;
#127079=CARTESIAN_POINT ( 'NONE',  ( 4.977251789548238214, 7.860525283564661514, -1.082531754730548412 ) ) ;
#127080=CARTESIAN_POINT ( 'NONE',  ( -5.058600711230246461, 7.955432358860325515, 1.082531754730549967 ) ) ;
#127088=CARTESIAN_POINT ( 'NONE',  ( 4.797606254389322089, 6.690569611577942943, 1.599625672291268286 ) ) ;
#127096=CARTESIAN_POINT ( 'NONE',  ( -2.981281212289682792, 6.492261378021210838, -0.0003813922843012157449 ) ) ;
#127117=CARTESIAN_POINT ( 'NONE',  ( 4.620579464570812256, 8.341333509328540785, -0.3192730525469981151 ) ) ;
#127122=CARTESIAN_POINT ( 'NONE',  ( 6.692885107001518286, 7.837396042037102717, -1.199719254218452047 ) ) ;
#127128=CARTESIAN_POINT ( 'NONE',  ( -4.964107424972056037, 7.970992240003957008, 1.031144368780096965 ) ) ;
#127134=CARTESIAN_POINT ( 'NONE',  ( -2.997761361953021009, 6.511488999004883205, -0.7216878364870458196 ) ) ;
#127145=CARTESIAN_POINT ( 'NONE',  ( -4.034433228518296666, 6.864533312316751790, -1.199719254218450271 ) ) ;
#127147=CARTESIAN_POINT ( 'NONE',  ( 6.688968683495743583, 8.897159112202094988, -1.599625672291283607 ) ) ;
#127158=CARTESIAN_POINT ( 'NONE',  ( 3.718679271898170491, 7.560485927181699317, 0.7998128361456271485 ) ) ;
#127161=CARTESIAN_POINT ( 'NONE',  ( 4.380693030546905398, 8.124909279031149012, 0.7216878364870247253 ) ) ;
#127171=CARTESIAN_POINT ( 'NONE',  ( -6.121671443416687453, 7.010146470470823843, 0.9629068762325782016 ) ) ;
#127179=CARTESIAN_POINT ( 'NONE',  ( -3.623772196602547346, 7.449761006003425834, 0.000000000000000000 ) ) ;
#127180=CARTESIAN_POINT ( 'NONE',  ( 6.536439455564150514, 9.679577560583279450, 1.082531754730549078 ) ) ;
#127193=CARTESIAN_POINT ( 'NONE',  ( -4.911796789900812144, 8.952456364851418158, 0.7998128361456291469 ) ) ;
#127194=CARTESIAN_POINT ( 'NONE',  ( -4.111865726694519552, 8.019203457777400956, 0.000000000000000000 ) ) ;
#127196=CARTESIAN_POINT ( 'NONE',  ( 7.973603738168424826, 8.475161580717541554, 0.000000000000000000 ) ) ;
#127201=CARTESIAN_POINT ( 'NONE',  ( 3.390947817193682656, 6.009837315817661008, -1.082531754730549967 ) ) ;
#127207=CARTESIAN_POINT ( 'NONE',  ( -6.374142478797011790, 6.840173217398676897, -0.5947513654121737714 ) ) ;
#127216=CARTESIAN_POINT ( 'NONE',  ( -5.921879234118920365, 10.13088588310589699, 0.000000000000000000 ) ) ;
#127223=CARTESIAN_POINT ( 'NONE',  ( 2.449293598294706414E-16, 9.999999999999998224, 2.000000000000000000 ) ) ;
#127232=CARTESIAN_POINT ( 'NONE',  ( 7.178115983792402233, 7.339166500704784823, 0.7998128361456281477 ) ) ;
#127266=CARTESIAN_POINT ( 'NONE',  ( 3.984117037569365305, 5.741498858621315371, 1.599625672291261402 ) ) ;
#127297=CARTESIAN_POINT ( 'NONE',  ( -4.468294144155606773, 7.370704380560280100, 1.199719254218452935 ) ) ;
#127299=CARTESIAN_POINT ( 'NONE',  ( 5.031484404002878996, 7.923796667095108326, 1.082531754730548412 ) ) ;
#127304=CARTESIAN_POINT ( 'NONE',  ( -4.444040490229335560, 8.406740681901359480, 0.7998128361456352531 ) ) ;
#127309=CARTESIAN_POINT ( 'NONE',  ( -4.659162064951642535, 5.464719159645540003, 1.199719254218452935 ) ) ;
#127310=VECTOR ( 'NONE', #75862, 1000.000000000000000 ) ;
#127317=CARTESIAN_POINT ( 'NONE',  ( -5.960744811863571968, 6.983232364376142698, 1.199719254218452935 ) ) ;
#127327=CARTESIAN_POINT ( 'NONE',  ( -3.311934663488232733, 7.085950550703385531, -0.7998128361456481317 ) ) ;
#127331=CARTESIAN_POINT ( 'NONE',  ( -4.502716413514296079, 8.267269892493059658, -0.7216878364870338292 ) ) ;
#127332=CARTESIAN_POINT ( 'NONE',  ( -6.143253000323532831, 7.300121600866474658, 1.082531754730548412 ) ) ;
#127333=CARTESIAN_POINT ( 'NONE',  ( 5.189738938980948291, 9.276722205444929870, 0.000000000000000000 ) ) ;
#127334=CARTESIAN_POINT ( 'NONE',  ( -5.094831863685302942, 9.165997284266655498, 0.7998128361456291469 ) ) ;
#127341=ORIENTED_EDGE ( 'NONE', *, *, #6236, .F. ) ;
#127352=CARTESIAN_POINT ( 'NONE',  ( 6.016786309414542622, 10.24161080428416426, 0.7998128361456341429 ) ) ;
#127370=CARTESIAN_POINT ( 'NONE',  ( 4.617922728991994852, 8.461530327540957686, 0.3091873533234041904 ) ) ;
#127383=CARTESIAN_POINT ( 'NONE',  ( 5.189738938980948291, 9.276722205444929870, 0.000000000000000000 ) ) ;
#127386=CARTESIAN_POINT ( 'NONE',  ( -5.354544322754380303, 5.211666229493680191, 0.7998128361456281477 ) ) ;
#127390=CARTESIAN_POINT ( 'NONE',  ( -7.227905289416804102, 8.565549271475310533, -1.082531754730549967 ) ) ;
#127402=CARTESIAN_POINT ( 'NONE',  ( 7.289443866002793371, 8.533381260871966134, 1.199719254218452047 ) ) ;
#127403=CARTESIAN_POINT ( 'NONE',  ( 5.448397627845284141, 7.449826213943242514, 1.599625672291268286 ) ) ;
#127411=VERTEX_POINT ( 'NONE', #133351 ) ;
#127418=CARTESIAN_POINT ( 'NONE',  ( 5.027041095616958444, 9.086908054853605421, 0.000000000000000000 ) ) ;
#127432=CARTESIAN_POINT ( 'NONE',  ( -4.733481511527885210, 4.890303307122107590, -0.5491554243041256722 ) ) ;
#127435=CARTESIAN_POINT ( 'NONE',  ( -5.966997003790240228, 6.134120390609613338, -0.7216878364870338292 ) ) ;
#127436=CARTESIAN_POINT ( 'NONE',  ( -5.749539660647037032, 8.865490816466966351, 1.199719254218454489 ) ) ;
#127442=VERTEX_POINT ( 'NONE', #117126 ) ;
#127448=CARTESIAN_POINT ( 'NONE',  ( -2.986538976760251263, 6.706322249520737522, -0.7998128361456481317 ) ) ;
#127449=CARTESIAN_POINT ( 'NONE',  ( 5.203297092594585393, 9.292540051327542017, 0.7998128361456341429 ) ) ;
#127452=CARTESIAN_POINT ( 'NONE',  ( 6.016786309414542622, 10.24161080428416426, 0.7998128361456341429 ) ) ;
#127472=CARTESIAN_POINT ( 'NONE',  ( 6.222266154028957885, 6.224008365980749247, 0.7998128361456352531 ) ) ;
#127477=CARTESIAN_POINT ( 'NONE',  ( 4.376249722160992839, 8.327651452488305850, 0.000000000000000000 ) ) ;
#127481=CARTESIAN_POINT ( 'NONE',  ( 4.689424523294686509, 8.358602041046323095, -0.7454045323363468478 ) ) ;
#127487=CARTESIAN_POINT ( 'NONE',  ( 6.211043768836170820, 9.299949259400630552, 1.082531754730549967 ) ) ;
#127489=CARTESIAN_POINT ( 'NONE',  ( -7.065734331377342414, 8.272386803808890576, -1.199719254218452047 ) ) ;
#127490=CARTESIAN_POINT ( 'NONE',  ( 3.881377115262159894, 7.750300077773022878, 0.7998128361456271485 ) ) ;
#127500=CARTESIAN_POINT ( 'NONE',  ( -6.134138155540168391, 6.121192367743780949, 0.000000000000000000 ) ) ;
#127533=CARTESIAN_POINT ( 'NONE',  ( 6.966220764712121927, 6.002124920821316323, 2.420000000000000373 ) ) ;
#127534=CARTESIAN_POINT ( 'NONE',  ( 5.031484404002889654, 6.003058238492422483, 1.082531754730549078 ) ) ;
#127546=CARTESIAN_POINT ( 'NONE',  ( -4.294900800479008574, 8.232744377192641849, 0.000000000000000000 ) ) ;
#127548=CARTESIAN_POINT ( 'NONE',  ( -6.237633190739009237, 9.434933268240943249, 1.199719254218452047 ) ) ;
#127550=CARTESIAN_POINT ( 'NONE',  ( 5.953438849732186178, 8.999410187112612647, -1.082531754730548412 ) ) ;
#127562=CARTESIAN_POINT ( 'NONE',  ( -4.613517410400161722, 8.604463755433990002, -0.7998128361456362523 ) ) ;
#127568=CARTESIAN_POINT ( 'NONE',  ( -3.689227196694341515, 7.318199139536432973, -0.7216878364870458196 ) ) ;
#127573=CARTESIAN_POINT ( 'NONE',  ( -4.285259070371116863, 7.157163461145040095, 1.199719254218452935 ) ) ;
#127594=CARTESIAN_POINT ( 'NONE',  ( -6.577640801285370209, 7.702944352034914566, -1.199719254218452047 ) ) ;
#127596=CARTESIAN_POINT ( 'NONE',  ( -3.494969737272722643, 7.299491470118629088, -0.7998128361456481317 ) ) ;
#127621=CARTESIAN_POINT ( 'NONE',  ( -5.607179047703544583, 8.699403434699558346, 1.199719254218454489 ) ) ;
#127648=CARTESIAN_POINT ( 'NONE',  ( 7.343676480457483002, 8.596652644402405841, -1.199719254218452047 ) ) ;
#127649=LINE ( 'NONE', #178448, #162464 ) ;
#127662=CARTESIAN_POINT ( 'NONE',  ( 6.017777097630443883, 7.067734144800174256, 1.048426327298467742 ) ) ;
#127664=CARTESIAN_POINT ( 'NONE',  ( 6.373741612200162443, 8.529394195690610303, 1.443375672974065660 ) ) ;
#127670=CARTESIAN_POINT ( 'NONE',  ( -6.134138155540168391, 6.121192367743780949, 0.000000000000000000 ) ) ;
#127677=CARTESIAN_POINT ( 'NONE',  ( -5.844973620822877969, 7.912498205750389424, 1.443375672974058777 ) ) ;
#127681=CARTESIAN_POINT ( 'NONE',  ( -5.646002790254049941, 6.144272845372873881, 0.7680594912782515715 ) ) ;
#127687=CARTESIAN_POINT ( 'NONE',  ( -4.981695098378565945, 4.776675467721892332, -0.7998128361456362523 ) ) ;
#127697=CARTESIAN_POINT ( 'NONE',  ( 6.156284269057003655, 9.340026192945279249, -1.199719254218452047 ) ) ;
#127703=CARTESIAN_POINT ( 'NONE',  ( -4.858757509019071996, 5.629766575900002401, 7.500000000000000000 ) ) ;
#127709=CIRCLE ( 'NONE', #124161, 0.07999999999999998779 ) ;
#127719=CARTESIAN_POINT ( 'NONE',  ( 4.844006021832467646, 8.873367135438366304, 0.000000000000000000 ) ) ;
#127722=CARTESIAN_POINT ( 'NONE',  ( -6.220586654761008027, 6.942393398233093649, 0.8502372543972673835 ) ) ;
#127729=CARTESIAN_POINT ( 'NONE',  ( 6.229045230835819069, 6.231917288922055320, -0.7998128361456481317 ) ) ;
#127742=CARTESIAN_POINT ( 'NONE',  ( 6.726253606155519371, 7.019919760035800316, -0.7216878364870458196 ) ) ;
#127743=ORIENTED_EDGE ( 'NONE', *, *, #136398, .F. ) ;
#127754=CARTESIAN_POINT ( 'NONE',  ( -5.560252395380252288, 7.580323442733986283, 1.443375672974058777 ) ) ;
#127777=TOROIDAL_SURFACE ( 'NONE', #27334, 2.080000000000000071, 0.08000000000000000167 ) ;
#127788=CARTESIAN_POINT ( 'NONE',  ( 4.746236293235721604, 7.694970221153795364, 1.199719254218451159 ) ) ;
#127799=CARTESIAN_POINT ( 'NONE',  ( -4.990809943606269172, 8.836712344267034780, -0.7216878364870338292 ) ) ;
#127803=CARTESIAN_POINT ( 'NONE',  ( 4.299344108864946890, 6.109263775132799168, -1.443375672974068769 ) ) ;
#127820=CARTESIAN_POINT ( 'NONE',  ( -3.011319516011047082, 6.527306845405913549, 0.7216878364870328300 ) ) ;
#127858=CARTESIAN_POINT ( 'NONE',  ( -7.099629715411508890, 8.311931418515415615, 1.199719254218452047 ) ) ;
#127859=CARTESIAN_POINT ( 'NONE',  ( -5.337921042252067316, 7.714266718146587820, 1.325459453385816833 ) ) ;
#127860=CARTESIAN_POINT ( 'NONE',  ( -5.606333003394546211, 5.691104718644762528, 0.3812976639747498453 ) ) ;
#127861=CARTESIAN_POINT ( 'NONE',  ( -4.694467135394339685, 8.285658806408200405, 0.6022741701859417596 ) ) ;
#127864=DIRECTION ( 'NONE',  ( -0.6507913734559650498, 0.7592566023652995710, 0.000000000000000000 ) ) ;
#127867=CARTESIAN_POINT ( 'NONE',  ( -4.248501033035892327, 6.049946853332221153, -1.599625672291271394 ) ) ;
#127870=CARTESIAN_POINT ( 'NONE',  ( -3.305155586681401303, 7.078041627762083898, 0.7998128361456352531 ) ) ;
#127883=CARTESIAN_POINT ( 'NONE',  ( 5.574337433874081427, 6.532423756721743580, -1.199719254218452047 ) ) ;
#127889=CARTESIAN_POINT ( 'NONE',  ( 0.3999999999910882620, 3.122291170403207694, -2.023857702510297507 ) ) ;
#127906=CARTESIAN_POINT ( 'NONE',  ( 3.881377115262159894, 7.750300077773022878, 0.7998128361456271485 ) ) ;
#127907=CARTESIAN_POINT ( 'NONE',  ( 4.869313445963426190, 5.709895770826003414, 1.199719254218452935 ) ) ;
#127909=CARTESIAN_POINT ( 'NONE',  ( 5.090160327287878594, 4.903218234782778850, -0.7998128361456481317 ) ) ;
#127923=CARTESIAN_POINT ( 'NONE',  ( 4.842126824027952026, 8.201492973507317430, 0.9351865777775794086 ) ) ;
#127925=CARTESIAN_POINT ( 'NONE',  ( -5.451787166026575981, 5.533042246551999277, 0.000000000000000000 ) ) ;
#127926=CARTESIAN_POINT ( 'NONE',  ( 3.607878275012313285, 6.262922849939428716, 1.082531754730549078 ) ) ;
#127939=ORIENTED_EDGE ( 'NONE', *, *, #26150, .T. ) ;
#127952=CARTESIAN_POINT ( 'NONE',  ( 5.252858170651868441, 5.093032385374103299, -0.7998128361456481317 ) ) ;
#127972=CARTESIAN_POINT ( 'NONE',  ( -6.149505192250180663, 9.332117270003974951, -1.199719254218452047 ) ) ;
#127982=CARTESIAN_POINT ( 'NONE',  ( 5.936491157937257235, 8.019268665717216749, 1.599625672291268286 ) ) ;
#127985=ORIENTED_EDGE ( 'NONE', *, *, #84476, .T. ) ;
#127987=CARTESIAN_POINT ( 'NONE',  ( 5.037736595929563244, 8.035053907629919223, -1.199719254218452047 ) ) ;
#128016=CARTESIAN_POINT ( 'NONE',  ( -4.956387674247580755, 7.940146832334256111, 1.199719254218452935 ) ) ;
#128018=CARTESIAN_POINT ( 'NONE',  ( 4.213551878797002992, 8.137837301896977849, 0.000000000000000000 ) ) ;
#128022=CARTESIAN_POINT ( 'NONE',  ( -6.050681693448748177, 10.28115541899069463, 0.7998128361456291469 ) ) ;
#128030=CARTESIAN_POINT ( 'NONE',  ( -4.620524454801235414, 8.454239455966142458, -0.3877863265914320845 ) ) ;
#128042=ORIENTED_EDGE ( 'NONE', *, *, #20908, .T. ) ;
#128046=CARTESIAN_POINT ( 'NONE',  ( 6.726253606155519371, 7.019919760035800316, -0.7216878364870458196 ) ) ;
#128051=ORIENTED_EDGE ( 'NONE', *, *, #8784, .T. ) ;
#128064=CARTESIAN_POINT ( 'NONE',  ( 6.222266154028957885, 6.224008365980749247, 0.7998128361456352531 ) ) ;
#128103=FACE_OUTER_BOUND ( 'NONE', #100730, .T. ) ;
#128113=CARTESIAN_POINT ( 'NONE',  ( -5.451787166026575981, 5.533042246551999277, 0.000000000000000000 ) ) ;
#128114=DIRECTION ( 'NONE',  ( -1.000000000000000000, 0.000000000000000000, 0.000000000000000000 ) ) ;
#128118=CARTESIAN_POINT ( 'NONE',  ( -5.315678745009726924, 8.359319748223434487, -1.199719254218453823 ) ) ;
#128127=CARTESIAN_POINT ( 'NONE',  ( -4.655245641445871385, 6.524482229810530498, 1.599625672291263179 ) ) ;
#128129=CARTESIAN_POINT ( 'NONE',  ( 5.678247172832384670, 7.430942480705488684, 1.324022058552588366 ) ) ;
#128132=CARTESIAN_POINT ( 'NONE',  ( -4.260029445439585061, 7.236136616047151193, -2.420000000000000373 ) ) ;
#128134=CARTESIAN_POINT ( 'NONE',  ( 4.746236293235721604, 7.694970221153795364, 1.199719254218451159 ) ) ;
#128143=DIRECTION ( 'NONE',  ( 1.000000000000000000, 0.000000000000000000, 0.000000000000000000 ) ) ;
#128144=CARTESIAN_POINT ( 'NONE',  ( -8.100070429521727178, 8.414780020722290033, 0.7998128361456341429 ) ) ;
#128149=CARTESIAN_POINT ( 'NONE',  ( -4.285259070371116863, 7.157163461145040095, 1.199719254218452935 ) ) ;
#128153=CARTESIAN_POINT ( 'NONE',  ( 6.821160681006793070, 7.130644680695653825, 0.7216878364870328300 ) ) ;
#128155=CARTESIAN_POINT ( 'NONE',  ( -4.936577328707246082, 8.773440960218172435, 0.000000000000000000 ) ) ;
#128159=CARTESIAN_POINT ( 'NONE',  ( -5.448397627845328550, 7.449826213943242514, 1.599625672291263401 ) ) ;
#128162=CARTESIAN_POINT ( 'NONE',  ( 5.554000203453580475, 6.508696987897830688, -1.199719254218452047 ) ) ;
#128168=CARTESIAN_POINT ( 'NONE',  ( 4.206772801990143584, 8.129928378955675328, 0.7998128361456271485 ) ) ;
#128175=EDGE_CURVE ( 'NONE', #512, #58907, #170495, .T. ) ;
#128192=CARTESIAN_POINT ( 'NONE',  ( 4.920187338115698417, 7.999083482620499730, 0.9937779052983791717 ) ) ;
#128201=CARTESIAN_POINT ( 'NONE',  ( 6.180537922983273091, 8.303989891604203422, -1.599625672291281386 ) ) ;
#128206=CARTESIAN_POINT ( 'NONE',  ( -4.940673843451318881, 7.995311821131723562, 1.007273293859496155 ) ) ;
#128213=CARTESIAN_POINT ( 'NONE',  ( -3.160459205317013076, 6.701303149596211206, -0.7216878364870458196 ) ) ;
#128223=CARTESIAN_POINT ( 'NONE',  ( -5.490125858891038213, 5.369844688319787451, -0.7998128361456362523 ) ) ;
#128225=CARTESIAN_POINT ( 'NONE',  ( 8.011942431032855083, 8.311964022485323511, 0.7998128361456291469 ) ) ;
#128229=CARTESIAN_POINT ( 'NONE',  ( -2.907411709271221945, 6.510044087496495990, 0.000000000000000000 ) ) ;
#128234=CARTESIAN_POINT ( 'NONE',  ( 4.746236293235721604, 7.694970221153795364, 1.199719254218451159 ) ) ;
#128237=CARTESIAN_POINT ( 'NONE',  ( 6.170369307550823912, 7.331757292631694511, 1.082531754730549967 ) ) ;
#128245=CARTESIAN_POINT ( 'NONE',  ( -6.286530415420750195, 6.898050863092263896, 0.7571273896394186131 ) ) ;
#128253=CARTESIAN_POINT ( 'NONE',  ( -4.984557751679625781, 5.844347460828191565, 1.199719254218452935 ) ) ;
#128254=CARTESIAN_POINT ( 'NONE',  ( 5.713835393516482952, 5.630839145382857680, 0.7998128361456352531 ) ) ;
#128257=ADVANCED_FACE ( 'NONE', ( #57962 ), #206300, .T. ) ;
#128266=CARTESIAN_POINT ( 'NONE',  ( -7.259464905474441565, 7.434073576000447048, -0.7998128361456362523 ) ) ;
#128267=CARTESIAN_POINT ( 'NONE',  ( 6.261886844665240481, 8.398896966899865646, 1.599625672291268286 ) ) ;
#128269=CARTESIAN_POINT ( 'NONE',  ( 7.661766205054107992, 8.111351125417501251, -0.7216878364870317197 ) ) ;
#128274=CARTESIAN_POINT ( 'NONE',  ( 5.063044020060520900, 4.871582543017558109, 0.7998128361456352531 ) ) ;
#128281=CARTESIAN_POINT ( 'NONE',  ( -5.527359202251545867, 7.456348097644321271, -1.248928334283349040 ) ) ;
#128290=CARTESIAN_POINT ( 'NONE',  ( -5.935437387732586778, 10.14670372898850381, -0.7998128361456362523 ) ) ;
#128306=CARTESIAN_POINT ( 'NONE',  ( 5.668190738965027897, 8.770583741171307679, -1.199719254218452047 ) ) ;
#128340=CARTESIAN_POINT ( 'NONE',  ( 7.349928672384119288, 8.707909884937221179, 1.082531754730549967 ) ) ;
#128353=FACE_BOUND ( 'NONE', #171776, .T. ) ;
#128368=CARTESIAN_POINT ( 'NONE',  ( -5.981082042284069367, 7.006959133200059142, 1.199719254218452935 ) ) ;
#128370=CARTESIAN_POINT ( 'NONE',  ( 4.855228407025239612, 8.678533884922511987, 0.000000000000000000 ) ) ;
#128375=CARTESIAN_POINT ( 'NONE',  ( -3.969505113751027547, 7.853116076009993840, 1.214306433183764966E-14 ) ) ;
#128381=CARTESIAN_POINT ( 'NONE',  ( -7.919371124158132602, 8.411890197705517380, -0.7216878364870338292 ) ) ;
#128387=CARTESIAN_POINT ( 'NONE',  ( -6.394605727500880299, 7.489403432619674561, -1.199719254218452047 ) ) ;
#128397=CARTESIAN_POINT ( 'NONE',  ( -3.284818356260900796, 7.054314858938165678, 0.7998128361456352531 ) ) ;
#128400=CARTESIAN_POINT ( 'NONE',  ( -6.807602527837528505, 7.114826835331461652, 0.7216878364870317197 ) ) ;
#128401=CARTESIAN_POINT ( 'NONE',  ( -5.912764388891193157, 9.912325863766124456, 0.000000000000000000 ) ) ;
#128402=CARTESIAN_POINT ( 'NONE',  ( 7.876360894896227371, 8.153785563659219804, -0.7998128361456341429 ) ) ;
#128403=CARTESIAN_POINT ( 'NONE',  ( -5.596483547390937119, 9.751257581923240991, 0.000000000000000000 ) ) ;
#128417=EDGE_LOOP ( 'NONE', ( #120116, #212261, #190614, #29841 ) ) ;
#128442=CARTESIAN_POINT ( 'NONE',  ( 4.868750418105482147, 8.172599172502351905, -0.9747704861028365642 ) ) ;
#128455=CARTESIAN_POINT ( 'NONE',  ( 4.688087255275310561, 8.691461907788344377, -0.7998128361456381397 ) ) ;
#128458=CARTESIAN_POINT ( 'NONE',  ( -4.817943484809863008, 6.714296380401858499, 1.599625672291263179 ) ) ;
#128462=CARTESIAN_POINT ( 'NONE',  ( -5.750066545527201534, 9.722511713174800008, 0.000000000000000000 ) ) ;
#128473=CARTESIAN_POINT ( 'NONE',  ( 7.693325821111733021, 7.940244644243982464, -0.7998128361456341429 ) ) ;
#128474=CARTESIAN_POINT ( 'NONE',  ( 4.369470645354133431, 8.319742529546998000, 0.7998128361456271485 ) ) ;
#128477=CARTESIAN_POINT ( 'NONE',  ( 4.637309883081485395, 8.320457421531981979, 0.4059539251603030974 ) ) ;
#128481=ORIENTED_EDGE ( 'NONE', *, *, #21723, .F. ) ;
#128489=CARTESIAN_POINT ( 'NONE',  ( 5.742760583840166966, 8.857581893525663830, 1.199719254218452047 ) ) ;
#128498=DIRECTION ( 'NONE',  ( 0.000000000000000000, 0.000000000000000000, 1.000000000000000000 ) ) ;
#128502=CARTESIAN_POINT ( 'NONE',  ( -5.695833931516914639, 6.778132687258748845, 1.082531754730549078 ) ) ;
#128503=CARTESIAN_POINT ( 'NONE',  ( -7.584860592202423035, 7.813701877183096833, -0.7998128361456362523 ) ) ;
#128514=CARTESIAN_POINT ( 'NONE',  ( -4.442231607132987925, 5.211633625523774960, -1.199719254218453823 ) ) ;
#128515=CARTESIAN_POINT ( 'NONE',  ( 6.550524494058025837, 7.671308660269694712, -1.199719254218452047 ) ) ;
#128518=CARTESIAN_POINT ( 'NONE',  ( 3.377389663135653031, 6.954388683717978026, -0.7216878364870338292 ) ) ;
#128524=CYLINDRICAL_SURFACE ( 'NONE', #51312, 1.250000000000000000 ) ;
#128532=DIRECTION ( 'NONE',  ( 1.224646799147353207E-16, 1.000000000000000000, -0.000000000000000000 ) ) ;
#128534=CARTESIAN_POINT ( 'NONE',  ( 6.574778147984297938, 6.635272358928617997, -0.7998128361456481317 ) ) ;
#128536=CARTESIAN_POINT ( 'NONE',  ( -4.305596300791617814, 7.180890229968955651, 1.199719254218452935 ) ) ;
#128550=CARTESIAN_POINT ( 'NONE',  ( 6.034787771858531435, 10.05468647722803865, 0.000000000000000000 ) ) ;
#128552=CARTESIAN_POINT ( 'NONE',  ( -6.038177310039794854, 8.137902509836795417, -1.599625672291271394 ) ) ;
#128553=CARTESIAN_POINT ( 'NONE',  ( 4.505052181490820651, 8.477920988373101707, -0.7998128361456381397 ) ) ;
#128563=CARTESIAN_POINT ( 'NONE',  ( -4.339491684825780737, 7.220434844675483355, -1.199719254218455378 ) ) ;
#128591=CARTESIAN_POINT ( 'NONE',  ( 5.912764389335563919, 6.070849007079172743, -0.7216878364870458196 ) ) ;
#128597=CARTESIAN_POINT ( 'NONE',  ( 4.163762572728282763, 6.911454530608037494, -1.082531754730548412 ) ) ;
#128609=CARTESIAN_POINT ( 'NONE',  ( -5.607179047703544583, 8.699403434699558346, 1.199719254218454489 ) ) ;
#128611=CARTESIAN_POINT ( 'NONE',  ( -8.100070429521727178, 8.414780020722290033, 0.7998128361456341429 ) ) ;
#128618=CARTESIAN_POINT ( 'NONE',  ( 3.065552130021340194, 6.590578228417936835, 0.000000000000000000 ) ) ;
#128623=CARTESIAN_POINT ( 'NONE',  ( -5.608756857104943094, 5.628625835799693888, 0.4592586763518708426 ) ) ;
#128624=CARTESIAN_POINT ( 'NONE',  ( -4.288121723672178476, 8.224835454251337552, -0.7998128361456362523 ) ) ;
#128630=CARTESIAN_POINT ( 'NONE',  ( -5.492461627311929995, 5.580495784718250363, 0.000000000000000000 ) ) ;
#128634=CARTESIAN_POINT ( 'NONE',  ( -6.296835998904160014, 6.311006518335105397, 0.000000000000000000 ) ) ;
#128655=CARTESIAN_POINT ( 'NONE',  ( -6.084577077482911101, 10.32070003369722144, 0.000000000000000000 ) ) ;
#128657=CARTESIAN_POINT ( 'NONE',  ( -6.005335696210345020, 5.970922831858983315, 0.7998128361456281477 ) ) ;
#128658=VERTEX_POINT ( 'NONE', #199963 ) ;
#128681=CARTESIAN_POINT ( 'NONE',  ( -7.117104292530948229, 7.267986194233038155, -0.7998128361456362523 ) ) ;
#128704=CARTESIAN_POINT ( 'NONE',  ( 7.472478939787284169, 8.746922180287201698, 1.199719254218452935 ) ) ;
#128705=CARTESIAN_POINT ( 'NONE',  ( 5.982890925380405456, 10.20206618957764100, 0.000000000000000000 ) ) ;
#128718=CARTESIAN_POINT ( 'NONE',  ( 5.355423173304108886, 7.585870477640591858, 1.239999553246450725 ) ) ;
#128721=CARTESIAN_POINT ( 'NONE',  ( 6.211043768836173484, 8.339580045099285854, 1.443375672974065660 ) ) ;
#128726=CARTESIAN_POINT ( 'NONE',  ( -4.634908411025374875, 6.500755460986618495, 1.599625672291263179 ) ) ;
#128732=CARTESIAN_POINT ( 'NONE',  ( -6.739811759324840779, 7.035737605399991601, -0.7216878364870338292 ) ) ;
#128734=( BOUNDED_SURFACE ( )  B_SPLINE_SURFACE ( 1, 2, ( 
 ( #37430, #198053, #81116, #83233, #203106, #17159, #15025, #149318, #96326, #147202, #213227, #103508, #64859, #212161, #137081, #131004, #69903, #80043, #136013, #53686, #119817, #54751, #120901, #169567, #196996, #16087, #82171, #148265, #49682, #115809, #181797, #33430, #124117, #104584, #190080, #157607, #40658, #126242, #170629, #141390, #22215, #9203, #73115, #155455, #5970, #56887, #24360, #172788, #92622, #76337, #26514, #8128, #41732, #139216, #107841, #55817, #38506, #106759, #123062, #39568, #205246, #158664, #105670, #89406, #121974, #173869, #142444, #207400, #75275, #189016, #90471, #156538, #208452, #187938, #74214, #191137, #154392, #171697, #72040, #140309, #23296, #59019, #206327, #42802, #125175, #88328, #108911, #60084, #174933, #204162, #57952, #138153, #7038, #25443, #91550, #10262, #78467, #63290, #209514, #192203, #45997, #62229, #193287, #144586, #97946, #44932, #28664, #61155, #129450, #15576, #146703, #162935, #12388, #29734, #112116, #81663, #127317, #210600, #130504, #93683, #111040, #11324, #95816, #177047, #212719, #13462, #196491, #64358, #109981, #14516, #213767, #48133, #143519, #178119, #27585, #94749, #179183, #147749, #114246, #80610, #79538, #65388, #30806, #161875, #180243, #194354, #31867, #164000, #128387, #145656, #195433, #43865, #211652, #47062, #113179, #96886, #175991, #159725, #77402, #160797, #132587, #53424, #197537, #37177, #16641, #167187, #66445, #69653, #119561, #49182, #2512, #3578, #35027, #116356, #118497, #20897, #134710, #198589, #200717, #131535, #82725, #148802, #135761, #371, #181291, #185548, #165049, #102181, #115301, #52368, #184479, #152006, #103252, #153066, #36096, #50236, #32918, #182346, #17699, #201784, #101100, #68585, #150948, #168248, #98994, #19847, #85934, #133656, #4643, #33975, #169313, #100050, #86993, #166114, #83786, #149881, #1446, #117428, #51303, #67511, #199657, #183426, #18774, #84860, #72864, #173617, #58765, #89153, #188760, #73952, #25189, #155206, #40400, #206069, #106502, #24113, #90216, #104324, #54500, #71785, #207141 ),
 ( #190881, #123860, #39315, #170372, #158406, #174678, #154140, #21959, #41474, #189825, #171448, #70713, #202852, #156280, #8940, #124919, #5708, #137900, #105410, #6787, #157351, #107584, #42546, #120644, #26251, #23037, #108650, #92369, #203919, #91293, #172529, #75020, #186623, #138970, #141131, #136826, #7864, #38250, #140044, #55567, #88067, #121721, #187686, #204993, #56637, #122801, #57703, #109722, #13208, #79282, #28399, #94494, #160532, #111858, #80345, #46807, #145400, #128127, #97686, #125982, #12137, #45739, #10005, #76081, #211400, #78210, #144334, #161616, #159464, #142182, #210334, #177863, #208197, #64104, #195173, #44670, #96626, #59830, #178933, #146446, #61972, #93425, #194090, #29475, #196237, #63029, #95566, #193018, #129196, #191940, #175729, #113993, #77142, #112921, #30548, #110782, #43605, #162681, #14254, #27323, #11063, #212459, #47880, #130246, #179988, #31611, #143263, #209253, #60897, #127056, #176784, #16387, #69399, #2258, #132334, #48925, #36915, #53177, #32658, #197285, #134466, #68334, #49980, #163744, #81413, #117172, #101928, #3329, #98737, #164795, #198340, #33720, #35850, #200469, #135506, #147495, #119305, #116098, #151760, #201529, #82467, #52116, #67260, #167994, #213516, #182090, #118244, #185291, #100852, #19600, #183174, #148556, #65139, #122, #85672, #66190, #15323, #99798, #17449, #115045, #166938, #18530, #165863, #83533, #149615, #51048, #131295, #184226, #84607, #133398, #181043, #1197, #199402, #34778, #150696, #190623, #106247, #105149, #171189, #40134, #37997, #102998, #22779, #138712, #86741, #157093, #73689, #137645, #189571, #152811, #57446, #24929, #121465, #186362, #187435, #88896, #74764, #172271, #204729, #71535, #154950, #20651, #54250, #206879, #170116, #23858, #6535, #203665, #4389, #56379, #205814, #70460, #104069, #139787, #140867, #41217, #123607, #136577, #72613, #91033, #21702, #39063, #8682, #169054, #89965, #58511, #173347, #122542, #107323, #5455, #188503, #156017, #124666, #7605, #202597, #55315, #120387, #87814, #153886, #110530, #126798 ) ),
 .UNSPECIFIED., .F., .F., .F. ) 
 B_SPLINE_SURFACE_WITH_KNOTS ( ( 2, 2 ),
 ( 3, 2, 2, 2, 2, 2, 2, 2, 2, 2, 2, 2, 2, 2, 2, 2, 2, 2, 2, 2, 2, 2, 2, 2, 2, 2, 2, 2, 2, 2, 2, 2, 2, 2, 2, 2, 2, 2, 2, 2, 2, 2, 2, 2, 2, 2, 2, 2, 2, 2, 2, 2, 2, 2, 2, 2, 2, 2, 2, 2, 2, 2, 2, 2, 2, 2, 2, 2, 2, 2, 2, 2, 2, 2, 2, 2, 2, 2, 2, 2, 2, 2, 2, 2, 2, 2, 2, 2, 2, 2, 2, 2, 2, 2, 2, 2, 2, 2, 2, 2, 2, 2, 2, 2, 2, 2, 2, 2, 2, 2, 2, 2, 2, 2, 2, 2, 2, 2, 2, 2, 3 ),
 ( 0.000000000000000000, 1.000000000000000000 ),
 ( 0.000000000000000000, 0.008333333333333333218, 0.01666666666666666644, 0.02500000000000000139, 0.03333333333333333287, 0.04166666666666666435, 0.05000000000000000278, 0.05833333333333333426, 0.06666666666666666574, 0.07499999999999999722, 0.08333333333333332871, 0.09166666666666666019, 0.1000000000000000056, 0.1083333333333333370, 0.1166666666666666685, 0.1250000000000000000, 0.1333333333333333315, 0.1416666666666666630, 0.1499999999999999944, 0.1583333333333333259, 0.1666666666666666574, 0.1749999999999999889, 0.1833333333333333204, 0.1916666666666666796, 0.2000000000000000111, 0.2083333333333333426, 0.2166666666666666741, 0.2250000000000000056, 0.2333333333333333370, 0.2416666666666666685, 0.2500000000000000000, 0.2583333333333333592, 0.2666666666666666630, 0.2750000000000000222, 0.2833333333333333259, 0.2916666666666666852, 0.2999999999999999889, 0.3083333333333333481, 0.3166666666666666519, 0.3250000000000000111, 0.3333333333333333148, 0.3416666666666666741, 0.3499999999999999778, 0.3583333333333333370, 0.3666666666666666408, 0.3750000000000000000, 0.3833333333333333592, 0.3916666666666666630, 0.4000000000000000222, 0.4083333333333333259, 0.4166666666666666852, 0.4249999999999999889, 0.4333333333333333481, 0.4416666666666666519, 0.4500000000000000111, 0.4583333333333333148, 0.4666666666666666741, 0.4749999999999999778, 0.4833333333333333370, 0.4916666666666666408, 0.5000000000000000000, 0.5083333333333333037, 0.5166666666666667185, 0.5250000000000000222, 0.5333333333333333259, 0.5416666666666666297, 0.5500000000000000444, 0.5583333333333333481, 0.5666666666666666519, 0.5749999999999999556, 0.5833333333333333703, 0.5916666666666666741, 0.5999999999999999778, 0.6083333333333332815, 0.6166666666666666963, 0.6250000000000000000, 0.6333333333333333037, 0.6416666666666667185, 0.6500000000000000222, 0.6583333333333333259, 0.6666666666666666297, 0.6750000000000000444, 0.6833333333333333481, 0.6916666666666666519, 0.6999999999999999556, 0.7083333333333333703, 0.7166666666666666741, 0.7249999999999999778, 0.7333333333333332815, 0.7416666666666666963, 0.7500000000000000000, 0.7583333333333333037, 0.7666666666666667185, 0.7750000000000000222, 0.7833333333333333259, 0.7916666666666666297, 0.8000000000000000444, 0.8083333333333333481, 0.8166666666666666519, 0.8249999999999999556, 0.8333333333333333703, 0.8416666666666666741, 0.8499999999999999778, 0.8583333333333332815, 0.8666666666666666963, 0.8750000000000000000, 0.8833333333333333037, 0.8916666666666667185, 0.9000000000000000222, 0.9083333333333333259, 0.9166666666666666297, 0.9250000000000000444, 0.9333333333333333481, 0.9416666666666666519, 0.9499999999999999556, 0.9583333333333333703, 0.9666666666666666741, 0.9749999999999999778, 0.9833333333333332815, 0.9916666666666666963, 1.000000000000000000 ),
 .UNSPECIFIED. ) 
 GEOMETRIC_REPRESENTATION_ITEM ( )  RATIONAL_B_SPLINE_SURFACE ( (
 ( 1.000000000000000000, 0.8660254037844387076, 1.000000000000000000, 0.8660254037844387076, 1.000000000000000000, 0.8660254037844387076, 1.000000000000000000, 0.8660254037844387076, 1.000000000000000000, 0.8660254037844387076, 1.000000000000000000, 0.8660254037844387076, 1.000000000000000000, 0.8660254037844387076, 1.000000000000000000, 0.8660254037844387076, 1.000000000000000000, 0.8660254037844387076, 1.000000000000000000, 0.8660254037844387076, 1.000000000000000000, 0.8660254037844387076, 1.000000000000000000, 0.8660254037844387076, 1.000000000000000000, 0.8660254037844387076, 1.000000000000000000, 0.8660254037844387076, 1.000000000000000000, 0.8660254037844387076, 1.000000000000000000, 0.8660254037844387076, 1.000000000000000000, 0.8660254037844387076, 1.000000000000000000, 0.8660254037844387076, 1.000000000000000000, 0.8660254037844387076, 1.000000000000000000, 0.8660254037844387076, 1.000000000000000000, 0.8660254037844387076, 1.000000000000000000, 0.8660254037844387076, 1.000000000000000000, 0.8660254037844387076, 1.000000000000000000, 0.8660254037844387076, 1.000000000000000000, 0.8660254037844387076, 1.000000000000000000, 0.8660254037844387076, 1.000000000000000000, 0.8660254037844387076, 1.000000000000000000, 0.8660254037844387076, 1.000000000000000000, 0.8660254037844387076, 1.000000000000000000, 0.8660254037844387076, 1.000000000000000000, 0.8660254037844387076, 1.000000000000000000, 0.8660254037844387076, 1.000000000000000000, 0.8660254037844387076, 1.000000000000000000, 0.8660254037844387076, 1.000000000000000000, 0.8660254037844387076, 1.000000000000000000, 0.8660254037844387076, 1.000000000000000000, 0.8660254037844387076, 1.000000000000000000, 0.8660254037844387076, 1.000000000000000000, 0.8660254037844387076, 1.000000000000000000, 0.8660254037844387076, 1.000000000000000000, 0.8660254037844387076, 1.000000000000000000, 0.8660254037844387076, 1.000000000000000000, 0.8660254037844387076, 1.000000000000000000, 0.8660254037844387076, 1.000000000000000000, 0.8660254037844387076, 1.000000000000000000, 0.8660254037844387076, 1.000000000000000000, 0.8660254037844387076, 1.000000000000000000, 0.8660254037844387076, 1.000000000000000000, 0.8660254037844387076, 1.000000000000000000, 0.8660254037844387076, 1.000000000000000000, 0.8660254037844387076, 1.000000000000000000, 0.8660254037844387076, 1.000000000000000000, 0.8660254037844387076, 1.000000000000000000, 0.8660254037844387076, 1.000000000000000000, 0.8660254037844387076, 1.000000000000000000, 0.8660254037844387076, 1.000000000000000000, 0.8660254037844387076, 1.000000000000000000, 0.8660254037844387076, 1.000000000000000000, 0.8660254037844387076, 1.000000000000000000, 0.8660254037844387076, 1.000000000000000000, 0.8660254037844387076, 1.000000000000000000, 0.8660254037844387076, 1.000000000000000000, 0.8660254037844387076, 1.000000000000000000, 0.8660254037844387076, 1.000000000000000000, 0.8660254037844387076, 1.000000000000000000, 0.8660254037844387076, 1.000000000000000000, 0.8660254037844387076, 1.000000000000000000, 0.8660254037844387076, 1.000000000000000000, 0.8660254037844387076, 1.000000000000000000, 0.8660254037844387076, 1.000000000000000000, 0.8660254037844387076, 1.000000000000000000, 0.8660254037844387076, 1.000000000000000000, 0.8660254037844387076, 1.000000000000000000, 0.8660254037844387076, 1.000000000000000000, 0.8660254037844387076, 1.000000000000000000, 0.8660254037844387076, 1.000000000000000000, 0.8660254037844387076, 1.000000000000000000, 0.8660254037844387076, 1.000000000000000000, 0.8660254037844387076, 1.000000000000000000, 0.8660254037844387076, 1.000000000000000000, 0.8660254037844387076, 1.000000000000000000, 0.8660254037844387076, 1.000000000000000000, 0.8660254037844387076, 1.000000000000000000, 0.8660254037844387076, 1.000000000000000000, 0.8660254037844387076, 1.000000000000000000, 0.8660254037844387076, 1.000000000000000000, 0.8660254037844387076, 1.000000000000000000, 0.8660254037844387076, 1.000000000000000000, 0.8660254037844387076, 1.000000000000000000, 0.8660254037844387076, 1.000000000000000000, 0.8660254037844387076, 1.000000000000000000, 0.8660254037844387076, 1.000000000000000000, 0.8660254037844387076, 1.000000000000000000, 0.8660254037844387076, 1.000000000000000000, 0.8660254037844387076, 1.000000000000000000, 0.8660254037844387076, 1.000000000000000000, 0.8660254037844387076, 1.000000000000000000, 0.8660254037844387076, 1.000000000000000000, 0.8660254037844387076, 1.000000000000000000, 0.8660254037844387076, 1.000000000000000000, 0.8660254037844387076, 1.000000000000000000, 0.8660254037844387076, 1.000000000000000000, 0.8660254037844387076, 1.000000000000000000, 0.8660254037844387076, 1.000000000000000000, 0.8660254037844387076, 1.000000000000000000, 0.8660254037844387076, 1.000000000000000000, 0.8660254037844387076, 1.000000000000000000, 0.8660254037844387076, 1.000000000000000000, 0.8660254037844387076, 1.000000000000000000, 0.8660254037844387076, 1.000000000000000000, 0.8660254037844387076, 1.000000000000000000, 0.8660254037844387076, 1.000000000000000000, 0.8660254037844387076, 1.000000000000000000, 0.8660254037844387076, 1.000000000000000000, 0.8660254037844387076, 1.000000000000000000, 0.8660254037844387076, 1.000000000000000000, 0.8660254037844387076, 1.000000000000000000, 0.8660254037844387076, 1.000000000000000000, 0.8660254037844387076, 1.000000000000000000, 0.8660254037844387076, 1.000000000000000000),
 ( 1.000000000000000000, 0.8660254037844387076, 1.000000000000000000, 0.8660254037844387076, 1.000000000000000000, 0.8660254037844387076, 1.000000000000000000, 0.8660254037844387076, 1.000000000000000000, 0.8660254037844387076, 1.000000000000000000, 0.8660254037844387076, 1.000000000000000000, 0.8660254037844387076, 1.000000000000000000, 0.8660254037844387076, 1.000000000000000000, 0.8660254037844387076, 1.000000000000000000, 0.8660254037844387076, 1.000000000000000000, 0.8660254037844387076, 1.000000000000000000, 0.8660254037844387076, 1.000000000000000000, 0.8660254037844387076, 1.000000000000000000, 0.8660254037844387076, 1.000000000000000000, 0.8660254037844387076, 1.000000000000000000, 0.8660254037844387076, 1.000000000000000000, 0.8660254037844387076, 1.000000000000000000, 0.8660254037844387076, 1.000000000000000000, 0.8660254037844387076, 1.000000000000000000, 0.8660254037844387076, 1.000000000000000000, 0.8660254037844387076, 1.000000000000000000, 0.8660254037844387076, 1.000000000000000000, 0.8660254037844387076, 1.000000000000000000, 0.8660254037844387076, 1.000000000000000000, 0.8660254037844387076, 1.000000000000000000, 0.8660254037844387076, 1.000000000000000000, 0.8660254037844387076, 1.000000000000000000, 0.8660254037844387076, 1.000000000000000000, 0.8660254037844387076, 1.000000000000000000, 0.8660254037844387076, 1.000000000000000000, 0.8660254037844387076, 1.000000000000000000, 0.8660254037844387076, 1.000000000000000000, 0.8660254037844387076, 1.000000000000000000, 0.8660254037844387076, 1.000000000000000000, 0.8660254037844387076, 1.000000000000000000, 0.8660254037844387076, 1.000000000000000000, 0.8660254037844387076, 1.000000000000000000, 0.8660254037844387076, 1.000000000000000000, 0.8660254037844387076, 1.000000000000000000, 0.8660254037844387076, 1.000000000000000000, 0.8660254037844387076, 1.000000000000000000, 0.8660254037844387076, 1.000000000000000000, 0.8660254037844387076, 1.000000000000000000, 0.8660254037844387076, 1.000000000000000000, 0.8660254037844387076, 1.000000000000000000, 0.8660254037844387076, 1.000000000000000000, 0.8660254037844387076, 1.000000000000000000, 0.8660254037844387076, 1.000000000000000000, 0.8660254037844387076, 1.000000000000000000, 0.8660254037844387076, 1.000000000000000000, 0.8660254037844387076, 1.000000000000000000, 0.8660254037844387076, 1.000000000000000000, 0.8660254037844387076, 1.000000000000000000, 0.8660254037844387076, 1.000000000000000000, 0.8660254037844387076, 1.000000000000000000, 0.8660254037844387076, 1.000000000000000000, 0.8660254037844387076, 1.000000000000000000, 0.8660254037844387076, 1.000000000000000000, 0.8660254037844387076, 1.000000000000000000, 0.8660254037844387076, 1.000000000000000000, 0.8660254037844387076, 1.000000000000000000, 0.8660254037844387076, 1.000000000000000000, 0.8660254037844387076, 1.000000000000000000, 0.8660254037844387076, 1.000000000000000000, 0.8660254037844387076, 1.000000000000000000, 0.8660254037844387076, 1.000000000000000000, 0.8660254037844387076, 1.000000000000000000, 0.8660254037844387076, 1.000000000000000000, 0.8660254037844387076, 1.000000000000000000, 0.8660254037844387076, 1.000000000000000000, 0.8660254037844387076, 1.000000000000000000, 0.8660254037844387076, 1.000000000000000000, 0.8660254037844387076, 1.000000000000000000, 0.8660254037844387076, 1.000000000000000000, 0.8660254037844387076, 1.000000000000000000, 0.8660254037844387076, 1.000000000000000000, 0.8660254037844387076, 1.000000000000000000, 0.8660254037844387076, 1.000000000000000000, 0.8660254037844387076, 1.000000000000000000, 0.8660254037844387076, 1.000000000000000000, 0.8660254037844387076, 1.000000000000000000, 0.8660254037844387076, 1.000000000000000000, 0.8660254037844387076, 1.000000000000000000, 0.8660254037844387076, 1.000000000000000000, 0.8660254037844387076, 1.000000000000000000, 0.8660254037844387076, 1.000000000000000000, 0.8660254037844387076, 1.000000000000000000, 0.8660254037844387076, 1.000000000000000000, 0.8660254037844387076, 1.000000000000000000, 0.8660254037844387076, 1.000000000000000000, 0.8660254037844387076, 1.000000000000000000, 0.8660254037844387076, 1.000000000000000000, 0.8660254037844387076, 1.000000000000000000, 0.8660254037844387076, 1.000000000000000000, 0.8660254037844387076, 1.000000000000000000, 0.8660254037844387076, 1.000000000000000000, 0.8660254037844387076, 1.000000000000000000, 0.8660254037844387076, 1.000000000000000000, 0.8660254037844387076, 1.000000000000000000, 0.8660254037844387076, 1.000000000000000000, 0.8660254037844387076, 1.000000000000000000, 0.8660254037844387076, 1.000000000000000000, 0.8660254037844387076, 1.000000000000000000, 0.8660254037844387076, 1.000000000000000000, 0.8660254037844387076, 1.000000000000000000, 0.8660254037844387076, 1.000000000000000000, 0.8660254037844387076, 1.000000000000000000, 0.8660254037844387076, 1.000000000000000000, 0.8660254037844387076, 1.000000000000000000, 0.8660254037844387076, 1.000000000000000000, 0.8660254037844387076, 1.000000000000000000, 0.8660254037844387076, 1.000000000000000000, 0.8660254037844387076, 1.000000000000000000, 0.8660254037844387076, 1.000000000000000000, 0.8660254037844387076, 1.000000000000000000, 0.8660254037844387076, 1.000000000000000000, 0.8660254037844387076, 1.000000000000000000, 0.8660254037844387076, 1.000000000000000000, 0.8660254037844387076, 1.000000000000000000, 0.8660254037844387076, 1.000000000000000000) ) ) 
 REPRESENTATION_ITEM ( '' )  SURFACE ( )  );
#128750=CARTESIAN_POINT ( 'NONE',  ( 3.464990776744291345, 6.200183785247111778, 1.199719254218452047 ) ) ;
#128754=VERTEX_POINT ( 'NONE', #56933 ) ;
#128762=TOROIDAL_SURFACE ( 'NONE', #35280, 3.970406073902761790, 0.08000000000000000167 ) ;
#128767=CARTESIAN_POINT ( 'NONE',  ( -7.262327558775498737, 8.501745569106741840, 1.199719254218452047 ) ) ;
#128770=CARTESIAN_POINT ( 'NONE',  ( 5.020262018810099924, 9.078999131912302900, 0.7998128361456331437 ) ) ;
#128772=CARTESIAN_POINT ( 'NONE',  ( -6.232040409365024125, 6.934648621905299848, 0.8351839086257698552 ) ) ;
#128773=EDGE_CURVE ( 'NONE', #67360, #94475, #15252, .T. ) ;
#128779=CARTESIAN_POINT ( 'NONE',  ( 6.052789233858158369, 6.026285292448116948, 0.000000000000000000 ) ) ;
#128784=CARTESIAN_POINT ( 'NONE',  ( 5.085717018901939390, 5.105960408239938353, 0.000000000000000000 ) ) ;
#128786=CARTESIAN_POINT ( 'NONE',  ( 6.536439455564168277, 6.798469917679251573, 0.7216878364870328300 ) ) ;
#128796=CARTESIAN_POINT ( 'NONE',  ( -4.990809943606273613, 7.876343129965691858, -1.082531754730549967 ) ) ;
#128819=CARTESIAN_POINT ( 'NONE',  ( 5.112833325684902341, 7.058334528089427629, -1.443375672974078316 ) ) ;
#128826=VERTEX_POINT ( 'NONE', #174972 ) ;
#128830=CARTESIAN_POINT ( 'NONE',  ( 6.052789233858158369, 6.026285292448116948, 0.000000000000000000 ) ) ;
#128832=CARTESIAN_POINT ( 'NONE',  ( 6.387826650694035990, 7.481494509678370264, -1.199719254218452047 ) ) ;
#128843=CARTESIAN_POINT ( 'NONE',  ( -4.659162064951642535, 5.464719159645540003, 1.199719254218452935 ) ) ;
#128846=CARTESIAN_POINT ( 'NONE',  ( 3.716343503477301802, 7.349834830783237294, -1.734723475976807094E-15 ) ) ;
#128857=CARTESIAN_POINT ( 'NONE',  ( 5.009736938882257462, 7.905775019223336919, -1.089308093605208194 ) ) ;
#128863=CARTESIAN_POINT ( 'NONE',  ( -6.346625304972878467, 7.537389289624049304, 1.082531754730548412 ) ) ;
#128865=CARTESIAN_POINT ( 'NONE',  ( -5.316205630334268406, 6.335233002545657577, -1.082531754730549967 ) ) ;
#128902=CARTESIAN_POINT ( 'NONE',  ( -6.237633190739009237, 9.434933268240943249, 1.199719254218452047 ) ) ;
#128903=CARTESIAN_POINT ( 'NONE',  ( -4.599258460307840579, 8.480642220064158465, 0.2485357878534207865 ) ) ;
#128906=EDGE_LOOP ( 'NONE', ( #165784, #72537, #208188, #10904 ) ) ;
#128908=CARTESIAN_POINT ( 'NONE',  ( -7.553300976144787349, 8.945177572657957654, -1.082531754730549967 ) ) ;
#128914=CARTESIAN_POINT ( 'NONE',  ( -5.652823702255029836, 5.559658838911111900, -0.7998128361456362523 ) ) ;
#128930=CARTESIAN_POINT ( 'NONE',  ( 3.874598038455354665, 7.742391154831717692, -0.7998128361456362523 ) ) ;
#128943=CARTESIAN_POINT ( 'NONE',  ( 5.045036709957831711, 4.903268083610561767, 0.3063280728123271568 ) ) ;
#128953=CARTESIAN_POINT ( 'NONE',  ( 6.201928923608456046, 6.200281597156833691, 0.7998128361456352531 ) ) ;
#128954=CARTESIAN_POINT ( 'NONE',  ( 5.194709132691408549, 6.089524072008651423, 1.199719254218452935 ) ) ;
#128956=CARTESIAN_POINT ( 'NONE',  ( 3.902768115887398803, 5.646591783325653147, -1.599625672291269396 ) ) ;
#128969=CARTESIAN_POINT ( 'NONE',  ( 4.628438946891473726, 8.448539137754004003, 0.3726521946380862427 ) ) ;
#128971=CARTESIAN_POINT ( 'NONE',  ( -5.980555156959541208, 7.110307450275150210, 1.082531754730549078 ) ) ;
#128992=CARTESIAN_POINT ( 'NONE',  ( -5.607123201593087636, 5.580137643357920396, -0.3617017252367187852 ) ) ;
#129000=CARTESIAN_POINT ( 'NONE',  ( 5.017399365509065845, 8.011327138806002779, -1.199719254218450271 ) ) ;
#129002=CARTESIAN_POINT ( 'NONE',  ( 3.413620815590684199, 7.204584394822967752, 0.7998128361456281477 ) ) ;
#129021=CARTESIAN_POINT ( 'NONE',  ( -5.921879234118920365, 10.13088588310589699, 0.000000000000000000 ) ) ;
#129034=CARTESIAN_POINT ( 'NONE',  ( 6.703580607314123085, 6.785541894813420072, 0.000000000000000000 ) ) ;
#129040=CARTESIAN_POINT ( 'NONE',  ( 5.550083779947807550, 7.568460058062819407, -1.599625672291283607 ) ) ;
#129048=EDGE_CURVE ( 'NONE', #138779, #128826, #192244, .T. ) ;
#129052=CARTESIAN_POINT ( 'NONE',  ( -0.3642516066350167114, 3.313053037719472016, 1.968202613562980430 ) ) ;
#129053=CARTESIAN_POINT ( 'NONE',  ( 4.597294405107005488, 8.370805622008914426, 0.1071034531749150143 ) ) ;
#129068=CARTESIAN_POINT ( 'NONE',  ( -6.205606397109380445, 6.952550393956807184, 0.8692890898145851919 ) ) ;
#129075=CARTESIAN_POINT ( 'NONE',  ( -4.782994330570982555, 8.802186828966616972, 0.000000000000000000 ) ) ;
#129077=CARTESIAN_POINT ( 'NONE',  ( 5.631432701629774051, 7.663367133358481631, 1.599625672291269396 ) ) ;
#129081=CARTESIAN_POINT ( 'NONE',  ( -5.264308783856126439, 9.363720357799287797, -0.7998128361456362523 ) ) ;
#129089=CARTESIAN_POINT ( 'NONE',  ( -6.358822508390924888, 6.928531665952419871, -0.8607971499900844981 ) ) ;
#129101=DIRECTION ( 'NONE',  ( 0.000000000000000000, 0.000000000000000000, 1.000000000000000000 ) ) ;
#129106=ORIENTED_EDGE ( 'NONE', *, *, #88854, .T. ) ;
#129107=CARTESIAN_POINT ( 'NONE',  ( 5.966997003790217136, 8.054858819212300958, -1.443375672974078761 ) ) ;
#129120=CARTESIAN_POINT ( 'NONE',  ( -3.838381494955496187, 7.492212646896947881, -0.0007785181141982987826 ) ) ;
#129121=CARTESIAN_POINT ( 'NONE',  ( -5.316205630334268406, 6.335233002545657577, -1.082531754730549967 ) ) ;
#129125=CARTESIAN_POINT ( 'NONE',  ( 4.386945222473598527, 7.275797305264619652, -1.199719254218452047 ) ) ;
#129129=LINE ( 'NONE', #196174, #193992 ) ;
#129141=CARTESIAN_POINT ( 'NONE',  ( 5.764827401431699805, 7.068052664419874453, 2.440105445505980519 ) ) ;
#129144=CARTESIAN_POINT ( 'NONE',  ( 6.983858524370772258, 9.241197259889668558, 1.443375672974063439 ) ) ;
#129156=ORIENTED_EDGE ( 'NONE', *, *, #131609, .F. ) ;
#129176=CARTESIAN_POINT ( 'NONE',  ( 2.878073747850912412, 6.579779482459851003, -0.7998128361456362523 ) ) ;
#129180=CARTESIAN_POINT ( 'NONE',  ( -5.926322542504884439, 6.086666852443364029, -0.7216878364870338292 ) ) ;
#129186=CARTESIAN_POINT ( 'NONE',  ( -6.123442655227560927, 7.173046514967467147, 1.199719254218452047 ) ) ;
#129196=CARTESIAN_POINT ( 'NONE',  ( -5.601453741101424022, 6.564059448486966986, -1.199719254218453823 ) ) ;
#129199=CARTESIAN_POINT ( 'NONE',  ( 6.013528089337225602, 7.174620582783560963, 1.187335689305318853 ) ) ;
#129204=CARTESIAN_POINT ( 'NONE',  ( 4.844006021832467646, 8.873367135438366304, 0.000000000000000000 ) ) ;
#129212=CARTESIAN_POINT ( 'NONE',  ( -3.709037541790315640, 6.484905011134099340, -1.199719254218450271 ) ) ;
#129216=CARTESIAN_POINT ( 'NONE',  ( -5.472651281771599763, 6.413789912602166687, 1.199719254218452935 ) ) ;
#129221=CARTESIAN_POINT ( 'NONE',  ( 5.465345319640213972, 8.429967735338637524, -1.082531754730548412 ) ) ;
#129223=CARTESIAN_POINT ( 'NONE',  ( -6.251718229232856139, 8.387033582228697881, -1.443375672974066548 ) ) ;
#129230=CARTESIAN_POINT ( 'NONE',  ( 4.355912491740495440, 8.303924683664389406, 0.000000000000000000 ) ) ;
#129262=CARTESIAN_POINT ( 'NONE',  ( 4.784634885068531851, 8.146353749921887655, 0.8039021629790907841 ) ) ;
#129270=ORIENTED_EDGE ( 'NONE', *, *, #20366, .F. ) ;
#129274=CARTESIAN_POINT ( 'NONE',  ( -6.152945810502786550, 6.988564382810744213, -0.9301526061148736035 ) ) ;
#129277=VERTEX_POINT ( 'NONE', #166156 ) ;
#129280=CARTESIAN_POINT ( 'NONE',  ( -6.583366107887490770, 9.838288338247510367, 1.199719254218452935 ) ) ;
#129290=CARTESIAN_POINT ( 'NONE',  ( -5.004894982100124068, 5.868074229652107121, 1.199719254218452935 ) ) ;
#129301=CARTESIAN_POINT ( 'NONE',  ( 4.878955176071345434, 6.785476686873604280, -1.599625672291269396 ) ) ;
#129304=CARTESIAN_POINT ( 'NONE',  ( 6.685579144870162693, 6.972466221869550118, -0.7216878364870458196 ) ) ;
#129313=DIRECTION ( 'NONE',  ( 0.000000000000000000, 1.000000000000000000, 0.000000000000000000 ) ) ;
#129320=CARTESIAN_POINT ( 'NONE',  ( -5.255720823952942489, 6.160704378480398979, -1.199719254218453823 ) ) ;
#129321=CARTESIAN_POINT ( 'NONE',  ( 4.848976215542928792, 5.686169002002086970, 1.199719254218452047 ) ) ;
#129332=CARTESIAN_POINT ( 'NONE',  ( -7.584860592202423035, 7.813701877183096833, -0.7998128361456362523 ) ) ;
#129333=CARTESIAN_POINT ( 'NONE',  ( 5.332099551924443404, 9.442809587212341427, 0.000000000000000000 ) ) ;
#129335=CARTESIAN_POINT ( 'NONE',  ( -3.147653791585730776, 8.919999999999991047, -2.500000000000000444 ) ) ;
#129345=CARTESIAN_POINT ( 'NONE',  ( -6.596192096975760144, 6.770415987340496322, 0.2575442448356154990 ) ) ;
#129353=CARTESIAN_POINT ( 'NONE',  ( -4.624739795592948788, 5.528522862014106920, -1.082531754730549967 ) ) ;
#129354=EDGE_CURVE ( 'NONE', #116379, #172448, #62292, .T. ) ;
#129359=CARTESIAN_POINT ( 'NONE',  ( -5.408618258607211793, 6.146265696677264856, -1.009999807746956524 ) ) ;
#129368=CARTESIAN_POINT ( 'NONE',  ( 5.020262018810099924, 9.078999131912302900, 0.7998128361456331437 ) ) ;
#129401=CARTESIAN_POINT ( 'NONE',  ( 2.878073747850912412, 6.579779482459851003, -0.7998128361456362523 ) ) ;
#129431=CARTESIAN_POINT ( 'NONE',  ( -5.306037014901836990, 7.283738832175834510, 1.599625672291263179 ) ) ;
#129434=CARTESIAN_POINT ( 'NONE',  ( 5.329763783503544516, 9.232158490813878515, -0.7216878364870458196 ) ) ;
#129439=CARTESIAN_POINT ( 'NONE',  ( -4.281342646865346602, 8.216926531310035031, 0.7998128361456352531 ) ) ;
#129445=CARTESIAN_POINT ( 'NONE',  ( -4.496464221587651799, 5.274905009054215554, 1.199719254218452935 ) ) ;
#129450=CARTESIAN_POINT ( 'NONE',  ( -4.274563570058511175, 8.209017608368725405, 0.000000000000000000 ) ) ;
#129460=CARTESIAN_POINT ( 'NONE',  ( -4.014095998097799267, 6.840806543492835345, -1.199719254218450271 ) ) ;
#129463=CARTESIAN_POINT ( 'NONE',  ( -5.858531774880906262, 6.967946837850073294, 1.082531754730549078 ) ) ;
#129465=CARTESIAN_POINT ( 'NONE',  ( -5.424670858799220063, 9.342883411992149334, 0.000000000000000000 ) ) ;
#129466=CARTESIAN_POINT ( 'NONE',  ( 5.515134625708930649, 9.656350506627580543, 0.000000000000000000 ) ) ;
#129467=CARTESIAN_POINT ( 'NONE',  ( -6.607619761813764647, 8.802252036906432764, 1.599625672291269396 ) ) ;
#129505=CARTESIAN_POINT ( 'NONE',  ( 4.745935331938881951, 8.308991367555595531, -0.7587592799198628057 ) ) ;
#129519=CARTESIAN_POINT ( 'NONE',  ( 6.170896192875352959, 7.228408975556602556, 1.199719254218453823 ) ) ;
#129522=CARTESIAN_POINT ( 'NONE',  ( -6.330731382938325602, 6.350551133041632212, 0.7998128361456281477 ) ) ;
#129526=CARTESIAN_POINT ( 'NONE',  ( -7.444835747235459600, 8.818634805597074688, 1.082531754730549078 ) ) ;
#129536=CARTESIAN_POINT ( 'NONE',  ( 4.037295881819344956, 7.932205305423046582, -0.7998128361456362523 ) ) ;
#129538=CARTESIAN_POINT ( 'NONE',  ( 7.991605200612358573, 8.288237253661408843, 0.7998128361456281477 ) ) ;
#129545=CARTESIAN_POINT ( 'NONE',  ( 4.760848217054122422, 5.583353003765119560, -1.199719254218452047 ) ) ;
#129551=CARTESIAN_POINT ( 'NONE',  ( 7.212011367826596242, 7.378711115411311638, 0.000000000000000000 ) ) ;
#129561=CARTESIAN_POINT ( 'NONE',  ( -4.448483799059637533, 7.243629294661272588, 1.082531754730549967 ) ) ;
#129562=CARTESIAN_POINT ( 'NONE',  ( 4.746763178560250651, 7.591621904078704297, 1.082531754730549078 ) ) ;
#129574=DIRECTION ( 'NONE',  ( 0.6507913734559641616, -0.7592566023653004592, 0.000000000000000000 ) ) ;
#129575=CARTESIAN_POINT ( 'NONE',  ( -7.105881907338169157, 8.423188659050232729, -1.082531754730549967 ) ) ;
#129576=CARTESIAN_POINT ( 'NONE',  ( 8.025500584646550806, 8.327781868367935658, 0.000000000000000000 ) ) ;
#129579=CARTESIAN_POINT ( 'NONE',  ( 8.039058738260216330, 8.343599714250547805, -0.7998128361456341429 ) ) ;
#129592=CARTESIAN_POINT ( 'NONE',  ( -5.864945314351738936, 6.621640825619397042, 0.9118253242758539434 ) ) ;
#129596=CARTESIAN_POINT ( 'NONE',  ( 6.398522151006641678, 6.429640362454684954, 0.000000000000000000 ) ) ;
#129598=CARTESIAN_POINT ( 'NONE',  ( -5.492988512192097161, 6.437516681426083132, 1.199719254218452935 ) ) ;
#129612=CARTESIAN_POINT ( 'NONE',  ( 7.702440666339465558, 8.158804663583751449, -0.7216878364870317197 ) ) ;
#129614=CARTESIAN_POINT ( 'NONE',  ( -7.228432174741334038, 8.462200954400218578, -1.199719254218452047 ) ) ;
#129615=CARTESIAN_POINT ( 'NONE',  ( 5.825163275726873202, 6.825053905550038991, 1.199719254218452047 ) ) ;
#129625=CARTESIAN_POINT ( 'NONE',  ( -5.309953438407606363, 6.223975762010839574, 1.199719254218452935 ) ) ;
#129654=CARTESIAN_POINT ( 'NONE',  ( 4.746763178560261309, 5.670883475476017566, 1.082531754730549078 ) ) ;
#129661=CARTESIAN_POINT ( 'NONE',  ( 4.217995187182915551, 7.935095128439824563, 0.7216878364870257245 ) ) ;
#129674=CARTESIAN_POINT ( 'NONE',  ( -6.143779885648060102, 7.196773283791382703, 1.199719254218452047 ) ) ;
#129676=CARTESIAN_POINT ( 'NONE',  ( -7.286581212701773502, 7.465709267765667789, 0.7998128361456341429 ) ) ;
#129683=CARTESIAN_POINT ( 'NONE',  ( 4.882344714252594642, 4.868692719482363707, 0.000000000000000000 ) ) ;
#129688=CARTESIAN_POINT ( 'NONE',  ( 5.575758015699216585, 5.849789923344298259, -0.7899890411014517388 ) ) ;
#129689=CARTESIAN_POINT ( 'NONE',  ( -5.478376588373717659, 8.549133898814758936, -1.199719254218452047 ) ) ;
#129695=CARTESIAN_POINT ( 'NONE',  ( -4.502716413514301408, 7.306900678191715848, -1.082531754730549967 ) ) ;
#129699=CARTESIAN_POINT ( 'NONE',  ( -3.962726036944197894, 7.845207153068690431, -0.7998128361456481317 ) ) ;
#129713=CARTESIAN_POINT ( 'NONE',  ( -6.512525376672311239, 6.817996978042812906, 0.6578840964387155932 ) ) ;
#129718=VERTEX_POINT ( 'NONE', #143192 ) ;
#129719=CARTESIAN_POINT ( 'NONE',  ( -6.851666526859749418, 9.086973262793417661, -1.599625672291271394 ) ) ;
#129720=CARTESIAN_POINT ( 'NONE',  ( 5.096939404094710468, 4.911127157724081371, 0.000000000000000000 ) ) ;
#129721=CARTESIAN_POINT ( 'NONE',  ( -6.154475385960665790, 6.144919136567696505, 0.000000000000000000 ) ) ;
#129730=CARTESIAN_POINT ( 'NONE',  ( 4.543390873910903238, 7.354354215321133204, 1.082531754730548412 ) ) ;
#129746=CARTESIAN_POINT ( 'NONE',  ( -6.688968683495758683, 8.897159112202094988, -1.599625672291271394 ) ) ;
#129771=CARTESIAN_POINT ( 'NONE',  ( 8.025500584646550806, 8.327781868367935658, 0.000000000000000000 ) ) ;
#129772=CARTESIAN_POINT ( 'NONE',  ( 5.885121196783658526, 9.023669275293071834, 1.199719254218452047 ) ) ;
#129786=CARTESIAN_POINT ( 'NONE',  ( 5.324837791525375508, 7.612559486139466536, 1.234112182050936646 ) ) ;
#129788=CARTESIAN_POINT ( 'NONE',  ( 6.590672070018850803, 7.822110515511036866, -1.082531754730548412 ) ) ;
#129795=CARTESIAN_POINT ( 'NONE',  ( -4.122561227007127016, 6.967349310553715647, 1.199719254218452935 ) ) ;
#129805=CARTESIAN_POINT ( 'NONE',  ( -5.375696267714453747, 6.397419496268610395, 1.092131393413272811 ) ) ;
#129810=CARTESIAN_POINT ( 'NONE',  ( -4.285259070371116863, 7.157163461145040095, 1.199719254218452935 ) ) ;
#129819=CARTESIAN_POINT ( 'NONE',  ( 5.032011289327418702, 5.899709921417326974, 1.199719254218452935 ) ) ;
#129838=CARTESIAN_POINT ( 'NONE',  ( -6.454563648557663846, 9.688018802362710957, -1.199719254218452047 ) ) ;
#129841=CARTESIAN_POINT ( 'NONE',  ( 6.180537922983273091, 8.303989891604203422, -1.599625672291281386 ) ) ;
#129843=CARTESIAN_POINT ( 'NONE',  ( -5.568215224448921141, 7.423109701660543180, 1.245465753432648093 ) ) ;
#129849=CARTESIAN_POINT ( 'NONE',  ( 4.030516805012513082, 7.924296382481737844, 0.000000000000000000 ) ) ;
#129855=CARTESIAN_POINT ( 'NONE',  ( 3.553645660557675612, 6.199651466408984568, -1.082531754730549967 ) ) ;
#129860=CARTESIAN_POINT ( 'NONE',  ( 7.200788982633824276, 7.573544365927161515, 0.000000000000000000 ) ) ;
#129872=CARTESIAN_POINT ( 'NONE',  ( -4.651856103264620401, 8.441266197201775512, 0.000000000000000000 ) ) ;
#129905=CARTESIAN_POINT ( 'NONE',  ( 4.179656494762836516, 8.098292687190454586, -0.7998128361456362523 ) ) ;
#129907=CARTESIAN_POINT ( 'NONE',  ( 5.468734858265785093, 7.473552982767158070, 1.599625672291269396 ) ) ;
#129920=CARTESIAN_POINT ( 'NONE',  ( -6.943184063974175757, 9.193743722760251202, -1.443375672974066548 ) ) ;
#129923=CARTESIAN_POINT ( 'NONE',  ( 5.682275777458854371, 5.801945626556378244, 0.7216878364870328300 ) ) ;
#129936=CARTESIAN_POINT ( 'NONE',  ( -4.977251789992602760, 8.820894498384422633, 0.000000000000000000 ) ) ;
#129938=CARTESIAN_POINT ( 'NONE',  ( -5.994113311017573054, 6.165756082374834079, 0.7216878364870257245 ) ) ;
#129945=CARTESIAN_POINT ( 'NONE',  ( -5.443788192324133135, 7.193024429787462815, -1.249999997929073237 ) ) ;
#129967=CARTESIAN_POINT ( 'NONE',  ( -4.950662367645459305, 5.804802846121667415, -1.199719254218453823 ) ) ;
#129977=CARTESIAN_POINT ( 'NONE',  ( -5.427006627220116286, 9.553534508390610469, -0.7998128361456362523 ) ) ;
#129978=CARTESIAN_POINT ( 'NONE',  ( -4.973494386576447823, 8.059877448926631160, 1.114414082037382236 ) ) ;
#129983=CARTESIAN_POINT ( 'NONE',  ( -5.346851039111044201, 6.199209027673978412, 7.500000000000000000 ) ) ;
#129987=CARTESIAN_POINT ( 'NONE',  ( -4.817943484809863008, 6.714296380401858499, 1.599625672291263179 ) ) ;
#129998=CARTESIAN_POINT ( 'NONE',  ( 4.376249722160992839, 8.327651452488305850, 0.000000000000000000 ) ) ;
#130004=EDGE_CURVE ( 'NONE', #137303, #120691, #194765, .T. ) ;
#130021=CARTESIAN_POINT ( 'NONE',  ( 6.039231080244466199, 6.010467446565510130, 0.7998128361456352531 ) ) ;
#130022=CARTESIAN_POINT ( 'NONE',  ( 4.167152111353856547, 5.955039778036558040, 1.599625672291262513 ) ) ;
#130024=CARTESIAN_POINT ( 'NONE',  ( 3.984117037569365305, 5.741498858621315371, 1.599625672291261402 ) ) ;
#130027=CARTESIAN_POINT ( 'NONE',  ( -5.356880090730904875, 7.343055753976412525, 1.443375672974058777 ) ) ;
#130035=CARTESIAN_POINT ( 'NONE',  ( 4.783863686166085039, 8.265937597628173705, 0.8363946479656783062 ) ) ;
#130036=CARTESIAN_POINT ( 'NONE',  ( -6.102578539482539810, 6.292298848917299736, 0.000000000000000000 ) ) ;
#130037=FACE_OUTER_BOUND ( 'NONE', #111772, .T. ) ;
#130057=CARTESIAN_POINT ( 'NONE',  ( -3.947104627881229622, 8.980740528189222971, 0.7749999999999996891 ) ) ;
#130060=AXIS2_PLACEMENT_3D ( 'NONE', #22802, #205835, #91052 ) ;
#130064=CARTESIAN_POINT ( 'NONE',  ( 4.529305835417093640, 7.441884687032027657, -1.199719254218450271 ) ) ;
#130066=CARTESIAN_POINT ( 'NONE',  ( 4.435452530326143616, 5.203724702582467998, -1.199719254218452047 ) ) ;
#130082=CARTESIAN_POINT ( 'NONE',  ( -7.608060475923978494, 8.905100639113307182, 1.199719254218452047 ) ) ;
#130092=CARTESIAN_POINT ( 'NONE',  ( 5.063152511717405879, 4.908155404373435005, -0.2552525419090029835 ) ) ;
#130094=CARTESIAN_POINT ( 'NONE',  ( 5.692444392891300886, 7.734547439830227411, -1.599625672291281386 ) ) ;
#130099=CARTESIAN_POINT ( 'NONE',  ( 5.254667053748194760, 8.288139441751686931, 1.199719254218452047 ) ) ;
#130109=CARTESIAN_POINT ( 'NONE',  ( -1.858560999665793911, 8.965769984707671725, 0.7750000000000013545 ) ) ;
#130110=AXIS2_PLACEMENT_3D ( 'NONE', #111580, #112649, #178658 ) ;
#130112=CARTESIAN_POINT ( 'NONE',  ( 4.620579464570812256, 8.341333509328540785, -0.3192730525469981151 ) ) ;
#130120=CARTESIAN_POINT ( 'NONE',  ( 6.061904079085887354, 6.244845311787889486, 0.000000000000000000 ) ) ;
#130128=CARTESIAN_POINT ( 'NONE',  ( -6.096963755015523567, 7.027332905876572333, 0.9867296136132864826 ) ) ;
#130135=CARTESIAN_POINT ( 'NONE',  ( -5.468734858265826837, 7.473552982767158070, 1.599625672291263179 ) ) ;
#130137=CARTESIAN_POINT ( 'NONE',  ( 5.254667053748194760, 8.288139441751686931, 1.199719254218452047 ) ) ;
#130140=CARTESIAN_POINT ( 'NONE',  ( -6.994027139803241866, 9.253060644560830994, -1.599625672291271394 ) ) ;
#130147=CARTESIAN_POINT ( 'NONE',  ( -0.3349625572557037856, 2.646409141035024781, -1.974606604270766619 ) ) ;
#130161=CARTESIAN_POINT ( 'NONE',  ( 6.373741612200171325, 7.569024981389272710, 1.082531754730549967 ) ) ;
#130163=CARTESIAN_POINT ( 'NONE',  ( 4.318600669050608687, 4.999583595936801572, -2.499999999999996891 ) ) ;
#130176=CARTESIAN_POINT ( 'NONE',  ( -4.719646871332968452, 5.639247783710797712, 1.082531754730549078 ) ) ;
#130178=CARTESIAN_POINT ( 'NONE',  ( 6.412080304620304538, 6.445458208337293549, -0.7998128361456481317 ) ) ;
#130227=CARTESIAN_POINT ( 'NONE',  ( -4.163573865134853058, 7.871543801636343929, 0.01019316184158518962 ) ) ;
#130230=CARTESIAN_POINT ( 'NONE',  ( -5.167065940139584868, 6.161236697318522637, 1.082531754730549078 ) ) ;
#130236=VERTEX_POINT ( 'NONE', #4312 ) ;
#130237=CARTESIAN_POINT ( 'NONE',  ( -5.204350862799341115, 7.165104988056252289, -1.599625672291271394 ) ) ;
#130246=CARTESIAN_POINT ( 'NONE',  ( -6.330731382938325602, 6.350551133041632212, 0.7998128361456281477 ) ) ;
#130249=CARTESIAN_POINT ( 'NONE',  ( 6.257994703896152089, 7.000112715747270009, 0.9732540237740094913 ) ) ;
#130254=CARTESIAN_POINT ( 'NONE',  ( 6.475954649182838807, 7.584310507915338562, 1.199719254218452047 ) ) ;
#130263=CARTESIAN_POINT ( 'NONE',  ( -3.657667580636712934, 7.489305620709952649, -0.7998128361456481317 ) ) ;
#130268=CARTESIAN_POINT ( 'NONE',  ( -4.613517410400161722, 8.604463755433990002, -0.7998128361456362523 ) ) ;
#130272=CARTESIAN_POINT ( 'NONE',  ( 5.356880090730857802, 8.303424968277756335, 1.082531754730548412 ) ) ;
#130275=CARTESIAN_POINT ( 'NONE',  ( -4.950135482320914271, 8.789258806100786359, -0.7216878364870338292 ) ) ;
#130281=CARTESIAN_POINT ( 'NONE',  ( 5.716698046817569434, 6.698511138489155137, -1.199719254218452047 ) ) ;
#130310=CARTESIAN_POINT ( 'NONE',  ( 4.693755526227673336, 8.251780594207492214, -0.6034641085399840010 ) ) ;
#130318=CARTESIAN_POINT ( 'NONE',  ( 8.154303043976348420, 8.478051404252736845, 0.7998128361456281477 ) ) ;
#130323=CARTESIAN_POINT ( 'NONE',  ( -5.686128154004278734, 7.329579007619248188, -1.223094714244008729 ) ) ;
#130331=CARTESIAN_POINT ( 'NONE',  ( -4.841670253411603397, 5.781608396135871075, 1.082531754730549078 ) ) ;
#130342=CARTESIAN_POINT ( 'NONE',  ( -5.652823702255029836, 5.559658838911111900, -0.7998128361456362523 ) ) ;
#130352=CARTESIAN_POINT ( 'NONE',  ( 6.378184920586140727, 6.405913593630768510, 0.000000000000000000 ) ) ;
#130355=CARTESIAN_POINT ( 'NONE',  ( 6.875393295461478260, 8.154285278527437342, -1.082531754730548412 ) ) ;
#130359=EDGE_CURVE ( 'NONE', #197229, #160913, #162615, .T. ) ;
#130370=CARTESIAN_POINT ( 'NONE',  ( -5.635349125135588721, 6.603604063193491136, 1.199719254218452935 ) ) ;
#130372=CARTESIAN_POINT ( 'NONE',  ( 3.067887898442204442, 6.801229324816399746, 0.7998128361456271485 ) ) ;
#130383=CARTESIAN_POINT ( 'NONE',  ( -5.576146316970437944, 9.727530813099326323, 0.000000000000000000 ) ) ;
#130384=CARTESIAN_POINT ( 'NONE',  ( 5.342795052237045539, 8.390955439988655229, -1.199719254218450271 ) ) ;
#130389=CARTESIAN_POINT ( 'NONE',  ( 3.366167277942881064, 7.149221934233827014, -0.7998128361456362523 ) ) ;
#130397=CARTESIAN_POINT ( 'NONE',  ( -6.483603504774570148, 6.769331023298949646, -0.2299166613418425487 ) ) ;
#130408=CARTESIAN_POINT ( 'NONE',  ( -4.950135482320939140, 4.947781948895412008, -0.7216878364870338292 ) ) ;
#130414=EDGE_CURVE ( 'NONE', #145598, #176704, #78147, .T. ) ;
#130448=VERTEX_POINT ( 'NONE', #212396 ) ;
#130456=CARTESIAN_POINT ( 'NONE',  ( 3.902768115887398803, 5.646591783325653147, -1.599625672291269396 ) ) ;
#130457=CARTESIAN_POINT ( 'NONE',  ( -4.719646871332968452, 5.639247783710797712, 1.082531754730549078 ) ) ;
#130488=CARTESIAN_POINT ( 'NONE',  ( -5.010620288702242853, 8.003418215864698482, -1.199719254218453823 ) ) ;
#130491=CARTESIAN_POINT ( 'NONE',  ( 5.926322542504858681, 8.007405281046052536, -1.443375672974078761 ) ) ;
#130496=CARTESIAN_POINT ( 'NONE',  ( -6.967964602780620353, 7.093989889524320525, 0.000000000000000000 ) ) ;
#130504=CARTESIAN_POINT ( 'NONE',  ( -4.936050443827081580, 7.916420063510339666, 1.199719254218452935 ) ) ;
#130515=CARTESIAN_POINT ( 'NONE',  ( -6.445975688654487001, 6.485002823043819475, -0.7998128361456362523 ) ) ;
#130518=CARTESIAN_POINT ( 'NONE',  ( -6.129694847154220305, 8.244672969803623630, -1.443375672974066548 ) ) ;
#130519=CARTESIAN_POINT ( 'NONE',  ( -7.553300976144794454, 7.984808358356614733, -0.7216878364870338292 ) ) ;
#130520=CARTESIAN_POINT ( 'NONE',  ( 5.528692779322568640, 9.672168352510192690, 0.7998128361456341429 ) ) ;
#130521=CARTESIAN_POINT ( 'NONE',  ( -7.282664789195997912, 8.525472337930658284, 1.199719254218452047 ) ) ;
#130539=CARTESIAN_POINT ( 'NONE',  ( -1.845715822548411822, 2.495237285644507086, -2.490652812252487358 ) ) ;
#130559=CARTESIAN_POINT ( 'NONE',  ( 6.206332990038123221, 6.936436922908462144, -0.8583981852504622978 ) ) ;
#130576=CARTESIAN_POINT ( 'NONE',  ( -4.522526758610270647, 7.433975764090723359, -1.199719254218453823 ) ) ;
#130580=CARTESIAN_POINT ( 'NONE',  ( -8.054952659850432184, 8.570068656013202002, 0.000000000000000000 ) ) ;
#130591=CARTESIAN_POINT ( 'NONE',  ( 6.059568310664962709, 6.034194215389424798, 0.7998128361456352531 ) ) ;
#130593=CARTESIAN_POINT ( 'NONE',  ( 5.668190738965027897, 8.770583741171307679, -1.199719254218452047 ) ) ;
#130607=CARTESIAN_POINT ( 'NONE',  ( 7.049313524462606395, 7.188896964819984525, 0.000000000000000000 ) ) ;
#130617=CARTESIAN_POINT ( 'NONE',  ( -4.828112100242279325, 8.646898193675708555, -0.7216878364870338292 ) ) ;
#130619=CARTESIAN_POINT ( 'NONE',  ( 6.387299765813869712, 6.624473612970537495, 0.000000000000000000 ) ) ;
#130625=AXIS2_PLACEMENT_3D ( 'NONE', #97377, #110480, #15014 ) ;
#130628=VERTEX_POINT ( 'NONE', #134401 ) ;
#130630=CARTESIAN_POINT ( 'NONE',  ( -7.444835747679825033, 7.858265591814152629, 0.000000000000000000 ) ) ;
#130631=CARTESIAN_POINT ( 'NONE',  ( 7.014364370223726830, 9.276787413384745662, -1.599625672291269396 ) ) ;
#130634=CARTESIAN_POINT ( 'NONE',  ( 4.204437033569277560, 7.919277282557212416, 0.000000000000000000 ) ) ;
#130639=DIRECTION ( 'NONE',  ( 0.7592566023653005702, 0.6507913734559639396, 0.000000000000000000 ) ) ;
#130651=CARTESIAN_POINT ( 'NONE',  ( 4.376249722160992839, 8.327651452488305850, 0.000000000000000000 ) ) ;
#130653=CARTESIAN_POINT ( 'NONE',  ( -4.842197138736131556, 5.678260079060780008, 1.199719254218452935 ) ) ;
#130667=ADVANCED_FACE ( 'NONE', ( #184165 ), #3263, .T. ) ;
#130668=CARTESIAN_POINT ( 'NONE',  ( 6.211043768836173484, 8.339580045099285854, 1.443375672974065660 ) ) ;
#130670=CARTESIAN_POINT ( 'NONE',  ( -6.444921918449773024, 8.612437886315108315, 1.599625672291269396 ) ) ;
#130671=CARTESIAN_POINT ( 'NONE',  ( 6.879836604291781121, 6.991173891287354003, -0.7998128361456341429 ) ) ;
#130679=CARTESIAN_POINT ( 'NONE',  ( -4.776215253764153346, 8.794277906025310898, -0.7998128361456362523 ) ) ;
#130706=CARTESIAN_POINT ( 'NONE',  ( 5.573810548993915148, 5.675402860013913475, 0.000000000000000000 ) ) ;
#130712=CARTESIAN_POINT ( 'NONE',  ( 5.682275777458854371, 5.801945626556378244, 0.7216878364870328300 ) ) ;
#130723=CARTESIAN_POINT ( 'NONE',  ( -4.945692173934974178, 8.992000979557944973, 0.000000000000000000 ) ) ;
#130725=CARTESIAN_POINT ( 'NONE',  ( -6.936931872047518155, 8.122117267924091166, 1.199719254218452047 ) ) ;
#130731=CARTESIAN_POINT ( 'NONE',  ( 6.984385409695311964, 8.177479728513226576, 1.199719254218452935 ) ) ;
#130736=FACE_OUTER_BOUND ( 'NONE', #62878, .T. ) ;
#130737=CARTESIAN_POINT ( 'NONE',  ( -6.622231685632140596, 6.690634819517756959, 0.000000000000000000 ) ) ;
#130743=CARTESIAN_POINT ( 'NONE',  ( -4.936577329151611515, 7.813071746435248599, 1.082531754730549967 ) ) ;
#130746=CARTESIAN_POINT ( 'NONE',  ( -6.771371375382467583, 6.864631124226471037, -0.7998128361456362523 ) ) ;
#130753=CARTESIAN_POINT ( 'NONE',  ( -5.777182852754558340, 5.912670547734647286, 0.000000000000000000 ) ) ;
#130766=CARTESIAN_POINT ( 'NONE',  ( -7.781453819600577582, 8.043060642480948985, 0.000000000000000000 ) ) ;
#130767=CARTESIAN_POINT ( 'NONE',  ( 5.422335090822693715, 5.290755458906732933, 0.000000000000000000 ) ) ;
#130768=CARTESIAN_POINT ( 'NONE',  ( -6.306477729012051725, 7.386587434382707151, 1.199719254218452047 ) ) ;
#130787=CARTESIAN_POINT ( 'NONE',  ( 3.147653791585804051, 8.919999999999937756, -2.420000000000002149 ) ) ;
#130792=CARTESIAN_POINT ( 'NONE',  ( -6.312203035614172286, 9.521931420595302953, -1.199719254218452047 ) ) ;
#130821=CARTESIAN_POINT ( 'NONE',  ( 5.408776937209000657, 5.274937613024121674, 0.7998128361456352531 ) ) ;
#130833=CARTESIAN_POINT ( 'NONE',  ( 4.812442952513422689, 8.115120723895499211, -0.8517184758452013282 ) ) ;
#130835=CARTESIAN_POINT ( 'NONE',  ( 3.444653546323793947, 6.176457016423196222, 1.199719254218451159 ) ) ;
#130840=CARTESIAN_POINT ( 'NONE',  ( -4.990283058281743678, 7.979691447040783814, -1.199719254218453823 ) ) ;
#130845=CARTESIAN_POINT ( 'NONE',  ( -7.715998819508785189, 8.174622508947939181, -0.7216878364870338292 ) ) ;
#130852=EDGE_CURVE ( 'NONE', #209619, #199345, #93395, .T. ) ;
#130853=CARTESIAN_POINT ( 'NONE',  ( -3.800028193580205382, 7.655393002477360653, -0.7998128361456481317 ) ) ;
#130862=CARTESIAN_POINT ( 'NONE',  ( 5.246079093845007257, 5.085123462432798114, 0.7998128361456352531 ) ) ;
#130884=ORIENTED_EDGE ( 'NONE', *, *, #153998, .T. ) ;
#130885=CARTESIAN_POINT ( 'NONE',  ( -5.589704470584107909, 9.743348658981940247, -0.7998128361456362523 ) ) ;
#130895=CARTESIAN_POINT ( 'NONE',  ( 4.016958651398847557, 7.908478536599129249, -0.7998128361456362523 ) ) ;
#130903=CARTESIAN_POINT ( 'NONE',  ( 3.282482588284323821, 6.843663763058119187, 0.7216878364870257245 ) ) ;
#130907=CARTESIAN_POINT ( 'NONE',  ( 5.546694241766559230, 9.485244025454063532, 0.000000000000000000 ) ) ;
#130917=CARTESIAN_POINT ( 'NONE',  ( -4.990809943606269172, 8.836712344267034780, -0.7216878364870338292 ) ) ;
#130942=CARTESIAN_POINT ( 'NONE',  ( 5.595604037360608629, 5.769690798462138837, 0.6831429992372698434 ) ) ;
#130955=CARTESIAN_POINT ( 'NONE',  ( 6.717138760927786834, 6.801359740696030443, -0.7998128361456481317 ) ) ;
#130957=CARTESIAN_POINT ( 'NONE',  ( 5.254667053748194760, 8.288139441751686931, 1.199719254218452047 ) ) ;
#130968=CARTESIAN_POINT ( 'NONE',  ( -4.146814880933400005, 5.931313009212638931, 1.599625672291270506 ) ) ;
#130971=CARTESIAN_POINT ( 'NONE',  ( 5.194182247366878613, 6.192872389083746043, 1.082531754730549078 ) ) ;
#130985=CARTESIAN_POINT ( 'NONE',  ( -6.211043768836215229, 8.339580045099285854, 1.443375672974064550 ) ) ;
#130987=CARTESIAN_POINT ( 'NONE',  ( -4.177320726786315497, 7.887641591310407208, -0.7216878364870458196 ) ) ;
#130991=CARTESIAN_POINT ( 'NONE',  ( -5.599738924909661186, 5.745725798494749625, 0.2540040342395213369 ) ) ;
#131004=CARTESIAN_POINT ( 'NONE',  ( -4.065465959251405081, 5.836405933916976707, -1.599625672291271394 ) ) ;
#131015=CARTESIAN_POINT ( 'NONE',  ( -5.815521545619021460, 5.749472989502435460, -0.7998128361456362523 ) ) ;
#131016=CARTESIAN_POINT ( 'NONE',  ( -5.608757509019071108, 5.629766575892905855, -0.3787719694710602325 ) ) ;
#131018=CARTESIAN_POINT ( 'NONE',  ( 5.320709023819174099, 7.653582423498873410, -1.267626751378515326 ) ) ;
#131022=DIRECTION ( 'NONE',  ( 0.6507913734559640506, -0.7592566023653003482, 0.000000000000000000 ) ) ;
#131025=CARTESIAN_POINT ( 'NONE',  ( -7.449279056065764237, 7.655523418356991350, 0.7998128361456341429 ) ) ;
#131026=CARTESIAN_POINT ( 'NONE',  ( -4.749858536263919184, 8.300932276130108534, 0.7929127856809523589 ) ) ;
#131031=CARTESIAN_POINT ( 'NONE',  ( -6.089020385868850305, 10.11795786024005572, -0.7216878364870338292 ) ) ;
#131046=CARTESIAN_POINT ( 'NONE',  ( 6.900173834712277632, 7.014900660111269559, -0.7998128361456341429 ) ) ;
#131071=CARTESIAN_POINT ( 'NONE',  ( 7.530627977747744062, 7.750430493652658015, -0.7998128361456341429 ) ) ;
#131072=CARTESIAN_POINT ( 'NONE',  ( 5.794130544993763898, 7.853181283949808744, 1.599625672291269396 ) ) ;
#131074=CARTESIAN_POINT ( 'NONE',  ( 3.054329744828568227, 6.785411478933790264, 0.000000000000000000 ) ) ;
#131085=CARTESIAN_POINT ( 'NONE',  ( 5.098657496608274720, 7.938328561423579011, 1.202842226815619142 ) ) ;
#131086=CARTESIAN_POINT ( 'NONE',  ( -4.299344108864949554, 8.030002203735486788, -0.7216878364870338292 ) ) ;
#131087=CARTESIAN_POINT ( 'NONE',  ( 5.885648082108200896, 6.039213315313952002, 0.7216878364870328300 ) ) ;
#131111=CARTESIAN_POINT ( 'NONE',  ( 4.342354338126830804, 8.288106837781779035, -0.7998128361456381397 ) ) ;
#131113=CARTESIAN_POINT ( 'NONE',  ( 4.869313445963426190, 5.709895770826003414, 1.199719254218452935 ) ) ;
#131130=FACE_OUTER_BOUND ( 'NONE', #42035, .T. ) ;
#131132=CARTESIAN_POINT ( 'NONE',  ( -6.688968683495758683, 8.897159112202094988, -1.599625672291271394 ) ) ;
#131142=CARTESIAN_POINT ( 'NONE',  ( 7.028976294042106332, 7.165170195996068969, 0.000000000000000000 ) ) ;
#131146=CARTESIAN_POINT ( 'NONE',  ( 5.417364897112183719, 8.477953592343014932, 1.199719254218451159 ) ) ;
#131156=CARTESIAN_POINT ( 'NONE',  ( 4.637820276784100137, 8.319831082953612622, -0.4078742439591088731 ) ) ;
#131165=EDGE_CURVE ( 'NONE', #41470, #133393, #56564, .T. ) ;
#131172=CARTESIAN_POINT ( 'NONE',  ( -6.158576598851958295, 6.984695343647041810, 0.9239717604232693393 ) ) ;
#131180=CARTESIAN_POINT ( 'NONE',  ( -7.605197822622922210, 7.837428646007010613, -0.7998128361456362523 ) ) ;
#131182=CARTESIAN_POINT ( 'NONE',  ( 4.929271367020211514, 7.908511140569038922, 1.199719254218452047 ) ) ;
#131185=DIRECTION ( 'NONE',  ( -1.000000000000000000, 0.000000000000000000, 0.000000000000000000 ) ) ;
#131187=CARTESIAN_POINT ( 'NONE',  ( -4.990809943606294929, 4.995235487061662205, -0.7216878364870338292 ) ) ;
#131195=CARTESIAN_POINT ( 'NONE',  ( -6.392190997713585787, 6.905894197498253284, -0.8087526810517248199 ) ) ;
#131211=CARTESIAN_POINT ( 'NONE',  ( 7.200788982633824276, 7.573544365927161515, 0.000000000000000000 ) ) ;
#131219=CARTESIAN_POINT ( 'NONE',  ( -3.231779075379149546, 6.036511184309971689, -0.9899555337401846344 ) ) ;
#131225=CARTESIAN_POINT ( 'NONE',  ( -5.980555157403903976, 6.149938236492225485, 0.000000000000000000 ) ) ;
#131227=CARTESIAN_POINT ( 'NONE',  ( 7.035755370848908896, 7.173079118937375931, 0.7998128361456352531 ) ) ;
#131231=CARTESIAN_POINT ( 'NONE',  ( -4.625266680917477835, 5.425174544939014964, -1.199719254218453823 ) ) ;
#131247=CARTESIAN_POINT ( 'NONE',  ( -5.817856928050925802, 5.960123635580414359, -1.359047942450207100E-08 ) ) ;
#131275=CARTESIAN_POINT ( 'NONE',  ( 3.203469434578891661, 6.959407783642502565, -0.7998128361456362523 ) ) ;
#131279=CARTESIAN_POINT ( 'NONE',  ( -1.807185592549641395, 2.518115318451403795, 2.500000000000000444 ) ) ;
#131281=CARTESIAN_POINT ( 'NONE',  ( -5.953438849732214599, 6.118302544208584770, 0.7216878364870257245 ) ) ;
#131288=CARTESIAN_POINT ( 'NONE',  ( -5.692444392891315097, 7.734547439830227411, -1.599625672291271394 ) ) ;
#131295=CARTESIAN_POINT ( 'NONE',  ( -5.607179047703544583, 8.699403434699558346, 1.199719254218454489 ) ) ;
#131297=CARTESIAN_POINT ( 'NONE',  ( 6.440439394220377700, 6.875545743132385645, 0.7017714770480776298 ) ) ;
#131302=CARTESIAN_POINT ( 'NONE',  ( 5.169401708560450004, 9.252995436621013425, 0.000000000000000000 ) ) ;
#131310=DIRECTION ( 'NONE',  ( 0.000000000000000000, 1.000000000000000000, 0.000000000000000000 ) ) ;
#131311=CARTESIAN_POINT ( 'NONE',  ( -3.305155586681401303, 7.078041627762083898, 0.7998128361456352531 ) ) ;
#131315=CARTESIAN_POINT ( 'NONE',  ( -4.938913097128142304, 8.984092056616635347, -0.7998128361456362523 ) ) ;
#131318=CARTESIAN_POINT ( 'NONE',  ( 6.821160681006788629, 8.091013894996997635, 1.082531754730549967 ) ) ;
#131320=CARTESIAN_POINT ( 'NONE',  ( -6.658462837642833421, 8.861568958707010779, 1.443375672974064550 ) ) ;
#131326=CARTESIAN_POINT ( 'NONE',  ( 5.071631979963703962, 8.074598522336444262, 1.199719254218451159 ) ) ;
#131329=CARTESIAN_POINT ( 'NONE',  ( -4.932336382548663245, 4.883384536077152838, 0.5336735327908896931 ) ) ;
#131334=CARTESIAN_POINT ( 'NONE',  ( -2.995508107964761191, 6.411541510041463887, -0.7147908198718248007 ) ) ;
#131365=CARTESIAN_POINT ( 'NONE',  ( -5.448385796200811981, 7.521903143423984694, -1.249286997217812223 ) ) ;
#131371=DIRECTION ( 'NONE',  ( 0.000000000000000000, 0.000000000000000000, 1.000000000000000000 ) ) ;
#131383=CARTESIAN_POINT ( 'NONE',  ( -3.318713740295064163, 7.093859473644694269, 0.000000000000000000 ) ) ;
#131387=CARTESIAN_POINT ( 'NONE',  ( 4.517335436343476118, 8.499999999999996447, -0.7749999999999996891 ) ) ;
#131393=ORIENTED_EDGE ( 'NONE', *, *, #76686, .T. ) ;
#131394=CARTESIAN_POINT ( 'NONE',  ( 5.337069745634900997, 6.255611453776062980, 1.199719254218452047 ) ) ;
#131395=CARTESIAN_POINT ( 'NONE',  ( 5.695833931072550094, 5.817763472438987726, 0.000000000000000000 ) ) ;
#131397=CARTESIAN_POINT ( 'NONE',  ( 6.821160681006793070, 7.130644680695653825, 0.7216878364870328300 ) ) ;
#131409=CARTESIAN_POINT ( 'NONE',  ( -6.123442655227560927, 7.173046514967467147, 1.199719254218452047 ) ) ;
#131410=CARTESIAN_POINT ( 'NONE',  ( 5.225741863424510747, 5.061396693608882558, 0.7998128361456352531 ) ) ;
#131419=CARTESIAN_POINT ( 'NONE',  ( -3.709037541790315640, 6.484905011134099340, -1.199719254218450271 ) ) ;
#131420=CARTESIAN_POINT ( 'NONE',  ( 5.508355548902068577, 9.648441583686274470, 0.7998128361456331437 ) ) ;
#131427=CARTESIAN_POINT ( 'NONE',  ( 5.578253857379852576, 5.472660686556754861, -0.7998128361456481317 ) ) ;
#131433=CARTESIAN_POINT ( 'NONE',  ( -6.612576056032890115, 6.759750829040511277, 0.1256891304984939506 ) ) ;
#131442=CARTESIAN_POINT ( 'NONE',  ( -6.933015448541747006, 9.181880338089085214, 1.599625672291269396 ) ) ;
#131456=CARTESIAN_POINT ( 'NONE',  ( -6.966220764712148572, 6.002124920821316323, 2.500000000000000444 ) ) ;
#131472=CARTESIAN_POINT ( 'NONE',  ( 5.061990249855835344, 6.999017606288843396, -1.599625672291273393 ) ) ;
#131482=EDGE_LOOP ( 'NONE', ( #183159, #90407, #13348, #72169 ) ) ;
#131491=CARTESIAN_POINT ( 'NONE',  ( 6.536439455564150514, 9.679577560583279450, 1.082531754730549078 ) ) ;
#131492=CARTESIAN_POINT ( 'NONE',  ( -5.316205630334276400, 5.374863788244313767, -0.7216878364870338292 ) ) ;
#131506=DIRECTION ( 'NONE',  ( 0.000000000000000000, 0.000000000000000000, 1.000000000000000000 ) ) ;
#131519=CARTESIAN_POINT ( 'NONE',  ( -4.685224601974262271, 7.623789914682047808, -1.199719254218453823 ) ) ;
#131521=CARTESIAN_POINT ( 'NONE',  ( 7.471952054462756010, 7.889901283060952508, 0.7216878364870267237 ) ) ;
#131526=CARTESIAN_POINT ( 'NONE',  ( -6.805266759416629618, 6.904175738932996964, 0.000000000000000000 ) ) ;
#131532=( BOUNDED_SURFACE ( )  B_SPLINE_SURFACE ( 3, 2, ( 
 ( #188008, #137153, #203178 ),
 ( #54825, #120975, #38576 ),
 ( #138222, #170698, #204235 ),
 ( #122044, #39635, #212521 ),
 ( #79340, #209309, #205320 ),
 ( #62033, #81474, #47939 ) ),
 .UNSPECIFIED., .F., .F., .F. ) 
 B_SPLINE_SURFACE_WITH_KNOTS ( ( 4, 2, 4 ),
 ( 3, 3 ),
 ( 6.938893903907228378E-18, 0.002403677751102634413, 0.004807355502205261887 ),
 ( 0.000000000000000000, 1.000000000000000000 ),
 .UNSPECIFIED. ) 
 GEOMETRIC_REPRESENTATION_ITEM ( )  RATIONAL_B_SPLINE_SURFACE ( (
 ( 1.000000000000000000, 0.7789607113619931855, 1.000000000000000000),
 ( 1.000000000000000000, 0.7844575505954987094, 1.000000000000000000),
 ( 1.000000000000000000, 0.7910273759756240031, 1.000000000000000000),
 ( 1.000000000000000000, 0.8087931444444612650, 1.000000000000000000),
 ( 1.000000000000000000, 0.8199986536752662536, 1.000000000000000000),
 ( 1.000000000000000000, 0.8356624583022091990, 1.000000000000000000) ) ) 
 REPRESENTATION_ITEM ( '' )  SURFACE ( )  );
#131535=CARTESIAN_POINT ( 'NONE',  ( -5.237192476628793614, 9.332084666034067055, 0.7998128361456291469 ) ) ;
#131548=CARTESIAN_POINT ( 'NONE',  ( -4.447956913735107598, 7.346977611736363656, 1.199719254218452935 ) ) ;
#131551=CARTESIAN_POINT ( 'NONE',  ( -5.777182853198894463, 9.754147405458438058, 0.7216878364870267237 ) ) ;
#131553=CARTESIAN_POINT ( 'NONE',  ( -6.739811759324828344, 8.956476034002674780, -1.443375672974066548 ) ) ;
#131554=CARTESIAN_POINT ( 'NONE',  ( 6.393551957296131683, 9.616838495890963401, 1.199719254218452047 ) ) ;
#131556=CARTESIAN_POINT ( 'NONE',  ( -5.126391479298592735, 5.153413945369351268, 0.000000000000000000 ) ) ;
#131572=CARTESIAN_POINT ( 'NONE',  ( 0.3373309291320715220, 2.648944349799879472, 1.974167966546634956 ) ) ;
#131576=CARTESIAN_POINT ( 'NONE',  ( -1.878807924852155864, 2.480000000000016858, -2.465802685833468288 ) ) ;
#131577=CARTESIAN_POINT ( 'NONE',  ( 6.296370465541430761, 6.973533528358998979, 0.9269300130883666444 ) ) ;
#131589=ADVANCED_FACE ( 'NONE', ( #19278 ), #74741, .T. ) ;
#131596=CARTESIAN_POINT ( 'NONE',  ( 5.535985025370705692, 7.434063834270491000, -1.247683609459742549 ) ) ;
#131607=DIRECTION ( 'NONE',  ( 0.000000000000000000, 0.000000000000000000, -1.000000000000000000 ) ) ;
#131609=EDGE_CURVE ( 'NONE', #179029, #137516, #155083, .T. ) ;
#131610=B_SPLINE_SURFACE_WITH_KNOTS ( 'NONE', 1, 3, ( 
 ( #188870, #24218, #140157, #144446, #164646, #78322, #45854, #198190, #66037, #49825, #126095, #50893, #16229, #109836, #44789, #114888, #1042, #210449, #214406, #175847, #17298, #166779, #28515, #12247, #117018, #176901, #62087, #192057, #99642, #128245, #82313, #208310, #160647, #115950, #133241, #83376, #180887, #127171, #132184, #183015, #98584, #194209, #193141, #181940, #33570, #32509, #110895, #165709, #94606, #77255, #148407, #149459, #199246, #67105, #34632, #100703, #61013, #43721, #18375, #142300, #59941, #27438, #93536, #159580, #11177, #143370, #209368, #2104, #200316, #167839, #68178, #150540, #134309, #51967, #35695, #101771, #84452, #118091, #184076, #207213, #194167, #140115, #12210, #144409, #127128, #128206, #141202, #43680, #210409, #42615, #108725, #60972, #161692, #189901, #76153, #109799, #44747, #77213, #157423, #75090, #62051, #111934, #159538, #58837, #25262, #208269, #94565, #45814, #173686, #93498, #78281, #177936, #28473, #193098, #192017, #175806, #29549, #142257, #10077, #107657, #143332, #124992, #95641, #190951, #209325, #91363, #74025, #160608, #110853, #176861, #41543, #59902, #11136, #126055, #27398, #206141, #57772, #123933, #9014, #174751, #26324, #92438, #158477, #197360, #83610, #15400, #82542, #195247, #99874, #34849, #114072, #97763, #199478, #47957, #147568, #63106, #182165, #213589, #98816, #79359, #31687, #132413, #1274, #165937, #131365, #212542, #196, #51122, #181117, #65214, #64182, #50059, #198415, #49003, #130323, #116180, #196313, #162760, #180064, #33796, #67332, #16462, #149691, #163822, #146523, #211472, #17522, #100924, #13286, #66265, #81491, #115121, #32736, #164868, #129274, #14334, #148630, #145477, #133476, #46883, #112995, #80424, #117245, #183245, #179008, #30622, #96711, #85750, #72688, #18604, #105220, #2333, #122614, #19671, #151832, #22854, #150771, #3405 ),
 ( #69474, #200542, #134536, #135581, #121538, #39137, #155023, #84684, #202674, #201603, #138783, #68409, #171260, #88968, #53251, #204803, #20723, #86817, #152883, #36991, #6607, #167012, #4461, #103074, #168071, #70531, #56454, #102002, #118314, #5525, #136649, #54322, #52188, #119382, #188577, #169129, #35925, #55383, #40209, #185368, #184300, #120463, #21776, #186435, #38073, #104143, #170190, #87885, #153959, #71606, #137717, #203737, #187508, #179718, #47600, #110510, #161333, #62743, #212183, #81140, #147225, #61690, #31335, #96349, #97412, #146168, #112643, #93148, #176510, #127859, #194884, #144056, #159185, #163467, #45458, #192734, #160256, #145113, #63820, #193809, #95285, #10786, #15047, #44389, #129978, #76861, #111574, #213250, #43330, #11857, #80066, #64880, #177582, #77935, #142980, #131026, #109448, #208980, #175455, #210051, #27039, #12917, #60617, #126776, #28122, #94216, #162404, #29196, #78997, #211119, #13982, #46521, #128903, #178652, #30263, #195965, #113714, #49704, #166661, #52901, #165588, #17181, #183964, #70193, #98460, #199125, #18251, #167723, #200198, #65919, #198077, #119035, #20390, #68051, #115833, #148287, #116898, #3056, #185018, #82193, #1988, #201261, #36644, #151487, #35575, #100587, #84335, #102728, #50769, #133127, #16109, #51851, #181819, #168785, #33451, #86474, #152538, #99528, #150423, #134189, #69126, #4124, #197017, #920, #48653, #101655, #114770, #85401, #117971, #32394, #83256, #66988, #19324, #149341, #164524, #180766, #182898, #132066, #34514, #135248, #214286, #72335, #188228, #186093, #42019, #71262, #24657, #37723, #154679, #91837, #136305, #104874, #173076, #25727, #6264, #170917, #21439, #9488, #157895, #103802, #202327, #88624, #174155, #39868, #169851, #87547, #137376, #53977, #189304, #153615, #138441, #120113, #107050, #139514, #5187, #203392, #55045, #121195 ) ),
 .UNSPECIFIED., .F., .T., .F.,
 ( 2, 2 ),
 ( 4, 2, 2, 2, 2, 2, 2, 2, 2, 2, 2, 2, 2, 2, 2, 2, 2, 2, 2, 2, 2, 2, 2, 2, 2, 2, 2, 2, 2, 2, 2, 2, 2, 2, 2, 2, 2, 2, 2, 2, 2, 2, 2, 2, 2, 2, 2, 2, 2, 2, 2, 2, 2, 2, 2, 2, 2, 2, 2, 2, 2, 2, 2, 2, 2, 2, 2, 2, 2, 2, 2, 2, 2, 2, 2, 2, 2, 2, 2, 2, 2, 2, 2, 2, 2, 2, 2, 2, 2, 2, 2, 2, 2, 2, 2, 2, 2, 2, 2, 2, 2, 2, 2, 2, 2, 2, 2, 2, 4 ),
 ( 0.000000000000000000, 1.000000000000000000 ),
 ( -5.017377349295429334E-06, 6.045441312669188748E-05, 0.0001259262036026792043, 0.0002568697845546538379, 0.0003878133655066284716, 0.0004205492607446221706, 0.0004532851559826158155, 0.0005187569464586031052, 0.0005842287369345903949, 0.0006497005274105776846, 0.0007806441083625523724, 0.0008461158988385397706, 0.0009115876893145270603, 0.0009770594797905143500, 0.001042531270266501640, 0.001173474851218476219, 0.001238946641694463509, 0.001304418432170450799, 0.001369890222646438088, 0.001435362013122425378, 0.001500833803598412668, 0.001566305594074400174, 0.001631777384550387681, 0.001697249175026374970, 0.001762720965502362260, 0.001828192755978349550, 0.001893664546454336840, 0.001959136336930324129, 0.002090079917882298709, 0.002155551708358285998, 0.002221023498834273288, 0.002286495289310260578, 0.002351967079786247868, 0.002482910660738222447, 0.002548382451214209737, 0.002613854241690197026, 0.002679326032166184316, 0.002744797822642171606, 0.002810269613118158896, 0.002875741403594146185, 0.003006684984546120765, 0.003072156775022108488, 0.003137628565498095778, 0.003203100355974083067, 0.003268572146450070791, 0.003399515727402045370, 0.003530459308354019950, 0.003563195203592013811, 0.003595931098830007239, 0.003661402889305994529, 0.003726874679781981819, 0.003792346470257969109, 0.003923290051209943688, 0.003988761841685931411, 0.004054233632161918267, 0.004119705422637905123, 0.004185177213113892847, 0.004250649003589880570, 0.004316120794065867426, 0.004381592584541854282, 0.004447064375017842006, 0.004578007955969816585, 0.004643479746445803441, 0.004708951536921791164, 0.004774423327397778888, 0.004839895117873765744, 0.004970838698825740323, 0.005101782279777714903, 0.005232725860729689482, 0.005363669441681664062, 0.005494613022633638641, 0.005625556603585613220, 0.005691028394061600076, 0.005756500184537587800, 0.005821971975013575523, 0.005887443765489562379, 0.006018387346441536959, 0.006083859136917524682, 0.006149330927393512405, 0.006214802717869500129, 0.006280274508345486985, 0.006411218089297461564, 0.006476689879773449288, 0.006542161670249437011, 0.006607633460725424734, 0.006673105251201411590, 0.006738577041677398446, 0.006804048832153386170, 0.006869520622629373893, 0.006934992413105360749, 0.007000464203581347605, 0.007065935994057335329, 0.007131407784533323052, 0.007196879575009309908, 0.007327823155961284488, 0.007393294946437272211, 0.007458766736913259067, 0.007491502632151252061, 0.007524238527389245923, 0.007589710317865233646, 0.007720653898817208226, 0.007786125689293195082, 0.007851597479769182805, 0.007917069270245168794, 0.007982541060721156517, 0.008113484641673131964, 0.008244428222625107411, 0.008309900013101095134, 0.008375371803577081123 ),
 .UNSPECIFIED. ) ;
#131611=CARTESIAN_POINT ( 'NONE',  ( 5.691390622686558487, 9.861982503101517139, 0.7998128361456341429 ) ) ;
#131614=CARTESIAN_POINT ( 'NONE',  ( -6.303615075710993665, 6.318915441276411471, -0.7998128361456362523 ) ) ;
#131628=CARTESIAN_POINT ( 'NONE',  ( 4.441177836928239309, 7.339068688795062911, 1.199719254218452047 ) ) ;
#131630=CARTESIAN_POINT ( 'NONE',  ( 7.018280793729500644, 8.217024343219755167, -1.199719254218452047 ) ) ;
#131635=CARTESIAN_POINT ( 'NONE',  ( -5.872089928050201024, 8.904503111816948646, 1.082531754730550855 ) ) ;
#131642=CARTESIAN_POINT ( 'NONE',  ( 6.502017186205484300, 9.743381262951846367, -1.199719254218452047 ) ) ;
#131647=CARTESIAN_POINT ( 'NONE',  ( 1.843739406749204335, 8.928444911142053186, 0.7750000000000004663 ) ) ;
#131651=DIRECTION ( 'NONE',  ( 1.000000000000000000, 0.000000000000000000, 0.000000000000000000 ) ) ;
#131654=CARTESIAN_POINT ( 'NONE',  ( -6.129694847154222970, 7.284303755502281597, -1.082531754730549967 ) ) ;
#131655=CARTESIAN_POINT ( 'NONE',  ( 5.316205630334249754, 7.295602216847000498, -1.443375672974078761 ) ) ;
#131666=CARTESIAN_POINT ( 'NONE',  ( -6.943184063974186415, 7.273005294157565359, -0.7216878364870338292 ) ) ;
#131667=CARTESIAN_POINT ( 'NONE',  ( 1.841070778277279718, 2.501489970915801830, -2.494084679671781046 ) ) ;
#131671=CARTESIAN_POINT ( 'NONE',  ( 4.163762572728282763, 6.911454530608037494, -1.082531754730548412 ) ) ;
#131689=CARTESIAN_POINT ( 'NONE',  ( -5.004894982100124068, 5.868074229652107121, 1.199719254218452935 ) ) ;
#131700=CARTESIAN_POINT ( 'NONE',  ( 3.607351389687783794, 6.366271167014519783, 1.199719254218451159 ) ) ;
#131703=CARTESIAN_POINT ( 'NONE',  ( 4.857564175446106525, 8.889184981320973122, 0.7998128361456331437 ) ) ;
#131712=CARTESIAN_POINT ( 'NONE',  ( -4.599959256786493533, 8.588645909551377855, 0.000000000000000000 ) ) ;
#131715=DIRECTION ( 'NONE',  ( 0.7592566023652995710, -0.6507913734559650498, 0.000000000000000000 ) ) ;
#131734=EDGE_CURVE ( 'NONE', #157380, #196200, #177578, .T. ) ;
#131739=CARTESIAN_POINT ( 'NONE',  ( 5.234856708652235291, 5.279956712948652431, 0.7216878364870338292 ) ) ;
#131740=ORIENTED_EDGE ( 'NONE', *, *, #161304, .T. ) ;
#131745=CARTESIAN_POINT ( 'NONE',  ( 4.380693030546905398, 8.124909279031149012, 0.7216878364870247253 ) ) ;
#131757=CARTESIAN_POINT ( 'NONE',  ( -5.956828388357799042, 8.042995434541133193, 1.599625672291263179 ) ) ;
#131759=CARTESIAN_POINT ( 'NONE',  ( -5.427006627220116286, 9.553534508390610469, -0.7998128361456362523 ) ) ;
#131767=CARTESIAN_POINT ( 'NONE',  ( 5.854088466050551887, 10.05179665369283981, 0.7998128361456341429 ) ) ;
#131774=CARTESIAN_POINT ( 'NONE',  ( -7.286581212701773502, 7.465709267765667789, 0.7998128361456341429 ) ) ;
#131780=CARTESIAN_POINT ( 'NONE',  ( -6.129694847154222970, 7.284303755502281597, -1.082531754730549967 ) ) ;
#131783=CARTESIAN_POINT ( 'NONE',  ( -6.784929528996132220, 6.880448970109080520, 0.000000000000000000 ) ) ;
#131799=CARTESIAN_POINT ( 'NONE',  ( -6.599398278744054380, 6.760864547338558239, 0.4146307598744238820 ) ) ;
#131802=CARTESIAN_POINT ( 'NONE',  ( -5.343321937561608337, 5.406499480009534508, 0.7216878364870257245 ) ) ;
#131804=CARTESIAN_POINT ( 'NONE',  ( -4.624739795592948788, 5.528522862014106920, -1.082531754730549967 ) ) ;
#131805=CARTESIAN_POINT ( 'NONE',  ( 5.273195401072370281, 5.116759154198018855, -0.7998128361456481317 ) ) ;
#131807=CARTESIAN_POINT ( 'NONE',  ( -5.926849427829407269, 6.943687749669614995, -1.199719254218453823 ) ) ;
#131822=CARTESIAN_POINT ( 'NONE',  ( -5.514013019825418915, 5.994650414344389056, -0.9619886414689113874 ) ) ;
#131826=CARTESIAN_POINT ( 'NONE',  ( -6.343551558972118976, 6.506286488053500072, -2.500000000000000000 ) ) ;
#131846=EDGE_CURVE ( 'NONE', #155820, #97415, #96913, .T. ) ;
#131857=CARTESIAN_POINT ( 'NONE',  ( 3.410758162289653672, 6.136912401716668519, -1.199719254218453823 ) ) ;
#131870=CARTESIAN_POINT ( 'NONE',  ( 4.789099507923308963, 8.141322699134850183, 0.8117711051834965996 ) ) ;
#131872=CARTESIAN_POINT ( 'NONE',  ( 5.239300017038202917, 5.077214539491492928, 0.000000000000000000 ) ) ;
#131878=CARTESIAN_POINT ( 'NONE',  ( -7.123883369337781879, 7.275895117174344229, 0.7998128361456341429 ) ) ;
#131883=CIRCLE ( 'NONE', #52380, 0.08000000000000020983 ) ;
#131884=CARTESIAN_POINT ( 'NONE',  ( -7.390603132780795725, 8.755363422066633206, -1.082531754730549967 ) ) ;
#131888=CARTESIAN_POINT ( 'NONE',  ( -4.446850669412495627, 7.248452911037940538, 1.092318573022862616 ) ) ;
#131893=CARTESIAN_POINT ( 'NONE',  ( -3.461074353238556167, 7.259946855412102273, 0.000000000000000000 ) ) ;
#131904=CARTESIAN_POINT ( 'NONE',  ( 3.627688620108284745, 6.389997935838436227, 1.199719254218452047 ) ) ;
#131928=CARTESIAN_POINT ( 'NONE',  ( 7.856023664475727308, 8.130058794835305136, -0.7998128361456341429 ) ) ;
#131935=CARTESIAN_POINT ( 'NONE',  ( 7.042534447655770080, 7.180988041878682004, -0.7998128361456341429 ) ) ;
#131942=CARTESIAN_POINT ( 'NONE',  ( 4.095971805104285934, 6.832365301713403838, 1.082531754730549078 ) ) ;
#131945=CARTESIAN_POINT ( 'NONE',  ( 6.048345925472178308, 9.110135108809304327, 1.082531754730549967 ) ) ;
#131956=CARTESIAN_POINT ( 'NONE',  ( -4.963693636378939011, 8.805076652501815815, 0.7216878364870267237 ) ) ;
#131976=AXIS2_PLACEMENT_3D ( 'NONE', #162797, #129313, #180103 ) ;
#131991=VERTEX_POINT ( 'NONE', #4916 ) ;
#131995=CARTESIAN_POINT ( 'NONE',  ( 5.123001941117305336, 7.070197912760590064, 1.599625672291268286 ) ) ;
#131997=CARTESIAN_POINT ( 'NONE',  ( 6.333594036239346359, 7.418223126147930557, 1.199719254218453823 ) ) ;
#132002=DIRECTION ( 'NONE',  ( 0.000000000000000000, 0.000000000000000000, 1.000000000000000000 ) ) ;
#132004=DIRECTION ( 'NONE',  ( 0.3321398189114310173, 0.9432301631592798774, 0.000000000000000000 ) ) ;
#132009=CARTESIAN_POINT ( 'NONE',  ( -7.756673280794142755, 8.222076047114187602, -0.7216878364870338292 ) ) ;
#132012=CARTESIAN_POINT ( 'NONE',  ( 4.543390873910903238, 7.354354215321133204, 1.082531754730548412 ) ) ;
#132014=B_SPLINE_CURVE_WITH_KNOTS ( 'NONE', 3,
 ( #111564, #191656, #25968, #178643, #175446, #93139, #76851, #94206, #110501, #28112 ),
 .UNSPECIFIED., .F., .F.,
 ( 4, 3, 3, 4 ),
 ( 5.442583568837955947E-16, 3.125183826620649906E-05, 6.400261867760048467E-05, 9.676915533390859927E-05 ),
 .UNSPECIFIED. ) ;
#132026=CARTESIAN_POINT ( 'NONE',  ( -5.804299160426229953, 8.825413882922319431, -1.082531754730549967 ) ) ;
#132028=CARTESIAN_POINT ( 'NONE',  ( -5.478903473698260029, 6.525047153136981137, -1.082531754730549967 ) ) ;
#132054=CARTESIAN_POINT ( 'NONE',  ( -4.305596300791617814, 7.180890229968955651, 1.199719254218452935 ) ) ;
#132065=CARTESIAN_POINT ( 'NONE',  ( 1.813555757143400893, 2.470689410283006371, -2.499999999999999556 ) ) ;
#132066=CARTESIAN_POINT ( 'NONE',  ( -5.830795741961422252, 7.309361553235873998, -1.292907557591252088 ) ) ;
#132084=CARTESIAN_POINT ( 'NONE',  ( 6.886615681098613884, 6.999082814228660077, 0.000000000000000000 ) ) ;
#132091=CARTESIAN_POINT ( 'NONE',  ( -5.458264003855187951, 7.602368174425948588, -1.382272695577278387 ) ) ;
#132097=EDGE_CURVE ( 'NONE', #182295, #157478, #98018, .T. ) ;
#132105=ADVANCED_FACE ( 'NONE', ( #190100, #88351 ), #101390, .T. ) ;
#132108=CARTESIAN_POINT ( 'NONE',  ( 6.261886844665240481, 8.398896966899865646, 1.599625672291268286 ) ) ;
#132109=CARTESIAN_POINT ( 'NONE',  ( 6.900173834712277632, 7.014900660111269559, -0.7998128361456341429 ) ) ;
#132111=CARTESIAN_POINT ( 'NONE',  ( 4.095444919779759552, 6.935713618788495793, 1.199719254218451159 ) ) ;
#132121=CARTESIAN_POINT ( 'NONE',  ( 4.890561790263044273, 8.149264200713410844, -1.004099907704804950 ) ) ;
#132122=CARTESIAN_POINT ( 'NONE',  ( -6.577113915960849155, 6.845923454808663600, -0.7216878364870338292 ) ) ;
#132123=CARTESIAN_POINT ( 'NONE',  ( 5.424670859243587273, 5.501406555305196733, -0.7216878364870458196 ) ) ;
#132150=CARTESIAN_POINT ( 'NONE',  ( 5.123001941117305336, 7.070197912760590064, 1.599625672291268286 ) ) ;
#132152=CARTESIAN_POINT ( 'NONE',  ( 5.598591087800349086, 5.496387455380669529, -0.7998128361456481317 ) ) ;
#132180=CARTESIAN_POINT ( 'NONE',  ( 5.071631979963703962, 8.074598522336444262, 1.199719254218451159 ) ) ;
#132184=CARTESIAN_POINT ( 'NONE',  ( -6.108552962726611746, 7.019250575032890183, 0.9758408306729206005 ) ) ;
#132185=CARTESIAN_POINT ( 'NONE',  ( 6.496291879603339758, 7.608037276739255006, 1.199719254218452935 ) ) ;
#132192=CARTESIAN_POINT ( 'NONE',  ( -1.872868072690844432, 8.979822391611987698, 0.7750000000000013545 ) ) ;
#132194=CARTESIAN_POINT ( 'NONE',  ( 4.594747986498664005, 8.374059380672374431, -0.03693212167796278145 ) ) ;
#132214=CARTESIAN_POINT ( 'NONE',  ( -5.433785704026946384, 9.561443431331920095, 0.000000000000000000 ) ) ;
#132216=CARTESIAN_POINT ( 'NONE',  ( 4.389807875774629942, 8.343469298370917997, 0.7998128361456271485 ) ) ;
#132217=CARTESIAN_POINT ( 'NONE',  ( -6.966220764712148572, 6.002124920821316323, 2.500000000000000444 ) ) ;
#132219=CARTESIAN_POINT ( 'NONE',  ( -4.855228407469635243, 4.837057028235559386, 0.7216878364870257245 ) ) ;
#132225=CARTESIAN_POINT ( 'NONE',  ( 3.719872605471085336, 6.605953636083950364, 2.420000000000000373 ) ) ;
#132241=CARTESIAN_POINT ( 'NONE',  ( 0.000000000000000000, 8.999999999999998224, 0.000000000000000000 ) ) ;
#132246=CARTESIAN_POINT ( 'NONE',  ( 5.343321937561575474, 8.287607122913563273, -1.082531754730548412 ) ) ;
#132259=CARTESIAN_POINT ( 'NONE',  ( -5.478903473698268023, 5.564677938835638216, -0.7216878364870338292 ) ) ;
#132261=CARTESIAN_POINT ( 'NONE',  ( 6.723917837734620484, 6.809268663637336516, 0.000000000000000000 ) ) ;
#132266=CARTESIAN_POINT ( 'NONE',  ( -7.533490631048818109, 8.818102486758951031, -1.199719254218452047 ) ) ;
#132279=DIRECTION ( 'NONE',  ( -1.000000000000000000, 0.000000000000000000, 0.000000000000000000 ) ) ;
#132307=CARTESIAN_POINT ( 'NONE',  ( 4.312902262922978736, 5.164712407232485702, -1.082531754730548412 ) ) ;
#132314=CARTESIAN_POINT ( 'NONE',  ( 3.555981428534177091, 7.370671776590375757, 0.7998128361456271485 ) ) ;
#132319=CARTESIAN_POINT ( 'NONE',  ( -6.916067756302494374, 7.241369601873926420, 0.000000000000000000 ) ) ;
#132325=CARTESIAN_POINT ( 'NONE',  ( -5.101610940492132151, 9.173906207207963348, -0.7998128361456362523 ) ) ;
#132332=PLANE ( 'NONE',  #136264 ) ;
#132333=CARTESIAN_POINT ( 'NONE',  ( 8.167861197590044142, 8.493869250135347215, 0.000000000000000000 ) ) ;
#132334=CARTESIAN_POINT ( 'NONE',  ( -6.479871072688648148, 6.524547437750345402, 0.000000000000000000 ) ) ;
#132337=CARTESIAN_POINT ( 'NONE',  ( 5.371503168974233411, 7.687194297833679357, 1.321221623412481394 ) ) ;
#132342=CARTESIAN_POINT ( 'NONE',  ( 6.373214726875630731, 9.593111727067046957, 1.199719254218452047 ) ) ;
#132349=CARTESIAN_POINT ( 'NONE',  ( -4.359828915246279024, 7.244161613499399799, -1.199719254218455378 ) ) ;
#132356=CARTESIAN_POINT ( 'NONE',  ( -5.074494633264801990, 9.142270515442742607, 0.7998128361456291469 ) ) ;
#132359=CARTESIAN_POINT ( 'NONE',  ( 4.977251789548238214, 7.860525283564661514, -1.082531754730548412 ) ) ;
#132361=CARTESIAN_POINT ( 'NONE',  ( 7.160114521348466710, 7.526090827760914870, 0.000000000000000000 ) ) ;
#132363=CARTESIAN_POINT ( 'NONE',  ( -5.736508391913536897, 9.706693867292189637, 0.7216878364870267237 ) ) ;
#132369=CARTESIAN_POINT ( 'NONE',  ( 6.530187263637528439, 7.647581891445782709, -1.199719254218452047 ) ) ;
#132385=CARTESIAN_POINT ( 'NONE',  ( 5.696489930276292135, 7.416392257432566026, -1.320530921439456273 ) ) ;
#132400=CARTESIAN_POINT ( 'NONE',  ( 4.768187943840554333, 8.164982483533503199, -0.7738548252242994918 ) ) ;
#132413=CARTESIAN_POINT ( 'NONE',  ( -5.355672060655169098, 7.601107163255693244, -1.239215230201977436 ) ) ;
#132432=CARTESIAN_POINT ( 'NONE',  ( -4.359828915246279024, 7.244161613499399799, -1.199719254218455378 ) ) ;
#132434=CARTESIAN_POINT ( 'NONE',  ( 7.526711554241970248, 8.810193563817646734, -1.199719254218452047 ) ) ;
#132449=CARTESIAN_POINT ( 'NONE',  ( 6.540882763950133238, 6.595727744222092959, 0.000000000000000000 ) ) ;
#132452=CARTESIAN_POINT ( 'NONE',  ( 6.089020385868848528, 8.197219431637373432, -1.443375672974078761 ) ) ;
#132463=CARTESIAN_POINT ( 'NONE',  ( -5.448397627845328550, 7.449826213943242514, 1.599625672291263179 ) ) ;
#132464=CARTESIAN_POINT ( 'NONE',  ( 4.716257332707354699, 6.595662536282280719, -1.599625672291269396 ) ) ;
#132473=CARTESIAN_POINT ( 'NONE',  ( -7.075376061485238566, 9.347967719856493218, 1.599625672291269396 ) ) ;
#132474=CARTESIAN_POINT ( 'NONE',  ( 7.666209513884374438, 7.908608952478760834, 0.7998128361456281477 ) ) ;
#132476=CARTESIAN_POINT ( 'NONE',  ( 4.726684935852882852, 4.891486930089099516, -0.8194250277325196841 ) ) ;
#132481=CARTESIAN_POINT ( 'NONE',  ( 4.309512724297349884, 6.121127159803966933, 1.599625672291261402 ) ) ;
#132482=CIRCLE ( 'NONE', #11360, 0.08000000000000025147 ) ;
#132487=CARTESIAN_POINT ( 'NONE',  ( -6.126043159632901691, 7.090966632250176538, 1.117993467579528222 ) ) ;
#132497=CARTESIAN_POINT ( 'NONE',  ( -7.608060475923978494, 8.905100639113307182, 1.199719254218452047 ) ) ;
#132547=FACE_OUTER_BOUND ( 'NONE', #99508, .T. ) ;
#132548=CARTESIAN_POINT ( 'NONE',  ( 3.528865121306874464, 7.339036084825155015, -0.7998128361456362523 ) ) ;
#132549=CARTESIAN_POINT ( 'NONE',  ( -3.797692425603673705, 6.484372692295976570, 1.082531754730549967 ) ) ;
#132572=CARTESIAN_POINT ( 'NONE',  ( -4.769436176957319695, 8.786368983084006601, 0.7998128361456281477 ) ) ;
#132573=CARTESIAN_POINT ( 'NONE',  ( 6.116136693096175136, 9.189224337703940648, -1.082531754730548412 ) ) ;
#132578=CARTESIAN_POINT ( 'NONE',  ( -7.456058132872594335, 7.663432341298296535, 0.000000000000000000 ) ) ;
#132579=CARTESIAN_POINT ( 'NONE',  ( -3.363304624641834106, 6.081549941127532222, -1.199719254218452047 ) ) ;
#132587=CARTESIAN_POINT ( 'NONE',  ( -6.557303570864871034, 7.679217583210999010, -1.199719254218452047 ) ) ;
#132594=CARTESIAN_POINT ( 'NONE',  ( 3.984117037569365305, 5.741498858621315371, 1.599625672291261402 ) ) ;
#132598=CARTESIAN_POINT ( 'NONE',  ( -6.622231685632140596, 6.690634819517756959, 0.000000000000000000 ) ) ;
#132601=CARTESIAN_POINT ( 'NONE',  ( -7.444835747679825033, 7.858265591814152629, 0.000000000000000000 ) ) ;
#132603=CARTESIAN_POINT ( 'NONE',  ( -6.577113915960841162, 7.806292669110006521, -1.082531754730549967 ) ) ;
#132604=CARTESIAN_POINT ( 'NONE',  ( 7.849244587668864348, 8.122149871893999062, 0.7998128361456291469 ) ) ;
#132605=CARTESIAN_POINT ( 'NONE',  ( -3.146901051703345331, 6.685485303713597283, 0.000000000000000000 ) ) ;
#132624=CARTESIAN_POINT ( 'NONE',  ( 6.589288424369031283, 6.777081280454712697, 0.2339771526987007022 ) ) ;
#132643=CARTESIAN_POINT ( 'NONE',  ( 5.772745519453025054, 7.247817053759448847, -1.191736586928717978 ) ) ;
#132650=EDGE_CURVE ( 'NONE', #141262, #79190, #191150, .T. ) ;
#132659=CARTESIAN_POINT ( 'NONE',  ( 6.016786309414542622, 10.24161080428416426, 0.7998128361456341429 ) ) ;
#132662=CARTESIAN_POINT ( 'NONE',  ( -6.005335696210345020, 5.970922831858983315, 0.7998128361456281477 ) ) ;
#132676=CARTESIAN_POINT ( 'NONE',  ( 4.492547798081839794, 6.334668079219206049, 1.599625672291262513 ) ) ;
#132678=CARTESIAN_POINT ( 'NONE',  ( 5.820193082016415609, 10.01225203898631655, 0.000000000000000000 ) ) ;
#132682=CARTESIAN_POINT ( 'NONE',  ( -7.227905289416804102, 8.565549271475310533, -1.082531754730549967 ) ) ;
#132689=CARTESIAN_POINT ( 'NONE',  ( 6.339319342841494453, 9.553567112360518365, -1.199719254218452047 ) ) ;
#132691=ORIENTED_EDGE ( 'NONE', *, *, #16190, .F. ) ;
#132695=CARTESIAN_POINT ( 'NONE',  ( 1.879585681373342698, 8.984805382992709255, 0.7750000000000004663 ) ) ;
#132703=CARTESIAN_POINT ( 'NONE',  ( -4.651856103264620401, 8.441266197201775512, 0.000000000000000000 ) ) ;
#132704=CARTESIAN_POINT ( 'NONE',  ( 5.912764389335563919, 6.070849007079172743, -0.7216878364870458196 ) ) ;
#132710=DIRECTION ( 'NONE',  ( 0.000000000000000000, -1.000000000000000000, 0.000000000000000000 ) ) ;
#132714=CARTESIAN_POINT ( 'NONE',  ( -5.334207092333882017, 5.187939460669764635, 0.7998128361456281477 ) ) ;
#132715=CARTESIAN_POINT ( 'NONE',  ( -6.780486220610184134, 9.003929572168926754, -1.443375672974066548 ) ) ;
#132719=CARTESIAN_POINT ( 'NONE',  ( 5.275531169048895741, 7.248148678680751189, -1.443375672974078761 ) ) ;
#132735=CARTESIAN_POINT ( 'NONE',  ( 4.923019175537949543, 4.916146257648610352, 0.000000000000000000 ) ) ;
#132739=CARTESIAN_POINT ( 'NONE',  ( -3.654804927335652209, 6.421633627603656080, 1.199719254218452935 ) ) ;
#132751=CARTESIAN_POINT ( 'NONE',  ( 3.067887898442204442, 6.801229324816399746, 0.7998128361456271485 ) ) ;
#132789=CARTESIAN_POINT ( 'NONE',  ( 6.211043768836185031, 6.418841616496599123, 0.7216878364870328300 ) ) ;
#132796=CARTESIAN_POINT ( 'NONE',  ( 5.356880090730857802, 8.303424968277756335, 1.082531754730548412 ) ) ;
#132810=CARTESIAN_POINT ( 'NONE',  ( -5.257529707049291900, 9.355811434857983500, 0.7998128361456291469 ) ) ;
#132821=CARTESIAN_POINT ( 'NONE',  ( 4.434925645001613681, 5.307073019657559065, -1.082531754730548412 ) ) ;
#132827=CARTESIAN_POINT ( 'NONE',  ( -7.611976899429754084, 7.845337568948314022, 0.7998128361456341429 ) ) ;
#132833=CARTESIAN_POINT ( 'NONE',  ( -5.804299160426237059, 7.865044668620976509, -1.443375672974066548 ) ) ;
#132836=CARTESIAN_POINT ( 'NONE',  ( -6.635789839245807897, 6.706452665400368218, 0.7998128361456341429 ) ) ;
#132854=CARTESIAN_POINT ( 'NONE',  ( -3.363831509966363598, 5.978201624052440266, -1.082531754730548412 ) ) ;
#132856=CARTESIAN_POINT ( 'NONE',  ( -5.610041701004606196, 9.767075427805856691, -0.7998128361456362523 ) ) ;
#132857=CARTESIAN_POINT ( 'NONE',  ( 5.086243903782109221, 5.962981304947771122, -1.199719254218452047 ) ) ;
#132858=CARTESIAN_POINT ( 'NONE',  ( -6.656127069666307072, 6.730179434224282886, 0.7998128361456341429 ) ) ;
#132910=CARTESIAN_POINT ( 'NONE',  ( 4.923546060418115822, 5.773167154356443120, -1.199719254218452047 ) ) ;
#132912=CARTESIAN_POINT ( 'NONE',  ( 2.796816994357219865, 2.968434822912331850, -2.452793345967703154 ) ) ;
#132922=CARTESIAN_POINT ( 'NONE',  ( 4.629651883607522223, 8.329987488807731211, -0.3686744245932921937 ) ) ;
#132924=CARTESIAN_POINT ( 'NONE',  ( 5.076602173674213070, 4.887400388900169368, 0.000000000000000000 ) ) ;
#132930=CARTESIAN_POINT ( 'NONE',  ( -5.586841817283045408, 8.675676665875643678, 1.199719254218454489 ) ) ;
#132936=CARTESIAN_POINT ( 'NONE',  ( -6.034787771414192648, 9.094317262408276648, 1.082531754730549967 ) ) ;
#132945=CARTESIAN_POINT ( 'NONE',  ( 5.207740401424913124, 9.089797878388800711, -0.7216878364870458196 ) ) ;
#132948=CARTESIAN_POINT ( 'NONE',  ( -4.122561227007127016, 6.967349310553715647, 1.199719254218452935 ) ) ;
#132960=CARTESIAN_POINT ( 'NONE',  ( 3.932747076415766596, 6.745899468197171345, 1.199719254218451159 ) ) ;
#132961=CARTESIAN_POINT ( 'NONE',  ( 3.386504508363381571, 7.172948703057747011, -0.7998128361456362523 ) ) ;
#132962=ORIENTED_EDGE ( 'NONE', *, *, #143867, .T. ) ;
#132979=DIRECTION ( 'NONE',  ( 0.000000000000000000, 1.000000000000000000, 0.000000000000000000 ) ) ;
#132986=CARTESIAN_POINT ( 'NONE',  ( 7.075376061485196821, 9.347967719856493218, 1.599625672291268286 ) ) ;
#132994=CARTESIAN_POINT ( 'NONE',  ( 5.559725510055676168, 8.644040974110419384, 1.199719254218451159 ) ) ;
#133003=CARTESIAN_POINT ( 'NONE',  ( 5.722950238744211937, 5.849399164722627553, 0.7216878364870328300 ) ) ;
#133006=CARTESIAN_POINT ( 'NONE',  ( 6.617788377246179188, 8.814115421577600529, -1.443375672974078761 ) ) ;
#133018=CARTESIAN_POINT ( 'NONE',  ( -4.977251789992602760, 8.820894498384422633, 0.000000000000000000 ) ) ;
#133047=ORIENTED_EDGE ( 'NONE', *, *, #201142, .F. ) ;
#133051=CARTESIAN_POINT ( 'NONE',  ( 7.018280793729500644, 8.217024343219755167, -1.199719254218452047 ) ) ;
#133054=CARTESIAN_POINT ( 'NONE',  ( 5.091969210384201361, 8.098325291160362482, 1.199719254218452047 ) ) ;
#133070=CARTESIAN_POINT ( 'NONE',  ( -4.111865726694519552, 8.019203457777400956, 0.000000000000000000 ) ) ;
#133072=CARTESIAN_POINT ( 'NONE',  ( 4.353576723319599218, 8.093273587265928271, -0.7216878364870357165 ) ) ;
#133086=CARTESIAN_POINT ( 'NONE',  ( -7.119440060951841787, 7.478637290631501067, 0.000000000000000000 ) ) ;
#133088=CARTESIAN_POINT ( 'NONE',  ( -4.990809943606286048, 5.955604701363006015, -1.082531754730549967 ) ) ;
#133115=CARTESIAN_POINT ( 'NONE',  ( -5.191846479390389568, 5.021852078902356631, 0.7998128361456281477 ) ) ;
#133126=CARTESIAN_POINT ( 'NONE',  ( 6.181863768892743138, 5.311700300033169952, -2.438145242048101569 ) ) ;
#133127=CARTESIAN_POINT ( 'NONE',  ( -5.058680321808019187, 7.974527835229765493, -1.188367278328520849 ) ) ;
#133143=CARTESIAN_POINT ( 'NONE',  ( 6.561219994370630637, 6.619454513046008515, 0.000000000000000000 ) ) ;
#133166=CARTESIAN_POINT ( 'NONE',  ( 5.559725510055676168, 8.644040974110419384, 1.199719254218451159 ) ) ;
#133167=CARTESIAN_POINT ( 'NONE',  ( 5.737035277238070385, 6.722237907313067140, -1.199719254218452047 ) ) ;
#133169=CARTESIAN_POINT ( 'NONE',  ( 5.337069745634900997, 6.255611453776062980, 1.199719254218452047 ) ) ;
#133181=CYLINDRICAL_SURFACE ( 'NONE', #31858, 0.08000000000000020983 ) ;
#133182=CARTESIAN_POINT ( 'NONE',  ( 4.623177087595867540, 8.455029494522658950, -0.3425024339245314464 ) ) ;
#133183=CARTESIAN_POINT ( 'NONE',  ( -5.112833325684908559, 8.018703742390766109, -1.082531754730549967 ) ) ;
#133184=CARTESIAN_POINT ( 'NONE',  ( 3.906157654512984134, 7.571284673658201569, -0.7216878364870338292 ) ) ;
#133207=CARTESIAN_POINT ( 'NONE',  ( 3.867818961648523235, 7.734482231890414283, 1.040834085586084257E-14 ) ) ;
#133208=CARTESIAN_POINT ( 'NONE',  ( 3.898851692381625877, 6.706354853490643642, -1.199719254218452047 ) ) ;
#133237=CARTESIAN_POINT ( 'NONE',  ( 5.155843554946782703, 9.237177590738404831, -0.7998128361456481317 ) ) ;
#133241=CARTESIAN_POINT ( 'NONE',  ( -6.184982820901517186, 6.966600618058066630, 0.8941503475990535410 ) ) ;
#133242=CARTESIAN_POINT ( 'NONE',  ( 5.580062740476173566, 8.667767742934335828, 1.199719254218451159 ) ) ;
#133271=CARTESIAN_POINT ( 'NONE',  ( 4.760321332173959696, 4.726332107057286791, 0.000000000000000000 ) ) ;
#133276=CARTESIAN_POINT ( 'NONE',  ( -7.228432174741334038, 8.462200954400218578, -1.199719254218452047 ) ) ;
#133278=CARTESIAN_POINT ( 'NONE',  ( 6.176621499477501054, 9.363752961769195693, -1.199719254218452047 ) ) ;
#133291=CARTESIAN_POINT ( 'NONE',  ( -6.597731880524014159, 6.769412454161013670, -0.2479414380717175903 ) ) ;
#133301=B_SPLINE_CURVE_WITH_KNOTS ( 'NONE', 3,
 ( #30972, #95981, #113345, #81829 ),
 .UNSPECIFIED., .F., .F.,
 ( 4, 4 ),
 ( 0.0005609329959280208141, 0.0008723013827243832410 ),
 .UNSPECIFIED. ) ;
#133309=CARTESIAN_POINT ( 'NONE',  ( 6.319508997745523438, 9.426492026461511742, -1.082531754730548412 ) ) ;
#133325=CARTESIAN_POINT ( 'NONE',  ( -5.506019780925599960, 5.596313630600862510, 0.7216878364870257245 ) ) ;
#133327=CARTESIAN_POINT ( 'NONE',  ( 4.701645408888975197, 8.707279753670952971, 0.000000000000000000 ) ) ;
#133332=CARTESIAN_POINT ( 'NONE',  ( -5.113360211009450040, 5.994616996712990975, -1.199719254218453823 ) ) ;
#133342=CYLINDRICAL_SURFACE ( 'NONE', #120050, 1.250000000000000000 ) ;
#133345=CARTESIAN_POINT ( 'NONE',  ( 6.170369307550806148, 10.21286493553572328, 0.7216878364870317197 ) ) ;
#133351=CARTESIAN_POINT ( 'NONE',  ( -2.981281212289682792, 6.492261378021210838, -0.0003813922843012157449 ) ) ;
#133352=CIRCLE ( 'NONE', #147093, 0.7499999999999997780 ) ;
#133376=CARTESIAN_POINT ( 'NONE',  ( 4.716257332707354699, 6.595662536282280719, -1.599625672291269396 ) ) ;
#133379=CARTESIAN_POINT ( 'NONE',  ( -5.822300622425855110, 5.757381912443740646, 0.7998128361456281477 ) ) ;
#133383=CARTESIAN_POINT ( 'NONE',  ( -5.275531169048901958, 8.208517892982092334, -1.082531754730549967 ) ) ;
#133388=CARTESIAN_POINT ( 'NONE',  ( -7.761116589180078407, 8.019333873657032541, 0.000000000000000000 ) ) ;
#133393=VERTEX_POINT ( 'NONE', #229 ) ;
#133398=CARTESIAN_POINT ( 'NONE',  ( -5.121948170912633991, 9.197632976031879792, -0.7998128361456362523 ) ) ;
#133399=DIRECTION ( 'NONE',  ( 0.6507913734559641616, -0.7592566023653004592, 0.000000000000000000 ) ) ;
#133401=CARTESIAN_POINT ( 'NONE',  ( 4.783863686166085039, 8.265937597628173705, 0.8363946479656783062 ) ) ;
#133406=CARTESIAN_POINT ( 'NONE',  ( 7.191674137406095291, 7.354984346587396082, 0.000000000000000000 ) ) ;
#133413=CARTESIAN_POINT ( 'NONE',  ( -4.522526758610270647, 7.433975764090723359, -1.199719254218453823 ) ) ;
#133418=CARTESIAN_POINT ( 'NONE',  ( -6.099189001301292379, 8.209082816308541197, 1.599625672291263179 ) ) ;
#133422=CARTESIAN_POINT ( 'NONE',  ( 6.156811153937166381, 10.19704708965311468, 0.000000000000000000 ) ) ;
#133424=CARTESIAN_POINT ( 'NONE',  ( -7.905812970100109638, 8.396072351304486148, 0.7216878364870317197 ) ) ;
#133430=CARTESIAN_POINT ( 'NONE',  ( 4.857564175446106525, 8.889184981320973122, 0.7998128361456331437 ) ) ;
#133438=( NAMED_UNIT ( * ) PLANE_ANGLE_UNIT ( ) SI_UNIT ( $, .RADIAN. ) );
#133445=CARTESIAN_POINT ( 'NONE',  ( 6.127784903196001665, 7.091900248975262500, -1.102264294108054266 ) ) ;
#133453=B_SPLINE_CURVE_WITH_KNOTS ( 'NONE', 3,
 ( #19781, #151938, #57637, #189754, #53359, #119493, #170303 ),
 .UNSPECIFIED., .F., .F.,
 ( 4, 3, 4 ),
 ( 0.000000000000000000, 6.254074696316652595E-05, 0.0001680160826026134415 ),
 .UNSPECIFIED. ) ;
#133456=EDGE_CURVE ( 'NONE', #130448, #179867, #36128, .T. ) ;
#133476=CARTESIAN_POINT ( 'NONE',  ( -6.202194133424988820, 6.954874670134298498, -0.8734430727420500196 ) ) ;
#133494=CARTESIAN_POINT ( 'NONE',  ( -4.685224601974262271, 7.623789914682047808, -1.199719254218453823 ) ) ;
#133508=CARTESIAN_POINT ( 'NONE',  ( 5.505492895601038938, 8.580769590579979678, -1.199719254218452047 ) ) ;
#133511=CARTESIAN_POINT ( 'NONE',  ( 6.577113915960825175, 8.766661883411348555, -1.443375672974078761 ) ) ;
#133524=CARTESIAN_POINT ( 'NONE',  ( -6.296835998904160014, 6.311006518335105397, 0.000000000000000000 ) ) ;
#133525=CARTESIAN_POINT ( 'NONE',  ( 4.179656494762836516, 8.098292687190454586, -0.7998128361456362523 ) ) ;
#133535=CARTESIAN_POINT ( 'NONE',  ( -3.383641855062333281, 6.105276709951447778, -1.199719254218452047 ) ) ;
#133536=CARTESIAN_POINT ( 'NONE',  ( 4.947799714344386146, 4.737130853015369958, -0.7998128361456481317 ) ) ;
#133538=CARTESIAN_POINT ( 'NONE',  ( -4.496171506534503592, 8.048216686630619066, -2.444650791391935307 ) ) ;
#133543=CARTESIAN_POINT ( 'NONE',  ( 5.252858170651868441, 5.093032385374103299, -0.7998128361456481317 ) ) ;
#133549=CARTESIAN_POINT ( 'NONE',  ( -5.939261241470221719, 7.227352081167748743, 1.243796156610659454 ) ) ;
#133558=CARTESIAN_POINT ( 'NONE',  ( -5.126391479298592735, 5.153413945369351268, 0.000000000000000000 ) ) ;
#133565=CARTESIAN_POINT ( 'NONE',  ( -5.293864907607930270, 4.747529046662118724, 2.500000000000000444 ) ) ;
#133579=( BOUNDED_SURFACE ( )  B_SPLINE_SURFACE ( 1, 2, ( 
 ( #68738, #200867, #83938, #33071, #99149, #35179, #66592, #116507, #169460, #102326, #118645, #166263, #132735, #198739, #101256, #168399, #117579, #151101, #86080, #152155, #3726, #150028, #70863, #185694, #1597, #67658, #2665, #136978, #167339, #133804, #199814, #51458, #18925, #134859, #76231, #141284, #171591, #107740, #170523, #75174, #40548, #206219, #186770, #139111, #25341, #108805, #207293, #24256, #105558, #173764, #92519, #74105, #172679, #23185, #157503, #26407, #205139, #204058, #9098, #208350, #39462, #125076, #8014, #189974, #138045, #90362, #106652, #55711, #140197, #57846, #89300, #142341, #38397, #122949, #5863, #121864, #174829, #124007, #41625, #187835, #88218, #120793, #188908, #91441, #56782, #156428, #58917, #191032, #42699, #104476, #158558, #10156, #154288, #155349, #22106, #71935, #6933, #73013, #126134, #11217, #143411, #109875, #59981, #192095, #27478, #77299, #43761, #175887, #93577, #159623, #115652, #67873, #168609, #37546, #136130, #167548, #34335, #36473, #21266, #2879, #101477, #100410, #86299, #20211, #19148, #166479, #152369, #18071, #198950, #84159, #3947, #103626, #52725, #185912, #1815, #182717, #33273, #70014, #71086, #137203, #102545, #150246, #134019, #200026, #51678, #165409, #50592, #117799, #49528, #183791, #83080, #17005, #116717, #202145, #53806, #169678, #181647, #85222, #35399, #87371, #99358, #119936, #118858, #153441, #68950, #149159, #151311, #135071, #201084, #5013, #737, #184844, #66803, #132945, #189135, #191250, #138268, #154509, #41849, #40774, #106879, #38622, #89524, #42915, #204282, #6090, #107960, #172905, #24480, #104699, #155578, #109025, #73232, #72159, #91671, #76449, #122092, #207514, #90592, #58069, #55939, #156651, #8244, #188056, #74328, #140430, #39685, #10372, #121024, #205369, #88450, #105797, #175044, #206442, #124232, #171820, #170750, #203226, #57004, #190191, #139339, #173987, #25560, #157724, #9319, #186991, #26629, #75393, #22336, #23413, #141505, #59132, #123176, #125291, #7161, #92731, #54870, #158776, #156094, #11953, #41293 ),
 ( #94310, #192829, #9824, #91107, #93244, #78026, #59645, #158233, #157168, #143077, #76952, #75900, #8760, #209070, #74841, #107401, #140941, #60707, #160351, #109545, #28217, #58584, #25005, #90035, #126871, #127952, #193905, #159278, #206955, #124739, #190698, #42359, #7679, #173423, #108471, #106319, #174494, #139858, #73763, #26071, #44487, #110604, #144150, #172343, #142004, #92183, #210142, #23931, #176605, #175549, #61786, #125803, #205889, #208019, #191766, #43421, #57522, #123680, #27138, #10877, #189642, #31422, #16195, #97498, #96445, #148371, #162496, #194977, #14068, #214370, #99608, #48739, #181901, #212273, #178745, #29286, #82276, #67071, #133207, #98546, #146260, #30358, #63908, #80155, #161429, #46613, #47689, #45553, #130064, #79089, #13012, #112735, #66000, #132150, #33536, #111669, #81226, #196057, #165674, #177676, #198156, #114852, #49789, #213334, #95380, #113801, #179803, #163555, #115915, #145207, #15138, #147308, #64959, #131111, #17263, #197098, #211213, #164610, #180852, #32474, #62838, #83339, #149424, #1007, #129000, #87626, #72419, #118058, #203474, #86556, #54062, #2071, #36725, #185098, #134275, #152620, #4207, #35660, #6347, #116983, #201343, #84421, #68142, #187248, #202407, #70275, #200283, #166746, #199211, #52983, #136391, #135329, #102811, #37807, #120197, #103882, #182983, #104960, #186173, #18340, #101739, #168867, #55128, #119119, #169930, #150510, #71343, #50858, #85486, #69209, #171001, #19407, #20470, #34600, #153697, #21514, #5266, #100668, #3139, #137459, #38875, #121273, #22599, #184043, #88706, #154764, #51934, #167808, #151572, #175290, #43168, #126603, #10618, #42097, #123423, #125540, #110342, #91918, #190437, #189385, #26876, #109281, #108212, #41027, #92979, #107137, #73497, #173161, #159025, #192565, #141751, #60445, #90843, #57261, #122353, #76693, #160086, #11688, #191502, #24742, #156906, #8495, #74577, #39952, #139598, #140680, #138520, #206696, #172081, #106059, #205621, #142809, #208813, #44220, #204544, #174235, #58324, #176345, #56192, #27953, #207758 ) ),
 .UNSPECIFIED., .F., .F., .T. ) 
 B_SPLINE_SURFACE_WITH_KNOTS ( ( 2, 2 ),
 ( 3, 2, 2, 2, 2, 2, 2, 2, 2, 2, 2, 2, 2, 2, 2, 2, 2, 2, 2, 2, 2, 2, 2, 2, 2, 2, 2, 2, 2, 2, 2, 2, 2, 2, 2, 2, 2, 2, 2, 2, 2, 2, 2, 2, 2, 2, 2, 2, 2, 2, 2, 2, 2, 2, 2, 2, 2, 2, 2, 2, 2, 2, 2, 2, 2, 2, 2, 2, 2, 2, 2, 2, 2, 2, 2, 2, 2, 2, 2, 2, 2, 2, 2, 2, 2, 2, 2, 2, 2, 2, 2, 2, 2, 2, 2, 2, 2, 2, 2, 2, 2, 2, 2, 2, 2, 2, 2, 2, 2, 2, 2, 2, 2, 2, 2, 2, 2, 2, 2, 2, 3 ),
 ( 0.000000000000000000, 1.000000000000000000 ),
 ( 0.000000000000000000, 0.008333333333333333218, 0.01666666666666666644, 0.02500000000000000139, 0.03333333333333333287, 0.04166666666666666435, 0.05000000000000000278, 0.05833333333333333426, 0.06666666666666666574, 0.07499999999999999722, 0.08333333333333332871, 0.09166666666666666019, 0.1000000000000000056, 0.1083333333333333370, 0.1166666666666666685, 0.1250000000000000000, 0.1333333333333333315, 0.1416666666666666630, 0.1499999999999999944, 0.1583333333333333259, 0.1666666666666666574, 0.1749999999999999889, 0.1833333333333333204, 0.1916666666666666796, 0.2000000000000000111, 0.2083333333333333426, 0.2166666666666666741, 0.2250000000000000056, 0.2333333333333333370, 0.2416666666666666685, 0.2500000000000000000, 0.2583333333333333592, 0.2666666666666666630, 0.2750000000000000222, 0.2833333333333333259, 0.2916666666666666852, 0.2999999999999999889, 0.3083333333333333481, 0.3166666666666666519, 0.3250000000000000111, 0.3333333333333333148, 0.3416666666666666741, 0.3499999999999999778, 0.3583333333333333370, 0.3666666666666666408, 0.3750000000000000000, 0.3833333333333333592, 0.3916666666666666630, 0.4000000000000000222, 0.4083333333333333259, 0.4166666666666666852, 0.4249999999999999889, 0.4333333333333333481, 0.4416666666666666519, 0.4500000000000000111, 0.4583333333333333148, 0.4666666666666666741, 0.4749999999999999778, 0.4833333333333333370, 0.4916666666666666408, 0.5000000000000000000, 0.5083333333333333037, 0.5166666666666667185, 0.5250000000000000222, 0.5333333333333333259, 0.5416666666666666297, 0.5500000000000000444, 0.5583333333333333481, 0.5666666666666666519, 0.5749999999999999556, 0.5833333333333333703, 0.5916666666666666741, 0.5999999999999999778, 0.6083333333333332815, 0.6166666666666666963, 0.6250000000000000000, 0.6333333333333333037, 0.6416666666666667185, 0.6500000000000000222, 0.6583333333333333259, 0.6666666666666666297, 0.6750000000000000444, 0.6833333333333333481, 0.6916666666666666519, 0.6999999999999999556, 0.7083333333333333703, 0.7166666666666666741, 0.7249999999999999778, 0.7333333333333332815, 0.7416666666666666963, 0.7500000000000000000, 0.7583333333333333037, 0.7666666666666667185, 0.7750000000000000222, 0.7833333333333333259, 0.7916666666666666297, 0.8000000000000000444, 0.8083333333333333481, 0.8166666666666666519, 0.8249999999999999556, 0.8333333333333333703, 0.8416666666666666741, 0.8499999999999999778, 0.8583333333333332815, 0.8666666666666666963, 0.8750000000000000000, 0.8833333333333333037, 0.8916666666666667185, 0.9000000000000000222, 0.9083333333333333259, 0.9166666666666666297, 0.9250000000000000444, 0.9333333333333333481, 0.9416666666666666519, 0.9499999999999999556, 0.9583333333333333703, 0.9666666666666666741, 0.9749999999999999778, 0.9833333333333332815, 0.9916666666666666963, 1.000000000000000000 ),
 .UNSPECIFIED. ) 
 GEOMETRIC_REPRESENTATION_ITEM ( )  RATIONAL_B_SPLINE_SURFACE ( (
 ( 1.000000000000000000, 0.8660254037844387076, 1.000000000000000000, 0.8660254037844387076, 1.000000000000000000, 0.8660254037844387076, 1.000000000000000000, 0.8660254037844387076, 1.000000000000000000, 0.8660254037844387076, 1.000000000000000000, 0.8660254037844387076, 1.000000000000000000, 0.8660254037844387076, 1.000000000000000000, 0.8660254037844387076, 1.000000000000000000, 0.8660254037844387076, 1.000000000000000000, 0.8660254037844387076, 1.000000000000000000, 0.8660254037844387076, 1.000000000000000000, 0.8660254037844387076, 1.000000000000000000, 0.8660254037844387076, 1.000000000000000000, 0.8660254037844387076, 1.000000000000000000, 0.8660254037844387076, 1.000000000000000000, 0.8660254037844387076, 1.000000000000000000, 0.8660254037844387076, 1.000000000000000000, 0.8660254037844387076, 1.000000000000000000, 0.8660254037844387076, 1.000000000000000000, 0.8660254037844387076, 1.000000000000000000, 0.8660254037844387076, 1.000000000000000000, 0.8660254037844387076, 1.000000000000000000, 0.8660254037844387076, 1.000000000000000000, 0.8660254037844387076, 1.000000000000000000, 0.8660254037844387076, 1.000000000000000000, 0.8660254037844387076, 1.000000000000000000, 0.8660254037844387076, 1.000000000000000000, 0.8660254037844387076, 1.000000000000000000, 0.8660254037844387076, 1.000000000000000000, 0.8660254037844387076, 1.000000000000000000, 0.8660254037844387076, 1.000000000000000000, 0.8660254037844387076, 1.000000000000000000, 0.8660254037844387076, 1.000000000000000000, 0.8660254037844387076, 1.000000000000000000, 0.8660254037844387076, 1.000000000000000000, 0.8660254037844387076, 1.000000000000000000, 0.8660254037844387076, 1.000000000000000000, 0.8660254037844387076, 1.000000000000000000, 0.8660254037844387076, 1.000000000000000000, 0.8660254037844387076, 1.000000000000000000, 0.8660254037844387076, 1.000000000000000000, 0.8660254037844387076, 1.000000000000000000, 0.8660254037844387076, 1.000000000000000000, 0.8660254037844387076, 1.000000000000000000, 0.8660254037844387076, 1.000000000000000000, 0.8660254037844387076, 1.000000000000000000, 0.8660254037844387076, 1.000000000000000000, 0.8660254037844387076, 1.000000000000000000, 0.8660254037844387076, 1.000000000000000000, 0.8660254037844387076, 1.000000000000000000, 0.8660254037844387076, 1.000000000000000000, 0.8660254037844387076, 1.000000000000000000, 0.8660254037844387076, 1.000000000000000000, 0.8660254037844387076, 1.000000000000000000, 0.8660254037844387076, 1.000000000000000000, 0.8660254037844387076, 1.000000000000000000, 0.8660254037844387076, 1.000000000000000000, 0.8660254037844387076, 1.000000000000000000, 0.8660254037844387076, 1.000000000000000000, 0.8660254037844387076, 1.000000000000000000, 0.8660254037844387076, 1.000000000000000000, 0.8660254037844387076, 1.000000000000000000, 0.8660254037844387076, 1.000000000000000000, 0.8660254037844387076, 1.000000000000000000, 0.8660254037844387076, 1.000000000000000000, 0.8660254037844387076, 1.000000000000000000, 0.8660254037844387076, 1.000000000000000000, 0.8660254037844387076, 1.000000000000000000, 0.8660254037844387076, 1.000000000000000000, 0.8660254037844387076, 1.000000000000000000, 0.8660254037844387076, 1.000000000000000000, 0.8660254037844387076, 1.000000000000000000, 0.8660254037844387076, 1.000000000000000000, 0.8660254037844387076, 1.000000000000000000, 0.8660254037844387076, 1.000000000000000000, 0.8660254037844387076, 1.000000000000000000, 0.8660254037844387076, 1.000000000000000000, 0.8660254037844387076, 1.000000000000000000, 0.8660254037844387076, 1.000000000000000000, 0.8660254037844387076, 1.000000000000000000, 0.8660254037844387076, 1.000000000000000000, 0.8660254037844387076, 1.000000000000000000, 0.8660254037844387076, 1.000000000000000000, 0.8660254037844387076, 1.000000000000000000, 0.8660254037844387076, 1.000000000000000000, 0.8660254037844387076, 1.000000000000000000, 0.8660254037844387076, 1.000000000000000000, 0.8660254037844387076, 1.000000000000000000, 0.8660254037844387076, 1.000000000000000000, 0.8660254037844387076, 1.000000000000000000, 0.8660254037844387076, 1.000000000000000000, 0.8660254037844387076, 1.000000000000000000, 0.8660254037844387076, 1.000000000000000000, 0.8660254037844387076, 1.000000000000000000, 0.8660254037844387076, 1.000000000000000000, 0.8660254037844387076, 1.000000000000000000, 0.8660254037844387076, 1.000000000000000000, 0.8660254037844387076, 1.000000000000000000, 0.8660254037844387076, 1.000000000000000000, 0.8660254037844387076, 1.000000000000000000, 0.8660254037844387076, 1.000000000000000000, 0.8660254037844387076, 1.000000000000000000, 0.8660254037844387076, 1.000000000000000000, 0.8660254037844387076, 1.000000000000000000, 0.8660254037844387076, 1.000000000000000000, 0.8660254037844387076, 1.000000000000000000, 0.8660254037844387076, 1.000000000000000000, 0.8660254037844387076, 1.000000000000000000, 0.8660254037844387076, 1.000000000000000000, 0.8660254037844387076, 1.000000000000000000, 0.8660254037844387076, 1.000000000000000000, 0.8660254037844387076, 1.000000000000000000, 0.8660254037844387076, 1.000000000000000000, 0.8660254037844387076, 1.000000000000000000, 0.8660254037844387076, 1.000000000000000000, 0.8660254037844387076, 1.000000000000000000, 0.8660254037844387076, 1.000000000000000000, 0.8660254037844387076, 1.000000000000000000, 0.8660254037844387076, 1.000000000000000000, 0.8660254037844387076, 1.000000000000000000),
 ( 1.000000000000000000, 0.8660254037844387076, 1.000000000000000000, 0.8660254037844387076, 1.000000000000000000, 0.8660254037844387076, 1.000000000000000000, 0.8660254037844387076, 1.000000000000000000, 0.8660254037844387076, 1.000000000000000000, 0.8660254037844387076, 1.000000000000000000, 0.8660254037844387076, 1.000000000000000000, 0.8660254037844387076, 1.000000000000000000, 0.8660254037844387076, 1.000000000000000000, 0.8660254037844387076, 1.000000000000000000, 0.8660254037844387076, 1.000000000000000000, 0.8660254037844387076, 1.000000000000000000, 0.8660254037844387076, 1.000000000000000000, 0.8660254037844387076, 1.000000000000000000, 0.8660254037844387076, 1.000000000000000000, 0.8660254037844387076, 1.000000000000000000, 0.8660254037844387076, 1.000000000000000000, 0.8660254037844387076, 1.000000000000000000, 0.8660254037844387076, 1.000000000000000000, 0.8660254037844387076, 1.000000000000000000, 0.8660254037844387076, 1.000000000000000000, 0.8660254037844387076, 1.000000000000000000, 0.8660254037844387076, 1.000000000000000000, 0.8660254037844387076, 1.000000000000000000, 0.8660254037844387076, 1.000000000000000000, 0.8660254037844387076, 1.000000000000000000, 0.8660254037844387076, 1.000000000000000000, 0.8660254037844387076, 1.000000000000000000, 0.8660254037844387076, 1.000000000000000000, 0.8660254037844387076, 1.000000000000000000, 0.8660254037844387076, 1.000000000000000000, 0.8660254037844387076, 1.000000000000000000, 0.8660254037844387076, 1.000000000000000000, 0.8660254037844387076, 1.000000000000000000, 0.8660254037844387076, 1.000000000000000000, 0.8660254037844387076, 1.000000000000000000, 0.8660254037844387076, 1.000000000000000000, 0.8660254037844387076, 1.000000000000000000, 0.8660254037844387076, 1.000000000000000000, 0.8660254037844387076, 1.000000000000000000, 0.8660254037844387076, 1.000000000000000000, 0.8660254037844387076, 1.000000000000000000, 0.8660254037844387076, 1.000000000000000000, 0.8660254037844387076, 1.000000000000000000, 0.8660254037844387076, 1.000000000000000000, 0.8660254037844387076, 1.000000000000000000, 0.8660254037844387076, 1.000000000000000000, 0.8660254037844387076, 1.000000000000000000, 0.8660254037844387076, 1.000000000000000000, 0.8660254037844387076, 1.000000000000000000, 0.8660254037844387076, 1.000000000000000000, 0.8660254037844387076, 1.000000000000000000, 0.8660254037844387076, 1.000000000000000000, 0.8660254037844387076, 1.000000000000000000, 0.8660254037844387076, 1.000000000000000000, 0.8660254037844387076, 1.000000000000000000, 0.8660254037844387076, 1.000000000000000000, 0.8660254037844387076, 1.000000000000000000, 0.8660254037844387076, 1.000000000000000000, 0.8660254037844387076, 1.000000000000000000, 0.8660254037844387076, 1.000000000000000000, 0.8660254037844387076, 1.000000000000000000, 0.8660254037844387076, 1.000000000000000000, 0.8660254037844387076, 1.000000000000000000, 0.8660254037844387076, 1.000000000000000000, 0.8660254037844387076, 1.000000000000000000, 0.8660254037844387076, 1.000000000000000000, 0.8660254037844387076, 1.000000000000000000, 0.8660254037844387076, 1.000000000000000000, 0.8660254037844387076, 1.000000000000000000, 0.8660254037844387076, 1.000000000000000000, 0.8660254037844387076, 1.000000000000000000, 0.8660254037844387076, 1.000000000000000000, 0.8660254037844387076, 1.000000000000000000, 0.8660254037844387076, 1.000000000000000000, 0.8660254037844387076, 1.000000000000000000, 0.8660254037844387076, 1.000000000000000000, 0.8660254037844387076, 1.000000000000000000, 0.8660254037844387076, 1.000000000000000000, 0.8660254037844387076, 1.000000000000000000, 0.8660254037844387076, 1.000000000000000000, 0.8660254037844387076, 1.000000000000000000, 0.8660254037844387076, 1.000000000000000000, 0.8660254037844387076, 1.000000000000000000, 0.8660254037844387076, 1.000000000000000000, 0.8660254037844387076, 1.000000000000000000, 0.8660254037844387076, 1.000000000000000000, 0.8660254037844387076, 1.000000000000000000, 0.8660254037844387076, 1.000000000000000000, 0.8660254037844387076, 1.000000000000000000, 0.8660254037844387076, 1.000000000000000000, 0.8660254037844387076, 1.000000000000000000, 0.8660254037844387076, 1.000000000000000000, 0.8660254037844387076, 1.000000000000000000, 0.8660254037844387076, 1.000000000000000000, 0.8660254037844387076, 1.000000000000000000, 0.8660254037844387076, 1.000000000000000000, 0.8660254037844387076, 1.000000000000000000, 0.8660254037844387076, 1.000000000000000000, 0.8660254037844387076, 1.000000000000000000, 0.8660254037844387076, 1.000000000000000000, 0.8660254037844387076, 1.000000000000000000, 0.8660254037844387076, 1.000000000000000000, 0.8660254037844387076, 1.000000000000000000, 0.8660254037844387076, 1.000000000000000000, 0.8660254037844387076, 1.000000000000000000, 0.8660254037844387076, 1.000000000000000000, 0.8660254037844387076, 1.000000000000000000, 0.8660254037844387076, 1.000000000000000000, 0.8660254037844387076, 1.000000000000000000, 0.8660254037844387076, 1.000000000000000000, 0.8660254037844387076, 1.000000000000000000, 0.8660254037844387076, 1.000000000000000000, 0.8660254037844387076, 1.000000000000000000, 0.8660254037844387076, 1.000000000000000000, 0.8660254037844387076, 1.000000000000000000, 0.8660254037844387076, 1.000000000000000000, 0.8660254037844387076, 1.000000000000000000, 0.8660254037844387076, 1.000000000000000000, 0.8660254037844387076, 1.000000000000000000) ) ) 
 REPRESENTATION_ITEM ( '' )  SURFACE ( )  );
#133582=CARTESIAN_POINT ( 'NONE',  ( -6.014495906177975471, 7.161312607523874441, -1.265080238494860509 ) ) ;
#133603=ORIENTED_EDGE ( 'NONE', *, *, #8484, .T. ) ;
#133616=CARTESIAN_POINT ( 'NONE',  ( 5.890091390494168522, 5.836471141856793388, 0.000000000000000000 ) ) ;
#133642=CARTESIAN_POINT ( 'NONE',  ( -6.526270840131767059, 8.707344961610770540, -1.599625672291271394 ) ) ;
#133644=CARTESIAN_POINT ( 'NONE',  ( 6.658462837642791676, 8.861568958707010779, 1.443375672974063439 ) ) ;
#133656=CARTESIAN_POINT ( 'NONE',  ( -6.668631453075260396, 8.873432343378178544, -1.599625672291271394 ) ) ;
#133663=CARTESIAN_POINT ( 'NONE',  ( 4.913904330310220558, 4.697586238308844919, 0.000000000000000000 ) ) ;
#133668=CARTESIAN_POINT ( 'NONE',  ( -3.935609729716867289, 7.813571461303467913, 0.7998128361456352531 ) ) ;
#133671=CARTESIAN_POINT ( 'NONE',  ( -5.790741006812557323, 9.769965251341050205, 0.000000000000000000 ) ) ;
#133674=CARTESIAN_POINT ( 'NONE',  ( 3.065552130021340194, 6.590578228417936835, 0.000000000000000000 ) ) ;
#133675=CARTESIAN_POINT ( 'NONE',  ( -8.120407659942227241, 8.438506789546210030, 0.7998128361456341429 ) ) ;
#133690=CARTESIAN_POINT ( 'NONE',  ( -0.001447835942344739097, 2.586556732995649366, 2.083545908858529749 ) ) ;
#133694=CARTESIAN_POINT ( 'NONE',  ( 0.1054570145121072472, 2.614151819895196738, -2.076146791065091701 ) ) ;
#133695=CARTESIAN_POINT ( 'NONE',  ( 6.246047416222394233, 7.008439898793222156, -0.9866338212708870570 ) ) ;
#133701=CARTESIAN_POINT ( 'NONE',  ( 5.558836782162523527, 7.518240855878357110, -1.384758111419038817 ) ) ;
#133715=CARTESIAN_POINT ( 'NONE',  ( 5.441225816562971218, 7.512442699629209741, -1.249814574298679926 ) ) ;
#133730=CARTESIAN_POINT ( 'NONE',  ( 7.472478939787284169, 8.746922180287201698, 1.199719254218452935 ) ) ;
#133733=CARTESIAN_POINT ( 'NONE',  ( -5.010620288702242853, 8.003418215864698482, -1.199719254218453823 ) ) ;
#133746=CARTESIAN_POINT ( 'NONE',  ( 5.896870467300973750, 5.844380064798101237, 0.7998128361456352531 ) ) ;
#133748=CARTESIAN_POINT ( 'NONE',  ( 7.828907357248368726, 8.098423103070084395, 0.7998128361456281477 ) ) ;
#133753=CARTESIAN_POINT ( 'NONE',  ( -6.956742217143487395, 8.249192353823097790, 1.082531754730549078 ) ) ;
#133758=CARTESIAN_POINT ( 'NONE',  ( 8.039058738260216330, 8.343599714250547805, -0.7998128361456341429 ) ) ;
#133764=CARTESIAN_POINT ( 'NONE',  ( 1.865749732055407728, 8.973930515401084662, 0.7750000000000004663 ) ) ;
#133770=AXIS2_PLACEMENT_3D ( 'NONE', #58976, #56841, #74167 ) ;
#133772=CARTESIAN_POINT ( 'NONE',  ( -5.478903473698247595, 8.445785581739666981, -1.082531754730549967 ) ) ;
#133773=CARTESIAN_POINT ( 'NONE',  ( 6.400857919427532572, 6.640291458853147866, -0.7216878364870458196 ) ) ;
#133776=EDGE_CURVE ( 'NONE', #128754, #128826, #134432, .T. ) ;
#133784=CARTESIAN_POINT ( 'NONE',  ( -5.093022980588950865, 5.970890227889075419, -1.199719254218453823 ) ) ;
#133785=CARTESIAN_POINT ( 'NONE',  ( -5.465345320084574965, 9.390336950158399532, 0.000000000000000000 ) ) ;
#133786=CARTESIAN_POINT ( 'NONE',  ( 1.836270655118562800, 2.510430850797893410, -2.497621424930284384 ) ) ;
#133789=CARTESIAN_POINT ( 'NONE',  ( 5.519577934094861860, 6.572500690266394940, 1.082531754730549078 ) ) ;
#133791=ORIENTED_EDGE ( 'NONE', *, *, #199073, .F. ) ;
#133799=CARTESIAN_POINT ( 'NONE',  ( -5.288707357724018898, 7.660230058424141397, 1.223219983389673748 ) ) ;
#133803=DIRECTION ( 'NONE',  ( 0.000000000000000000, 0.000000000000000000, 1.000000000000000000 ) ) ;
#133804=CARTESIAN_POINT ( 'NONE',  ( 3.255366281057017197, 6.812028071292901998, -0.7216878364870338292 ) ) ;
#133806=CARTESIAN_POINT ( 'NONE',  ( -6.303615075710993665, 6.318915441276411471, -0.7998128361456362523 ) ) ;
#133817=ADVANCED_FACE ( 'NONE', ( #119418 ), #73459, .T. ) ;
#133818=CARTESIAN_POINT ( 'NONE',  ( 4.686278372178935392, 5.496354851410763409, 1.199719254218452047 ) ) ;
#133826=AXIS2_PLACEMENT_3D ( 'NONE', #59924, #126079, #110879 ) ;
#133829=EDGE_CURVE ( 'NONE', #184855, #154238, #184086, .T. ) ;
#133832=CARTESIAN_POINT ( 'NONE',  ( 3.024201889537345700, 6.315044714278881699, 0.6036835607809933890 ) ) ;
#133860=CARTESIAN_POINT ( 'NONE',  ( 4.584065335196252811, 8.362176967788721882, 0.7216878364870328300 ) ) ;
#133867=CARTESIAN_POINT ( 'NONE',  ( 6.170369307550823912, 7.331757292631694511, 1.082531754730549967 ) ) ;
#133891=CARTESIAN_POINT ( 'NONE',  ( 5.221298554594243413, 5.264138866547622975, -0.7216878364870458196 ) ) ;
#133897=CARTESIAN_POINT ( 'NONE',  ( -5.966470118465691641, 9.118576350588734059, -1.199719254218452047 ) ) ;
#133903=CARTESIAN_POINT ( 'NONE',  ( -4.489158259900630554, 8.251452046610447510, 0.000000000000000000 ) ) ;
#133907=CARTESIAN_POINT ( 'NONE',  ( -5.261446130555064826, 8.296048364692991228, 1.199719254218452935 ) ) ;
#133927=CARTESIAN_POINT ( 'NONE',  ( -4.340018570150318666, 6.156717313299049366, -1.443375672974066548 ) ) ;
#133930=CARTESIAN_POINT ( 'NONE',  ( -5.275531169048911728, 6.287779464379406491, -1.082531754730549967 ) ) ;
#133931=CARTESIAN_POINT ( 'NONE',  ( 3.464990776744291345, 6.200183785247111778, 1.199719254218452047 ) ) ;
#133932=CARTESIAN_POINT ( 'NONE',  ( -5.829079699232685208, 5.765290835385048496, 0.000000000000000000 ) ) ;
#133933=CARTESIAN_POINT ( 'NONE',  ( -6.038177310039794854, 8.137902509836795417, -1.599625672291271394 ) ) ;
#133949=CARTESIAN_POINT ( 'NONE',  ( -5.527925976246812034, 5.968540277179252840, -0.9326450038637500439 ) ) ;
#133964=ADVANCED_FACE ( 'NONE', ( #97823 ), #15463, .F. ) ;
#133985=CARTESIAN_POINT ( 'NONE',  ( 5.585032934186686226, 5.480569609498057382, 0.000000000000000000 ) ) ;
#134000=CARTESIAN_POINT ( 'NONE',  ( 4.768187943840554333, 8.164982483533503199, -0.7738548252242994918 ) ) ;
#134003=CARTESIAN_POINT ( 'NONE',  ( 3.203469434578891661, 6.959407783642502565, -0.7998128361456362523 ) ) ;
#134008=CARTESIAN_POINT ( 'NONE',  ( -6.961185525973791144, 7.086080966583015339, 0.7998128361456341429 ) ) ;
#134012=CARTESIAN_POINT ( 'NONE',  ( -8.068510813464099485, 8.585886501895810596, 0.7216878364870317197 ) ) ;
#134014=CARTESIAN_POINT ( 'NONE',  ( -3.765305043611756552, 7.354576300424668922, -0.6638232778202641793 ) ) ;
#134019=CARTESIAN_POINT ( 'NONE',  ( 6.211043768836181478, 7.379210830797944709, 1.082531754730549967 ) ) ;
#134021=CARTESIAN_POINT ( 'NONE',  ( -3.797692425159308716, 7.444741906078900406, 0.000000000000000000 ) ) ;
#134022=CARTESIAN_POINT ( 'NONE',  ( -6.310394152517827315, 6.326824364217716656, 0.7998128361456281477 ) ) ;
#134034=CARTESIAN_POINT ( 'NONE',  ( 3.393283585170187688, 7.180857625999046867, 0.7998128361456271485 ) ) ;
#134035=CARTESIAN_POINT ( 'NONE',  ( 4.980641328173811999, 6.904110530993182948, 1.599625672291269396 ) ) ;
#134054=CARTESIAN_POINT ( 'NONE',  ( 4.204437033569277560, 7.919277282557212416, 0.000000000000000000 ) ) ;
#134060=CARTESIAN_POINT ( 'NONE',  ( 5.982890925380405456, 10.20206618957764100, 0.000000000000000000 ) ) ;
#134067=CARTESIAN_POINT ( 'NONE',  ( 5.342795052237045539, 8.390955439988655229, -1.199719254218450271 ) ) ;
#134072=CARTESIAN_POINT ( 'NONE',  ( 6.061904079085887354, 6.244845311787889486, 0.000000000000000000 ) ) ;
#134075=CARTESIAN_POINT ( 'NONE',  ( 7.024532985656141371, 7.367912369453226695, 0.7216878364870328300 ) ) ;
#134086=CARTESIAN_POINT ( 'NONE',  ( 6.244837129360077732, 6.910362811036335096, 0.8058565020967979331 ) ) ;
#134088=CARTESIAN_POINT ( 'NONE',  ( -6.699137298928187434, 8.909022496873262753, 1.443375672974064550 ) ) ;
#134122=CARTESIAN_POINT ( 'NONE',  ( 5.345657705538078730, 9.458627433094950021, 0.7998128361456331437 ) ) ;
#134123=CARTESIAN_POINT ( 'NONE',  ( -5.763624699140883934, 6.857221916153382502, -1.082531754730549967 ) ) ;
#134124=CARTESIAN_POINT ( 'NONE',  ( 6.607619761813720238, 8.802252036906432764, 1.599625672291268286 ) ) ;
#134131=SHAPE_REPRESENTATION_RELATIONSHIP ( 'NONE' , 'NONE' ,  #11178, #210156 ) ;
#134138=CARTESIAN_POINT ( 'NONE',  ( -5.204350862799341115, 7.165104988056252289, -1.599625672291271394 ) ) ;
#134140=CARTESIAN_POINT ( 'NONE',  ( 5.709392084686216506, 5.833581318321598985, -0.7216878364870458196 ) ) ;
#134154=CARTESIAN_POINT ( 'NONE',  ( -6.861835142292179057, 9.098836647464588978, 1.443375672974064550 ) ) ;
#134156=CARTESIAN_POINT ( 'NONE',  ( -6.617788377246204945, 6.893376992974917350, -0.7216878364870338292 ) ) ;
#134179=CARTESIAN_POINT ( 'NONE',  ( -5.340986169140711226, 5.195848383611072485, 0.000000000000000000 ) ) ;
#134188=FACE_OUTER_BOUND ( 'NONE', #118617, .T. ) ;
#134189=CARTESIAN_POINT ( 'NONE',  ( -5.328968068096138211, 7.722205811214136517, -1.323081262718794893 ) ) ;
#134192=EDGE_LOOP ( 'NONE', ( #42011, #141133, #191162, #124469 ) ) ;
#134207=CARTESIAN_POINT ( 'NONE',  ( 4.538947565524982686, 8.517465603079630299, 0.000000000000000000 ) ) ;
#134227=EDGE_CURVE ( 'NONE', #22322, #52415, #173164, .T. ) ;
#134230=CARTESIAN_POINT ( 'NONE',  ( 5.481239241674765950, 9.616805891921051952, -0.7998128361456481317 ) ) ;
#134231=CARTESIAN_POINT ( 'NONE',  ( 6.062430963966053632, 7.101866208495718702, -1.199719254218452047 ) ) ;
#134233=CARTESIAN_POINT ( 'NONE',  ( 4.016958651398847557, 7.908478536599129249, -0.7998128361456362523 ) ) ;
#134238=CARTESIAN_POINT ( 'NONE',  ( -5.300029851643866863, 4.752152409900321395, -2.500000000000000444 ) ) ;
#134248=CARTESIAN_POINT ( 'NONE',  ( 5.142555292688428814, 7.778213139218437711, -1.168464917166486039 ) ) ;
#134249=CARTESIAN_POINT ( 'NONE',  ( -5.099275172071237705, 8.963255110809500437, 0.000000000000000000 ) ) ;
#134250=CARTESIAN_POINT ( 'NONE',  ( 3.580761967785000888, 7.191656372475549119, -0.7216878364870338292 ) ) ;
#134258=EDGE_CURVE ( 'NONE', #193413, #2249, #95651, .T. ) ;
#134270=CARTESIAN_POINT ( 'NONE',  ( -3.648552735408990166, 6.310376387068841630, -1.082531754730546636 ) ) ;
#134275=CARTESIAN_POINT ( 'NONE',  ( 6.204791576909545192, 7.267953590263130259, -1.199719254218452047 ) ) ;
#134276=ADVANCED_FACE ( 'NONE', ( #148691 ), #102554, .T. ) ;
#134304=CARTESIAN_POINT ( 'NONE',  ( 6.424584688029230328, 8.588711117491191871, 1.599625672291268286 ) ) ;
#134309=CARTESIAN_POINT ( 'NONE',  ( -5.244114872543307548, 7.700386654371578210, 1.209007019071134170 ) ) ;
#134310=CARTESIAN_POINT ( 'NONE',  ( 6.770317605177710085, 8.992066187497757213, 1.599625672291268286 ) ) ;
#134321=CARTESIAN_POINT ( 'NONE',  ( 1.812896364438529417, 2.514517768406685061, 2.499891510452758592 ) ) ;
#134330=DIRECTION ( 'NONE',  ( 0.000000000000000000, 1.000000000000000000, 0.000000000000000000 ) ) ;
#134337=CARTESIAN_POINT ( 'NONE',  ( 3.851925040058331806, 5.587274861525073355, -1.443375672974066548 ) ) ;
#134342=CARTESIAN_POINT ( 'NONE',  ( -6.851666526859749418, 9.086973262793417661, -1.599625672291271394 ) ) ;
#134344=CARTESIAN_POINT ( 'NONE',  ( 6.119526231721748033, 8.232809585132461194, 1.599625672291269396 ) ) ;
#134354=DIRECTION ( 'NONE',  ( 0.000000000000000000, 0.000000000000000000, -1.000000000000000000 ) ) ;
#134359=CARTESIAN_POINT ( 'NONE',  ( -5.019912524233729911, 4.821262464552921401, 0.2549627792466685472 ) ) ;
#134368=ADVANCED_FACE ( 'NONE', ( #4526 ), #185435, .T. ) ;
#134369=CARTESIAN_POINT ( 'NONE',  ( 7.842465510862060896, 8.114240948952696542, 0.000000000000000000 ) ) ;
#134378=CARTESIAN_POINT ( 'NONE',  ( 7.404161286838808920, 8.771181268467660885, -1.082531754730548412 ) ) ;
#134381=DIRECTION ( 'NONE',  ( 0.6507913734559627184, -0.7592566023653016805, 0.000000000000000000 ) ) ;
#134391=CARTESIAN_POINT ( 'NONE',  ( -4.773879485787619892, 7.623257595843924150, 1.082531754730549967 ) ) ;
#134393=CARTESIAN_POINT ( 'NONE',  ( 6.170896192875352959, 7.228408975556602556, 1.199719254218453823 ) ) ;
#134396=CARTESIAN_POINT ( 'NONE',  ( -8.120407659942227241, 8.438506789546210030, 0.7998128361456341429 ) ) ;
#134399=CARTESIAN_POINT ( 'NONE',  ( -2.830620210203090181, 6.524417021870718258, 0.000000000000000000 ) ) ;
#134401=CARTESIAN_POINT ( 'NONE',  ( 2.969872605471104876, 6.605953636086679737, -0.06813560672779371552 ) ) ;
#134409=CARTESIAN_POINT ( 'NONE',  ( 6.116136693540529912, 10.14959355252369910, 1.530808498934192557E-16 ) ) ;
#134411=CARTESIAN_POINT ( 'NONE',  ( -3.469446951953614189E-15, 8.999999999999998224, -0.7749999999999996891 ) ) ;
#134432=B_SPLINE_CURVE_WITH_KNOTS ( 'NONE', 3,
 ( #85786, #120502, #199513, #51158, #103107, #104181, #69508 ),
 .UNSPECIFIED., .F., .F.,
 ( 4, 3, 4 ),
 ( 6.824963372777353392E-15, 6.253410770929631051E-05, 0.0001562177157599490304 ),
 .UNSPECIFIED. ) ;
#134439=CARTESIAN_POINT ( 'NONE',  ( 4.963693636378940788, 5.923969009597785274, -1.082531754730548412 ) ) ;
#134444=CARTESIAN_POINT ( 'NONE',  ( 4.146814880933355596, 5.931313009212638931, 1.599625672291261402 ) ) ;
#134447=CARTESIAN_POINT ( 'NONE',  ( -6.147696309153835692, 6.137010213626392208, 0.7998128361456281477 ) ) ;
#134451=CARTESIAN_POINT ( 'NONE',  ( -4.950135482320918712, 7.828889591799445213, -1.082531754730549967 ) ) ;
#134452=LINE ( 'NONE', #200455, #87403 ) ;
#134456=ORIENTED_EDGE ( 'NONE', *, *, #129048, .T. ) ;
#134457=CARTESIAN_POINT ( 'NONE',  ( -7.286581212701773502, 7.465709267765667789, 0.7998128361456341429 ) ) ;
#134461=VERTEX_POINT ( 'NONE', #200604 ) ;
#134463=CARTESIAN_POINT ( 'NONE',  ( 4.754910920499133553, 4.886969541830044506, -0.7851691560945832649 ) ) ;
#134466=CARTESIAN_POINT ( 'NONE',  ( -4.457598643843001973, 8.422558527783969851, 0.000000000000000000 ) ) ;
#134467=ORIENTED_EDGE ( 'NONE', *, *, #49896, .T. ) ;
#134468=CARTESIAN_POINT ( 'NONE',  ( 4.602896574056089207, 8.480248385054199645, 0.1803159889683242367 ) ) ;
#134473=CARTESIAN_POINT ( 'NONE',  ( 6.180537922983273091, 8.303989891604203422, -1.599625672291281386 ) ) ;
#134480=CARTESIAN_POINT ( 'NONE',  ( -4.655245641445871385, 6.524482229810530498, 1.599625672291263179 ) ) ;
#134485=CARTESIAN_POINT ( 'NONE',  ( -6.720001414228860881, 7.869031733802326123, -1.199719254218452047 ) ) ;
#134489=CARTESIAN_POINT ( 'NONE',  ( 8.136301581532414673, 8.664975731308866003, 0.000000000000000000 ) ) ;
#134491=CARTESIAN_POINT ( 'NONE',  ( -7.715998819508785189, 8.174622508947939181, -0.7216878364870338292 ) ) ;
#134498=CARTESIAN_POINT ( 'NONE',  ( 4.830447868218803897, 8.857549289555754157, -0.7998128361456481317 ) ) ;
#134510=CARTESIAN_POINT ( 'NONE',  ( 6.505076094845553492, 6.832456077006010098, -0.5564590407885674495 ) ) ;
#134523=VERTEX_POINT ( 'NONE', #86884 ) ;
#134529=CARTESIAN_POINT ( 'NONE',  ( 3.933273961740297864, 7.602920365423412541, 0.7216878364870341622 ) ) ;
#134532=ORIENTED_EDGE ( 'NONE', *, *, #144165, .T. ) ;
#134536=CARTESIAN_POINT ( 'NONE',  ( -6.606676129765223671, 6.763588582595081000, -0.1820296311667093936 ) ) ;
#134557=CARTESIAN_POINT ( 'NONE',  ( -5.224688093219839402, 7.188831756880171397, -1.599625672291271394 ) ) ;
#134573=CARTESIAN_POINT ( 'NONE',  ( 7.018280793729500644, 8.217024343219755167, -1.199719254218452047 ) ) ;
#134576=CARTESIAN_POINT ( 'NONE',  ( 5.506019780481205217, 9.437790487287811558, 0.000000000000000000 ) ) ;
#134590=CARTESIAN_POINT ( 'NONE',  ( -6.459533842268148973, 6.500820668926428958, 0.000000000000000000 ) ) ;
#134591=CARTESIAN_POINT ( 'NONE',  ( 5.662465432362883355, 6.635239754958710989, 1.199719254218451159 ) ) ;
#134599=ORIENTED_EDGE ( 'NONE', *, *, #72719, .F. ) ;
#134600=CARTESIAN_POINT ( 'NONE',  ( -7.533490631048818109, 8.818102486758951031, -1.199719254218452047 ) ) ;
#134601=CARTESIAN_POINT ( 'NONE',  ( 4.167152111353856547, 5.955039778036558040, 1.599625672291262513 ) ) ;
#134607=CARTESIAN_POINT ( 'NONE',  ( 4.362691568547328202, 8.311833606605697256, -0.7998128361456381397 ) ) ;
#134613=CARTESIAN_POINT ( 'NONE',  ( -4.866517195131829787, 8.171732932056599452, 0.9908671576431731243 ) ) ;
#134615=B_SPLINE_CURVE_WITH_KNOTS ( 'NONE', 3,
 ( #66452, #101108, #169320, #148809, #102188, #99001, #136832, #165056, #51310, #168255 ),
 .UNSPECIFIED., .F., .F.,
 ( 4, 2, 2, 2, 4 ),
 ( 0.1967386737735414559, 0.2725667127094347775, 0.3483947516453281268, 0.4242227905812214206, 0.5000508295171147699 ),
 .UNSPECIFIED. ) ;
#134623=CARTESIAN_POINT ( 'NONE',  ( -5.759181390754928742, 9.941071732514568993, 0.000000000000000000 ) ) ;
#134624=CIRCLE ( 'NONE', #165194, 0.08000000000000025147 ) ;
#134627=CARTESIAN_POINT ( 'NONE',  ( -2.728371075039041305, 2.952267909019561376, 2.500000000000000444 ) ) ;
#134632=CARTESIAN_POINT ( 'NONE',  ( 3.553645660557675612, 6.199651466408984568, -1.082531754730549967 ) ) ;
#134653=( BOUNDED_SURFACE ( )  B_SPLINE_SURFACE ( 1, 2, ( 
 ( #88689, #70260, #7401, #169916, #73482, #87611, #123406, #90829, #5251, #203459, #71327, #22583, #170984, #137442, #172067, #139582, #154749, #152604, #187232, #120182, #205609, #206680, #20456, #121259, #38861, #6333, #72405, #122339, #189370, #138505, #188296, #74566, #41013, #39936, #107122, #173145, #156891, #8479, #140665, #58312, #124467, #174222, #27941, #44209, #175277, #109269, #210937, #75631, #96168, #43157, #13806, #112455, #26864, #11677, #125530, #25797, #193631, #128726, #129795, #63639, #159013, #94036, #9555, #10607, #62563, #76683, #194698, #209866, #178467, #79877, #160075, #177398, #29011, #30077, #191488, #77752, #141740, #211999, #143873, #176334, #61504, #161146, #142799, #208804, #92968, #60433, #157963, #126593, #192554, #110331, #127670, #45273, #111394, #95098, #195774, #12733, #47413, #78807, #91906, #46340, #207746, #145988, #144931, #59372, #162219, #151296, #179534, #85210, #83067, #114591, #200014, #2867, #164338, #166465, #48474, #18058, #67859, #725, #165393, #181632, #97226, #34322, #130840, #182703, #64695, #1802, #117788, #180582, #82009, #32203, #115636, #197887, #196833, #50581, #100396, #33261, #31153, #65731, #163279, #84145, #68937, #201071, #135059, #113527, #98279, #99344, #66791, #150231, #15926, #49516, #167535, #134008, #14863, #80952, #148099, #51665, #183777, #35388, #101464, #19133, #147043, #213066, #214102, #131878, #16989, #149145, #132930, #198936, #116703, #188039, #121006, #143349, #21249, #119921, #103608, #87356, #169664, #36458, #4993, #3930, #6074, #24464, #38605, #52713, #153424, #202129, #168596, #204266, #71070, #7145, #118846, #20196, #137187, #185896, #70000, #184828, #205354, #203209, #102534, #186973, #39668, #89509, #77230, #54855, #53790, #106862, #22318, #105779, #171804, #104683, #86284, #37531, #170732, #23396, #88431, #155563, #154495, #72144, #11153, #152355, #136114, #55919, #138254, #122077, #73217, #139323, #56988, #123161, #189121, #40756, #172889, #90577, #156637, #115139, #97780, #32755, #12226, #209344, #113015, #163840, #213606 ),
 ( #94582, #181135, #210426, #176879, #44766, #80443, #146544, #114091, #28491, #15419, #164887, #46901, #49020, #45830, #31705, #29567, #60992, #194186, #145494, #79375, #63126, #98837, #212562, #180082, #95659, #160625, #96726, #78299, #16481, #62068, #64201, #81509, #161710, #144424, #147588, #65233, #131383, #110874, #195266, #197379, #111951, #128223, #177953, #13302, #129290, #211489, #179024, #30642, #82562, #162775, #127145, #14353, #193118, #130342, #196331, #47975, #199497, #38092, #34867, #186455, #214, #120483, #118333, #149711, #20741, #104163, #51141, #201620, #83628, #53269, #103090, #35943, #200560, #2352, #132432, #69492, #165955, #3425, #99894, #37008, #152901, #1291, #117265, #67349, #150789, #18623, #17539, #85768, #135599, #68428, #66285, #100941, #198433, #119400, #170211, #21796, #148648, #50079, #133494, #134557, #102022, #185389, #183263, #116200, #182187, #169148, #33815, #167028, #84702, #86836, #4479, #70550, #136669, #54344, #202694, #52207, #184318, #168091, #19690, #151849, #92205, #41312, #205907, #87904, #156115, #172361, #88988, #22872, #124758, #203758, #9844, #171280, #142022, #26090, #155041, #139876, #39157, #153977, #107419, #42380, #43440, #191784, #72706, #7697, #137738, #138801, #190718, #204821, #108490, #123699, #158255, #208037, #73780, #91123, #157182, #75919, #105240, #57542, #55401, #125823, #189660, #90055, #173444, #74860, #56472, #122634, #6627, #188597, #71625, #109564, #175568, #40228, #25023, #121555, #106339, #174514, #23951, #59664, #8777, #5544, #187526, #140963, #206973, #58604, #31442, #192847, #95399, #76971, #64977, #211231, #29305, #161451, #14086, #78046, #144170, #44506, #210162, #10896, #94328, #160370, #110623, #13031, #28235, #11972, #61803, #197121, #127972, #131132, #193924, #48760, #63927, #114872, #147328, #45571, #27159, #111687, #93264, #159297, #213356, #62856, #177694, #113824, #143098, #79108, #80177, #176624, #146282, #196077, #129021, #145226, #194997, #209091, #162514, #46631, #96465, #112754, #130082, #97521, #178766, #30379, #212295 ) ),
 .UNSPECIFIED., .F., .F., .T. ) 
 B_SPLINE_SURFACE_WITH_KNOTS ( ( 2, 2 ),
 ( 3, 2, 2, 2, 2, 2, 2, 2, 2, 2, 2, 2, 2, 2, 2, 2, 2, 2, 2, 2, 2, 2, 2, 2, 2, 2, 2, 2, 2, 2, 2, 2, 2, 2, 2, 2, 2, 2, 2, 2, 2, 2, 2, 2, 2, 2, 2, 2, 2, 2, 2, 2, 2, 2, 2, 2, 2, 2, 2, 2, 2, 2, 2, 2, 2, 2, 2, 2, 2, 2, 2, 2, 2, 2, 2, 2, 2, 2, 2, 2, 2, 2, 2, 2, 2, 2, 2, 2, 2, 2, 2, 2, 2, 2, 2, 2, 2, 2, 2, 2, 2, 2, 2, 2, 2, 2, 2, 2, 2, 2, 2, 2, 2, 2, 2, 2, 2, 2, 2, 2, 3 ),
 ( 0.000000000000000000, 1.000000000000000000 ),
 ( 0.000000000000000000, 0.008333333333333333218, 0.01666666666666666644, 0.02500000000000000139, 0.03333333333333333287, 0.04166666666666666435, 0.05000000000000000278, 0.05833333333333333426, 0.06666666666666666574, 0.07499999999999999722, 0.08333333333333332871, 0.09166666666666666019, 0.1000000000000000056, 0.1083333333333333370, 0.1166666666666666685, 0.1250000000000000000, 0.1333333333333333315, 0.1416666666666666630, 0.1499999999999999944, 0.1583333333333333259, 0.1666666666666666574, 0.1749999999999999889, 0.1833333333333333204, 0.1916666666666666796, 0.2000000000000000111, 0.2083333333333333426, 0.2166666666666666741, 0.2250000000000000056, 0.2333333333333333370, 0.2416666666666666685, 0.2500000000000000000, 0.2583333333333333592, 0.2666666666666666630, 0.2750000000000000222, 0.2833333333333333259, 0.2916666666666666852, 0.2999999999999999889, 0.3083333333333333481, 0.3166666666666666519, 0.3250000000000000111, 0.3333333333333333148, 0.3416666666666666741, 0.3499999999999999778, 0.3583333333333333370, 0.3666666666666666408, 0.3750000000000000000, 0.3833333333333333592, 0.3916666666666666630, 0.4000000000000000222, 0.4083333333333333259, 0.4166666666666666852, 0.4249999999999999889, 0.4333333333333333481, 0.4416666666666666519, 0.4500000000000000111, 0.4583333333333333148, 0.4666666666666666741, 0.4749999999999999778, 0.4833333333333333370, 0.4916666666666666408, 0.5000000000000000000, 0.5083333333333333037, 0.5166666666666667185, 0.5250000000000000222, 0.5333333333333333259, 0.5416666666666666297, 0.5500000000000000444, 0.5583333333333333481, 0.5666666666666666519, 0.5749999999999999556, 0.5833333333333333703, 0.5916666666666666741, 0.5999999999999999778, 0.6083333333333332815, 0.6166666666666666963, 0.6250000000000000000, 0.6333333333333333037, 0.6416666666666667185, 0.6500000000000000222, 0.6583333333333333259, 0.6666666666666666297, 0.6750000000000000444, 0.6833333333333333481, 0.6916666666666666519, 0.6999999999999999556, 0.7083333333333333703, 0.7166666666666666741, 0.7249999999999999778, 0.7333333333333332815, 0.7416666666666666963, 0.7500000000000000000, 0.7583333333333333037, 0.7666666666666667185, 0.7750000000000000222, 0.7833333333333333259, 0.7916666666666666297, 0.8000000000000000444, 0.8083333333333333481, 0.8166666666666666519, 0.8249999999999999556, 0.8333333333333333703, 0.8416666666666666741, 0.8499999999999999778, 0.8583333333333332815, 0.8666666666666666963, 0.8750000000000000000, 0.8833333333333333037, 0.8916666666666667185, 0.9000000000000000222, 0.9083333333333333259, 0.9166666666666666297, 0.9250000000000000444, 0.9333333333333333481, 0.9416666666666666519, 0.9499999999999999556, 0.9583333333333333703, 0.9666666666666666741, 0.9749999999999999778, 0.9833333333333332815, 0.9916666666666666963, 1.000000000000000000 ),
 .UNSPECIFIED. ) 
 GEOMETRIC_REPRESENTATION_ITEM ( )  RATIONAL_B_SPLINE_SURFACE ( (
 ( 1.000000000000000000, 0.8660254037844387076, 1.000000000000000000, 0.8660254037844387076, 1.000000000000000000, 0.8660254037844387076, 1.000000000000000000, 0.8660254037844387076, 1.000000000000000000, 0.8660254037844387076, 1.000000000000000000, 0.8660254037844387076, 1.000000000000000000, 0.8660254037844387076, 1.000000000000000000, 0.8660254037844387076, 1.000000000000000000, 0.8660254037844387076, 1.000000000000000000, 0.8660254037844387076, 1.000000000000000000, 0.8660254037844387076, 1.000000000000000000, 0.8660254037844387076, 1.000000000000000000, 0.8660254037844387076, 1.000000000000000000, 0.8660254037844387076, 1.000000000000000000, 0.8660254037844387076, 1.000000000000000000, 0.8660254037844387076, 1.000000000000000000, 0.8660254037844387076, 1.000000000000000000, 0.8660254037844387076, 1.000000000000000000, 0.8660254037844387076, 1.000000000000000000, 0.8660254037844387076, 1.000000000000000000, 0.8660254037844387076, 1.000000000000000000, 0.8660254037844387076, 1.000000000000000000, 0.8660254037844387076, 1.000000000000000000, 0.8660254037844387076, 1.000000000000000000, 0.8660254037844387076, 1.000000000000000000, 0.8660254037844387076, 1.000000000000000000, 0.8660254037844387076, 1.000000000000000000, 0.8660254037844387076, 1.000000000000000000, 0.8660254037844387076, 1.000000000000000000, 0.8660254037844387076, 1.000000000000000000, 0.8660254037844387076, 1.000000000000000000, 0.8660254037844387076, 1.000000000000000000, 0.8660254037844387076, 1.000000000000000000, 0.8660254037844387076, 1.000000000000000000, 0.8660254037844387076, 1.000000000000000000, 0.8660254037844387076, 1.000000000000000000, 0.8660254037844387076, 1.000000000000000000, 0.8660254037844387076, 1.000000000000000000, 0.8660254037844387076, 1.000000000000000000, 0.8660254037844387076, 1.000000000000000000, 0.8660254037844387076, 1.000000000000000000, 0.8660254037844387076, 1.000000000000000000, 0.8660254037844387076, 1.000000000000000000, 0.8660254037844387076, 1.000000000000000000, 0.8660254037844387076, 1.000000000000000000, 0.8660254037844387076, 1.000000000000000000, 0.8660254037844387076, 1.000000000000000000, 0.8660254037844387076, 1.000000000000000000, 0.8660254037844387076, 1.000000000000000000, 0.8660254037844387076, 1.000000000000000000, 0.8660254037844387076, 1.000000000000000000, 0.8660254037844387076, 1.000000000000000000, 0.8660254037844387076, 1.000000000000000000, 0.8660254037844387076, 1.000000000000000000, 0.8660254037844387076, 1.000000000000000000, 0.8660254037844387076, 1.000000000000000000, 0.8660254037844387076, 1.000000000000000000, 0.8660254037844387076, 1.000000000000000000, 0.8660254037844387076, 1.000000000000000000, 0.8660254037844387076, 1.000000000000000000, 0.8660254037844387076, 1.000000000000000000, 0.8660254037844387076, 1.000000000000000000, 0.8660254037844387076, 1.000000000000000000, 0.8660254037844387076, 1.000000000000000000, 0.8660254037844387076, 1.000000000000000000, 0.8660254037844387076, 1.000000000000000000, 0.8660254037844387076, 1.000000000000000000, 0.8660254037844387076, 1.000000000000000000, 0.8660254037844387076, 1.000000000000000000, 0.8660254037844387076, 1.000000000000000000, 0.8660254037844387076, 1.000000000000000000, 0.8660254037844387076, 1.000000000000000000, 0.8660254037844387076, 1.000000000000000000, 0.8660254037844387076, 1.000000000000000000, 0.8660254037844387076, 1.000000000000000000, 0.8660254037844387076, 1.000000000000000000, 0.8660254037844387076, 1.000000000000000000, 0.8660254037844387076, 1.000000000000000000, 0.8660254037844387076, 1.000000000000000000, 0.8660254037844387076, 1.000000000000000000, 0.8660254037844387076, 1.000000000000000000, 0.8660254037844387076, 1.000000000000000000, 0.8660254037844387076, 1.000000000000000000, 0.8660254037844387076, 1.000000000000000000, 0.8660254037844387076, 1.000000000000000000, 0.8660254037844387076, 1.000000000000000000, 0.8660254037844387076, 1.000000000000000000, 0.8660254037844387076, 1.000000000000000000, 0.8660254037844387076, 1.000000000000000000, 0.8660254037844387076, 1.000000000000000000, 0.8660254037844387076, 1.000000000000000000, 0.8660254037844387076, 1.000000000000000000, 0.8660254037844387076, 1.000000000000000000, 0.8660254037844387076, 1.000000000000000000, 0.8660254037844387076, 1.000000000000000000, 0.8660254037844387076, 1.000000000000000000, 0.8660254037844387076, 1.000000000000000000, 0.8660254037844387076, 1.000000000000000000, 0.8660254037844387076, 1.000000000000000000, 0.8660254037844387076, 1.000000000000000000, 0.8660254037844387076, 1.000000000000000000, 0.8660254037844387076, 1.000000000000000000, 0.8660254037844387076, 1.000000000000000000, 0.8660254037844387076, 1.000000000000000000, 0.8660254037844387076, 1.000000000000000000, 0.8660254037844387076, 1.000000000000000000, 0.8660254037844387076, 1.000000000000000000, 0.8660254037844387076, 1.000000000000000000, 0.8660254037844387076, 1.000000000000000000, 0.8660254037844387076, 1.000000000000000000, 0.8660254037844387076, 1.000000000000000000, 0.8660254037844387076, 1.000000000000000000, 0.8660254037844387076, 1.000000000000000000, 0.8660254037844387076, 1.000000000000000000, 0.8660254037844387076, 1.000000000000000000, 0.8660254037844387076, 1.000000000000000000, 0.8660254037844387076, 1.000000000000000000, 0.8660254037844387076, 1.000000000000000000, 0.8660254037844387076, 1.000000000000000000, 0.8660254037844387076, 1.000000000000000000),
 ( 1.000000000000000000, 0.8660254037844387076, 1.000000000000000000, 0.8660254037844387076, 1.000000000000000000, 0.8660254037844387076, 1.000000000000000000, 0.8660254037844387076, 1.000000000000000000, 0.8660254037844387076, 1.000000000000000000, 0.8660254037844387076, 1.000000000000000000, 0.8660254037844387076, 1.000000000000000000, 0.8660254037844387076, 1.000000000000000000, 0.8660254037844387076, 1.000000000000000000, 0.8660254037844387076, 1.000000000000000000, 0.8660254037844387076, 1.000000000000000000, 0.8660254037844387076, 1.000000000000000000, 0.8660254037844387076, 1.000000000000000000, 0.8660254037844387076, 1.000000000000000000, 0.8660254037844387076, 1.000000000000000000, 0.8660254037844387076, 1.000000000000000000, 0.8660254037844387076, 1.000000000000000000, 0.8660254037844387076, 1.000000000000000000, 0.8660254037844387076, 1.000000000000000000, 0.8660254037844387076, 1.000000000000000000, 0.8660254037844387076, 1.000000000000000000, 0.8660254037844387076, 1.000000000000000000, 0.8660254037844387076, 1.000000000000000000, 0.8660254037844387076, 1.000000000000000000, 0.8660254037844387076, 1.000000000000000000, 0.8660254037844387076, 1.000000000000000000, 0.8660254037844387076, 1.000000000000000000, 0.8660254037844387076, 1.000000000000000000, 0.8660254037844387076, 1.000000000000000000, 0.8660254037844387076, 1.000000000000000000, 0.8660254037844387076, 1.000000000000000000, 0.8660254037844387076, 1.000000000000000000, 0.8660254037844387076, 1.000000000000000000, 0.8660254037844387076, 1.000000000000000000, 0.8660254037844387076, 1.000000000000000000, 0.8660254037844387076, 1.000000000000000000, 0.8660254037844387076, 1.000000000000000000, 0.8660254037844387076, 1.000000000000000000, 0.8660254037844387076, 1.000000000000000000, 0.8660254037844387076, 1.000000000000000000, 0.8660254037844387076, 1.000000000000000000, 0.8660254037844387076, 1.000000000000000000, 0.8660254037844387076, 1.000000000000000000, 0.8660254037844387076, 1.000000000000000000, 0.8660254037844387076, 1.000000000000000000, 0.8660254037844387076, 1.000000000000000000, 0.8660254037844387076, 1.000000000000000000, 0.8660254037844387076, 1.000000000000000000, 0.8660254037844387076, 1.000000000000000000, 0.8660254037844387076, 1.000000000000000000, 0.8660254037844387076, 1.000000000000000000, 0.8660254037844387076, 1.000000000000000000, 0.8660254037844387076, 1.000000000000000000, 0.8660254037844387076, 1.000000000000000000, 0.8660254037844387076, 1.000000000000000000, 0.8660254037844387076, 1.000000000000000000, 0.8660254037844387076, 1.000000000000000000, 0.8660254037844387076, 1.000000000000000000, 0.8660254037844387076, 1.000000000000000000, 0.8660254037844387076, 1.000000000000000000, 0.8660254037844387076, 1.000000000000000000, 0.8660254037844387076, 1.000000000000000000, 0.8660254037844387076, 1.000000000000000000, 0.8660254037844387076, 1.000000000000000000, 0.8660254037844387076, 1.000000000000000000, 0.8660254037844387076, 1.000000000000000000, 0.8660254037844387076, 1.000000000000000000, 0.8660254037844387076, 1.000000000000000000, 0.8660254037844387076, 1.000000000000000000, 0.8660254037844387076, 1.000000000000000000, 0.8660254037844387076, 1.000000000000000000, 0.8660254037844387076, 1.000000000000000000, 0.8660254037844387076, 1.000000000000000000, 0.8660254037844387076, 1.000000000000000000, 0.8660254037844387076, 1.000000000000000000, 0.8660254037844387076, 1.000000000000000000, 0.8660254037844387076, 1.000000000000000000, 0.8660254037844387076, 1.000000000000000000, 0.8660254037844387076, 1.000000000000000000, 0.8660254037844387076, 1.000000000000000000, 0.8660254037844387076, 1.000000000000000000, 0.8660254037844387076, 1.000000000000000000, 0.8660254037844387076, 1.000000000000000000, 0.8660254037844387076, 1.000000000000000000, 0.8660254037844387076, 1.000000000000000000, 0.8660254037844387076, 1.000000000000000000, 0.8660254037844387076, 1.000000000000000000, 0.8660254037844387076, 1.000000000000000000, 0.8660254037844387076, 1.000000000000000000, 0.8660254037844387076, 1.000000000000000000, 0.8660254037844387076, 1.000000000000000000, 0.8660254037844387076, 1.000000000000000000, 0.8660254037844387076, 1.000000000000000000, 0.8660254037844387076, 1.000000000000000000, 0.8660254037844387076, 1.000000000000000000, 0.8660254037844387076, 1.000000000000000000, 0.8660254037844387076, 1.000000000000000000, 0.8660254037844387076, 1.000000000000000000, 0.8660254037844387076, 1.000000000000000000, 0.8660254037844387076, 1.000000000000000000, 0.8660254037844387076, 1.000000000000000000, 0.8660254037844387076, 1.000000000000000000, 0.8660254037844387076, 1.000000000000000000, 0.8660254037844387076, 1.000000000000000000, 0.8660254037844387076, 1.000000000000000000, 0.8660254037844387076, 1.000000000000000000, 0.8660254037844387076, 1.000000000000000000, 0.8660254037844387076, 1.000000000000000000, 0.8660254037844387076, 1.000000000000000000, 0.8660254037844387076, 1.000000000000000000, 0.8660254037844387076, 1.000000000000000000, 0.8660254037844387076, 1.000000000000000000, 0.8660254037844387076, 1.000000000000000000, 0.8660254037844387076, 1.000000000000000000, 0.8660254037844387076, 1.000000000000000000, 0.8660254037844387076, 1.000000000000000000, 0.8660254037844387076, 1.000000000000000000, 0.8660254037844387076, 1.000000000000000000, 0.8660254037844387076, 1.000000000000000000, 0.8660254037844387076, 1.000000000000000000) ) ) 
 REPRESENTATION_ITEM ( '' )  SURFACE ( )  );
#134662=ORIENTED_EDGE ( 'NONE', *, *, #99445, .F. ) ;
#134674=CARTESIAN_POINT ( 'NONE',  ( 4.553559489343365740, 6.405848385690952718, -1.599625672291269396 ) ) ;
#134675=CARTESIAN_POINT ( 'NONE',  ( -4.177320726786319049, 6.927272377009067839, -1.082531754730551743 ) ) ;
#134698=CARTESIAN_POINT ( 'NONE',  ( -6.981522756394290319, 7.109807735406931783, 0.7998128361456341429 ) ) ;
#134707=CARTESIAN_POINT ( 'NONE',  ( 2.907633421442281207, 6.614265768316455407, -0.2557691087421434251 ) ) ;
#134710=CARTESIAN_POINT ( 'NONE',  ( -6.774234028683526532, 7.932303117332766718, 1.199719254218452047 ) ) ;
#134718=CARTESIAN_POINT ( 'NONE',  ( 5.090160327287878594, 4.903218234782778850, -0.7998128361456481317 ) ) ;
#134723=CARTESIAN_POINT ( 'NONE',  ( -6.784929528996132220, 6.880448970109080520, 0.000000000000000000 ) ) ;
#134726=CARTESIAN_POINT ( 'NONE',  ( -5.478903473698241378, 9.406154796041011679, -0.7216878364870338292 ) ) ;
#134730=CARTESIAN_POINT ( 'NONE',  ( 4.624739795592929248, 6.488892076315451618, -1.443375672974068769 ) ) ;
#134731=CARTESIAN_POINT ( 'NONE',  ( -4.950135482320929370, 5.908151163196758482, -1.082531754730549967 ) ) ;
#134736=EDGE_CURVE ( 'NONE', #210733, #123356, #49296, .T. ) ;
#134749=CARTESIAN_POINT ( 'NONE',  ( 6.440439394220377700, 6.875545743132385645, 0.7017714770480776298 ) ) ;
#134756=CARTESIAN_POINT ( 'NONE',  ( 5.704082950214642622, 7.400961370687027419, -1.366768684276008283 ) ) ;
#134769=CARTESIAN_POINT ( 'NONE',  ( 5.969043672405669909, 7.102642550806028687, -1.084880274121432064 ) ) ;
#134785=CARTESIAN_POINT ( 'NONE',  ( 6.526270840131753737, 8.707344961610770540, -1.599625672291283607 ) ) ;
#134788=CARTESIAN_POINT ( 'NONE',  ( -7.144220599758281054, 7.299621885998258897, 0.7998128361456341429 ) ) ;
#134800=CARTESIAN_POINT ( 'NONE',  ( 5.550083779947807550, 7.568460058062819407, -1.599625672291283607 ) ) ;
#134802=CARTESIAN_POINT ( 'NONE',  ( 5.982890925380405456, 10.20206618957764100, 0.000000000000000000 ) ) ;
#134808=CARTESIAN_POINT ( 'NONE',  ( -6.089020385868856522, 9.157588645938716354, -1.082531754730549967 ) ) ;
#134813=CARTESIAN_POINT ( 'NONE',  ( 7.309781096423290769, 8.557108029695882578, 1.199719254218452935 ) ) ;
#134826=CARTESIAN_POINT ( 'NONE',  ( -5.126391479742927970, 8.994890803093138487, 0.7216878364870267237 ) ) ;
#134827=CARTESIAN_POINT ( 'NONE',  ( 6.712695452541852070, 7.004101914153185504, 0.000000000000000000 ) ) ;
#134833=ORIENTED_EDGE ( 'NONE', *, *, #43875, .T. ) ;
#134834=DIRECTION ( 'NONE',  ( 0.6507913734559640506, -0.7592566023653003482, 0.000000000000000000 ) ) ;
#134838=CARTESIAN_POINT ( 'NONE',  ( -5.808742468812186033, 5.741564066561132940, 0.000000000000000000 ) ) ;
#134839=CARTESIAN_POINT ( 'NONE',  ( -3.149236820124241110, 6.896136400112061970, -0.7998128361456481317 ) ) ;
#134842=CARTESIAN_POINT ( 'NONE',  ( 3.892599500454932304, 7.555466827257172113, 0.7216878364870257245 ) ) ;
#134854=CARTESIAN_POINT ( 'NONE',  ( -6.184982820901517186, 6.966600618058066630, 0.8941503475990535410 ) ) ;
#134858=CARTESIAN_POINT ( 'NONE',  ( -4.398886013728402489, 7.974527572605470738, 0.5967842075597221685 ) ) ;
#134859=CARTESIAN_POINT ( 'NONE',  ( 4.258669648468281110, 6.061810238003387141, 1.443375672974058777 ) ) ;
#134863=CARTESIAN_POINT ( 'NONE',  ( -6.143779885648060102, 7.196773283791382703, 1.199719254218452047 ) ) ;
#134875=CARTESIAN_POINT ( 'NONE',  ( 5.415556014015861841, 5.282846535965431300, -0.7998128361456481317 ) ) ;
#134910=CARTESIAN_POINT ( 'NONE',  ( 5.804299160426222848, 7.865044668620976509, -1.443375672974078761 ) ) ;
#134916=CARTESIAN_POINT ( 'NONE',  ( 5.004368096775565711, 8.852530189631227842, -0.7216878364870458196 ) ) ;
#134932=CARTESIAN_POINT ( 'NONE',  ( -6.420668264523499147, 9.648474187656182366, 1.199719254218452935 ) ) ;
#134940=CARTESIAN_POINT ( 'NONE',  ( -5.178288325776719603, 5.006034233019745372, 0.000000000000000000 ) ) ;
#134942=CARTESIAN_POINT ( 'NONE',  ( 3.567203813726949058, 7.175838526074521440, 0.7216878364870257245 ) ) ;
#134948=CARTESIAN_POINT ( 'NONE',  ( -6.237633190739009237, 9.434933268240943249, 1.199719254218452047 ) ) ;
#134953=CARTESIAN_POINT ( 'NONE',  ( -6.319508997745553636, 6.545384383557486530, 0.7216878364870257245 ) ) ;
#134956=CARTESIAN_POINT ( 'NONE',  ( -5.803772275101700906, 8.928762199997411386, -1.199719254218452047 ) ) ;
#134964=CARTESIAN_POINT ( 'NONE',  ( 4.558697364098442506, 8.332581001507888274, -0.6286255394594755241 ) ) ;
#134976=CARTESIAN_POINT ( 'NONE',  ( -3.933273961740340496, 5.682181936820735579, 1.443375672974065660 ) ) ;
#134977=ORIENTED_EDGE ( 'NONE', *, *, #157268, .F. ) ;
#134978=CARTESIAN_POINT ( 'NONE',  ( -4.245111494410291897, 7.006361605903701495, 1.082531754730549967 ) ) ;
#134979=CARTESIAN_POINT ( 'NONE',  ( 5.910428620914669473, 5.860197910680708944, 0.000000000000000000 ) ) ;
#134980=CARTESIAN_POINT ( 'NONE',  ( -3.955946960137363799, 7.837298230127379917, 0.7998128361456352531 ) ) ;
#134981=CARTESIAN_POINT ( 'NONE',  ( -5.468734858265826837, 7.473552982767158070, 1.599625672291263179 ) ) ;
#135025=CARTESIAN_POINT ( 'NONE',  ( 2.992204144738932481, 6.423898490107104564, -0.5069251535329973857 ) ) ;
#135034=CARTESIAN_POINT ( 'NONE',  ( 5.248941747146098180, 6.152795455539095570, -1.199719254218452047 ) ) ;
#135048=CARTESIAN_POINT ( 'NONE',  ( 4.595929827128614420, 8.372548788374160722, -0.07784623617661419470 ) ) ;
#135051=CARTESIAN_POINT ( 'NONE',  ( 3.878514461961128479, 6.682628084666728085, -1.199719254218448494 ) ) ;
#135059=CARTESIAN_POINT ( 'NONE',  ( -5.261446130555064826, 8.296048364692991228, 1.199719254218452935 ) ) ;
#135071=CARTESIAN_POINT ( 'NONE',  ( 7.024532985656141371, 7.367912369453226695, 0.7216878364870328300 ) ) ;
#135074=CARTESIAN_POINT ( 'NONE',  ( -7.110325215724114578, 7.260077271291732082, 0.000000000000000000 ) ) ;
#135081=ORIENTED_EDGE ( 'NONE', *, *, #50358, .T. ) ;
#135085=CARTESIAN_POINT ( 'NONE',  ( 5.388439706788500594, 5.251210844200210559, 0.7998128361456352531 ) ) ;
#135086=CARTESIAN_POINT ( 'NONE',  ( 6.008198349511364000, 7.038594824965278995, 1.199719254218453823 ) ) ;
#135107=CARTESIAN_POINT ( 'NONE',  ( 3.147653791585776517, 8.920000000000001705, 2.419999999999890239 ) ) ;
#135109=DIRECTION ( 'NONE',  ( 0.000000000000000000, 0.000000000000000000, 1.000000000000000000 ) ) ;
#135112=CARTESIAN_POINT ( 'NONE',  ( 6.224601922449876312, 6.434659462379210382, 0.000000000000000000 ) ) ;
#135114=CARTESIAN_POINT ( 'NONE',  ( 2.911969131885072670, 6.619324097166378706, 0.000000000000000000 ) ) ;
#135119=CARTESIAN_POINT ( 'NONE',  ( 6.475954649182838807, 7.584310507915338562, 1.199719254218452047 ) ) ;
#135124=CARTESIAN_POINT ( 'NONE',  ( 4.095971805104276164, 7.792734516014745871, 0.7216878364870257245 ) ) ;
#135127=CARTESIAN_POINT ( 'NONE',  ( 5.090160327287878594, 4.903218234782778850, -0.7998128361456481317 ) ) ;
#135139=CARTESIAN_POINT ( 'NONE',  ( 6.474762296362193581, 6.758873339713582062, -0.2294044474360455721 ) ) ;
#135140=CARTESIAN_POINT ( 'NONE',  ( -7.132998214565509087, 7.494455136514109661, 0.7216878364870317197 ) ) ;
#135157=ORIENTED_EDGE ( 'NONE', *, *, #125035, .F. ) ;
#135176=CARTESIAN_POINT ( 'NONE',  ( 6.879836604291781121, 6.991173891287354003, -0.7998128361456341429 ) ) ;
#135177=CARTESIAN_POINT ( 'NONE',  ( -4.787437638956927977, 7.639075441208117212, -1.082531754730549967 ) ) ;
#135178=CARTESIAN_POINT ( 'NONE',  ( 6.230854113932139171, 9.427024345299638952, 1.199719254218452047 ) ) ;
#135192=CARTESIAN_POINT ( 'NONE',  ( -4.447956913735107598, 7.346977611736363656, 1.199719254218452935 ) ) ;
#135194=CARTESIAN_POINT ( 'NONE',  ( 7.309254211098767051, 7.700087132469628948, 0.7216878364870267237 ) ) ;
#135211=CARTESIAN_POINT ( 'NONE',  ( -7.458393901293492334, 7.874083437696761223, 0.7216878364870317197 ) ) ;
#135213=CARTESIAN_POINT ( 'NONE',  ( -6.794044374223859428, 7.099008989448849505, 0.000000000000000000 ) ) ;
#135237=CARTESIAN_POINT ( 'NONE',  ( -5.981082042284069367, 7.006959133200059142, 1.199719254218452935 ) ) ;
#135247=CARTESIAN_POINT ( 'NONE',  ( 5.351240958524983604, 4.712734197347588250, -2.500000000000000888 ) ) ;
#135248=CARTESIAN_POINT ( 'NONE',  ( -5.880564528862151974, 7.271459349814712425, -1.272365726499018246 ) ) ;
#135285=CARTESIAN_POINT ( 'NONE',  ( 4.844006021832467646, 8.873367135438366304, 0.000000000000000000 ) ) ;
#135286=CARTESIAN_POINT ( 'NONE',  ( 6.235824307642648279, 6.239826211863360506, 0.000000000000000000 ) ) ;
#135288=CARTESIAN_POINT ( 'NONE',  ( 4.206772801990143584, 8.129928378955675328, 0.7998128361456271485 ) ) ;
#135294=EDGE_CURVE ( 'NONE', #45181, #63797, #212344, .T. ) ;
#135301=CARTESIAN_POINT ( 'NONE',  ( 5.865087380380676230, 7.178575736046542310, -1.148900262672468475 ) ) ;
#135304=CARTESIAN_POINT ( 'NONE',  ( -5.763624699140882157, 7.817591130454727200, -1.443375672974066548 ) ) ;
#135305=CARTESIAN_POINT ( 'NONE',  ( 4.665414256878284149, 6.536345614481700927, -1.443375672974068769 ) ) ;
#135323=EDGE_CURVE ( 'NONE', #29771, #121694, #38463, .T. ) ;
#135324=CARTESIAN_POINT ( 'NONE',  ( -4.950135482320918712, 7.828889591799445213, -1.082531754730549967 ) ) ;
#135329=CARTESIAN_POINT ( 'NONE',  ( 4.857564175446106525, 8.889184981320973122, 0.7998128361456331437 ) ) ;
#135355=CARTESIAN_POINT ( 'NONE',  ( 7.452141709366786770, 8.723195411463290583, 1.199719254218452047 ) ) ;
#135360=TOROIDAL_SURFACE ( 'NONE', #131976, 2.080000000000000071, 0.08000000000000000167 ) ;
#135364=ORIENTED_EDGE ( 'NONE', *, *, #31576, .F. ) ;
#135367=CARTESIAN_POINT ( 'NONE',  ( -3.011287625495571607, 6.360174617139689346, -0.7852620323503290978 ) ) ;
#135382=CARTESIAN_POINT ( 'NONE',  ( 5.234856708652233515, 6.240325927249993576, 1.082531754730549078 ) ) ;
#135387=CARTESIAN_POINT ( 'NONE',  ( -7.442499979258930587, 7.647614495415686164, -0.7998128361456362523 ) ) ;
#135389=CARTESIAN_POINT ( 'NONE',  ( 7.849244587668864348, 8.122149871893999062, 0.7998128361456291469 ) ) ;
#135410=CARTESIAN_POINT ( 'NONE',  ( 6.587282531393223728, 8.778525268082516320, 1.599625672291268286 ) ) ;
#135420=CARTESIAN_POINT ( 'NONE',  ( 6.916067756746836714, 8.201738816693689316, -1.082531754730548412 ) ) ;
#135429=DIRECTION ( 'NONE',  ( -0.000000000000000000, 1.000000000000000000, -0.000000000000000000 ) ) ;
#135431=CARTESIAN_POINT ( 'NONE',  ( -4.651856103264620401, 8.441266197201775512, 0.000000000000000000 ) ) ;
#135434=CARTESIAN_POINT ( 'NONE',  ( 6.821687566331318564, 7.987665577921906568, 1.199719254218452935 ) ) ;
#135437=CARTESIAN_POINT ( 'NONE',  ( -6.474900878978163021, 9.711745571186627402, -1.199719254218452047 ) ) ;
#135440=CARTESIAN_POINT ( 'NONE',  ( -4.248501033035892327, 6.049946853332221153, -1.599625672291271394 ) ) ;
#135452=FACE_OUTER_BOUND ( 'NONE', #78837, .T. ) ;
#135468=VERTEX_POINT ( 'NONE', #19473 ) ;
#135481=CARTESIAN_POINT ( 'NONE',  ( 5.573810548993915148, 5.675402860013913475, 0.000000000000000000 ) ) ;
#135488=CARTESIAN_POINT ( 'NONE',  ( -4.339491684825780737, 7.220434844675483355, -1.199719254218455378 ) ) ;
#135492=CARTESIAN_POINT ( 'NONE',  ( -4.448483798615272100, 8.203998508444197313, 0.000000000000000000 ) ) ;
#135497=VERTEX_POINT ( 'NONE', #2138 ) ;
#135498=CARTESIAN_POINT ( 'NONE',  ( -6.424584688029276514, 8.588711117491191871, 1.599625672291269396 ) ) ;
#135504=CARTESIAN_POINT ( 'NONE',  ( 3.610856454189071751, 7.348000977992388272, 0.3914447831331854810 ) ) ;
#135506=CARTESIAN_POINT ( 'NONE',  ( -5.173318132066234476, 8.193232366456022930, -1.199719254218453823 ) ) ;
#135508=CARTESIAN_POINT ( 'NONE',  ( 4.648548116941726427, 8.423941524322412278, -0.4686463081053967583 ) ) ;
#135514=CARTESIAN_POINT ( 'NONE',  ( 7.340813827156391191, 7.528980651296110160, 0.7998128361456281477 ) ) ;
#135525=CARTESIAN_POINT ( 'NONE',  ( -5.576146316970437944, 9.727530813099326323, 0.000000000000000000 ) ) ;
#135537=CARTESIAN_POINT ( 'NONE',  ( 5.234329823327693809, 8.264412672927770487, 1.199719254218451159 ) ) ;
#135547=CARTESIAN_POINT ( 'NONE',  ( 1.843739406749228538, 8.920000000000001705, -0.7749999999999996891 ) ) ;
#135552=CARTESIAN_POINT ( 'NONE',  ( 5.207906507908255378, 7.834591108650524660, -1.266300940072472736 ) ) ;
#135581=CARTESIAN_POINT ( 'NONE',  ( -6.611092229237963025, 6.760716375176868631, -0.1380881291089108287 ) ) ;
#135599=CARTESIAN_POINT ( 'NONE',  ( -5.601453741101424022, 6.564059448486966986, -1.199719254218453823 ) ) ;
#135619=CARTESIAN_POINT ( 'NONE',  ( 7.810905894804431426, 8.285347430126213553, 0.000000000000000000 ) ) ;
#135625=CARTESIAN_POINT ( 'NONE',  ( 3.919715808126649659, 7.587102519540811940, 0.000000000000000000 ) ) ;
#135632=CARTESIAN_POINT ( 'NONE',  ( -6.961185525973791144, 7.086080966583015339, 0.7998128361456341429 ) ) ;
#135634=CARTESIAN_POINT ( 'NONE',  ( 6.540882763950133238, 6.595727744222092959, 0.000000000000000000 ) ) ;
#135642=CARTESIAN_POINT ( 'NONE',  ( -4.085803189671902480, 5.860132702740892263, -1.599625672291271394 ) ) ;
#135643=CARTESIAN_POINT ( 'NONE',  ( 6.994027139803230320, 9.253060644560830994, -1.599625672291267398 ) ) ;
#135650=CARTESIAN_POINT ( 'NONE',  ( 7.388267364804250725, 7.584343111885245570, -0.7998128361456341429 ) ) ;
#135656=CARTESIAN_POINT ( 'NONE',  ( -4.804518813248800591, 8.239360463340183571, 0.8967481634083998010 ) ) ;
#135668=CARTESIAN_POINT ( 'NONE',  ( -5.275531169048922386, 5.327410250078064458, -0.7216878364870338292 ) ) ;
#135671=CARTESIAN_POINT ( 'NONE',  ( -5.345219749366619588, 4.708221922861152819, 2.500000000000000444 ) ) ;
#135677=CARTESIAN_POINT ( 'NONE',  ( 4.773879485787624333, 4.742149952939897162, -0.7216878364870357165 ) ) ;
#135681=CARTESIAN_POINT ( 'NONE',  ( -4.762657100150483380, 8.778460060142702304, 0.000000000000000000 ) ) ;
#135694=CARTESIAN_POINT ( 'NONE',  ( 4.329849954717849947, 6.144853928627882489, 1.599625672291262513 ) ) ;
#135720=CARTESIAN_POINT ( 'NONE',  ( 4.095444919779759552, 6.935713618788495793, 1.199719254218451159 ) ) ;
#135721=CARTESIAN_POINT ( 'NONE',  ( -4.421367491832313590, 6.251624388594711590, 1.443375672974065660 ) ) ;
#135746=CARTESIAN_POINT ( 'NONE',  ( -6.688968683495758683, 8.897159112202094988, -1.599625672291271394 ) ) ;
#135761=CARTESIAN_POINT ( 'NONE',  ( -5.803772275101700906, 8.928762199997411386, -1.199719254218452047 ) ) ;
#135763=CARTESIAN_POINT ( 'NONE',  ( 5.038060948978250408, 7.997685013099862239, -1.157798351953726490 ) ) ;
#135768=CARTESIAN_POINT ( 'NONE',  ( 4.228163802615382494, 6.026220084508304708, -1.599625672291269396 ) ) ;
#135772=DIRECTION ( 'NONE',  ( 0.6507913734559606089, -0.7592566023653033458, 0.000000000000000000 ) ) ;
#135773=CARTESIAN_POINT ( 'NONE',  ( -6.448838341955544173, 7.552674816150118708, 1.199719254218452047 ) ) ;
#135776=CARTESIAN_POINT ( 'NONE',  ( -7.607533591043815768, 8.048079742405473525, 0.000000000000000000 ) ) ;
#135779=CARTESIAN_POINT ( 'NONE',  ( -7.878696662872776812, 8.364436659539265406, -0.7216878364870338292 ) ) ;
#135780=CARTESIAN_POINT ( 'NONE',  ( 5.709392084686216506, 5.833581318321598985, -0.7216878364870458196 ) ) ;
#135781=CARTESIAN_POINT ( 'NONE',  ( -3.472296738431328134, 7.065113604896248845, 0.000000000000000000 ) ) ;
#135798=CARTESIAN_POINT ( 'NONE',  ( 6.378761646814803399, 6.917158162233129737, 0.8102004381213165907 ) ) ;
#135806=AXIS2_PLACEMENT_3D ( 'NONE', #45725, #39052, #18517 ) ;
#135818=CARTESIAN_POINT ( 'NONE',  ( 5.748548729368831545, 7.266256959964179529, 1.200940202139972435 ) ) ;
#135836=CARTESIAN_POINT ( 'NONE',  ( -5.661411662158206681, 8.762674818229999829, -1.199719254218452047 ) ) ;
#135848=CARTESIAN_POINT ( 'NONE',  ( 5.956828388357757298, 8.042995434541133193, 1.599625672291269396 ) ) ;
#135851=CARTESIAN_POINT ( 'NONE',  ( 3.615147460157889903, 7.348606074266929689, 0.4009180521483968196 ) ) ;
#135856=CARTESIAN_POINT ( 'NONE',  ( -6.197485614778184271, 9.284131412999601096, 1.082531754730549967 ) ) ;
#135857=ORIENTED_EDGE ( 'NONE', *, *, #189993, .T. ) ;
#135861=CARTESIAN_POINT ( 'NONE',  ( 7.201315867513990554, 8.430565262634994284, -1.199719254218452047 ) ) ;
#135862=CARTESIAN_POINT ( 'NONE',  ( -1.843739406749240750, 8.499999999999996447, 0.7750000000000013545 ) ) ;
#135870=DIRECTION ( 'NONE',  ( -0.7592566023653004592, 0.6507913734559639396, -0.000000000000000000 ) ) ;
#135876=CARTESIAN_POINT ( 'NONE',  ( -6.943184063974178422, 8.233374508458908281, -1.082531754730549967 ) ) ;
#135877=CARTESIAN_POINT ( 'NONE',  ( 6.102578539926878598, 7.252668063737060855, -1.082531754730548412 ) ) ;
#135880=VECTOR ( 'NONE', #12080, 1000.000000000000000 ) ;
#135883=EDGE_LOOP ( 'NONE', ( #186439, #153189, #80453, #138168 ) ) ;
#135889=CARTESIAN_POINT ( 'NONE',  ( -5.309953438407606363, 6.223975762010839574, 1.199719254218452935 ) ) ;
#135890=CARTESIAN_POINT ( 'NONE',  ( -3.688700311369816909, 6.461178242310183784, -1.199719254218450271 ) ) ;
#135892=CARTESIAN_POINT ( 'NONE',  ( 6.007671464186825183, 8.102312356341712984, 1.443375672974064550 ) ) ;
#135904=CARTESIAN_POINT ( 'NONE',  ( -4.789308618567226006, 8.160042084799258078, 0.7984581689710170682 ) ) ;
#135910=CARTESIAN_POINT ( 'NONE',  ( -6.252245114557387851, 7.323316050852266557, -1.199719254218453823 ) ) ;
#135921=CARTESIAN_POINT ( 'NONE',  ( 5.876533236880477240, 5.820653295974182129, 0.7998128361456352531 ) ) ;
#135961=CARTESIAN_POINT ( 'NONE',  ( 5.234856708652227297, 7.200695141551334721, 1.443375672974065660 ) ) ;
#135965=CARTESIAN_POINT ( 'NONE',  ( 7.010974831598141499, 7.352094523052197239, -0.7216878364870317197 ) ) ;
#135980=CARTESIAN_POINT ( 'NONE',  ( -5.908321080505254841, 10.11506803722328129, 0.7998128361456291469 ) ) ;
#135993=CARTESIAN_POINT ( 'NONE',  ( 3.892599500454932304, 7.555466827257172113, 0.7216878364870257245 ) ) ;
#135998=AXIS2_PLACEMENT_3D ( 'NONE', #93848, #92780, #10421 ) ;
#136000=CARTESIAN_POINT ( 'NONE',  ( -7.262327558775498737, 8.501745569106741840, 1.199719254218452047 ) ) ;
#136005=CARTESIAN_POINT ( 'NONE',  ( -6.455090533882201775, 8.624301270986276080, -1.443375672974066548 ) ) ;
#136008=CARTESIAN_POINT ( 'NONE',  ( -7.045397100956844127, 8.248660034984974132, -1.199719254218452047 ) ) ;
#136013=CARTESIAN_POINT ( 'NONE',  ( -5.157951095356222204, 4.982307464195829816, 0.000000000000000000 ) ) ;
#136028=CARTESIAN_POINT ( 'NONE',  ( -3.024877669624710386, 6.543124691288523920, 0.000000000000000000 ) ) ;
#136030=CARTESIAN_POINT ( 'NONE',  ( -5.926322542504884439, 6.086666852443364029, -0.7216878364870338292 ) ) ;
#136032=CARTESIAN_POINT ( 'NONE',  ( 4.115782150200256950, 6.959440387612411349, 1.199719254218452047 ) ) ;
#136033=CARTESIAN_POINT ( 'NONE',  ( -5.517242166118370150, 5.401480380085008193, 0.7998128361456281477 ) ) ;
#136034=CARTESIAN_POINT ( 'NONE',  ( -6.282224075085783177, 8.422623735723785643, 1.599625672291269396 ) ) ;
#136061=CARTESIAN_POINT ( 'NONE',  ( -6.933015448541747006, 9.181880338089085214, 1.599625672291269396 ) ) ;
#136088=DIRECTION ( 'NONE',  ( 0.000000000000000000, 0.000000000000000000, -1.000000000000000000 ) ) ;
#136089=CARTESIAN_POINT ( 'NONE',  ( 5.520104819419390907, 6.469152373191302985, 1.199719254218452935 ) ) ;
#136092=( BOUNDED_CURVE ( )  B_SPLINE_CURVE ( 2, ( #176271, #96100, #129730, #78745, #195714, #27873, #60365 ),
 .UNSPECIFIED., .F., .T. ) 
 B_SPLINE_CURVE_WITH_KNOTS ( ( 3, 2, 2, 3 ),
 ( 0.3250000000000001776, 0.3333333333333334814, 0.3416666666666667851, 0.3500000000000000888 ),
 .UNSPECIFIED. ) 
 CURVE ( )  GEOMETRIC_REPRESENTATION_ITEM ( )  RATIONAL_B_SPLINE_CURVE ( ( 0.9999999999999973355, 0.8660254037844413721, 1.000000000000000000, 0.8660254037844387076, 1.000000000000000000, 0.8660254037844369313, 1.000000000000001776 ) ) 
 REPRESENTATION_ITEM ( '' )  );
#136107=CARTESIAN_POINT ( 'NONE',  ( 6.039231080244466199, 6.010467446565510130, 0.7998128361456352531 ) ) ;
#136114=CARTESIAN_POINT ( 'NONE',  ( -7.370792787684826486, 8.628288336167626582, -1.199719254218452047 ) ) ;
#136125=CARTESIAN_POINT ( 'NONE',  ( -4.595387861177860245, 8.132925338238120361, 0.6295658974326902024 ) ) ;
#136130=CARTESIAN_POINT ( 'NONE',  ( 4.407809338218622308, 8.156544971314787063, 0.000000000000000000 ) ) ;
#136133=CARTESIAN_POINT ( 'NONE',  ( -5.960744811863571968, 6.983232364376142698, 1.199719254218452935 ) ) ;
#136144=CARTESIAN_POINT ( 'NONE',  ( 4.686278372178935392, 5.496354851410763409, 1.199719254218452047 ) ) ;
#136145=CARTESIAN_POINT ( 'NONE',  ( 6.384963997392946844, 6.413822516572072807, 0.7998128361456352531 ) ) ;
#136165=CARTESIAN_POINT ( 'NONE',  ( 4.936581118797800372, 8.100871430792054184, -1.059671831818540966 ) ) ;
#136173=CARTESIAN_POINT ( 'NONE',  ( 3.573456005653643519, 6.326726552307992080, -1.199719254218453823 ) ) ;
#136179=CARTESIAN_POINT ( 'NONE',  ( 4.857564175446106525, 8.889184981320973122, 0.7998128361456331437 ) ) ;
#136184=CARTESIAN_POINT ( 'NONE',  ( 5.072158865288243668, 6.050511776658669127, 1.082531754730549078 ) ) ;
#136189=CARTESIAN_POINT ( 'NONE',  ( 7.404161286838808920, 8.771181268467660885, -1.082531754730548412 ) ) ;
#136201=CARTESIAN_POINT ( 'NONE',  ( 6.365646016822680942, 6.829858545691475769, 0.5939985411197836740 ) ) ;
#136202=CARTESIAN_POINT ( 'NONE',  ( -4.981695098378565945, 4.776675467721892332, -0.7998128361456362523 ) ) ;
#136225=CARTESIAN_POINT ( 'NONE',  ( 4.868786560638889149, 6.773613302202437403, 1.443375672974065660 ) ) ;
#136233=CARTESIAN_POINT ( 'NONE',  ( 5.993586425693011144, 9.150212042353954800, -1.199719254218452047 ) ) ;
#136235=CARTESIAN_POINT ( 'NONE',  ( 5.203297092594585393, 9.292540051327542017, 0.7998128361456341429 ) ) ;
#136236=B_SPLINE_CURVE_WITH_KNOTS ( 'NONE', 3,
 ( #72976, #51421, #117542, #183536 ),
 .UNSPECIFIED., .F., .F.,
 ( 4, 4 ),
 ( 0.001855645002180106307, 0.002097104276149275998 ),
 .UNSPECIFIED. ) ;
#136243=EDGE_CURVE ( 'NONE', #182271, #22322, #162222, .T. ) ;
#136251=CARTESIAN_POINT ( 'NONE',  ( -4.472210567661380587, 6.310941310395290493, 1.599625672291270506 ) ) ;
#136254=CARTESIAN_POINT ( 'NONE',  ( 4.868786560638878491, 8.694351730805124134, 0.7216878364870317197 ) ) ;
#136262=CARTESIAN_POINT ( 'NONE',  ( -4.604929450496978660, 5.401447776115099408, -1.199719254218453823 ) ) ;
#136264=AXIS2_PLACEMENT_3D ( 'NONE', #101926, #66187, #167992 ) ;
#136269=CARTESIAN_POINT ( 'NONE',  ( -6.563555762791521531, 9.711213252348503744, 1.082531754730549967 ) ) ;
#136271=CARTESIAN_POINT ( 'NONE',  ( -6.455090533882206216, 7.663932056684933158, -1.082531754730549967 ) ) ;
#136294=CARTESIAN_POINT ( 'NONE',  ( -5.655686355556086120, 6.627330832017406692, 1.199719254218452935 ) ) ;
#136296=FACE_OUTER_BOUND ( 'NONE', #180691, .T. ) ;
#136300=ORIENTED_EDGE ( 'NONE', *, *, #169774, .F. ) ;
#136305=CARTESIAN_POINT ( 'NONE',  ( -6.175853536056814086, 7.055546168579414079, -1.074032317439767903 ) ) ;
#136308=ORIENTED_EDGE ( 'NONE', *, *, #961, .F. ) ;
#136320=CARTESIAN_POINT ( 'NONE',  ( 2.278321918429430770, 2.687264847272027968, 2.500000000000000888 ) ) ;
#136329=CARTESIAN_POINT ( 'NONE',  ( 1.843739406749228538, 8.923774302061360686, -0.7749999999999996891 ) ) ;
#136338=CARTESIAN_POINT ( 'NONE',  ( 5.520104819419390907, 6.469152373191302985, 1.199719254218452935 ) ) ;
#136346=CARTESIAN_POINT ( 'NONE',  ( 6.013923656113508542, 9.173938811177871244, -1.199719254218452047 ) ) ;
#136349=CARTESIAN_POINT ( 'NONE',  ( 4.634908411025333130, 6.500755460986618495, 1.599625672291268286 ) ) ;
#136363=CARTESIAN_POINT ( 'NONE',  ( 5.535985025370705692, 7.434063834270491000, -1.247683609459742549 ) ) ;
#136365=CARTESIAN_POINT ( 'NONE',  ( -4.923019175093582334, 8.757623114335565617, 0.7216878364870267237 ) ) ;
#136366=CARTESIAN_POINT ( 'NONE',  ( 6.699137298928158124, 6.988284068270579574, 0.7216878364870328300 ) ) ;
#136379=EDGE_CURVE ( 'NONE', #44793, #17896, #30151, .T. ) ;
#136385=CARTESIAN_POINT ( 'NONE',  ( -6.089020385868876062, 6.276481003034692030, -0.7216878364870338292 ) ) ;
#136391=CARTESIAN_POINT ( 'NONE',  ( 4.844006021832467646, 8.873367135438366304, 0.000000000000000000 ) ) ;
#136398=EDGE_CURVE ( 'NONE', #84217, #138803, #196907, .T. ) ;
#136399=FACE_OUTER_BOUND ( 'NONE', #121669, .T. ) ;
#136411=CARTESIAN_POINT ( 'NONE',  ( -4.163763581353360443, 7.871824920094959488, -5.011504818508299590E-05 ) ) ;
#136420=CARTESIAN_POINT ( 'NONE',  ( 6.912678218121202534, 9.158153569265168770, 1.599625672291268286 ) ) ;
#136441=DIRECTION ( 'NONE',  ( -0.6507913734559658270, 0.7592566023652989049, 0.000000000000000000 ) ) ;
#136449=VERTEX_POINT ( 'NONE', #33338 ) ;
#136450=CARTESIAN_POINT ( 'NONE',  ( 4.502716413514295191, 6.346531463890372926, -1.443375672974068769 ) ) ;
#136457=CARTESIAN_POINT ( 'NONE',  ( 7.225569521440261767, 7.394528961293920233, -0.7998128361456341429 ) ) ;
#136461=CARTESIAN_POINT ( 'NONE',  ( -4.014622883422329203, 6.737458226417744278, -1.082531754730546636 ) ) ;
#136478=CARTESIAN_POINT ( 'NONE',  ( 6.481679955784983349, 9.719654494127929922, -1.199719254218452047 ) ) ;
#136488=CARTESIAN_POINT ( 'NONE',  ( 5.090160327287878594, 4.903218234782778850, -0.7998128361456481317 ) ) ;
#136501=CARTESIAN_POINT ( 'NONE',  ( -6.794044374223859428, 7.099008989448849505, 0.000000000000000000 ) ) ;
#136504=CARTESIAN_POINT ( 'NONE',  ( 5.851225812749518695, 8.984124660586543243, -1.199719254218452047 ) ) ;
#136509=CARTESIAN_POINT ( 'NONE',  ( -5.926849427829407269, 6.943687749669614995, -1.199719254218453823 ) ) ;
#136553=CARTESIAN_POINT ( 'NONE',  ( -6.089547271193396227, 7.133501900260939443, -1.199719254218453823 ) ) ;
#136557=CARTESIAN_POINT ( 'NONE',  ( -4.827585214917754719, 7.789877296449459365, -1.199719254218453823 ) ) ;
#136558=CARTESIAN_POINT ( 'NONE',  ( -3.793249116773374841, 7.647484079536056356, 0.7998128361456350310 ) ) ;
#136562=CARTESIAN_POINT ( 'NONE',  ( -5.085717018457573957, 8.947437264926888290, 0.7216878364870267237 ) ) ;
#136564=CARTESIAN_POINT ( 'NONE',  ( -4.733481511527885210, 4.890303307122107590, -0.5491554243041256722 ) ) ;
#136568=CARTESIAN_POINT ( 'NONE',  ( -6.400331034103001748, 9.624747418832267698, 1.199719254218452935 ) ) ;
#136572=VERTEX_POINT ( 'NONE', #51741 ) ;
#136577=CARTESIAN_POINT ( 'NONE',  ( -5.772739544368596043, 9.956889578397179363, -0.7998128361456362523 ) ) ;
#136579=CARTESIAN_POINT ( 'NONE',  ( 4.757636082118741783, 8.295611710538327799, 0.7840751985381082534 ) ) ;
#136584=CARTESIAN_POINT ( 'NONE',  ( 3.413620815590684199, 7.204584394822967752, 0.7998128361456281477 ) ) ;
#136594=CARTESIAN_POINT ( 'NONE',  ( -6.400331034103001748, 9.624747418832267698, 1.199719254218452935 ) ) ;
#136597=CARTESIAN_POINT ( 'NONE',  ( 3.940069096733910037, 8.986657997193951530, -0.7749999999999996891 ) ) ;
#136606=CARTESIAN_POINT ( 'NONE',  ( 6.855582950365507244, 8.027210192628430718, -1.199719254218452047 ) ) ;
#136613=CARTESIAN_POINT ( 'NONE',  ( 1.930226670627029684, 8.999999999999998224, 0.7750000000000004663 ) ) ;
#136616=CARTESIAN_POINT ( 'NONE',  ( -4.260029445439560192, 7.236136616047151193, 2.419999999999999485 ) ) ;
#136620=CARTESIAN_POINT ( 'NONE',  ( 5.959663945170571075, 7.214374732172471383, -1.219933935757764099 ) ) ;
#136632=ORIENTED_EDGE ( 'NONE', *, *, #183283, .F. ) ;
#136643=CARTESIAN_POINT ( 'NONE',  ( -5.578701055370745010, 7.405485896932115786, -1.243560882958130387 ) ) ;
#136649=CARTESIAN_POINT ( 'NONE',  ( -6.365373075063135211, 6.924066019909299818, 0.8511317711424144505 ) ) ;
#136665=CARTESIAN_POINT ( 'NONE',  ( 3.571793831781210127, 7.341190112860298100, -0.2923163854498100345 ) ) ;
#136669=CARTESIAN_POINT ( 'NONE',  ( -5.926849427829407269, 6.943687749669614995, -1.199719254218453823 ) ) ;
#136685=CARTESIAN_POINT ( 'NONE',  ( 4.706615602599436343, 5.520081620234675412, 1.199719254218452935 ) ) ;
#136687=CARTESIAN_POINT ( 'NONE',  ( 7.146556367734764770, 9.431011410480991231, 1.443375672974063439 ) ) ;
#136696=CARTESIAN_POINT ( 'NONE',  ( 6.333067150914817312, 6.561202228921680479, 0.7216878364870358276 ) ) ;
#136702=CARTESIAN_POINT ( 'NONE',  ( 6.717138760927786834, 6.801359740696030443, -0.7998128361456481317 ) ) ;
#136712=CARTESIAN_POINT ( 'NONE',  ( -4.492547798081878874, 6.334668079219206049, 1.599625672291263179 ) ) ;
#136713=CARTESIAN_POINT ( 'NONE',  ( 4.934241560730721510, 4.721313007132757811, 0.000000000000000000 ) ) ;
#136719=CARTESIAN_POINT ( 'NONE',  ( 4.850785098639300408, 8.881276058379668825, -0.7998128361456481317 ) ) ;
#136725=CARTESIAN_POINT ( 'NONE',  ( -4.762965077474956566, 8.286028185285090331, 0.8196324637163689975 ) ) ;
#136734=CARTESIAN_POINT ( 'NONE',  ( -4.950135482320929370, 5.908151163196758482, -1.082531754730549967 ) ) ;
#136743=CARTESIAN_POINT ( 'NONE',  ( 4.475600106286968582, 5.354526557823810151, -1.082531754730548412 ) ) ;
#136747=CARTESIAN_POINT ( 'NONE',  ( -5.611095471209320174, 7.639640364534566075, 1.599625672291263179 ) ) ;
#136751=VERTEX_POINT ( 'NONE', #152435 ) ;
#136760=CARTESIAN_POINT ( 'NONE',  ( 4.004454267989866700, 5.765225627445230927, 1.599625672291262513 ) ) ;
#136764=CARTESIAN_POINT ( 'NONE',  ( 4.362691568547327314, 8.311833606605697256, -0.7998128361456381397 ) ) ;
#136783=CARTESIAN_POINT ( 'NONE',  ( -0.3364766900451948706, 3.351562295342669806, 1.974266290975867699 ) ) ;
#136786=CARTESIAN_POINT ( 'NONE',  ( -5.316205630334268406, 6.335233002545657577, -1.082531754730549967 ) ) ;
#136789=EDGE_CURVE ( 'NONE', #179029, #7836, #89720, .T. ) ;
#136811=CARTESIAN_POINT ( 'NONE',  ( -6.282224075085783177, 8.422623735723785643, 1.599625672291269396 ) ) ;
#136821=ORIENTED_EDGE ( 'NONE', *, *, #32706, .T. ) ;
#136826=CARTESIAN_POINT ( 'NONE',  ( -3.305155586681401303, 7.078041627762083898, 0.7998128361456352531 ) ) ;
#136832=CARTESIAN_POINT ( 'NONE',  ( 6.586134412937156846, 6.778852895089745090, 0.3294091213778785887 ) ) ;
#136838=CARTESIAN_POINT ( 'NONE',  ( -5.237192476628793614, 9.332084666034067055, 0.7998128361456291469 ) ) ;
#136842=CARTESIAN_POINT ( 'NONE',  ( -5.483346782084204563, 5.361935765378481378, 0.000000000000000000 ) ) ;
#136846=CARTESIAN_POINT ( 'NONE',  ( 3.892599500454941630, 6.595097612955829192, 1.082531754730549078 ) ) ;
#136848=CARTESIAN_POINT ( 'NONE',  ( -5.492461626867567226, 6.540864998501174199, 1.082531754730549078 ) ) ;
#136853=CARTESIAN_POINT ( 'NONE',  ( -3.949167883330528372, 7.829389307186077396, 1.214306433183764966E-14 ) ) ;
#136862=CARTESIAN_POINT ( 'NONE',  ( 3.854260808034858155, 7.718664386007802136, -0.7998128361456361413 ) ) ;
#136866=CARTESIAN_POINT ( 'NONE',  ( 0.3701041174201537554, 2.825470661167653663, -2.033038120852537656 ) ) ;
#136867=CARTESIAN_POINT ( 'NONE',  ( 5.017113787211129328, 8.018716392533608683, 1.139262206072016559 ) ) ;
#136873=CARTESIAN_POINT ( 'NONE',  ( 4.082413651490639062, 7.776916670132135501, 0.000000000000000000 ) ) ;
#136877=CARTESIAN_POINT ( 'NONE',  ( 5.091969210384201361, 8.098325291160362482, 1.199719254218452047 ) ) ;
#136887=CARTESIAN_POINT ( 'NONE',  ( 5.975194856099406593, 7.098212677808693805, 1.080521340106417982 ) ) ;
#136906=CARTESIAN_POINT ( 'NONE',  ( -6.252245114557387851, 7.323316050852266557, -1.199719254218453823 ) ) ;
#136919=CARTESIAN_POINT ( 'NONE',  ( 5.224688093219824303, 7.188831756880171397, -1.599625672291283607 ) ) ;
#136933=CARTESIAN_POINT ( 'NONE',  ( 5.031484404002889654, 6.003058238492422483, 1.082531754730549078 ) ) ;
#136949=CARTESIAN_POINT ( 'NONE',  ( -6.129694847154211423, 9.205042184104968328, -1.082531754730549967 ) ) ;
#136950=CARTESIAN_POINT ( 'NONE',  ( 6.726253606155519371, 7.019919760035800316, -0.7216878364870458196 ) ) ;
#136959=CARTESIAN_POINT ( 'NONE',  ( -5.469788628470539926, 5.346117919495872783, -0.7998128361456362523 ) ) ;
#136960=CARTESIAN_POINT ( 'NONE',  ( -4.821859908315634158, 5.654533310236863564, 1.199719254218452935 ) ) ;
#136962=CARTESIAN_POINT ( 'NONE',  ( 6.007671464186834065, 7.141943142040370063, 1.082531754730549967 ) ) ;
#136974=CARTESIAN_POINT ( 'NONE',  ( -4.636404737997885661, 8.342837909782009120, -0.3584692566244596645 ) ) ;
#136978=CARTESIAN_POINT ( 'NONE',  ( 4.177320726786311056, 5.966903162707725805, -1.443375672974068769 ) ) ;
#136982=CARTESIAN_POINT ( 'NONE',  ( -6.140917232347002042, 6.129101290685087911, -0.7998128361456362523 ) ) ;
#136993=CARTESIAN_POINT ( 'NONE',  ( 5.228604516725597229, 6.129068686715179126, -1.199719254218450271 ) ) ;
#137029=CARTESIAN_POINT ( 'NONE',  ( 4.245111494854632461, 7.966730820723463502, 0.000000000000000000 ) ) ;
#137035=CARTESIAN_POINT ( 'NONE',  ( 4.977251789548238214, 7.860525283564661514, -1.082531754730548412 ) ) ;
#137043=EDGE_CURVE ( 'NONE', #2366, #137116, #48674, .T. ) ;
#137050=CARTESIAN_POINT ( 'NONE',  ( -7.391130018105325661, 8.652015104991543026, -1.199719254218452047 ) ) ;
#137062=CARTESIAN_POINT ( 'NONE',  ( 3.729901657090948230, 6.405283462364505631, 1.082531754730549078 ) ) ;
#137068=CARTESIAN_POINT ( 'NONE',  ( -6.563028877466991595, 9.814561569423593923, 1.199719254218452935 ) ) ;
#137073=CARTESIAN_POINT ( 'NONE',  ( -7.160114521792834807, 8.486460042580672436, 1.082531754730549078 ) ) ;
#137076=CARTESIAN_POINT ( 'NONE',  ( -5.915100157312088491, 10.12297696016459092, -0.7998128361456362523 ) ) ;
#137081=CARTESIAN_POINT ( 'NONE',  ( -3.526002468005825286, 6.271364091718859335, -1.199719254218450271 ) ) ;
#137098=CARTESIAN_POINT ( 'NONE',  ( -4.502716413514301408, 7.306900678191715848, -1.082531754730549967 ) ) ;
#137100=CARTESIAN_POINT ( 'NONE',  ( -5.600926855776894975, 6.667407765562058053, -1.082531754730549967 ) ) ;
#137101=CARTESIAN_POINT ( 'NONE',  ( 4.603875680292229156, 7.528882839386387360, 1.199719254218452047 ) ) ;
#137102=CARTESIAN_POINT ( 'NONE',  ( -4.281342646865346602, 8.216926531310035031, 0.7998128361456352531 ) ) ;
#137103=CARTESIAN_POINT ( 'NONE',  ( -5.932574734431526942, 9.079031735882207244, 1.199719254218454489 ) ) ;
#137116=VERTEX_POINT ( 'NONE', #141565 ) ;
#137128=CARTESIAN_POINT ( 'NONE',  ( 0.4000000000000000777, 2.999999999999999112, -2.420000000000000373 ) ) ;
#137153=CARTESIAN_POINT ( 'NONE',  ( 7.006746397889325628, 6.052176462752766106, -2.500000000000000444 ) ) ;
#137159=ORIENTED_EDGE ( 'NONE', *, *, #107594, .F. ) ;
#137163=CARTESIAN_POINT ( 'NONE',  ( 4.362691568547328202, 8.311833606605697256, -0.7998128361456381397 ) ) ;
#137165=CARTESIAN_POINT ( 'NONE',  ( 2.353140975214496944, 2.704741401632033249, -2.456000212125921678 ) ) ;
#137179=CARTESIAN_POINT ( 'NONE',  ( 5.041653019435334393, 6.975290837464928728, -1.599625672291269396 ) ) ;
#137187=CARTESIAN_POINT ( 'NONE',  ( -5.413448473606448985, 9.537716662508005427, 0.000000000000000000 ) ) ;
#137192=CARTESIAN_POINT ( 'NONE',  ( 4.817943484809818600, 6.714296380401858499, 1.599625672291269396 ) ) ;
#137197=CARTESIAN_POINT ( 'NONE',  ( -5.963818478108997567, 6.870746658508759097, 0.9995729632361770589 ) ) ;
#137203=CARTESIAN_POINT ( 'NONE',  ( 4.746763178560241769, 8.551991118380046331, 0.7216878364870328300 ) ) ;
#137206=CARTESIAN_POINT ( 'NONE',  ( -4.665414256878304577, 5.575976400180357118, -1.082531754730549967 ) ) ;
#137207=CARTESIAN_POINT ( 'NONE',  ( -5.098748287191073203, 8.106234214101666780, 1.199719254218452935 ) ) ;
#137220=CARTESIAN_POINT ( 'NONE',  ( 3.054329744828568227, 6.785411478933790264, 0.000000000000000000 ) ) ;
#137221=CARTESIAN_POINT ( 'NONE',  ( 5.143339171537801846, 7.093924681584509173, 1.599625672291269396 ) ) ;
#137238=CARTESIAN_POINT ( 'NONE',  ( 5.544801429207002030, 7.539493339695484408, -1.337888636821100041 ) ) ;
#137240=ORIENTED_EDGE ( 'NONE', *, *, #98017, .T. ) ;
#137248=CARTESIAN_POINT ( 'NONE',  ( 5.408776937209000657, 5.274937613024121674, 0.7998128361456352531 ) ) ;
#137252=CARTESIAN_POINT ( 'NONE',  ( 5.969332771766739931, 10.18624834369502885, -0.7998128361456481317 ) ) ;
#137257=CARTESIAN_POINT ( 'NONE',  ( 4.733205024946604667, 8.536173272497439513, 0.000000000000000000 ) ) ;
#137260=CARTESIAN_POINT ( 'NONE',  ( 3.054329744828568227, 6.785411478933790264, 0.000000000000000000 ) ) ;
#137271=CARTESIAN_POINT ( 'NONE',  ( 5.969043672405669909, 7.102642550806028687, -1.084880274121432064 ) ) ;
#137272=CARTESIAN_POINT ( 'NONE',  ( -3.298376509874564988, 7.070132704820777825, 0.000000000000000000 ) ) ;
#137281=CARTESIAN_POINT ( 'NONE',  ( 0.1216811705908975444, 2.536982183874235908, -1.996294991408742447 ) ) ;
#137292=ORIENTED_EDGE ( 'NONE', *, *, #208628, .T. ) ;
#137295=LINE ( 'NONE', #130163, #98756 ) ;
#137303=VERTEX_POINT ( 'NONE', #49099 ) ;
#137307=CARTESIAN_POINT ( 'NONE',  ( 5.559725510055676168, 8.644040974110419384, 1.199719254218451159 ) ) ;
#137309=CARTESIAN_POINT ( 'NONE',  ( 6.875920180786008196, 8.050936961452347163, -1.199719254218452047 ) ) ;
#137322=CARTESIAN_POINT ( 'NONE',  ( -3.637330350216213759, 7.465578851886037093, -0.7998128361456481317 ) ) ;
#137324=CARTESIAN_POINT ( 'NONE',  ( 5.682275777458841048, 8.683053269460405232, 1.082531754730547524 ) ) ;
#137334=CARTESIAN_POINT ( 'NONE',  ( -3.447516199624892419, 7.244129009529488350, 0.7998128361456352531 ) ) ;
#137340=CARTESIAN_POINT ( 'NONE',  ( -5.632486471834530661, 5.535932070087196344, -0.7998128361456362523 ) ) ;
#137342=CARTESIAN_POINT ( 'NONE',  ( -4.977251789992602760, 8.820894498384422633, 0.000000000000000000 ) ) ;
#137365=CARTESIAN_POINT ( 'NONE',  ( -6.252245114557387851, 7.323316050852266557, -1.199719254218453823 ) ) ;
#137367=CARTESIAN_POINT ( 'NONE',  ( -4.167152111353897403, 5.955039778036558040, 1.599625672291270506 ) ) ;
#137376=CARTESIAN_POINT ( 'NONE',  ( -6.462985781203115287, 6.858296038324478872, -0.6802466501308057634 ) ) ;
#137384=DIRECTION ( 'NONE',  ( 0.7592566023653003482, 0.6507913734559641616, 0.000000000000000000 ) ) ;
#137390=CARTESIAN_POINT ( 'NONE',  ( 4.046711340876006702, 3.801480273782092745, 2.500000000000000444 ) ) ;
#137395=CARTESIAN_POINT ( 'NONE',  ( 4.635512016184385686, 8.422473116793771197, 0.5971484286424336707 ) ) ;
#137405=CARTESIAN_POINT ( 'NONE',  ( 4.869313445963426190, 5.709895770826003414, 1.199719254218452935 ) ) ;
#137414=CARTESIAN_POINT ( 'NONE',  ( 6.496291879603339758, 7.608037276739255006, 1.199719254218452935 ) ) ;
#137416=CARTESIAN_POINT ( 'NONE',  ( 6.866278450678116485, 6.975356045404744521, 0.000000000000000000 ) ) ;
#137430=CARTESIAN_POINT ( 'NONE',  ( 6.484283628081795037, 6.752753718119230975, 0.1579380340677779548 ) ) ;
#137432=CARTESIAN_POINT ( 'NONE',  ( 6.387299765813869712, 6.624473612970537495, 0.000000000000000000 ) ) ;
#137442=CARTESIAN_POINT ( 'NONE',  ( -2.986538976760251263, 6.706322249520737522, -0.7998128361456481317 ) ) ;
#137454=CARTESIAN_POINT ( 'NONE',  ( -6.116136693096208887, 6.308116694799912771, 0.7216878364870257245 ) ) ;
#137459=CARTESIAN_POINT ( 'NONE',  ( 7.340813827156391191, 7.528980651296110160, 0.7998128361456281477 ) ) ;
#137467=DIRECTION ( 'NONE',  ( -1.000000000000000000, 0.000000000000000000, 0.000000000000000000 ) ) ;
#137476=CARTESIAN_POINT ( 'NONE',  ( -3.667627899390105473, 3.521066046765052970, -2.447586748966623649 ) ) ;
#137481=ORIENTED_EDGE ( 'NONE', *, *, #187556, .T. ) ;
#137514=CARTESIAN_POINT ( 'NONE',  ( 3.716343503921665459, 6.389465617000312569, -1.082531754730549967 ) ) ;
#137516=VERTEX_POINT ( 'NONE', #182268 ) ;
#137520=CARTESIAN_POINT ( 'NONE',  ( -5.908321080505254841, 10.11506803722328129, 0.7998128361456291469 ) ) ;
#137522=CARTESIAN_POINT ( 'NONE',  ( 7.523848900940885542, 7.742521570711348389, 0.7998128361456291469 ) ) ;
#137527=CARTESIAN_POINT ( 'NONE',  ( -4.001064729808656573, 7.682009594836471500, 1.214306433183764966E-14 ) ) ;
#137547=CARTESIAN_POINT ( 'NONE',  ( 6.964048179274811012, 8.153752959689313684, 1.199719254218452047 ) ) ;
#137558=CARTESIAN_POINT ( 'NONE',  ( 7.688882512725796481, 8.142986817701137525, 0.000000000000000000 ) ) ;
#137571=CARTESIAN_POINT ( 'NONE',  ( -4.312902262922974295, 8.045820050136510915, 0.7216878364870338292 ) ) ;
#137573=CARTESIAN_POINT ( 'NONE',  ( 5.691390622686558487, 9.861982503101517139, 0.7998128361456341429 ) ) ;
#137578=CARTESIAN_POINT ( 'NONE',  ( -4.817943484809863008, 6.714296380401858499, 1.599625672291263179 ) ) ;
#137583=VECTOR ( 'NONE', #201223, 1000.000000000000000 ) ;
#137595=AXIS2_PLACEMENT_3D ( 'NONE', #140079, #123893, #58798 ) ;
#137618=CARTESIAN_POINT ( 'NONE',  ( 3.607878275012302627, 7.223292064240769861, 0.7216878364870257245 ) ) ;
#137623=CARTESIAN_POINT ( 'NONE',  ( -6.200875153403786477, 8.327716660428123419, -1.599625672291271394 ) ) ;
#137627=CARTESIAN_POINT ( 'NONE',  ( -4.423703259808839938, 8.383013913077441259, 0.7998128361456352531 ) ) ;
#137632=CARTESIAN_POINT ( 'NONE',  ( -6.821160681006823268, 9.051383109298335228, 1.443375672974064550 ) ) ;
#137638=CARTESIAN_POINT ( 'NONE',  ( -7.425025402139490360, 8.691559719698066289, 1.199719254218452047 ) ) ;
#137645=CARTESIAN_POINT ( 'NONE',  ( -7.469616286486262524, 7.679250187180907794, 0.7998128361456341429 ) ) ;
#137647=CARTESIAN_POINT ( 'NONE',  ( 5.834480046583573554, 7.201333694826374199, -1.164487238324034557 ) ) ;
#137652=CARTESIAN_POINT ( 'NONE',  ( 3.386504508363381571, 7.172948703057747011, -0.7998128361456362523 ) ) ;
#137655=CIRCLE ( 'NONE', #148148, 0.08000000000000020983 ) ;
#137662=CARTESIAN_POINT ( 'NONE',  ( -7.370792787684826486, 8.628288336167626582, -1.199719254218452047 ) ) ;
#137665=CARTESIAN_POINT ( 'NONE',  ( 2.938820208668512901, 6.442724320172973584, -0.2506311418671491320 ) ) ;
#137675=CARTESIAN_POINT ( 'NONE',  ( 4.543917759235442944, 5.330267469643351852, 1.199719254218452935 ) ) ;
#137688=CARTESIAN_POINT ( 'NONE',  ( 5.917965873332177829, 7.245500866451762612, 1.242176317587460943 ) ) ;
#137717=CARTESIAN_POINT ( 'NONE',  ( -5.922807744518227224, 7.239652023730190677, 1.252291340712426981 ) ) ;
#137722=ORIENTED_EDGE ( 'NONE', *, *, #45594, .F. ) ;
#137738=CARTESIAN_POINT ( 'NONE',  ( -4.782994330570982555, 8.802186828966616972, 0.000000000000000000 ) ) ;
#137755=CARTESIAN_POINT ( 'NONE',  ( 5.110497557708379546, 4.926945003606695295, -0.7998128361456481317 ) ) ;
#137757=CARTESIAN_POINT ( 'NONE',  ( 5.817857313595521163, 9.801600942587855414, -0.7216878364870458196 ) ) ;
#137772=CARTESIAN_POINT ( 'NONE',  ( 5.367048706163317640, 7.354919138647580290, -1.599625672291281386 ) ) ;
#137782=CARTESIAN_POINT ( 'NONE',  ( -5.004894982100124068, 5.868074229652107121, 1.199719254218452935 ) ) ;
#137783=CARTESIAN_POINT ( 'NONE',  ( 5.982890925380405456, 10.20206618957764100, 0.000000000000000000 ) ) ;
#137787=CARTESIAN_POINT ( 'NONE',  ( -4.437261413422502798, 8.398831758960053406, 0.000000000000000000 ) ) ;
#137790=CARTESIAN_POINT ( 'NONE',  ( 5.688527969385528849, 8.794310509995222347, -1.199719254218452047 ) ) ;
#137796=CARTESIAN_POINT ( 'NONE',  ( -5.386518286579200954, 7.671588192869585043, 1.336358942847740927 ) ) ;
#137806=CARTESIAN_POINT ( 'NONE',  ( -6.265276382846530545, 6.482112999508623297, 0.000000000000000000 ) ) ;
#137816=CARTESIAN_POINT ( 'NONE',  ( 3.607878275012302627, 7.223292064240769861, 0.7216878364870257245 ) ) ;
#137820=CARTESIAN_POINT ( 'NONE',  ( -5.915100157312088491, 10.12297696016459092, -0.7998128361456362523 ) ) ;
#137833=CARTESIAN_POINT ( 'NONE',  ( 2.898410978271408922, 6.603506251283770112, -0.7998128361456362523 ) ) ;
#137837=CARTESIAN_POINT ( 'NONE',  ( -4.875303370615012177, 4.879929216858088559, -0.6230339956202604057 ) ) ;
#137862=CARTESIAN_POINT ( 'NONE',  ( -5.506019780925599960, 5.596313630600862510, 0.7216878364870257245 ) ) ;
#137886=CARTESIAN_POINT ( 'NONE',  ( -7.469616286486262524, 7.679250187180907794, 0.7998128361456341429 ) ) ;
#137893=CARTESIAN_POINT ( 'NONE',  ( -3.610214042988883598, 7.433943160120816351, 0.7998128361456352531 ) ) ;
#137900=CARTESIAN_POINT ( 'NONE',  ( -5.164730172163054966, 4.990216387137135889, -0.7998128361456362523 ) ) ;
#137906=CARTESIAN_POINT ( 'NONE',  ( 4.258142763143749399, 7.125527769379820242, 1.199719254218451159 ) ) ;
#137910=CARTESIAN_POINT ( 'NONE',  ( -7.259464905474441565, 7.434073576000447048, -0.7998128361456362523 ) ) ;
#137913=CARTESIAN_POINT ( 'NONE',  ( -4.390861645979385663, 6.216034235099629157, -1.599625672291271394 ) ) ;
#137917=CARTESIAN_POINT ( 'NONE',  ( 5.085717018457579286, 6.066329622022862189, -1.082531754730548412 ) ) ;
#137918=CARTESIAN_POINT ( 'NONE',  ( -3.973948422136968084, 7.650373902552835226, -0.7216878364870458196 ) ) ;
#137924=CARTESIAN_POINT ( 'NONE',  ( 5.727393547130178675, 5.646656991265468939, 0.000000000000000000 ) ) ;
#137930=FACE_OUTER_BOUND ( 'NONE', #97484, .T. ) ;
#137935=CARTESIAN_POINT ( 'NONE',  ( 6.013528089337225602, 7.174620582783560963, 1.187335689305318853 ) ) ;
#137945=CARTESIAN_POINT ( 'NONE',  ( 5.688527969385528849, 8.794310509995222347, -1.199719254218452047 ) ) ;
#137956=CARTESIAN_POINT ( 'NONE',  ( 5.871284023695358734, 7.173991544917035945, 1.145568358895364458 ) ) ;
#137972=CARTESIAN_POINT ( 'NONE',  ( -4.308458954092677651, 8.248562223075252220, -0.7998128361456362523 ) ) ;
#137980=EDGE_CURVE ( 'NONE', #213748, #40754, #61307, .T. ) ;
#137987=CARTESIAN_POINT ( 'NONE',  ( 6.723917837734620484, 6.809268663637336516, 0.000000000000000000 ) ) ;
#137995=CARTESIAN_POINT ( 'NONE',  ( -6.238160075619175515, 10.29195416494877513, 0.000000000000000000 ) ) ;
#137996=EDGE_LOOP ( 'NONE', ( #61693, #125463, #67632, #116645 ) ) ;
#137999=CARTESIAN_POINT ( 'NONE',  ( 4.055297343818931033, 6.784911763547157193, 1.082531754730549078 ) ) ;
#138014=CARTESIAN_POINT ( 'NONE',  ( -3.902768115887413014, 5.646591783325653147, -1.599625672291283607 ) ) ;
#138015=CARTESIAN_POINT ( 'NONE',  ( 6.861835142292143530, 8.138467433163244280, 1.082531754730549967 ) ) ;
#138025=CARTESIAN_POINT ( 'NONE',  ( -6.459533842268148973, 6.500820668926428958, 0.000000000000000000 ) ) ;
#138026=CARTESIAN_POINT ( 'NONE',  ( -4.228163802615396705, 6.026220084508304708, -1.599625672291271394 ) ) ;
#138029=CARTESIAN_POINT ( 'NONE',  ( 6.089020385868848528, 8.197219431637373432, -1.443375672974078761 ) ) ;
#138033=AXIS2_PLACEMENT_3D ( 'NONE', #179682, #31302, #196982 ) ;
#138041=CARTESIAN_POINT ( 'NONE',  ( -4.784432227305938312, 8.165582598138012571, -0.7895561949947740299 ) ) ;
#138045=CARTESIAN_POINT ( 'NONE',  ( 4.204437034013637664, 6.958908068774287692, -1.082531754730548412 ) ) ;
#138049=CARTESIAN_POINT ( 'NONE',  ( -6.089547271193396227, 7.133501900260939443, -1.199719254218453823 ) ) ;
#138062=CARTESIAN_POINT ( 'NONE',  ( 4.797606254389322089, 6.690569611577942943, 1.599625672291268286 ) ) ;
#138101=CARTESIAN_POINT ( 'NONE',  ( 5.872089928494542477, 9.864872326636710653, 0.000000000000000000 ) ) ;
#138106=CARTESIAN_POINT ( 'NONE',  ( 5.953438849732186178, 8.999410187112612647, -1.082531754730548412 ) ) ;
#138122=CARTESIAN_POINT ( 'NONE',  ( -6.084577077482911101, 10.32070003369722144, 0.000000000000000000 ) ) ;
#138131=CARTESIAN_POINT ( 'NONE',  ( -4.462568837553487100, 5.235360394347691404, -1.199719254218453823 ) ) ;
#138133=CARTESIAN_POINT ( 'NONE',  ( 4.597623488365603528, 5.496887170248887067, -1.082531754730548412 ) ) ;
#138139=CARTESIAN_POINT ( 'NONE',  ( -2.979759899953417612, 6.698413326579433225, 0.7998128361456352531 ) ) ;
#138144=CARTESIAN_POINT ( 'NONE',  ( -6.129694847154220305, 8.244672969803623630, -1.443375672974066548 ) ) ;
#138148=CARTESIAN_POINT ( 'NONE',  ( -6.424584688029276514, 8.588711117491191871, 1.599625672291269396 ) ) ;
#138153=CARTESIAN_POINT ( 'NONE',  ( -6.147696309153835692, 6.137010213626392208, 0.7998128361456281477 ) ) ;
#138167=CARTESIAN_POINT ( 'NONE',  ( -5.655159470675923394, 5.770309935309573923, 0.000000000000000000 ) ) ;
#138168=ORIENTED_EDGE ( 'NONE', *, *, #104484, .F. ) ;
#138169=CARTESIAN_POINT ( 'NONE',  ( -3.621436428181653788, 7.239109909604962922, 0.7216878364870338292 ) ) ;
#138170=CARTESIAN_POINT ( 'NONE',  ( 5.224688093219824303, 7.188831756880171397, -1.599625672291283607 ) ) ;
#138171=CARTESIAN_POINT ( 'NONE',  ( -4.793689830883590020, 7.750332681742931662, 1.199719254218452935 ) ) ;
#138172=CARTESIAN_POINT ( 'NONE',  ( -6.957269102468015554, 8.145844036748005834, 1.199719254218452047 ) ) ;
#138186=B_SPLINE_CURVE_WITH_KNOTS ( 'NONE', 3,
 ( #45228, #157910, #75577, #207699 ),
 .UNSPECIFIED., .F., .F.,
 ( 4, 4 ),
 ( 0.000000000000000000, 0.0001873600508426472261 ),
 .UNSPECIFIED. ) ;
#138193=CARTESIAN_POINT ( 'NONE',  ( 5.712781623311797397, 7.758274208654143855, -1.599625672291283607 ) ) ;
#138219=CARTESIAN_POINT ( 'NONE',  ( 5.045036709957831711, 4.903268083610561767, 0.3063280728123271568 ) ) ;
#138220=CARTESIAN_POINT ( 'NONE',  ( -1.921775512840688371, 9.000000000008071765, -0.7749999999999996891 ) ) ;
#138222=CARTESIAN_POINT ( 'NONE',  ( 5.717509255324652706, 7.006698007003303807, -2.500000000000000444 ) ) ;
#138230=CARTESIAN_POINT ( 'NONE',  ( 5.910428620914669473, 5.860197910680708944, 0.000000000000000000 ) ) ;
#138247=CARTESIAN_POINT ( 'NONE',  ( 3.379725431556547477, 7.165039780116438273, -1.734723475976807094E-15 ) ) ;
#138254=CARTESIAN_POINT ( 'NONE',  ( -7.923814432544069142, 8.209148024248356990, 0.000000000000000000 ) ) ;
#138258=CARTESIAN_POINT ( 'NONE',  ( 4.712340909201580885, 7.655425606447271214, -1.199719254218452047 ) ) ;
#138268=CARTESIAN_POINT ( 'NONE',  ( 5.722950238744198614, 8.730506807626655430, 1.082531754730549967 ) ) ;
#138269=CARTESIAN_POINT ( 'NONE',  ( -3.960390268967665328, 6.674186842887300131, 1.082531754730549967 ) ) ;
#138270=CARTESIAN_POINT ( 'NONE',  ( -4.586401103172829785, 8.572828063668767484, 0.7998128361456281477 ) ) ;
#138282=CARTESIAN_POINT ( 'NONE',  ( 6.364626766972446781, 6.390095747748157251, 0.7998128361456352531 ) ) ;
#138283=CARTESIAN_POINT ( 'NONE',  ( 4.362691568547328202, 8.311833606605697256, -0.7998128361456381397 ) ) ;
#138286=CARTESIAN_POINT ( 'NONE',  ( 7.374709211190586089, 7.568525266002632534, 0.000000000000000000 ) ) ;
#138300=CARTESIAN_POINT ( 'NONE',  ( 5.696489930276292135, 7.416392257432566026, -1.320530921439456273 ) ) ;
#138304=ADVANCED_FACE ( 'NONE', ( #101283 ), #99175, .T. ) ;
#138309=CARTESIAN_POINT ( 'NONE',  ( 3.725458348705031231, 7.568394850123006279, -1.734723475976807094E-15 ) ) ;
#138313=CARTESIAN_POINT ( 'NONE',  ( 5.096939404094710468, 4.911127157724081371, 0.000000000000000000 ) ) ;
#138317=CARTESIAN_POINT ( 'NONE',  ( 6.373741612200171325, 7.569024981389272710, 1.082531754730549967 ) ) ;
#138319=CARTESIAN_POINT ( 'NONE',  ( -5.926849427829407269, 6.943687749669614995, -1.199719254218453823 ) ) ;
#138321=CARTESIAN_POINT ( 'NONE',  ( 7.241463443474815520, 8.581367117876336437, -1.082531754730548412 ) ) ;
#138329=CARTESIAN_POINT ( 'NONE',  ( -4.016220928916872879, 7.677703825520077352, -0.2262283546238970933 ) ) ;
#138332=CARTESIAN_POINT ( 'NONE',  ( 6.353009478083933459, 6.838182937092724956, 0.6209923359970755952 ) ) ;
#138333=CARTESIAN_POINT ( 'NONE',  ( -5.966997003790217136, 9.975597247814986801, -0.7216878364870338292 ) ) ;
#138363=( BOUNDED_SURFACE ( )  B_SPLINE_SURFACE ( 3, 2, ( 
 ( #181988, #80244, #213416 ),
 ( #16278, #1094, #67155 ),
 ( #49876, #212355, #163642 ),
 ( #13096, #199297, #130147 ),
 ( #96527, #179885, #197183 ),
 ( #111749, #148453, #23 ),
 ( #145292, #195061, #162576 ),
 ( #146342, #47777, #31509 ),
 ( #97584, #15223, #147389 ),
 ( #48820, #114936, #55206 ) ),
 .UNSPECIFIED., .F., .F., .T. ) 
 B_SPLINE_SURFACE_WITH_KNOTS ( ( 4, 2, 2, 2, 4 ),
 ( 3, 3 ),
 ( 0.001504998634567469764, 0.001881248293209337313, 0.002257497951851204863, 0.002633747610493072412, 0.003009997269134939962 ),
 ( 0.000000000000000000, 1.000000000000000000 ),
 .UNSPECIFIED. ) 
 GEOMETRIC_REPRESENTATION_ITEM ( )  RATIONAL_B_SPLINE_SURFACE ( (
 ( 1.000000000000000000, 0.7127552757490021040, 1.000000000000000000),
 ( 1.000000000000000000, 0.7006570731214798453, 1.000000000000000000),
 ( 1.000000000000000000, 0.7089665949506331888, 1.000000000000000000),
 ( 1.000000000000000000, 0.7450337546129037758, 1.000000000000000000),
 ( 1.000000000000000000, 0.7695313365922599180, 1.000000000000000000),
 ( 1.000000000000000000, 0.7891799723974980418, 1.000000000000000000),
 ( 1.000000000000000000, 0.7830193708541549613, 1.000000000000000000),
 ( 1.000000000000000000, 0.7491666546211300792, 1.000000000000000000),
 ( 1.000000000000000000, 0.7234076953912167429, 1.000000000000000000),
 ( 1.000000000000000000, 0.7127558927793078425, 1.000000000000000000) ) ) 
 REPRESENTATION_ITEM ( '' )  SURFACE ( )  );
#138369=CARTESIAN_POINT ( 'NONE',  ( 6.535912570239620578, 9.782925877658371405, 1.199719254218452047 ) ) ;
#138371=CARTESIAN_POINT ( 'NONE',  ( 6.550524494058025837, 7.671308660269694712, -1.199719254218452047 ) ) ;
#138377=EDGE_CURVE ( 'NONE', #190177, #58907, #208600, .T. ) ;
#138386=CARTESIAN_POINT ( 'NONE',  ( -5.152980901645737077, 8.169505597632108262, -1.199719254218453823 ) ) ;
#138388=CARTESIAN_POINT ( 'NONE',  ( 5.180624093753221970, 9.058162186105164437, 0.000000000000000000 ) ) ;
#138397=CARTESIAN_POINT ( 'NONE',  ( -4.098307573080856692, 8.003385611894792362, 0.7998128361456352531 ) ) ;
#138401=CARTESIAN_POINT ( 'NONE',  ( -4.990809943606294929, 4.995235487061662205, -0.7216878364870338292 ) ) ;
#138404=CARTESIAN_POINT ( 'NONE',  ( -4.065465959251405081, 5.836405933916976707, -1.599625672291271394 ) ) ;
#138413=CARTESIAN_POINT ( 'NONE',  ( 0.3633361122992279646, 3.192526366011316341, 2.035233858735807644 ) ) ;
#138428=CARTESIAN_POINT ( 'NONE',  ( -6.140917232347002042, 6.129101290685087911, -0.7998128361456362523 ) ) ;
#138441=CARTESIAN_POINT ( 'NONE',  ( -6.529347706211431124, 6.814240946220119000, -0.5220719126654594922 ) ) ;
#138454=CARTESIAN_POINT ( 'NONE',  ( -6.493429226302317225, 6.540365283632955773, 0.7998128361456341429 ) ) ;
#138461=CARTESIAN_POINT ( 'NONE',  ( 5.668717623845194176, 9.627604637879139560, 0.000000000000000000 ) ) ;
#138468=CARTESIAN_POINT ( 'NONE',  ( -5.984739259312381598, 6.154819375939016624, 0.1731420012108849660 ) ) ;
#138472=CARTESIAN_POINT ( 'NONE',  ( 3.237364818613055473, 6.998952398349030268, -1.734723475976807094E-15 ) ) ;
#138480=CARTESIAN_POINT ( 'NONE',  ( 5.027041095616958444, 9.086908054853605421, 0.000000000000000000 ) ) ;
#138482=CARTESIAN_POINT ( 'NONE',  ( 4.681308178468477799, 8.683552984847038303, 0.000000000000000000 ) ) ;
#138496=CARTESIAN_POINT ( 'NONE',  ( 6.491225937077876651, 6.748298437306541331, 0.07656069123261090292 ) ) ;
#138498=CARTESIAN_POINT ( 'NONE',  ( 4.421367491832258523, 8.172362817197399210, 0.7216878364870257245 ) ) ;
#138505=CARTESIAN_POINT ( 'NONE',  ( -5.307090785106547415, 5.156303768904543894, -0.7998128361456362523 ) ) ;
#138513=VERTEX_POINT ( 'NONE', #74136 ) ;
#138516=CARTESIAN_POINT ( 'NONE',  ( -4.624739795592931912, 8.409630504918133909, -0.7216878364870338292 ) ) ;
#138520=CARTESIAN_POINT ( 'NONE',  ( 7.452141709366786770, 8.723195411463290583, 1.199719254218452047 ) ) ;
#138527=CARTESIAN_POINT ( 'NONE',  ( -6.966220764712148572, 6.002124920821316323, 2.420000000000000373 ) ) ;
#138537=CARTESIAN_POINT ( 'NONE',  ( 6.099189001301251523, 8.209082816308541197, 1.599625672291268286 ) ) ;
#138553=LINE ( 'NONE', #42130, #82362 ) ;
#138562=CARTESIAN_POINT ( 'NONE',  ( -6.482157434489847603, 6.770256554395555959, 0.2388210531332583819 ) ) ;
#138577=ORIENTED_EDGE ( 'NONE', *, *, #141509, .T. ) ;
#138578=CARTESIAN_POINT ( 'NONE',  ( 5.736508392357904107, 5.865217010605237924, 0.000000000000000000 ) ) ;
#138579=ORIENTED_EDGE ( 'NONE', *, *, #168152, .T. ) ;
#138584=CARTESIAN_POINT ( 'NONE',  ( -7.014364370223741929, 9.276787413384745662, -1.599625672291271394 ) ) ;
#138586=CARTESIAN_POINT ( 'NONE',  ( 7.095713291905693332, 9.371694488680407886, 1.599625672291268286 ) ) ;
#138590=CARTESIAN_POINT ( 'NONE',  ( -5.506019780925599960, 5.596313630600862510, 0.7216878364870257245 ) ) ;
#138620=CARTESIAN_POINT ( 'NONE',  ( 4.146814880933355596, 5.931313009212638931, 1.599625672291261402 ) ) ;
#138634=CARTESIAN_POINT ( 'NONE',  ( -4.800995793014949165, 8.615262501910491366, 0.7216878364870267237 ) ) ;
#138637=CARTESIAN_POINT ( 'NONE',  ( 6.933015448541703485, 9.181880338089085214, 1.599625672291268286 ) ) ;
#138642=CARTESIAN_POINT ( 'NONE',  ( -4.980641328173854632, 6.904110530993182948, 1.599625672291263179 ) ) ;
#138669=B_SPLINE_CURVE_WITH_KNOTS ( 'NONE', 3,
 ( #158825, #191298, #189184, #76493 ),
 .UNSPECIFIED., .F., .F.,
 ( 4, 4 ),
 ( 0.000000000000000000, 0.0003110688635154432429 ),
 .UNSPECIFIED. ) ;
#138685=CARTESIAN_POINT ( 'NONE',  ( 3.716343503921665459, 6.389465617000312569, -1.082531754730549967 ) ) ;
#138689=CARTESIAN_POINT ( 'NONE',  ( 4.540400682753764627, 6.905156770093001661, -1.249999994511372448 ) ) ;
#138692=CARTESIAN_POINT ( 'NONE',  ( -7.123883369337781879, 7.275895117174344229, 0.7998128361456341429 ) ) ;
#138693=CARTESIAN_POINT ( 'NONE',  ( -4.468294144155606773, 7.370704380560280100, 1.199719254218452935 ) ) ;
#138697=CARTESIAN_POINT ( 'NONE',  ( -6.631346530415505036, 7.869564052640446228, 1.082531754730549078 ) ) ;
#138698=CARTESIAN_POINT ( 'NONE',  ( 7.146556367734764770, 9.431011410480991231, 1.443375672974063439 ) ) ;
#138704=CARTESIAN_POINT ( 'NONE',  ( -5.015590482412729756, 4.816220082428420923, 0.000000000000000000 ) ) ;
#138712=CARTESIAN_POINT ( 'NONE',  ( -6.363572996767778100, 8.517530811019446091, -1.599625672291271394 ) ) ;
#138713=VERTEX_POINT ( 'NONE', #106683 ) ;
#138714=CARTESIAN_POINT ( 'NONE',  ( 4.893454165248502186, 8.027304163657891678, -0.9628252682179049282 ) ) ;
#138717=CARTESIAN_POINT ( 'NONE',  ( 6.392116398765105956, 6.567141947924169720, 2.438447736777272112 ) ) ;
#138719=CARTESIAN_POINT ( 'NONE',  ( 5.083381250481017410, 4.895309311841474553, 0.7998128361456352531 ) ) ;
#138725=CARTESIAN_POINT ( 'NONE',  ( 8.014278199453780616, 8.522615118883788199, 0.000000000000000000 ) ) ;
#138729=CARTESIAN_POINT ( 'NONE',  ( -5.887983850084758330, 10.09134126839936840, 0.7998128361456291469 ) ) ;
#138735=CARTESIAN_POINT ( 'NONE',  ( -1.298432343300637860E-14, 2.519999999999999130, -2.000000000000000000 ) ) ;
#138741=CARTESIAN_POINT ( 'NONE',  ( 5.996449078994045223, 10.21788403546024782, 0.7998128361456331437 ) ) ;
#138754=CARTESIAN_POINT ( 'NONE',  ( -0.1054627972275519465, 3.385846599571567417, -2.076146368081344118 ) ) ;
#138755=CARTESIAN_POINT ( 'NONE',  ( 6.410638904775656677, 6.895589754593423493, 0.7569561588358000304 ) ) ;
#138779=VERTEX_POINT ( 'NONE', #157532 ) ;
#138783=CARTESIAN_POINT ( 'NONE',  ( -6.605427497552981642, 6.764401258476403278, 0.1916688254133581959 ) ) ;
#138797=CARTESIAN_POINT ( 'NONE',  ( 3.553238514845298734, 7.337208092372121904, -0.2327671511505452484 ) ) ;
#138801=CARTESIAN_POINT ( 'NONE',  ( -4.796552484184649856, 8.818004674849227342, -0.7998128361456362523 ) ) ;
#138803=VERTEX_POINT ( 'NONE', #107768 ) ;
#138818=CARTESIAN_POINT ( 'NONE',  ( 3.549202351727371862, 7.362762853649070571, -0.7998128361456362523 ) ) ;
#138831=CARTESIAN_POINT ( 'NONE',  ( 6.086061792568233209, 7.019478939793144967, 0.9900148145245997178 ) ) ;
#138849=CARTESIAN_POINT ( 'NONE',  ( -3.318713740295064163, 7.093859473644694269, 0.000000000000000000 ) ) ;
#138851=CARTESIAN_POINT ( 'NONE',  ( 4.061549535745618833, 6.896169004081968090, -1.199719254218452047 ) ) ;
#138854=CARTESIAN_POINT ( 'NONE',  ( -7.259464905474441565, 7.434073576000447048, -0.7998128361456362523 ) ) ;
#138859=CARTESIAN_POINT ( 'NONE',  ( 6.821687566331318564, 7.987665577921906568, 1.199719254218452935 ) ) ;
#138864=CARTESIAN_POINT ( 'NONE',  ( -5.066182726705734218, 7.967045547422810792, 1.194666625917781611 ) ) ;
#138870=TOROIDAL_SURFACE ( 'NONE', #145850, 0.8299999999999999600, 0.08000000000000000167 ) ;
#138874=CARTESIAN_POINT ( 'NONE',  ( -5.939880696118548187, 6.102484698325975288, 0.000000000000000000 ) ) ;
#138884=CARTESIAN_POINT ( 'NONE',  ( 5.126391479742934187, 6.113783160189109722, -1.082531754730548412 ) ) ;
#138888=CARTESIAN_POINT ( 'NONE',  ( -5.074494633264801990, 9.142270515442742607, 0.7998128361456291469 ) ) ;
#138902=CARTESIAN_POINT ( 'NONE',  ( 3.464990776744291345, 6.200183785247111778, 1.199719254218452047 ) ) ;
#138930=CARTESIAN_POINT ( 'NONE',  ( -3.662110889467009578, 7.286563447771212232, 0.7216878364870338292 ) ) ;
#138955=CARTESIAN_POINT ( 'NONE',  ( -5.935437387732586778, 10.14670372898850381, -0.7998128361456362523 ) ) ;
#138961=CARTESIAN_POINT ( 'NONE',  ( -3.122120512896910505, 6.864500708346841229, 0.7998128361456352531 ) ) ;
#138966=ORIENTED_EDGE ( 'NONE', *, *, #130414, .F. ) ;
#138970=CARTESIAN_POINT ( 'NONE',  ( -4.329849954717889915, 6.144853928627882489, 1.599625672291270506 ) ) ;
#138972=CARTESIAN_POINT ( 'NONE',  ( 6.328358748234019338, 6.951510624437585939, -0.8854765018257749754 ) ) ;
#138976=CARTESIAN_POINT ( 'NONE',  ( 4.016958651398847557, 7.908478536599129249, -0.7998128361456362523 ) ) ;
#138981=CARTESIAN_POINT ( 'NONE',  ( -7.099629715411508890, 8.311931418515415615, 1.199719254218452047 ) ) ;
#138986=CARTESIAN_POINT ( 'NONE',  ( -2.972980823146582186, 6.690504403638126263, 0.000000000000000000 ) ) ;
#138992=CARTESIAN_POINT ( 'NONE',  ( 6.183927461164522299, 6.387205924212962849, 0.000000000000000000 ) ) ;
#138993=CARTESIAN_POINT ( 'NONE',  ( -6.116136693096208887, 6.308116694799912771, 0.7216878364870257245 ) ) ;
#138999=CARTESIAN_POINT ( 'NONE',  ( 4.228163802615382494, 6.026220084508304708, -1.599625672291269396 ) ) ;
#139006=CARTESIAN_POINT ( 'NONE',  ( 3.867818961648523235, 7.734482231890414283, 1.040834085586084257E-14 ) ) ;
#139010=CARTESIAN_POINT ( 'NONE',  ( 6.059925523928845870, 7.140772946495586915, 1.155538509043469997 ) ) ;
#139016=CARTESIAN_POINT ( 'NONE',  ( -0.4640281877397542942, 3.122791860410086606, 2.027579305719746205 ) ) ;
#139020=CARTESIAN_POINT ( 'NONE',  ( 5.027041095616958444, 9.086908054853605421, 0.000000000000000000 ) ) ;
#139031=CARTESIAN_POINT ( 'NONE',  ( 5.324837791525375508, 7.612559486139466536, 1.234112182050936646 ) ) ;
#139042=CARTESIAN_POINT ( 'NONE',  ( 4.892487020634524342, 4.880525410245029505, -1.277330582746047388E-09 ) ) ;
#139046=CARTESIAN_POINT ( 'NONE',  ( -5.610041701004606196, 9.767075427805856691, -0.7998128361456362523 ) ) ;
#139051=CARTESIAN_POINT ( 'NONE',  ( -4.434768960748669997, 5.005376996850392501, -0.9481656214291103169 ) ) ;
#139058=CARTESIAN_POINT ( 'NONE',  ( 6.398522151006641678, 6.429640362454684954, 0.000000000000000000 ) ) ;
#139066=CARTESIAN_POINT ( 'NONE',  ( -8.054952659850432184, 8.570068656013202002, 0.000000000000000000 ) ) ;
#139069=CARTESIAN_POINT ( 'NONE',  ( 3.878514461961128479, 6.682628084666728085, -1.199719254218448494 ) ) ;
#139072=CARTESIAN_POINT ( 'NONE',  ( 5.709392084686216506, 5.833581318321598985, -0.7216878364870458196 ) ) ;
#139084=CARTESIAN_POINT ( 'NONE',  ( -7.593975437430151132, 8.032261896522864930, -0.7216878364870338292 ) ) ;
#139085=CARTESIAN_POINT ( 'NONE',  ( 6.211043768836181478, 7.379210830797944709, 1.082531754730549967 ) ) ;
#139095=CARTESIAN_POINT ( 'NONE',  ( -4.125423880308188629, 8.035021303660014880, -0.7998128361456481317 ) ) ;
#139096=CARTESIAN_POINT ( 'NONE',  ( -5.953438850176548947, 9.959779401932374654, 0.000000000000000000 ) ) ;
#139097=CARTESIAN_POINT ( 'NONE',  ( 6.170369307550815030, 8.292126506933040986, 1.443375672974064550 ) ) ;
#139108=CARTESIAN_POINT ( 'NONE',  ( -4.736138090107036902, 8.221507128720061175, -0.6901939221467829899 ) ) ;
#139111=CARTESIAN_POINT ( 'NONE',  ( 3.445180431648313224, 7.033477913649446300, 0.7216878364870257245 ) ) ;
#139116=CARTESIAN_POINT ( 'NONE',  ( -5.284646014276622950, 9.387447126623207794, -0.7998128361456362523 ) ) ;
#139129=CARTESIAN_POINT ( 'NONE',  ( 6.378184920586140727, 6.405913593630768510, 0.000000000000000000 ) ) ;
#139165=CARTESIAN_POINT ( 'NONE',  ( 6.048345925472183637, 8.149765894507963182, 1.443375672974065660 ) ) ;
#139170=CARTESIAN_POINT ( 'NONE',  ( 5.790741006368192778, 8.809596036521288198, -1.082531754730548412 ) ) ;
#139194=EDGE_CURVE ( 'NONE', #162079, #185175, #15507, .T. ) ;
#139195=CARTESIAN_POINT ( 'NONE',  ( -4.329849954717889915, 6.144853928627882489, 1.599625672291270506 ) ) ;
#139197=CARTESIAN_POINT ( 'NONE',  ( 6.224601922005513543, 7.395028676162137771, -1.082531754730548412 ) ) ;
#139203=CARTESIAN_POINT ( 'NONE',  ( -7.587723245503481095, 8.881373870289390737, 1.199719254218452047 ) ) ;
#139207=CARTESIAN_POINT ( 'NONE',  ( -7.322812365156824654, 8.676274193172000437, 1.082531754730549078 ) ) ;
#139210=CARTESIAN_POINT ( 'NONE',  ( -5.912237504011027767, 9.055304967058290799, 1.199719254218454489 ) ) ;
#139216=CARTESIAN_POINT ( 'NONE',  ( -5.632486471834530661, 5.535932070087196344, -0.7998128361456362523 ) ) ;
#139227=CARTESIAN_POINT ( 'NONE',  ( 2.993041990875914493, 6.420974562437304911, 0.3677586026352899218 ) ) ;
#139229=CARTESIAN_POINT ( 'NONE',  ( -4.014622883422322985, 7.697827440719083647, -0.7216878364870458196 ) ) ;
#139230=ORIENTED_EDGE ( 'NONE', *, *, #112332, .T. ) ;
#139231=CARTESIAN_POINT ( 'NONE',  ( -6.414416072596857532, 6.656109304217339151, -0.7216878364870338292 ) ) ;
#139233=CARTESIAN_POINT ( 'NONE',  ( 6.384963997392946844, 6.413822516572072807, 0.7998128361456352531 ) ) ;
#139234=CARTESIAN_POINT ( 'NONE',  ( -5.336015975430226099, 8.383046517047350932, -1.199719254218453823 ) ) ;
#139236=CARTESIAN_POINT ( 'NONE',  ( -6.740338644649361832, 7.892758502626242567, -1.199719254218452047 ) ) ;
#139258=CARTESIAN_POINT ( 'NONE',  ( 5.528692779322568640, 9.672168352510192690, 0.7998128361456341429 ) ) ;
#139298=CARTESIAN_POINT ( 'NONE',  ( 5.899733120602060232, 6.912052057904395141, -1.199719254218452047 ) ) ;
#139301=CARTESIAN_POINT ( 'NONE',  ( -3.654804927335652209, 6.421633627603656080, 1.199719254218452935 ) ) ;
#139316=CARTESIAN_POINT ( 'NONE',  ( 4.583538449871731757, 7.505156070562471804, 1.199719254218451159 ) ) ;
#139323=CARTESIAN_POINT ( 'NONE',  ( -6.912678218121246942, 9.158153569265168770, 1.599625672291269396 ) ) ;
#139328=CARTESIAN_POINT ( 'NONE',  ( 5.899733120602060232, 6.912052057904395141, -1.199719254218452047 ) ) ;
#139339=CARTESIAN_POINT ( 'NONE',  ( 6.319508997745523438, 9.426492026461511742, -1.082531754730548412 ) ) ;
#139340=CARTESIAN_POINT ( 'NONE',  ( -4.014622883422329203, 6.737458226417744278, -1.082531754730546636 ) ) ;
#139341=CARTESIAN_POINT ( 'NONE',  ( -5.936491157937300756, 8.019268665717216749, 1.599625672291263179 ) ) ;
#139353=CARTESIAN_POINT ( 'NONE',  ( 4.420840606507738357, 7.315341919971147355, 1.199719254218451159 ) ) ;
#139354=CARTESIAN_POINT ( 'NONE',  ( 5.200434439293556643, 8.224868058221247225, -1.199719254218452047 ) ) ;
#139357=CARTESIAN_POINT ( 'NONE',  ( 7.038618024149998043, 8.240751112043669835, -1.199719254218452047 ) ) ;
#139371=CARTESIAN_POINT ( 'NONE',  ( 5.461903044330952639, 7.609029316319980474, -1.335476589331906494 ) ) ;
#139374=CARTESIAN_POINT ( 'NONE',  ( 3.739016502318667445, 7.584212696005614873, 0.7998128361456271485 ) ) ;
#139378=CARTESIAN_POINT ( 'NONE',  ( 4.411198876399872404, 6.239761003923544713, -1.599625672291273171 ) ) ;
#139384=CARTESIAN_POINT ( 'NONE',  ( 5.820193082016415609, 10.01225203898631655, 0.000000000000000000 ) ) ;
#139388=CARTESIAN_POINT ( 'NONE',  ( 5.804299160426222848, 7.865044668620976509, -1.443375672974078761 ) ) ;
#139390=CARTESIAN_POINT ( 'NONE',  ( -5.336015975430226099, 8.383046517047350932, -1.199719254218453823 ) ) ;
#139392=CARTESIAN_POINT ( 'NONE',  ( 6.021229618244865023, 10.03886863134542828, -0.7216878364870458196 ) ) ;
#139403=CARTESIAN_POINT ( 'NONE',  ( -2.810282979782591006, 6.500690253046801814, 0.000000000000000000 ) ) ;
#139414=CARTESIAN_POINT ( 'NONE',  ( 0.1083990404229777937, 3.398882113126670657, -2.078799743937121303 ) ) ;
#139441=CARTESIAN_POINT ( 'NONE',  ( 4.380693030546916944, 6.204170850428461392, 1.443375672974058777 ) ) ;
#139455=CARTESIAN_POINT ( 'NONE',  ( -4.274563570058511175, 8.209017608368725405, 0.000000000000000000 ) ) ;
#139457=CARTESIAN_POINT ( 'NONE',  ( 7.634649897826745857, 8.079715433652276957, 0.7216878364870267237 ) ) ;
#139470=CARTESIAN_POINT ( 'NONE',  ( -4.878955176071358757, 6.785476686873604280, -1.599625672291271394 ) ) ;
#139475=CARTESIAN_POINT ( 'NONE',  ( -3.336715202739028552, 6.906935146588564223, 0.7216878364870338292 ) ) ;
#139479=CARTESIAN_POINT ( 'NONE',  ( -4.472210567661380587, 6.310941310395290493, 1.599625672291270506 ) ) ;
#139502=CARTESIAN_POINT ( 'NONE',  ( -5.492988512192097161, 6.437516681426083132, 1.199719254218452935 ) ) ;
#139504=CARTESIAN_POINT ( 'NONE',  ( -3.546339698426324460, 6.295090860542775779, -1.199719254218450271 ) ) ;
#139514=CARTESIAN_POINT ( 'NONE',  ( -6.581660514134937578, 6.779899958900003298, -0.3344319070191399401 ) ) ;
#139529=CARTESIAN_POINT ( 'NONE',  ( -4.633854640820660009, 8.628190524257904670, -0.7998128361456362523 ) ) ;
#139537=CARTESIAN_POINT ( 'NONE',  ( 5.682275777458829502, 9.643422483761748154, 0.7216878364870317197 ) ) ;
#139538=DIRECTION ( 'NONE',  ( -0.000000000000000000, -1.000000000000000000, -0.000000000000000000 ) ) ;
#139549=CARTESIAN_POINT ( 'NONE',  ( 4.573896719763862251, 6.429575154514868274, -1.599625672291273171 ) ) ;
#139557=CARTESIAN_POINT ( 'NONE',  ( 7.686546744304875389, 7.932335721302671949, 0.7998128361456291469 ) ) ;
#139559=CARTESIAN_POINT ( 'NONE',  ( 6.180537922983273091, 8.303989891604203422, -1.599625672291281386 ) ) ;
#139572=CARTESIAN_POINT ( 'NONE',  ( 6.151318917739748038, 6.974181327834800825, -0.9227930848511676221 ) ) ;
#139574=CARTESIAN_POINT ( 'NONE',  ( 4.882344714696929877, 8.710169577206153591, -0.7216878364870458196 ) ) ;
#139582=CARTESIAN_POINT ( 'NONE',  ( -4.065465959251405081, 5.836405933916976707, -1.599625672291271394 ) ) ;
#139583=CARTESIAN_POINT ( 'NONE',  ( 3.588273936444265289, 7.344317902764286643, -0.3372145678562175064 ) ) ;
#139590=VERTEX_POINT ( 'NONE', #67443 ) ;
#139594=CARTESIAN_POINT ( 'NONE',  ( -6.265276382846530545, 6.482112999508623297, 0.000000000000000000 ) ) ;
#139598=CARTESIAN_POINT ( 'NONE',  ( 6.373214726875630731, 9.593111727067046957, 1.199719254218452047 ) ) ;
#139606=DIRECTION ( 'NONE',  ( -0.6029061840396265914, -0.7978120914393163066, 0.000000000000000000 ) ) ;
#139617=CARTESIAN_POINT ( 'NONE',  ( 5.342795052237045539, 8.390955439988655229, -1.199719254218450271 ) ) ;
#139635=ORIENTED_EDGE ( 'NONE', *, *, #64317, .F. ) ;
#139636=CARTESIAN_POINT ( 'NONE',  ( -5.641074431737709283, 8.738948049406083385, -1.199719254218452047 ) ) ;
#139641=( BOUNDED_CURVE ( )  B_SPLINE_CURVE ( 2, ( #152701, #186251, #37886, #103964, #41108, #123501, #206770 ),
 .UNSPECIFIED., .F., .T. ) 
 B_SPLINE_CURVE_WITH_KNOTS ( ( 3, 2, 2, 3 ),
 ( 0.4499999999999996780, 0.4583333333333332038, 0.4666666666666668406, 0.4750000000000003664 ),
 .UNSPECIFIED. ) 
 CURVE ( )  GEOMETRIC_REPRESENTATION_ITEM ( )  RATIONAL_B_SPLINE_CURVE ( ( 1.000000000000005329, 0.8660254037844333785, 1.000000000000000000, 0.8660254037844387076, 1.000000000000000000, 0.8660254037844324904, 1.000000000000006217 ) ) 
 REPRESENTATION_ITEM ( '' )  );
#139645=EDGE_CURVE ( 'NONE', #111396, #84144, #133453, .T. ) ;
#139660=CARTESIAN_POINT ( 'NONE',  ( 3.282482588284323821, 6.843663763058119187, 0.7216878364870257245 ) ) ;
#139666=CARTESIAN_POINT ( 'NONE',  ( 8.011942431032855083, 8.311964022485323511, 0.7998128361456291469 ) ) ;
#139670=CARTESIAN_POINT ( 'NONE',  ( -3.526529353330350336, 7.128384988945109413, -0.7216878364870458196 ) ) ;
#139673=ORIENTED_EDGE ( 'NONE', *, *, #122982, .F. ) ;
#139685=AXIS2_PLACEMENT_3D ( 'NONE', #22004, #171492, #172573 ) ;
#139701=CARTESIAN_POINT ( 'NONE',  ( 5.890091390494168522, 5.836471141856793388, 0.000000000000000000 ) ) ;
#139712=CARTESIAN_POINT ( 'NONE',  ( -5.912764389335557702, 8.951956649983198844, 1.082531754730550855 ) ) ;
#139715=CARTESIAN_POINT ( 'NONE',  ( 6.393551957296131683, 9.616838495890963401, 1.199719254218452047 ) ) ;
#139732=CARTESIAN_POINT ( 'NONE',  ( 3.390420931869152721, 6.113185632892752075, -1.199719254218452047 ) ) ;
#139734=CARTESIAN_POINT ( 'NONE',  ( -2.875737979874388284, 6.369128386579808954, -0.7216878364870458196 ) ) ;
#139738=DIRECTION ( 'NONE',  ( -0.6507913734559650498, -0.7592566023652995710, 0.000000000000000000 ) ) ;
#139765=CARTESIAN_POINT ( 'NONE',  ( -7.618755976236585958, 7.853246491889623648, 0.000000000000000000 ) ) ;
#139768=CARTESIAN_POINT ( 'NONE',  ( -5.529746549527323474, 7.544733289238903851, -1.599625672291271394 ) ) ;
#139773=CARTESIAN_POINT ( 'NONE',  ( -6.089020385868856522, 9.157588645938716354, -1.082531754730549967 ) ) ;
#139779=CARTESIAN_POINT ( 'NONE',  ( -7.937372586157736443, 8.224965870130965584, 0.7998128361456341429 ) ) ;
#139787=CARTESIAN_POINT ( 'NONE',  ( -6.770317605177755382, 8.992066187497757213, 1.599625672291269396 ) ) ;
#139789=CARTESIAN_POINT ( 'NONE',  ( 5.318333368960210805, 7.618274611128187601, -1.232678415538956518 ) ) ;
#139794=CARTESIAN_POINT ( 'NONE',  ( 3.223806664999388172, 6.983134552466421674, -0.7998128361456362523 ) ) ;
#139816=CARTESIAN_POINT ( 'NONE',  ( 6.047819040147648373, 9.213483425884394507, 1.199719254218452047 ) ) ;
#139825=DIRECTION ( 'NONE',  ( 0.7592566023653005702, -0.6507913734559639396, 0.000000000000000000 ) ) ;
#139832=CARTESIAN_POINT ( 'NONE',  ( 5.644368669187761256, 7.458116220610145675, 1.329639117314229235 ) ) ;
#139833=CARTESIAN_POINT ( 'NONE',  ( -5.275531169048922386, 5.327410250078064458, -0.7216878364870338292 ) ) ;
#139858=CARTESIAN_POINT ( 'NONE',  ( 5.415556014015861841, 5.282846535965431300, -0.7998128361456481317 ) ) ;
#139876=CARTESIAN_POINT ( 'NONE',  ( -5.712781623311813384, 7.758274208654143855, -1.599625672291271394 ) ) ;
#139893=CARTESIAN_POINT ( 'NONE',  ( 5.411639590510088027, 6.342609606130419131, -1.199719254218452047 ) ) ;
#139905=CARTESIAN_POINT ( 'NONE',  ( 5.794989345469916842, 7.230977472937116346, 1.182549002416101835 ) ) ;
#139907=CARTESIAN_POINT ( 'NONE',  ( -6.329050364910258075, 6.923295760524523779, 0.8374253472341108839 ) ) ;
#139926=ORIENTED_EDGE ( 'NONE', *, *, #3121, .T. ) ;
#139928=CARTESIAN_POINT ( 'NONE',  ( -3.467853430045390706, 7.267855778353407459, 0.7998128361456352531 ) ) ;
#139930=CARTESIAN_POINT ( 'NONE',  ( 5.682802662783380754, 6.658966523782627434, 1.199719254218452935 ) ) ;
#139933=CARTESIAN_POINT ( 'NONE',  ( -6.771371375382467583, 6.864631124226471037, -0.7998128361456362523 ) ) ;
#139936=CARTESIAN_POINT ( 'NONE',  ( 5.203297092594585393, 9.292540051327542017, 0.7998128361456341429 ) ) ;
#139941=CARTESIAN_POINT ( 'NONE',  ( -5.543378919943204863, 7.538303290789565736, -1.349654061105177050 ) ) ;
#139950=CARTESIAN_POINT ( 'NONE',  ( -5.777182852754558340, 5.912670547734647286, 0.000000000000000000 ) ) ;
#139961=CARTESIAN_POINT ( 'NONE',  ( 4.746763178560254204, 6.631252689777363152, 1.443375672974065660 ) ) ;
#139965=CARTESIAN_POINT ( 'NONE',  ( -5.641074431737709283, 8.738948049406083385, -1.199719254218452047 ) ) ;
#139970=ORIENTED_EDGE ( 'NONE', *, *, #19832, .F. ) ;
#139975=CARTESIAN_POINT ( 'NONE',  ( -4.556949027968976829, 5.449433633119473264, 1.082531754730549078 ) ) ;
#139980=CARTESIAN_POINT ( 'NONE',  ( 4.543917759235442944, 5.330267469643351852, 1.199719254218452935 ) ) ;
#140007=CARTESIAN_POINT ( 'NONE',  ( -5.560252395380252288, 7.580323442733986283, 1.443375672974058777 ) ) ;
#140030=CARTESIAN_POINT ( 'NONE',  ( -5.759181390754928742, 9.941071732514568993, 0.000000000000000000 ) ) ;
#140031=CARTESIAN_POINT ( 'NONE',  ( -5.002032328799064231, 4.800402236545811441, -0.7998128361456362523 ) ) ;
#140036=CARTESIAN_POINT ( 'NONE',  ( -4.553559489343377287, 6.405848385690952718, -1.599625672291271394 ) ) ;
#140040=ORIENTED_EDGE ( 'NONE', *, *, #23441, .T. ) ;
#140044=CARTESIAN_POINT ( 'NONE',  ( -3.871735385154307263, 6.674719161725423788, -1.199719254218450271 ) ) ;
#140046=CARTESIAN_POINT ( 'NONE',  ( 5.620636616140949116, 7.477306742562066511, -1.332712173395997013 ) ) ;
#140050=CARTESIAN_POINT ( 'NONE',  ( 6.066347387471824781, 6.042103138330730872, -0.7998128361456481317 ) ) ;
#140053=ADVANCED_FACE ( 'NONE', ( #179136 ), #145631, .T. ) ;
#140054=EDGE_CURVE ( 'NONE', #107579, #92970, #155450, .T. ) ;
#140057=CARTESIAN_POINT ( 'NONE',  ( -6.668631453075260396, 8.873432343378178544, -1.599625672291271394 ) ) ;
#140062=CARTESIAN_POINT ( 'NONE',  ( -3.688700311369816909, 6.461178242310183784, -1.199719254218450271 ) ) ;
#140067=CARTESIAN_POINT ( 'NONE',  ( 6.672020991256494504, 6.956648375986938859, 0.000000000000000000 ) ) ;
#140068=CARTESIAN_POINT ( 'NONE',  ( -5.939880696118548187, 6.102484698325975288, 0.000000000000000000 ) ) ;
#140071=CARTESIAN_POINT ( 'NONE',  ( -4.339491684825780737, 7.220434844675483355, -1.199719254218455378 ) ) ;
#140074=CARTESIAN_POINT ( 'NONE',  ( 3.217027588192558074, 6.975225629525113824, -1.734723475976807094E-15 ) ) ;
#140078=VECTOR ( 'NONE', #202826, 1000.000000000000000 ) ;
#140079=CARTESIAN_POINT ( 'NONE',  ( -10.17567228521069467, -0.02076350362892331880, -2.420000000000000373 ) ) ;
#140085=CARTESIAN_POINT ( 'NONE',  ( 6.044612043767858545, 7.151903759757407109, 1.166429756139725660 ) ) ;
#140094=CARTESIAN_POINT ( 'NONE',  ( 6.496291879603339758, 7.608037276739255006, 1.199719254218452935 ) ) ;
#140104=CARTESIAN_POINT ( 'NONE',  ( 6.244837129360077732, 6.910362811036335096, 0.8058565020967979331 ) ) ;
#140115=CARTESIAN_POINT ( 'NONE',  ( -5.012700657095048307, 7.921469694614043711, 1.075264880722737182 ) ) ;
#140124=CARTESIAN_POINT ( 'NONE',  ( -5.759181390754928742, 9.941071732514568993, 0.000000000000000000 ) ) ;
#140137=CARTESIAN_POINT ( 'NONE',  ( 5.691390622686558487, 9.861982503101517139, 0.7998128361456341429 ) ) ;
#140142=CARTESIAN_POINT ( 'NONE',  ( -5.608664280835665927, 5.616119181489428236, -0.4078810573515170845 ) ) ;
#140146=CARTESIAN_POINT ( 'NONE',  ( 3.607351389687783794, 6.366271167014519783, 1.199719254218451159 ) ) ;
#140149=CARTESIAN_POINT ( 'NONE',  ( 4.706088717274895750, 6.583799151611112954, 1.443375672974065660 ) ) ;
#140157=CARTESIAN_POINT ( 'NONE',  ( -6.492003545397249553, 6.763960095814848472, -0.1687977717132038147 ) ) ;
#140164=CARTESIAN_POINT ( 'NONE',  ( -7.458393901293492334, 7.874083437696761223, 0.7216878364870317197 ) ) ;
#140165=CARTESIAN_POINT ( 'NONE',  ( 3.553118775233146120, 6.302999783484076524, -1.199719254218453823 ) ) ;
#140178=CARTESIAN_POINT ( 'NONE',  ( -6.445975688654487001, 6.485002823043819475, -0.7998128361456362523 ) ) ;
#140179=CARTESIAN_POINT ( 'NONE',  ( -4.098307573080856692, 8.003385611894792362, 0.7998128361456352531 ) ) ;
#140181=CARTESIAN_POINT ( 'NONE',  ( 6.414416072596830887, 8.576847732820027659, -1.443375672974078761 ) ) ;
#140182=AXIS2_PLACEMENT_3D ( 'NONE', #86797, #152863, #187487 ) ;
#140193=CARTESIAN_POINT ( 'NONE',  ( -6.171773824192762881, 6.975641918443353795, -0.9092550976456583722 ) ) ;
#140194=LINE ( 'NONE', #109871, #32725 ) ;
#140197=CARTESIAN_POINT ( 'NONE',  ( 4.258669648468278446, 7.022179452304728287, 1.082531754730549078 ) ) ;
#140203=CARTESIAN_POINT ( 'NONE',  ( -5.596483547390937119, 9.751257581923240991, 0.000000000000000000 ) ) ;
#140219=CARTESIAN_POINT ( 'NONE',  ( 4.369470645354133431, 8.319742529546998000, 0.7998128361456271485 ) ) ;
#140235=CARTESIAN_POINT ( 'NONE',  ( 2.547265342226494947E-16, 1.016439536705160407E-16, -2.080000000000000071 ) ) ;
#140242=CARTESIAN_POINT ( 'NONE',  ( 3.719872605471085336, 6.605953636083950364, 2.499999999999999556 ) ) ;
#140255=CARTESIAN_POINT ( 'NONE',  ( 5.831415467653547680, 8.857049574687536619, -1.082531754730548412 ) ) ;
#140261=CARTESIAN_POINT ( 'NONE',  ( 6.278834536460164983, 9.379038488295265097, -1.082531754730548412 ) ) ;
#140289=CARTESIAN_POINT ( 'NONE',  ( -3.305155586681401303, 7.078041627762083898, 0.7998128361456352531 ) ) ;
#140291=CARTESIAN_POINT ( 'NONE',  ( 5.519577934094852978, 7.532869904567736974, 1.443375672974064550 ) ) ;
#140297=CARTESIAN_POINT ( 'NONE',  ( -7.075376061485238566, 9.347967719856493218, 1.599625672291269396 ) ) ;
#140302=CARTESIAN_POINT ( 'NONE',  ( -7.268579750702160780, 8.613002809641560731, -1.082531754730549967 ) ) ;
#140304=CARTESIAN_POINT ( 'NONE',  ( -4.495411241332101682, 8.048790631822507535, 2.444653990452268832 ) ) ;
#140305=CARTESIAN_POINT ( 'NONE',  ( -7.262327558775498737, 8.501745569106741840, 1.199719254218452047 ) ) ;
#140309=CARTESIAN_POINT ( 'NONE',  ( -5.984998465789844069, 5.947196063035064206, 0.7998128361456281477 ) ) ;
#140321=CARTESIAN_POINT ( 'NONE',  ( -3.824808732831001201, 7.476377598362539345, 0.7216878364870338292 ) ) ;
#140323=CARTESIAN_POINT ( 'NONE',  ( -6.916067756302494374, 7.241369601873926420, 0.000000000000000000 ) ) ;
#140324=CARTESIAN_POINT ( 'NONE',  ( 6.737475991348287785, 6.825086509519945999, -0.7998128361456481317 ) ) ;
#140325=CARTESIAN_POINT ( 'NONE',  ( -7.117104292530948229, 7.267986194233038155, -0.7998128361456362523 ) ) ;
#140337=ORIENTED_EDGE ( 'NONE', *, *, #44262, .F. ) ;
#140346=CARTESIAN_POINT ( 'NONE',  ( 5.365994935958575240, 9.482354201918870018, 0.7998128361456341429 ) ) ;
#140382=CARTESIAN_POINT ( 'NONE',  ( 6.222266154028957885, 6.224008365980749247, 0.7998128361456352531 ) ) ;
#140385=CARTESIAN_POINT ( 'NONE',  ( -5.015590482412729756, 4.816220082428420923, 0.000000000000000000 ) ) ;
#140388=CARTESIAN_POINT ( 'NONE',  ( -5.600926855776882540, 8.588146194164741232, -1.082531754730549967 ) ) ;
#140400=CARTESIAN_POINT ( 'NONE',  ( 5.996449078994045223, 10.21788403546024782, 0.7998128361456331437 ) ) ;
#140401=CARTESIAN_POINT ( 'NONE',  ( 4.716257332707354699, 6.595662536282280719, -1.599625672291269396 ) ) ;
#140414=CARTESIAN_POINT ( 'NONE',  ( 6.235824307642648279, 6.239826211863360506, 0.000000000000000000 ) ) ;
#140417=CIRCLE ( 'NONE', #130110, 2.000000000000000000 ) ;
#140430=CARTESIAN_POINT ( 'NONE',  ( 7.539742822975472158, 7.968990512992423447, -0.7216878364870317197 ) ) ;
#140431=FACE_OUTER_BOUND ( 'NONE', #163034, .T. ) ;
#140432=CARTESIAN_POINT ( 'NONE',  ( -5.738844160334429567, 9.917344963690652548, 0.000000000000000000 ) ) ;
#140444=CARTESIAN_POINT ( 'NONE',  ( 6.964048179274811012, 8.153752959689313684, 1.199719254218452047 ) ) ;
#140446=CARTESIAN_POINT ( 'NONE',  ( 4.342354338126830804, 8.288106837781779035, -0.7998128361456381397 ) ) ;
#140447=CARTESIAN_POINT ( 'NONE',  ( 6.176621499477501054, 9.363752961769195693, -1.199719254218452047 ) ) ;
#140450=CARTESIAN_POINT ( 'NONE',  ( 5.854088466050551887, 10.05179665369283981, 0.7998128361456341429 ) ) ;
#140467=CARTESIAN_POINT ( 'NONE',  ( 5.259637247458703868, 5.100941308315409373, 0.000000000000000000 ) ) ;
#140469=CARTESIAN_POINT ( 'NONE',  ( -4.462568837553487100, 5.235360394347691404, -1.199719254218453823 ) ) ;
#140472=CARTESIAN_POINT ( 'NONE',  ( 4.199993725183334803, 8.122019456014369254, -0.7998128361456362523 ) ) ;
#140477=CARTESIAN_POINT ( 'NONE',  ( 6.994027139803230320, 9.253060644560830994, -1.599625672291267398 ) ) ;
#140481=CARTESIAN_POINT ( 'NONE',  ( 6.563555762791525972, 6.830105609444471426, -0.7216878364870458196 ) ) ;
#140483=CARTESIAN_POINT ( 'NONE',  ( -4.956387674247580755, 7.940146832334256111, 1.199719254218452935 ) ) ;
#140485=CARTESIAN_POINT ( 'NONE',  ( 5.740951700743842423, 5.662474837148078421, -0.7998128361456481317 ) ) ;
#140492=CARTESIAN_POINT ( 'NONE',  ( -5.853218251105561265, 6.233033923027780254, -0.5979115183833558778 ) ) ;
#140493=B_SPLINE_CURVE_WITH_KNOTS ( 'NONE', 3,
 ( #65499, #131647, #49297, #115412, #102283, #118602, #54607, #133764, #151062, #132695, #53538, #37288, #183533, #120756, #153175, #149986 ),
 .UNSPECIFIED., .F., .F.,
 ( 4, 3, 3, 3, 3, 4 ),
 ( 0.000000000000000000, 2.533473342638980266E-05, 5.061406379858541306E-05, 7.673069672129149185E-05, 0.0001048028779199227441, 0.0001300696341146172241 ),
 .UNSPECIFIED. ) ;
#140496=CARTESIAN_POINT ( 'NONE',  ( -4.604929450496978660, 5.401447776115099408, -1.199719254218453823 ) ) ;
#140524=CARTESIAN_POINT ( 'NONE',  ( 4.923019175537949543, 4.916146257648610352, 0.000000000000000000 ) ) ;
#140526=ORIENTED_EDGE ( 'NONE', *, *, #72682, .F. ) ;
#140531=CARTESIAN_POINT ( 'NONE',  ( 3.404505970362959655, 6.986024375483197879, 0.7216878364870257245 ) ) ;
#140544=CARTESIAN_POINT ( 'NONE',  ( -6.286140498591554326, 7.362860665558790707, 1.199719254218452047 ) ) ;
#140547=CARTESIAN_POINT ( 'NONE',  ( 6.658462837642791676, 8.861568958707010779, 1.443375672974063439 ) ) ;
#140550=CARTESIAN_POINT ( 'NONE',  ( -3.789102684798408838, 7.352775819508957866, -0.6979800873464858668 ) ) ;
#140557=CARTESIAN_POINT ( 'NONE',  ( -5.255720823952942489, 6.160704378480398979, -1.199719254218453823 ) ) ;
#140560=DIRECTION ( 'NONE',  ( -0.000000000000000000, -1.000000000000000000, -0.000000000000000000 ) ) ;
#140562=CARTESIAN_POINT ( 'NONE',  ( -5.004368097219957789, 5.011053332944274352, 0.000000000000000000 ) ) ;
#140567=CARTESIAN_POINT ( 'NONE',  ( -3.526002468005825286, 6.271364091718859335, -1.199719254218450271 ) ) ;
#140591=CARTESIAN_POINT ( 'NONE',  ( -4.796552484184649856, 8.818004674849227342, -0.7998128361456362523 ) ) ;
#140593=CARTESIAN_POINT ( 'NONE',  ( -5.327428015527048366, 5.180030537728460338, -0.7998128361456362523 ) ) ;
#140602=DIRECTION ( 'NONE',  ( 0.7592566023653005702, 0.6507913734559639396, 0.000000000000000000 ) ) ;
#140605=ORIENTED_EDGE ( 'NONE', *, *, #72682, .T. ) ;
#140616=CARTESIAN_POINT ( 'NONE',  ( -6.469175572376043348, 7.576401584974034265, 1.199719254218452047 ) ) ;
#140618=ORIENTED_EDGE ( 'NONE', *, *, #148050, .T. ) ;
#140624=CARTESIAN_POINT ( 'NONE',  ( 7.824464048418096951, 8.301165276008827476, -0.7216878364870317197 ) ) ;
#140633=CARTESIAN_POINT ( 'NONE',  ( 3.898851692381625877, 6.706354853490643642, -1.199719254218452047 ) ) ;
#140641=CARTESIAN_POINT ( 'NONE',  ( 5.875479466675786355, 7.948088359245467416, -1.599625672291283607 ) ) ;
#140643=CARTESIAN_POINT ( 'NONE',  ( 7.205232291019763480, 7.370802192470005565, -0.7998128361456341429 ) ) ;
#140656=CARTESIAN_POINT ( 'NONE',  ( 6.453003701063230402, 6.772902045581084884, 0.3391303328579304277 ) ) ;
#140658=CARTESIAN_POINT ( 'NONE',  ( 4.095971805104276164, 7.792734516014745871, 0.7216878364870257245 ) ) ;
#140665=CARTESIAN_POINT ( 'NONE',  ( -3.851398154733808088, 6.650992392901508232, -1.199719254218450271 ) ) ;
#140676=CARTESIAN_POINT ( 'NONE',  ( -5.424670858799220063, 9.342883411992149334, 0.000000000000000000 ) ) ;
#140680=CARTESIAN_POINT ( 'NONE',  ( 6.912678218121202534, 9.158153569265168770, 1.599625672291268286 ) ) ;
#140698=CARTESIAN_POINT ( 'NONE',  ( 7.015418140428412386, 7.149352350113456822, 0.7998128361456331437 ) ) ;
#140704=CARTESIAN_POINT ( 'NONE',  ( -3.797692425159308716, 7.444741906078900406, 0.000000000000000000 ) ) ;
#140716=CIRCLE ( 'NONE', #192466, 3.970406073902761790 ) ;
#140717=CARTESIAN_POINT ( 'NONE',  ( -7.435720902452096936, 7.639705572474380091, 0.000000000000000000 ) ) ;
#140739=DIRECTION ( 'NONE',  ( 0.000000000000000000, 0.000000000000000000, -1.000000000000000000 ) ) ;
#140740=CARTESIAN_POINT ( 'NONE',  ( 4.746763178560250651, 7.591621904078704297, 1.082531754730549078 ) ) ;
#140750=CARTESIAN_POINT ( 'NONE',  ( -4.502716413514310290, 6.346531463890372926, -1.443375672974066548 ) ) ;
#140769=CARTESIAN_POINT ( 'NONE',  ( -5.181866634007240791, 6.340624232048664766, 1.284222742053082733 ) ) ;
#140779=CARTESIAN_POINT ( 'NONE',  ( 3.528865121306874464, 7.339036084825155015, -0.7998128361456362523 ) ) ;
#140790=CARTESIAN_POINT ( 'NONE',  ( -5.777182853198894463, 9.754147405458438058, 0.7216878364870267237 ) ) ;
#140794=CARTESIAN_POINT ( 'NONE',  ( 8.188198428010544205, 8.517596018959260107, 0.000000000000000000 ) ) ;
#140810=CARTESIAN_POINT ( 'NONE',  ( 4.065465959251388206, 5.836405933916976707, -1.599625672291269396 ) ) ;
#140812=CARTESIAN_POINT ( 'NONE',  ( -4.828112100242303306, 4.805421336470338645, -0.7216878364870338292 ) ) ;
#140814=CARTESIAN_POINT ( 'NONE',  ( 5.194182247366869731, 7.153241603385088965, 1.443375672974064550 ) ) ;
#140844=CARTESIAN_POINT ( 'NONE',  ( -7.445362632559989535, 8.715286488521982733, 1.199719254218452047 ) ) ;
#140847=CARTESIAN_POINT ( 'NONE',  ( -6.557303570864871034, 7.679217583210999010, -1.199719254218452047 ) ) ;
#140852=CARTESIAN_POINT ( 'NONE',  ( -6.495764994278840021, 8.671754808115688107, 1.443375672974064550 ) ) ;
#140855=CARTESIAN_POINT ( 'NONE',  ( -3.156015896931072540, 6.904045323053366268, 0.000000000000000000 ) ) ;
#140858=CARTESIAN_POINT ( 'NONE',  ( -5.915100157312088491, 10.12297696016459092, -0.7998128361456362523 ) ) ;
#140867=CARTESIAN_POINT ( 'NONE',  ( -6.257970421159510188, 9.458660037064859694, 1.199719254218452047 ) ) ;
#140869=CARTESIAN_POINT ( 'NONE',  ( 5.631620320865258655, 7.357208097040313532, -1.234165276361798735 ) ) ;
#140874=CARTESIAN_POINT ( 'NONE',  ( 6.535912570239620578, 9.782925877658371405, 1.199719254218452047 ) ) ;
#140883=EDGE_CURVE ( 'NONE', #100853, #123093, #190763, .T. ) ;
#140897=CARTESIAN_POINT ( 'NONE',  ( 8.018721507839716267, 8.319872945426633137, -0.7998128361456341429 ) ) ;
#140912=CARTESIAN_POINT ( 'NONE',  ( 5.901825473515108555, 7.257632781371366804, 1.250113620240392631 ) ) ;
#140913=CARTESIAN_POINT ( 'NONE',  ( -4.841670253411603397, 5.781608396135871075, 1.082531754730549078 ) ) ;
#140926=EDGE_LOOP ( 'NONE', ( #159299, #183617, #147480 ) ) ;
#140934=CARTESIAN_POINT ( 'NONE',  ( -5.608178827873947725, 5.599964016548462986, -0.4038203069821116320 ) ) ;
#140941=CARTESIAN_POINT ( 'NONE',  ( 3.553118775233146120, 6.302999783484076524, -1.199719254218453823 ) ) ;
#140963=CARTESIAN_POINT ( 'NONE',  ( -5.284646014276622950, 9.387447126623207794, -0.7998128361456362523 ) ) ;
#140979=CARTESIAN_POINT ( 'NONE',  ( 4.224247379109608680, 7.085983154673295203, -1.199719254218452047 ) ) ;
#140989=CARTESIAN_POINT ( 'NONE',  ( 4.708566766960948335, 8.234178693335817201, 0.6429565889536159595 ) ) ;
#140991=B_SPLINE_CURVE_WITH_KNOTS ( 'NONE', 3,
 ( #152856, #203708, #170161, #55355, #187479, #86787, #6578, #171230, #53221, #87858 ),
 .UNSPECIFIED., .F., .F.,
 ( 4, 2, 2, 2, 4 ),
 ( 0.001366907522411799037, 0.001656827650609844034, 0.001946747778807889247, 0.002236667907005934243, 0.002526588035203979239 ),
 .UNSPECIFIED. ) ;
#140992=CARTESIAN_POINT ( 'NONE',  ( 5.220047253295719614, 7.706380104734268599, 1.202949228536150938 ) ) ;
#141012=CARTESIAN_POINT ( 'NONE',  ( -5.490125858891038213, 5.369844688319787451, -0.7998128361456362523 ) ) ;
#141014=CARTESIAN_POINT ( 'NONE',  ( 5.910428620914669473, 5.860197910680708944, 0.000000000000000000 ) ) ;
#141015=DIRECTION ( 'NONE',  ( 0.000000000000000000, 1.000000000000000000, 0.000000000000000000 ) ) ;
#141017=CARTESIAN_POINT ( 'NONE',  ( -4.938913097128142304, 8.984092056616635347, -0.7998128361456362523 ) ) ;
#141020=CARTESIAN_POINT ( 'NONE',  ( 7.526711554241970248, 8.810193563817646734, -1.199719254218452047 ) ) ;
#141027=CARTESIAN_POINT ( 'NONE',  ( -5.345048817422858534, 7.707963373851138833, -1.327269471787644317 ) ) ;
#141036=ADVANCED_FACE ( 'NONE', ( #147881 ), #48260, .F. ) ;
#141037=CARTESIAN_POINT ( 'NONE',  ( -4.109529958273628658, 7.808552361378938045, 0.7216878364870338292 ) ) ;
#141044=CARTESIAN_POINT ( 'NONE',  ( 4.570507181582611267, 8.346359121906111511, 0.000000000000000000 ) ) ;
#141049=CARTESIAN_POINT ( 'NONE',  ( -7.584860592202423035, 7.813701877183096833, -0.7998128361456362523 ) ) ;
#141058=CARTESIAN_POINT ( 'NONE',  ( -4.665414256878304577, 5.575976400180357118, -1.082531754730549967 ) ) ;
#141063=CARTESIAN_POINT ( 'NONE',  ( 3.386504508363381571, 7.172948703057747011, -0.7998128361456362523 ) ) ;
#141088=CARTESIAN_POINT ( 'NONE',  ( -5.139949633356594383, 9.010708648975750634, 0.000000000000000000 ) ) ;
#141091=EDGE_LOOP ( 'NONE', ( #117974, #54522, #160529, #28871, #31426, #65660, #145345, #194195 ) ) ;
#141103=ORIENTED_EDGE ( 'NONE', *, *, #43875, .F. ) ;
#141115=CARTESIAN_POINT ( 'NONE',  ( -3.323157048681004699, 6.891117300187535655, -0.7216878364870458196 ) ) ;
#141121=CARTESIAN_POINT ( 'NONE',  ( -4.472210567661380587, 6.310941310395290493, 1.599625672291270506 ) ) ;
#141131=CARTESIAN_POINT ( 'NONE',  ( -3.817502770699643388, 6.611447778194983194, 1.199719254218452935 ) ) ;
#141133=ORIENTED_EDGE ( 'NONE', *, *, #26463, .F. ) ;
#141134=CARTESIAN_POINT ( 'NONE',  ( 6.580239226864286195, 6.782991656975736028, -0.2881480849740332140 ) ) ;
#141138=CARTESIAN_POINT ( 'NONE',  ( 5.876533236880477240, 5.820653295974182129, 0.7998128361456352531 ) ) ;
#141142=CARTESIAN_POINT ( 'NONE',  ( -7.425025402139490360, 8.691559719698066289, 1.199719254218452047 ) ) ;
#141148=CARTESIAN_POINT ( 'NONE',  ( -4.339491684825780737, 7.220434844675483355, -1.199719254218455378 ) ) ;
#141155=CARTESIAN_POINT ( 'NONE',  ( 5.844973620822844218, 6.952128991449046502, 1.082531754730549967 ) ) ;
#141156=CARTESIAN_POINT ( 'NONE',  ( -5.600926855776894975, 6.667407765562058053, -1.082531754730549967 ) ) ;
#141162=CARTESIAN_POINT ( 'NONE',  ( 4.903208829997618423, 5.749440385532527564, -1.199719254218450271 ) ) ;
#141171=CARTESIAN_POINT ( 'NONE',  ( 5.184698244283005408, 7.856242361780820360, 1.254847465626233616 ) ) ;
#141181=CARTESIAN_POINT ( 'NONE',  ( 6.550524494058025837, 7.671308660269694712, -1.199719254218452047 ) ) ;
#141191=CARTESIAN_POINT ( 'NONE',  ( 4.798147134389644464, 8.131168186839138556, 0.8272934513729796047 ) ) ;
#141198=CARTESIAN_POINT ( 'NONE',  ( 5.332099551924443404, 9.442809587212341427, 0.000000000000000000 ) ) ;
#141202=CARTESIAN_POINT ( 'NONE',  ( -4.929275754869433257, 8.007250896656138650, 0.9949873637682864480 ) ) ;
#141209=CARTESIAN_POINT ( 'NONE',  ( -5.257529707049291900, 9.355811434857983500, 0.7998128361456291469 ) ) ;
#141217=B_SPLINE_CURVE_WITH_KNOTS ( 'NONE', 3,
 ( #140769, #208903, #75729, #192656 ),
 .UNSPECIFIED., .F., .F.,
 ( 4, 4 ),
 ( 0.000000000000000000, 0.0002445738358484001417 ),
 .UNSPECIFIED. ) ;
#141224=CARTESIAN_POINT ( 'NONE',  ( 6.282224075085741433, 8.422623735723785643, 1.599625672291268286 ) ) ;
#141228=CARTESIAN_POINT ( 'NONE',  ( -5.608757509019071108, 5.629766575892905855, -0.3787719694710602325 ) ) ;
#141230=CARTESIAN_POINT ( 'NONE',  ( -6.902509602688818191, 9.146290184594002781, -1.443375672974066548 ) ) ;
#141231=CARTESIAN_POINT ( 'NONE',  ( 4.390861645979372341, 6.216034235099629157, -1.599625672291269396 ) ) ;
#141234=CARTESIAN_POINT ( 'NONE',  ( 6.034787771414195312, 6.213209619504250547, -0.7216878364870458196 ) ) ;
#141249=CARTESIAN_POINT ( 'NONE',  ( -4.228163802615396705, 6.026220084508304708, -1.599625672291271394 ) ) ;
#141250=CARTESIAN_POINT ( 'NONE',  ( 3.444653546323793947, 6.176457016423196222, 1.199719254218451159 ) ) ;
#141252=ADVANCED_FACE ( 'NONE', ( #93813 ), #41856, .T. ) ;
#141257=ORIENTED_EDGE ( 'NONE', *, *, #208162, .T. ) ;
#141262=VERTEX_POINT ( 'NONE', #107199 ) ;
#141263=CARTESIAN_POINT ( 'NONE',  ( -5.692444392891315097, 7.734547439830227411, -1.599625672291271394 ) ) ;
#141264=CARTESIAN_POINT ( 'NONE',  ( -6.120580001926503755, 6.105374521861167914, -0.7998128361456362523 ) ) ;
#141266=CARTESIAN_POINT ( 'NONE',  ( 8.122743427918724279, 8.649157885426255632, 0.7216878364870267237 ) ) ;
#141279=CARTESIAN_POINT ( 'NONE',  ( -5.902949979233523159, 7.165898849449257924, -1.132310321155009847 ) ) ;
#141284=CARTESIAN_POINT ( 'NONE',  ( 5.234856708652235291, 5.279956712948652431, 0.7216878364870338292 ) ) ;
#141288=CARTESIAN_POINT ( 'NONE',  ( -6.282224075085783177, 8.422623735723785643, 1.599625672291269396 ) ) ;
#141289=EDGE_CURVE ( 'NONE', #195055, #137303, #143829, .T. ) ;
#141303=CARTESIAN_POINT ( 'NONE',  ( 4.844006021832467646, 8.873367135438366304, 0.000000000000000000 ) ) ;
#141319=CARTESIAN_POINT ( 'NONE',  ( 2.970855920843799236, 6.567331372341457474, 0.4599263646697975272 ) ) ;
#141333=AXIS2_PLACEMENT_3D ( 'NONE', #117567, #154278, #83927 ) ;
#141338=CARTESIAN_POINT ( 'NONE',  ( 7.526184669361807522, 7.953172667109813077, 0.000000000000000000 ) ) ;
#141342=CARTESIAN_POINT ( 'NONE',  ( 6.658462837642791676, 8.861568958707010779, 1.443375672974063439 ) ) ;
#141368=CARTESIAN_POINT ( 'NONE',  ( -4.248501033035892327, 6.049946853332221153, -1.599625672291271394 ) ) ;
#141370=CARTESIAN_POINT ( 'NONE',  ( 4.204437033569277560, 7.919277282557212416, 0.000000000000000000 ) ) ;
#141376=CARTESIAN_POINT ( 'NONE',  ( -6.140917232347002042, 6.129101290685087911, -0.7998128361456362523 ) ) ;
#141382=CARTESIAN_POINT ( 'NONE',  ( -5.496904935697871863, 5.377753611261092637, 0.7998128361456281477 ) ) ;
#141390=CARTESIAN_POINT ( 'NONE',  ( -4.390861645979385663, 6.216034235099629157, -1.599625672291271394 ) ) ;
#141402=CARTESIAN_POINT ( 'NONE',  ( -5.072158865288277418, 7.010880990960010273, 1.443375672974058777 ) ) ;
#141404=CARTESIAN_POINT ( 'NONE',  ( -6.265276382846530545, 6.482112999508623297, 0.000000000000000000 ) ) ;
#141405=CARTESIAN_POINT ( 'NONE',  ( 7.198453214212898743, 7.362893269528701268, 0.7998128361456291469 ) ) ;
#141406=CARTESIAN_POINT ( 'NONE',  ( -4.959250327548641479, 9.007818825440551791, -0.7998128361456362523 ) ) ;
#141415=ORIENTED_EDGE ( 'NONE', *, *, #392, .T. ) ;
#141427=CARTESIAN_POINT ( 'NONE',  ( 7.309781096423290769, 8.557108029695882578, 1.199719254218452935 ) ) ;
#141447=CARTESIAN_POINT ( 'NONE',  ( 5.228576739797318851, 7.698598165248225378, -1.206158463488806953 ) ) ;
#141452=CARTESIAN_POINT ( 'NONE',  ( 0.000000000000000000, 8.920000000000001705, 0.000000000000000000 ) ) ;
#141463=CARTESIAN_POINT ( 'NONE',  ( 6.038177310039780643, 8.137902509836795417, -1.599625672291283607 ) ) ;
#141465=CARTESIAN_POINT ( 'NONE',  ( -4.462568837553487100, 5.235360394347691404, -1.199719254218453823 ) ) ;
#141468=CARTESIAN_POINT ( 'NONE',  ( -5.411112705185557203, 9.327065566109540740, 0.7216878364870267237 ) ) ;
#141476=CARTESIAN_POINT ( 'NONE',  ( 0.000000000000000000, 1000.000000000000000, 0.000000000000000000 ) ) ;
#141479=CARTESIAN_POINT ( 'NONE',  ( 4.760848217054122422, 5.583353003765119560, -1.199719254218452047 ) ) ;
#141480=CARTESIAN_POINT ( 'NONE',  ( 7.178115983792402233, 7.339166500704784823, 0.7998128361456281477 ) ) ;
#141481=AXIS2_PLACEMENT_3D ( 'NONE', #58251, #42026, #6271 ) ;
#141494=CARTESIAN_POINT ( 'NONE',  ( 4.980641328173811999, 6.904110530993182948, 1.599625672291269396 ) ) ;
#141495=EDGE_LOOP ( 'NONE', ( #124769, #36145, #71401, #94180, #125911, #52746 ) ) ;
#141505=CARTESIAN_POINT ( 'NONE',  ( 7.404161286838808920, 8.771181268467660885, -1.082531754730548412 ) ) ;
#141506=CARTESIAN_POINT ( 'NONE',  ( -4.177320726786328819, 5.966903162707725805, -1.443375672974066548 ) ) ;
#141507=CARTESIAN_POINT ( 'NONE',  ( -7.259464905474441565, 7.434073576000447048, -0.7998128361456362523 ) ) ;
#141509=EDGE_CURVE ( 'NONE', #210733, #196836, #166544, .T. ) ;
#141520=CARTESIAN_POINT ( 'NONE',  ( 5.180097208873055692, 8.201141289397330780, -1.199719254218450271 ) ) ;
#141521=CARTESIAN_POINT ( 'NONE',  ( 5.352436782344940802, 9.466536356036257871, 0.000000000000000000 ) ) ;
#141524=CARTESIAN_POINT ( 'NONE',  ( 5.058600711230250013, 5.074324715956299414, -0.7216878364870458196 ) ) ;
#141539=CARTESIAN_POINT ( 'NONE',  ( 6.966220764712143243, 6.002124920821316323, -2.500000000000000444 ) ) ;
#141540=CARTESIAN_POINT ( 'NONE',  ( 4.167152111353856547, 5.955039778036558040, 1.599625672291262513 ) ) ;
#141542=CARTESIAN_POINT ( 'NONE',  ( -5.002032328799064231, 4.800402236545811441, -0.7998128361456362523 ) ) ;
#141545=CARTESIAN_POINT ( 'NONE',  ( 3.901714345682657292, 7.774026846596938434, 0.7998128361456271485 ) ) ;
#141549=CARTESIAN_POINT ( 'NONE',  ( 6.831329296439236032, 9.063246493969506545, -1.599625672291267398 ) ) ;
#141554=CARTESIAN_POINT ( 'NONE',  ( 5.343321937561575474, 8.287607122913563273, -1.082531754730548412 ) ) ;
#141557=CARTESIAN_POINT ( 'NONE',  ( -5.601453741101424022, 6.564059448486966986, -1.199719254218453823 ) ) ;
#141558=CARTESIAN_POINT ( 'NONE',  ( 3.878514461961128479, 6.682628084666728085, -1.199719254218448494 ) ) ;
#141565=CARTESIAN_POINT ( 'NONE',  ( -5.980802423990385641, 6.150226714305422782, 9.481663569016276247E-06 ) ) ;
#141568=CARTESIAN_POINT ( 'NONE',  ( -5.822300622425855110, 5.757381912443740646, 0.7998128361456281477 ) ) ;
#141602=CARTESIAN_POINT ( 'NONE',  ( 8.011942431032855083, 8.311964022485323511, 0.7998128361456291469 ) ) ;
#141614=CARTESIAN_POINT ( 'NONE',  ( -5.936491157937300756, 8.019268665717216749, 1.599625672291263179 ) ) ;
#141616=CARTESIAN_POINT ( 'NONE',  ( 7.146556367734771875, 8.470642196179646533, 1.082531754730549967 ) ) ;
#141619=CARTESIAN_POINT ( 'NONE',  ( -3.777115976154627131, 7.353790098116948393, -0.6809694117130314917 ) ) ;
#141625=CARTESIAN_POINT ( 'NONE',  ( -4.261005416444848315, 8.193199762486115034, 0.7998128361456352531 ) ) ;
#141626=AXIS2_PLACEMENT_3D ( 'NONE', #40436, #106537, #122838 ) ;
#141634=CARTESIAN_POINT ( 'NONE',  ( -3.363831509966363598, 5.978201624052440266, -1.082531754730548412 ) ) ;
#141637=CARTESIAN_POINT ( 'NONE',  ( -5.798046968499580345, 6.793418213784815585, 1.199719254218452935 ) ) ;
#141660=CARTESIAN_POINT ( 'NONE',  ( -7.442499979258930587, 7.647614495415686164, -0.7998128361456362523 ) ) ;
#141661=CARTESIAN_POINT ( 'NONE',  ( -4.260029445439585061, 7.236136616047151193, -2.500000000000000444 ) ) ;
#141662=CARTESIAN_POINT ( 'NONE',  ( -4.630991987519598396, 7.560518531151607213, 1.199719254218452935 ) ) ;
#141687=CARTESIAN_POINT ( 'NONE',  ( -4.769436176957319695, 8.786368983084006601, 0.7998128361456281477 ) ) ;
#141689=VERTEX_POINT ( 'NONE', #81620 ) ;
#141714=CARTESIAN_POINT ( 'NONE',  ( 6.393551957296131683, 9.616838495890963401, 1.199719254218452047 ) ) ;
#141716=CARTESIAN_POINT ( 'NONE',  ( 4.908934136599710563, 7.884784371745123366, 1.199719254218451159 ) ) ;
#141720=CARTESIAN_POINT ( 'NONE',  ( -1.823506805412349330, 2.449817705437798754, -2.460149088936845807 ) ) ;
#141730=CARTESIAN_POINT ( 'NONE',  ( 6.170003545802125622, 6.961323287618347955, -0.9016653442153206299 ) ) ;
#141732=CARTESIAN_POINT ( 'NONE',  ( 5.695833931516881776, 9.659240330162777610, -0.7216878364870458196 ) ) ;
#141740=CARTESIAN_POINT ( 'NONE',  ( -5.418418667316934112, 6.350518529071726981, -1.199719254218453823 ) ) ;
#141747=CARTESIAN_POINT ( 'NONE',  ( -5.546694241322218666, 8.524874810634301525, 1.082531754730550855 ) ) ;
#141751=CARTESIAN_POINT ( 'NONE',  ( 5.657495238652423097, 9.822437888394988548, 0.000000000000000000 ) ) ;
#141765=CARTESIAN_POINT ( 'NONE',  ( 8.005163354226054295, 8.304055099544019214, 0.000000000000000000 ) ) ;
#141785=CARTESIAN_POINT ( 'NONE',  ( -6.774234028683526532, 7.932303117332766718, 1.199719254218452047 ) ) ;
#141786=AXIS2_PLACEMENT_3D ( 'NONE', #121279, #5274, #137467 ) ;
#141789=CARTESIAN_POINT ( 'NONE',  ( 6.017840079619279692, 8.114175741012878973, -1.599625672291281386 ) ) ;
#141810=CARTESIAN_POINT ( 'NONE',  ( 5.777182853198898904, 6.873039762554409293, -1.082531754730548412 ) ) ;
#141820=CARTESIAN_POINT ( 'NONE',  ( 4.207966135563082410, 7.175396087857922822, -1.043745235818753780 ) ) ;
#141822=CARTESIAN_POINT ( 'NONE',  ( -6.156811154381562012, 6.355570232966157640, 0.7216878364870257245 ) ) ;
#141852=CARTESIAN_POINT ( 'NONE',  ( 5.903649544107831382, 5.852288987739402870, -0.7998128361456481317 ) ) ;
#141861=CARTESIAN_POINT ( 'NONE',  ( -5.641601317062239218, 8.635599732330991429, -1.082531754730549967 ) ) ;
#141863=CARTESIAN_POINT ( 'NONE',  ( 4.760321331729593375, 5.686701320840210627, -1.082531754730548412 ) ) ;
#141879=ORIENTED_EDGE ( 'NONE', *, *, #198557, .T. ) ;
#141880=CARTESIAN_POINT ( 'NONE',  ( -5.343321937561608337, 5.406499480009534508, 0.7216878364870257245 ) ) ;
#141895=ORIENTED_EDGE ( 'NONE', *, *, #15710, .T. ) ;
#141910=CARTESIAN_POINT ( 'NONE',  ( -6.312203035614172286, 9.521931420595302953, -1.199719254218452047 ) ) ;
#141913=CARTESIAN_POINT ( 'NONE',  ( -6.180537922983287302, 8.303989891604203422, -1.599625672291271394 ) ) ;
#141918=CARTESIAN_POINT ( 'NONE',  ( -7.282137903871469753, 8.628820655005750240, 1.082531754730549078 ) ) ;
#141925=CARTESIAN_POINT ( 'NONE',  ( -4.142898457427624415, 6.991076079377632091, 1.199719254218452935 ) ) ;
#141930=ORIENTED_EDGE ( 'NONE', *, *, #150147, .T. ) ;
#141935=CARTESIAN_POINT ( 'NONE',  ( 5.788239156490550208, 7.236076679697275083, -1.185412701995581797 ) ) ;
#141939=CARTESIAN_POINT ( 'NONE',  ( 5.747730777550676073, 5.670383760089384495, 0.000000000000000000 ) ) ;
#141951=CARTESIAN_POINT ( 'NONE',  ( 2.993041990875914493, 6.420974562437304911, 0.3677586026352899218 ) ) ;
#141960=CARTESIAN_POINT ( 'NONE',  ( 6.052789233858158369, 6.026285292448116948, 0.000000000000000000 ) ) ;
#141961=CARTESIAN_POINT ( 'NONE',  ( 5.671053392266061977, 9.838255734277600695, 0.7998128361456331437 ) ) ;
#141976=CARTESIAN_POINT ( 'NONE',  ( 6.580239226864286195, 6.782991656975736028, -0.2881480849740332140 ) ) ;
#141977=CARTESIAN_POINT ( 'NONE',  ( -3.973948422136970748, 6.690004688251493192, -1.082531754730546636 ) ) ;
#141999=CARTESIAN_POINT ( 'NONE',  ( -5.607584625718504689, 5.587669329723240708, -0.3781269150280338609 ) ) ;
#142004=CARTESIAN_POINT ( 'NONE',  ( 3.932747076415766596, 6.745899468197171345, 1.199719254218451159 ) ) ;
#142022=CARTESIAN_POINT ( 'NONE',  ( -4.620296487206990932, 8.612372678375294299, 0.000000000000000000 ) ) ;
#142035=CARTESIAN_POINT ( 'NONE',  ( 5.910428620914669473, 5.860197910680708944, 0.000000000000000000 ) ) ;
#142040=ADVANCED_FACE ( 'NONE', ( #22724, #37939 ), #153827, .F. ) ;
#142045=CARTESIAN_POINT ( 'NONE',  ( -5.600926855776894975, 6.667407765562058053, -1.082531754730549967 ) ) ;
#142046=CARTESIAN_POINT ( 'NONE',  ( 6.124909263556299166, 6.992440323537196356, 0.9511531368890328020 ) ) ;
#142049=CARTESIAN_POINT ( 'NONE',  ( -3.765305043611756552, 7.354576300424668922, -0.6638232778202641793 ) ) ;
#142069=CARTESIAN_POINT ( 'NONE',  ( -4.281342646865346602, 8.216926531310035031, 0.7998128361456352531 ) ) ;
#142071=CARTESIAN_POINT ( 'NONE',  ( 3.413620815590684199, 7.204584394822967752, 0.7998128361456281477 ) ) ;
#142075=CARTESIAN_POINT ( 'NONE',  ( -6.635789839245807897, 6.706452665400368218, 0.7998128361456341429 ) ) ;
#142079=CARTESIAN_POINT ( 'NONE',  ( 6.966220764712143243, 6.002124920821316323, -2.500000000000000444 ) ) ;
#142083=CARTESIAN_POINT ( 'NONE',  ( -4.712608863230891565, 8.343829661033030476, -0.7091526064728018719 ) ) ;
#142102=CARTESIAN_POINT ( 'NONE',  ( 5.899206235721897507, 6.055031161196562373, 0.000000000000000000 ) ) ;
#142106=CARTESIAN_POINT ( 'NONE',  ( -5.589704470584107909, 9.743348658981940247, -0.7998128361456362523 ) ) ;
#142119=CARTESIAN_POINT ( 'NONE',  ( 5.910428620914669473, 5.860197910680708944, 0.000000000000000000 ) ) ;
#142162=CARTESIAN_POINT ( 'NONE',  ( 5.063044020060520900, 4.871582543017558109, 0.7998128361456352531 ) ) ;
#142166=CARTESIAN_POINT ( 'NONE',  ( -4.055297343818976330, 5.824542549245813383, 1.443375672974065660 ) ) ;
#142173=CARTESIAN_POINT ( 'NONE',  ( -5.255720823952942489, 6.160704378480398979, -1.199719254218453823 ) ) ;
#142182=CARTESIAN_POINT ( 'NONE',  ( -4.817943484809863008, 6.714296380401858499, 1.599625672291263179 ) ) ;
#142184=CARTESIAN_POINT ( 'NONE',  ( 6.395636025722083673, 6.905704815116233242, -0.7835738547974178125 ) ) ;
#142189=CARTESIAN_POINT ( 'NONE',  ( 4.716257332707354699, 6.595662536282280719, -1.599625672291269396 ) ) ;
#142196=CARTESIAN_POINT ( 'NONE',  ( -5.738844160334429567, 9.917344963690652548, 0.000000000000000000 ) ) ;
#142200=CARTESIAN_POINT ( 'NONE',  ( -3.800028193580205382, 7.655393002477360653, -0.7998128361456481317 ) ) ;
#142204=CARTESIAN_POINT ( 'NONE',  ( 6.007671464186834065, 7.141943142040370063, 1.082531754730549967 ) ) ;
#142205=CARTESIAN_POINT ( 'NONE',  ( -6.333067150914850174, 8.481940657524365434, 1.443375672974064550 ) ) ;
#142207=ADVANCED_FACE ( 'NONE', ( #40079 ), #115275, .T. ) ;
#142214=CARTESIAN_POINT ( 'NONE',  ( 3.984117037569365305, 5.741498858621315371, 1.599625672291261402 ) ) ;
#142244=CARTESIAN_POINT ( 'NONE',  ( 4.599920620972065777, 8.367456947080912144, 0.1478172174028801744 ) ) ;
#142250=AXIS2_PLACEMENT_3D ( 'NONE', #212499, #28435, #64140 ) ;
#142252=CARTESIAN_POINT ( 'NONE',  ( 7.530627977747744062, 7.750430493652658015, -0.7998128361456341429 ) ) ;
#142253=VERTEX_POINT ( 'NONE', #208877 ) ;
#142257=CARTESIAN_POINT ( 'NONE',  ( -4.604461168338175980, 8.383524640989071131, 0.06638267717353450725 ) ) ;
#142261=ORIENTED_EDGE ( 'NONE', *, *, #112034, .T. ) ;
#142264=CARTESIAN_POINT ( 'NONE',  ( -5.908321080505254841, 10.11506803722328129, 0.7998128361456291469 ) ) ;
#142268=CARTESIAN_POINT ( 'NONE',  ( -3.716631501448782515, 7.355961102242025262, 0.5892660917431468137 ) ) ;
#142276=CARTESIAN_POINT ( 'NONE',  ( 7.388267364804250725, 7.584343111885245570, -0.7998128361456341429 ) ) ;
#142287=CARTESIAN_POINT ( 'NONE',  ( 5.252858170651868441, 5.093032385374103299, -0.7998128361456481317 ) ) ;
#142291=CARTESIAN_POINT ( 'NONE',  ( 4.868786560638885597, 7.733982516503781213, 1.082531754730548412 ) ) ;
#142300=CARTESIAN_POINT ( 'NONE',  ( -5.584154938098890852, 7.410262610144577877, 1.243513269814926492 ) ) ;
#142306=CARTESIAN_POINT ( 'NONE',  ( -3.688700311369816909, 6.461178242310183784, -1.199719254218450271 ) ) ;
#142308=CARTESIAN_POINT ( 'NONE',  ( 6.021229618244865023, 10.03886863134542828, -0.7216878364870458196 ) ) ;
#142320=CARTESIAN_POINT ( 'NONE',  ( -5.074494633264801990, 9.142270515442742607, 0.7998128361456291469 ) ) ;
#142321=CARTESIAN_POINT ( 'NONE',  ( -3.962726036944197894, 7.845207153068690431, -0.7998128361456481317 ) ) ;
#142323=CARTESIAN_POINT ( 'NONE',  ( 7.634649897826745857, 8.079715433652276957, 0.7216878364870267237 ) ) ;
#142335=CARTESIAN_POINT ( 'NONE',  ( -5.043389779576542331, 7.890798448915884222, -1.099773784605091009 ) ) ;
#142339=VECTOR ( 'NONE', #198702, 1000.000000000000114 ) ;
#142341=CARTESIAN_POINT ( 'NONE',  ( 5.722950238744211937, 5.849399164722627553, 0.7216878364870328300 ) ) ;
#142346=CARTESIAN_POINT ( 'NONE',  ( -7.618755976236585958, 7.853246491889623648, 0.000000000000000000 ) ) ;
#142352=EDGE_CURVE ( 'NONE', #37959, #66325, #31246, .T. ) ;
#142361=CARTESIAN_POINT ( 'NONE',  ( 6.717138760927786834, 6.801359740696030443, -0.7998128361456481317 ) ) ;
#142368=CARTESIAN_POINT ( 'NONE',  ( 4.318600669050608687, 4.999583595936801572, -2.420000000000000373 ) ) ;
#142376=CARTESIAN_POINT ( 'NONE',  ( 2.971951545985364262, 6.549969527005830905, 0.4930404537322597980 ) ) ;
#142395=CARTESIAN_POINT ( 'NONE',  ( 7.349928672384120176, 7.747540670635879145, 0.7216878364870267237 ) ) ;
#142423=CARTESIAN_POINT ( 'NONE',  ( -4.899292406491858820, 6.809203455697518947, -1.599625672291271394 ) ) ;
#142425=CARTESIAN_POINT ( 'NONE',  ( 5.438229012412886476, 7.437962829272074750, -1.443375672974078761 ) ) ;
#142431=CARTESIAN_POINT ( 'NONE',  ( -5.438755897737433287, 6.374245297895642537, -1.199719254218453823 ) ) ;
#142436=CARTESIAN_POINT ( 'NONE',  ( -5.659602779061863487, 5.567567761852417085, 0.7998128361456281477 ) ) ;
#142444=CARTESIAN_POINT ( 'NONE',  ( -5.808742468812186033, 5.741564066561132940, 0.000000000000000000 ) ) ;
#142453=CARTESIAN_POINT ( 'NONE',  ( -5.483346782084204563, 5.361935765378481378, 0.000000000000000000 ) ) ;
#142456=CARTESIAN_POINT ( 'NONE',  ( -6.292392690518214593, 7.474117906093608710, -1.082531754730549967 ) ) ;
#142457=CARTESIAN_POINT ( 'NONE',  ( -6.753369912938502750, 7.051555451282599307, 0.000000000000000000 ) ) ;
#142458=CARTESIAN_POINT ( 'NONE',  ( 5.254667053748194760, 8.288139441751686931, 1.199719254218452047 ) ) ;
#142459=CARTESIAN_POINT ( 'NONE',  ( -5.582925393777276035, 9.735439736040634173, 0.7998128361456291469 ) ) ;
#142477=CARTESIAN_POINT ( 'NONE',  ( 7.201315867513990554, 8.430565262634994284, -1.199719254218452047 ) ) ;
#142497=ADVANCED_FACE ( 'NONE', ( #166032 ), #166448, .T. ) ;
#142499=CARTESIAN_POINT ( 'NONE',  ( 4.602896574056089207, 8.480248385054199645, 0.1803159889683242367 ) ) ;
#142511=CARTESIAN_POINT ( 'NONE',  ( 4.701645408888975197, 8.707279753670952971, 0.000000000000000000 ) ) ;
#142517=CARTESIAN_POINT ( 'NONE',  ( -5.248414861821563804, 9.137251415518218067, 0.7216878364870267237 ) ) ;
#142525=EDGE_CURVE ( 'NONE', #114168, #173093, #85724, .T. ) ;
#142526=FACE_OUTER_BOUND ( 'NONE', #182541, .T. ) ;
#142529=CARTESIAN_POINT ( 'NONE',  ( 6.373214726875630731, 9.593111727067046957, 1.199719254218452047 ) ) ;
#142531=CARTESIAN_POINT ( 'NONE',  ( 6.690022453700429139, 6.769724048930809701, 0.7998128361456331437 ) ) ;
#142540=CARTESIAN_POINT ( 'NONE',  ( 5.096939404094710468, 4.911127157724081371, 0.000000000000000000 ) ) ;
#142546=CARTESIAN_POINT ( 'NONE',  ( 5.956828388357757298, 8.042995434541133193, 1.599625672291269396 ) ) ;
#142557=CARTESIAN_POINT ( 'NONE',  ( -5.668717624289589807, 5.786127781192186958, 0.7216878364870257245 ) ) ;
#142559=CARTESIAN_POINT ( 'NONE',  ( -5.589704470584107909, 9.743348658981940247, -0.7998128361456362523 ) ) ;
#142571=CARTESIAN_POINT ( 'NONE',  ( 4.518610335104485287, 8.493738834255713854, 0.000000000000000000 ) ) ;
#142572=CARTESIAN_POINT ( 'NONE',  ( 5.956828388357757298, 8.042995434541133193, 1.599625672291269396 ) ) ;
#142575=CARTESIAN_POINT ( 'NONE',  ( 3.675669042636310557, 6.342012078834061484, -1.082531754730549967 ) ) ;
#142591=DIRECTION ( 'NONE',  ( 0.7592566023653005702, -0.6507913734559639396, 0.000000000000000000 ) ) ;
#142594=CARTESIAN_POINT ( 'NONE',  ( 3.627688620108284745, 6.389997935838436227, 1.199719254218452047 ) ) ;
#142597=CARTESIAN_POINT ( 'NONE',  ( 4.525389411911321602, 8.501647757197021704, -0.7998128361456381397 ) ) ;
#142609=CARTESIAN_POINT ( 'NONE',  ( 7.865138509703455405, 8.348618814175074121, -0.7216878364870317197 ) ) ;
#142611=CARTESIAN_POINT ( 'NONE',  ( -6.629010762438975135, 6.698543742459062145, -0.7998128361456362523 ) ) ;
#142612=CARTESIAN_POINT ( 'NONE',  ( 5.041653019435334393, 6.975290837464928728, -1.599625672291269396 ) ) ;
#142619=CARTESIAN_POINT ( 'NONE',  ( -5.343912927829680193, 6.631183989036703252, -1.180091537758539921 ) ) ;
#142622=CARTESIAN_POINT ( 'NONE',  ( -4.984557751679625781, 5.844347460828191565, 1.199719254218452935 ) ) ;
#142651=CARTESIAN_POINT ( 'NONE',  ( 2.943528747942701695, 6.448217615992859919, 0.000000000000000000 ) ) ;
#142657=CARTESIAN_POINT ( 'NONE',  ( 3.065552130021340194, 6.590578228417936835, 0.000000000000000000 ) ) ;
#142668=CARTESIAN_POINT ( 'NONE',  ( -4.281342646865346602, 8.216926531310035031, 0.7998128361456352531 ) ) ;
#142670=CARTESIAN_POINT ( 'NONE',  ( -7.110325215724114578, 7.260077271291732082, 0.000000000000000000 ) ) ;
#142672=CARTESIAN_POINT ( 'NONE',  ( 5.519577934094840543, 9.453608333170423705, 0.7216878364870317197 ) ) ;
#142684=CARTESIAN_POINT ( 'NONE',  ( -6.445975688654487001, 6.485002823043819475, -0.7998128361456362523 ) ) ;
#142691=CARTESIAN_POINT ( 'NONE',  ( -4.163762573172648196, 7.871823745427799501, 0.000000000000000000 ) ) ;
#142695=CARTESIAN_POINT ( 'NONE',  ( -4.288121723672178476, 8.224835454251337552, -0.7998128361456362523 ) ) ;
#142704=CARTESIAN_POINT ( 'NONE',  ( -6.050251585826448952, 7.027409288634817841, -1.057721621305447890 ) ) ;
#142718=CARTESIAN_POINT ( 'NONE',  ( -6.981522756394290319, 7.109807735406931783, 0.7998128361456341429 ) ) ;
#142720=CARTESIAN_POINT ( 'NONE',  ( -3.644109427023046521, 7.473487774827342278, 0.000000000000000000 ) ) ;
#142732=VERTEX_POINT ( 'NONE', #90694 ) ;
#142747=CARTESIAN_POINT ( 'NONE',  ( -5.498713818794216834, 8.572860667638675380, -1.199719254218452047 ) ) ;
#142773=CARTESIAN_POINT ( 'NONE',  ( 6.933015448541703485, 9.181880338089085214, 1.599625672291268286 ) ) ;
#142775=CARTESIAN_POINT ( 'NONE',  ( 5.833751235630055376, 10.02806988486892514, 0.7998128361456331437 ) ) ;
#142789=CARTESIAN_POINT ( 'NONE',  ( 5.582388601459258304, 7.396495182493852738, 1.242574333668546638 ) ) ;
#142791=CARTESIAN_POINT ( 'NONE',  ( 5.994113311017540191, 9.046863725278862844, -1.082531754730548412 ) ) ;
#142799=CARTESIAN_POINT ( 'NONE',  ( -4.447956913735107598, 7.346977611736363656, 1.199719254218452935 ) ) ;
#142806=CARTESIAN_POINT ( 'NONE',  ( -5.275531169048901958, 8.208517892982092334, -1.082531754730549967 ) ) ;
#142809=CARTESIAN_POINT ( 'NONE',  ( 6.994027139803230320, 9.253060644560830994, -1.599625672291267398 ) ) ;
#142815=CARTESIAN_POINT ( 'NONE',  ( -5.320648938720212051, 5.172121614787156929, 0.000000000000000000 ) ) ;
#142822=CARTESIAN_POINT ( 'NONE',  ( 3.562760505341037831, 7.378580699531681830, -1.734723475976807094E-15 ) ) ;
#142824=CARTESIAN_POINT ( 'NONE',  ( 7.289443866002793371, 8.533381260871966134, 1.199719254218452047 ) ) ;
#142842=CARTESIAN_POINT ( 'NONE',  ( -7.611976899429754084, 7.845337568948314022, 0.7998128361456341429 ) ) ;
#142845=CARTESIAN_POINT ( 'NONE',  ( 6.343235766347262938, 8.493804042195527870, -1.599625672291281386 ) ) ;
#142847=AXIS2_PLACEMENT_3D ( 'NONE', #124569, #10712, #110432 ) ;
#142848=CARTESIAN_POINT ( 'NONE',  ( -6.489499031467138579, 6.765560312407735033, -0.1891594744549245088 ) ) ;
#142854=CARTESIAN_POINT ( 'NONE',  ( 4.518610335104485287, 8.493738834255713854, 0.000000000000000000 ) ) ;
#142864=CARTESIAN_POINT ( 'NONE',  ( 4.177320726786311056, 5.966903162707725805, -1.443375672974068769 ) ) ;
#142868=CARTESIAN_POINT ( 'NONE',  ( 6.563555762791525972, 6.830105609444471426, -0.7216878364870458196 ) ) ;
#142869=ORIENTED_EDGE ( 'NONE', *, *, #41407, .T. ) ;
#142879=CARTESIAN_POINT ( 'NONE',  ( -4.800995793014949165, 8.615262501910491366, 0.7216878364870267237 ) ) ;
#142883=ORIENTED_EDGE ( 'NONE', *, *, #164010, .F. ) ;
#142891=FACE_OUTER_BOUND ( 'NONE', #165031, .T. ) ;
#142893=CARTESIAN_POINT ( 'NONE',  ( 0.3999999999999758193, 2.999999999999999112, 2.420000000000000373 ) ) ;
#142913=CARTESIAN_POINT ( 'NONE',  ( 4.228163802615382494, 6.026220084508304708, -1.599625672291269396 ) ) ;
#142924=CARTESIAN_POINT ( 'NONE',  ( -7.105881907338178038, 7.462819444748888920, -0.7216878364870338292 ) ) ;
#142926=CARTESIAN_POINT ( 'NONE',  ( 3.051993976407674225, 6.574760382535328240, -0.7216878364870338292 ) ) ;
#142944=CARTESIAN_POINT ( 'NONE',  ( -4.014622883422336308, 5.777089012116397804, -1.443375672974066548 ) ) ;
#142949=DIRECTION ( 'NONE',  ( 1.953992523340275511E-14, 0.000000000000000000, -1.000000000000000000 ) ) ;
#142976=CARTESIAN_POINT ( 'NONE',  ( -6.420668264523499147, 9.648474187656182366, 1.199719254218452935 ) ) ;
#142979=CARTESIAN_POINT ( 'NONE',  ( -6.343235766347277149, 8.493804042195527870, -1.599625672291271394 ) ) ;
#142980=CARTESIAN_POINT ( 'NONE',  ( -4.758546912290684716, 8.291040531757728260, 0.8107885835855069834 ) ) ;
#142988=CARTESIAN_POINT ( 'NONE',  ( -5.029148636026397945, 4.832037928311032182, 0.7998128361456281477 ) ) ;
#142992=CARTESIAN_POINT ( 'NONE',  ( -5.330290668828105538, 6.247702530834755130, 1.199719254218452935 ) ) ;
#143001=CARTESIAN_POINT ( 'NONE',  ( -3.096514578442687515, 6.188910745953249304, -0.7944190528704382359 ) ) ;
#143006=CARTESIAN_POINT ( 'NONE',  ( 5.411639590510088027, 6.342609606130419131, -1.199719254218452047 ) ) ;
#143009=EDGE_CURVE ( 'NONE', #96770, #22085, #54112, .T. ) ;
#143032=CARTESIAN_POINT ( 'NONE',  ( 6.378184920586140727, 6.405913593630768510, 0.000000000000000000 ) ) ;
#143033=CARTESIAN_POINT ( 'NONE',  ( 4.899292406491845497, 6.809203455697518947, -1.599625672291273171 ) ) ;
#143035=CARTESIAN_POINT ( 'NONE',  ( 4.523580528814945545, 5.306540700819438960, 1.199719254218452047 ) ) ;
#143047=CARTESIAN_POINT ( 'NONE',  ( 4.831949485534527966, 8.212610664285437068, 0.9193987405316924599 ) ) ;
#143048=CARTESIAN_POINT ( 'NONE',  ( -5.004368096775595021, 5.971422546727199077, 1.082531754730549078 ) ) ;
#143077=CARTESIAN_POINT ( 'NONE',  ( 3.984117037569365305, 5.741498858621315371, 1.599625672291261402 ) ) ;
#143088=( BOUNDED_CURVE ( )  B_SPLINE_CURVE ( 2, ( #73236, #5018, #55943, #75397, #39689 ),
 .UNSPECIFIED., .F., .T. ) 
 B_SPLINE_CURVE_WITH_KNOTS ( ( 3, 2, 3 ),
 ( 0.2694919930870862679, 0.2750000000000000222, 0.2821090017918219117 ),
 .UNSPECIFIED. ) 
 CURVE ( )  GEOMETRIC_REPRESENTATION_ITEM ( )  RATIONAL_B_SPLINE_CURVE ( ( 0.9399548337079939309, 0.9114480397467834560, 1.000000000000000000, 0.8857089226533948478, 0.9664167589818952742 ) ) 
 REPRESENTATION_ITEM ( '' )  );
#143098=CARTESIAN_POINT ( 'NONE',  ( -7.944151662964566540, 8.232874793072271657, 0.000000000000000000 ) ) ;
#143115=CARTESIAN_POINT ( 'NONE',  ( 5.143339171537801846, 7.093924681584509173, 1.599625672291269396 ) ) ;
#143123=CARTESIAN_POINT ( 'NONE',  ( 4.860027775985512832, 8.063079866353717762, 0.9206262284592428013 ) ) ;
#143125=CARTESIAN_POINT ( 'NONE',  ( 5.638349000628050334, 7.351887578364292075, 1.232751772250343381 ) ) ;
#143131=CARTESIAN_POINT ( 'NONE',  ( -4.009193028827814587, 7.297902834095492786, -0.7581239365674132813 ) ) ;
#143146=CARTESIAN_POINT ( 'NONE',  ( -5.336015975430226099, 8.383046517047350932, -1.199719254218453823 ) ) ;
#143148=CARTESIAN_POINT ( 'NONE',  ( 3.400062661977048428, 7.188766548940353829, -1.734723475976807094E-15 ) ) ;
#143153=CARTESIAN_POINT ( 'NONE',  ( -5.576146316970437944, 9.727530813099326323, 0.000000000000000000 ) ) ;
#143156=CARTESIAN_POINT ( 'NONE',  ( 6.003228155800906407, 10.22579295840155744, 0.000000000000000000 ) ) ;
#143161=CARTESIAN_POINT ( 'NONE',  ( -5.188065202531182862, 7.850521293832936287, -1.269213148129512136 ) ) ;
#143172=CARTESIAN_POINT ( 'NONE',  ( 0.1265484174145335983, 2.536982183874235908, -2.076146791065092145 ) ) ;
#143177=ORIENTED_EDGE ( 'NONE', *, *, #83202, .F. ) ;
#143181=CARTESIAN_POINT ( 'NONE',  ( 5.478903473698239601, 7.485416367438324059, -1.443375672974078761 ) ) ;
#143184=CARTESIAN_POINT ( 'NONE',  ( -8.072954122294394352, 8.383144328957069291, -0.7998128361456362523 ) ) ;
#143192=CARTESIAN_POINT ( 'NONE',  ( 2.970157261343746136, 6.585292010301047938, 0.4235207732182846851 ) ) ;
#143195=CARTESIAN_POINT ( 'NONE',  ( -3.038435823238377687, 6.558942537171132514, -0.7216878364870458196 ) ) ;
#143200=CARTESIAN_POINT ( 'NONE',  ( 6.073126464278658432, 6.050012061272033392, 0.000000000000000000 ) ) ;
#143227=ORIENTED_EDGE ( 'NONE', *, *, #136379, .T. ) ;
#143243=CARTESIAN_POINT ( 'NONE',  ( 4.415115299905642665, 5.179997933758551554, -1.199719254218450271 ) ) ;
#143247=CARTESIAN_POINT ( 'NONE',  ( -5.275531169048911728, 6.287779464379406491, -1.082531754730549967 ) ) ;
#143254=CARTESIAN_POINT ( 'NONE',  ( -6.069210040772897052, 7.109775131437022999, -1.199719254218453823 ) ) ;
#143263=CARTESIAN_POINT ( 'NONE',  ( -4.793689830883590020, 7.750332681742931662, 1.199719254218452935 ) ) ;
#143265=CARTESIAN_POINT ( 'NONE',  ( 6.533654944624902150, 6.813559398729744032, -0.4760831665120857648 ) ) ;
#143270=CARTESIAN_POINT ( 'NONE',  ( 5.987861119090863049, 7.014868056141362551, 1.199719254218452047 ) ) ;
#143276=CARTESIAN_POINT ( 'NONE',  ( -7.747558435566414659, 8.003516027774422170, -0.7998128361456362523 ) ) ;
#143281=CARTESIAN_POINT ( 'NONE',  ( -4.610654757099099221, 7.536791762327691657, 1.199719254218452935 ) ) ;
#143284=CARTESIAN_POINT ( 'NONE',  ( 4.489158259456265121, 7.291082831790689056, -1.082531754730548412 ) ) ;
#143285=CARTESIAN_POINT ( 'NONE',  ( -6.753369912938502750, 7.051555451282599307, 0.000000000000000000 ) ) ;
#143293=CARTESIAN_POINT ( 'NONE',  ( 4.030516805012513082, 7.924296382481737844, 0.000000000000000000 ) ) ;
#143296=CARTESIAN_POINT ( 'NONE',  ( 2.972033609136344623, 6.549060441754430251, -0.4946758370507741698 ) ) ;
#143299=SURFACE_STYLE_FILL_AREA ( #190919 ) ;
#143301=CARTESIAN_POINT ( 'NONE',  ( -2.976926559254097437, 6.503136272932390050, -0.2410342056339362937 ) ) ;
#143319=CARTESIAN_POINT ( 'NONE',  ( 4.678042868546113731, 8.270637144445508682, 0.5573067791126932180 ) ) ;
#143326=CARTESIAN_POINT ( 'NONE',  ( 5.505492895601038938, 8.580769590579979678, -1.199719254218452047 ) ) ;
#143332=CARTESIAN_POINT ( 'NONE',  ( -4.603423314590644466, 8.384863137925270493, -0.01591256823598764802 ) ) ;
#143338=CARTESIAN_POINT ( 'NONE',  ( -7.957709816578236506, 8.248692638954882028, 0.7998128361456341429 ) ) ;
#143349=CARTESIAN_POINT ( 'NONE',  ( -6.180537922983287302, 8.303989891604203422, -1.599625672291271394 ) ) ;
#143351=CARTESIAN_POINT ( 'NONE',  ( 6.713222337422018349, 7.861122810861019161, -1.199719254218452047 ) ) ;
#143359=CARTESIAN_POINT ( 'NONE',  ( 5.551137550152489553, 5.441024994791534120, 0.7998128361456352531 ) ) ;
#143362=CARTESIAN_POINT ( 'NONE',  ( 4.055297343818923039, 7.745280977848496562, 0.7216878364870257245 ) ) ;
#143370=CARTESIAN_POINT ( 'NONE',  ( -5.425839481171796486, 7.540841100536294306, 1.248335065278019629 ) ) ;
#143374=ORIENTED_EDGE ( 'NONE', *, *, #76686, .F. ) ;
#143377=CARTESIAN_POINT ( 'NONE',  ( -3.122120512896910505, 6.864500708346841229, 0.7998128361456352531 ) ) ;
#143379=CARTESIAN_POINT ( 'NONE',  ( 6.319508997745523438, 9.426492026461511742, -1.082531754730548412 ) ) ;
#143390=CARTESIAN_POINT ( 'NONE',  ( -6.934069218746458318, 7.054445274817795486, -0.7998128361456362523 ) ) ;
#143391=CARTESIAN_POINT ( 'NONE',  ( -4.878955176071358757, 6.785476686873604280, -1.599625672291271394 ) ) ;
#143393=CARTESIAN_POINT ( 'NONE',  ( 7.960045584554727327, 8.459343734834927631, 0.7216878364870267237 ) ) ;
#143406=CARTESIAN_POINT ( 'NONE',  ( -6.357087581413799704, 6.851358791993434671, -0.6307199548913413611 ) ) ;
#143407=CARTESIAN_POINT ( 'NONE',  ( -9.336326716892640931, -1.000000000000000888, -2.500000000000000444 ) ) ;
#143411=CARTESIAN_POINT ( 'NONE',  ( 4.692530564105613422, 7.528350520548263702, -1.082531754730548412 ) ) ;
#143415=CARTESIAN_POINT ( 'NONE',  ( -4.207966135563104615, 7.175396087857926375, -2.420000000000000373 ) ) ;
#143416=CARTESIAN_POINT ( 'NONE',  ( -6.688968683495758683, 8.897159112202094988, -1.599625672291271394 ) ) ;
#143432=CARTESIAN_POINT ( 'NONE',  ( 5.936491157937257235, 8.019268665717216749, 1.599625672291268286 ) ) ;
#143467=CARTESIAN_POINT ( 'NONE',  ( 3.770049233051776749, 6.556085317605844232, 1.199719254218451159 ) ) ;
#143491=AXIS2_PLACEMENT_3D ( 'NONE', #112083, #131506, #163971 ) ;
#143499=CARTESIAN_POINT ( 'NONE',  ( -5.492988512192097161, 6.437516681426083132, 1.199719254218452935 ) ) ;
#143505=CARTESIAN_POINT ( 'NONE',  ( -4.630991987519598396, 7.560518531151607213, 1.199719254218452935 ) ) ;
#143511=CARTESIAN_POINT ( 'NONE',  ( -4.309512724297390740, 6.121127159803966933, 1.599625672291270506 ) ) ;
#143518=CIRCLE ( 'NONE', #84547, 0.08000000000000012657 ) ;
#143519=CARTESIAN_POINT ( 'NONE',  ( -4.599959256786493533, 8.588645909551377855, 0.000000000000000000 ) ) ;
#143526=EDGE_CURVE ( 'NONE', #52099, #162079, #62325, .T. ) ;
#143528=CARTESIAN_POINT ( 'NONE',  ( -5.144392941742557568, 4.966489618313220333, -0.7998128361456362523 ) ) ;
#143532=CARTESIAN_POINT ( 'NONE',  ( -5.804299160426242388, 6.904675454319632699, -1.082531754730549967 ) ) ;
#143533=CARTESIAN_POINT ( 'NONE',  ( -5.763624699140883934, 6.857221916153382502, -1.082531754730549967 ) ) ;
#143534=CARTESIAN_POINT ( 'NONE',  ( 5.363132282657546490, 8.414682208812571673, -1.199719254218452047 ) ) ;
#143537=CARTESIAN_POINT ( 'NONE',  ( -5.607179047703544583, 8.699403434699558346, 1.199719254218454489 ) ) ;
#143555=CARTESIAN_POINT ( 'NONE',  ( 6.933015448541703485, 9.181880338089085214, 1.599625672291268286 ) ) ;
#143575=CARTESIAN_POINT ( 'NONE',  ( 4.672271667806711548, 8.395315985019093930, 0.5582388282892002396 ) ) ;
#143589=ADVANCED_FACE ( 'NONE', ( #71994 ), #204116, .T. ) ;
#143590=CARTESIAN_POINT ( 'NONE',  ( 6.496291879603339758, 7.608037276739255006, 1.199719254218452935 ) ) ;
#143597=CARTESIAN_POINT ( 'NONE',  ( -6.414416072596845986, 8.576847732820027659, -1.443375672974066548 ) ) ;
#143598=CARTESIAN_POINT ( 'NONE',  ( 4.941190227301914817, 4.729419784799151927, -0.4099107353478681492 ) ) ;
#143608=CARTESIAN_POINT ( 'NONE',  ( 2.898410978271408922, 6.603506251283770112, -0.7998128361456362523 ) ) ;
#143609=CARTESIAN_POINT ( 'NONE',  ( 5.397027666691686321, 8.454226823519094935, 1.199719254218451159 ) ) ;
#143613=CARTESIAN_POINT ( 'NONE',  ( -5.608478439449225306, 5.609308656285654671, -0.4224404339892348093 ) ) ;
#143622=ORIENTED_EDGE ( 'NONE', *, *, #189993, .F. ) ;
#143623=CARTESIAN_POINT ( 'NONE',  ( 5.037736595929563244, 8.035053907629919223, -1.199719254218452047 ) ) ;
#143624=ORIENTED_EDGE ( 'NONE', *, *, #128773, .T. ) ;
#143639=CARTESIAN_POINT ( 'NONE',  ( -5.316205630334263965, 7.295602216847000498, -1.443375672974066548 ) ) ;
#143640=CARTESIAN_POINT ( 'NONE',  ( -6.400331034103001748, 9.624747418832267698, 1.199719254218452935 ) ) ;
#143652=CARTESIAN_POINT ( 'NONE',  ( 5.365994935958575240, 9.482354201918870018, 0.7998128361456341429 ) ) ;
#143655=CARTESIAN_POINT ( 'NONE',  ( 4.055297343818933697, 5.824542549245813383, 1.443375672974058777 ) ) ;
#143660=CARTESIAN_POINT ( 'NONE',  ( 5.346851039111009563, 6.199209027673978412, 2.419999999999999485 ) ) ;
#143663=DIRECTION ( 'NONE',  ( -0.6507913734559658270, -0.7592566023652989049, 0.000000000000000000 ) ) ;
#143675=CARTESIAN_POINT ( 'NONE',  ( 6.886615681098613884, 6.999082814228660077, 0.000000000000000000 ) ) ;
#143681=CARTESIAN_POINT ( 'NONE',  ( 5.306037014901791693, 7.283738832175834510, 1.599625672291269396 ) ) ;
#143692=CARTESIAN_POINT ( 'NONE',  ( 7.349928672384120176, 7.747540670635879145, 0.7216878364870267237 ) ) ;
#143694=CARTESIAN_POINT ( 'NONE',  ( -6.119526231721793330, 8.232809585132461194, 1.599625672291263179 ) ) ;
#143695=CARTESIAN_POINT ( 'NONE',  ( 5.415556014015861841, 5.282846535965431300, -0.7998128361456481317 ) ) ;
#143705=CARTESIAN_POINT ( 'NONE',  ( -4.930325137224961907, 5.781076077297750970, -1.199719254218453823 ) ) ;
#143729=ADVANCED_FACE ( 'NONE', ( #70923 ), #57905, .F. ) ;
#143739=CARTESIAN_POINT ( 'NONE',  ( 3.390947816749319443, 6.970206529600588397, -1.734723475976807094E-15 ) ) ;
#143750=CARTESIAN_POINT ( 'NONE',  ( -4.118644803501354978, 8.027112380718707030, 0.7998128361456352531 ) ) ;
#143752=CARTESIAN_POINT ( 'NONE',  ( -5.901542003698421190, 10.10715911428198055, 0.000000000000000000 ) ) ;
#143754=CARTESIAN_POINT ( 'NONE',  ( 7.363486825553451354, 8.723727730301414240, -1.082531754730548412 ) ) ;
#143764=CARTESIAN_POINT ( 'NONE',  ( -5.088052786878465739, 9.158088361325352977, 0.000000000000000000 ) ) ;
#143771=CARTESIAN_POINT ( 'NONE',  ( -4.014622883422329203, 6.737458226417744278, -1.082531754730546636 ) ) ;
#143775=CARTESIAN_POINT ( 'NONE',  ( -4.716257332707368910, 6.595662536282280719, -1.599625672291271394 ) ) ;
#143783=CARTESIAN_POINT ( 'NONE',  ( -5.826449692766521693, 7.206545609186315815, -1.206671273860264515 ) ) ;
#143794=CARTESIAN_POINT ( 'NONE',  ( -4.945692173934974178, 8.992000979557944973, 0.000000000000000000 ) ) ;
#143797=CARTESIAN_POINT ( 'NONE',  ( -5.517242166118370150, 5.401480380085008193, 0.7998128361456281477 ) ) ;
#143822=CARTESIAN_POINT ( 'NONE',  ( -5.284646014276622950, 9.387447126623207794, -0.7998128361456362523 ) ) ;
#143829=B_SPLINE_CURVE_WITH_KNOTS ( 'NONE', 3,
 ( #6411, #54126, #185166, #152686 ),
 .UNSPECIFIED., .F., .F.,
 ( 4, 4 ),
 ( 0.003282510000513595011, 0.004028258324140119966 ),
 .UNSPECIFIED. ) ;
#143847=ADVANCED_FACE ( 'NONE', ( #30762 ), #133342, .F. ) ;
#143852=CARTESIAN_POINT ( 'NONE',  ( 7.506374323821472849, 8.786466794993730289, -1.199719254218452047 ) ) ;
#143864=CARTESIAN_POINT ( 'NONE',  ( 5.931307043615195340, 7.129970210930432373, 1.110187140972586306 ) ) ;
#143866=CARTESIAN_POINT ( 'NONE',  ( 6.861835142292147083, 7.178098218861903135, 0.7216878364870328300 ) ) ;
#143867=EDGE_CURVE ( 'NONE', #185175, #162324, #84840, .T. ) ;
#143873=CARTESIAN_POINT ( 'NONE',  ( -5.971440312176176768, 5.931378217152456500, 0.000000000000000000 ) ) ;
#143880=CARTESIAN_POINT ( 'NONE',  ( -7.404161286394468355, 7.810812053647902431, 0.000000000000000000 ) ) ;
#143884=CARTESIAN_POINT ( 'NONE',  ( -5.032355315092804204, 6.712689635018381118, 1.249972437814668380 ) ) ;
#143900=CARTESIAN_POINT ( 'NONE',  ( 4.435452530326143616, 5.203724702582467998, -1.199719254218452047 ) ) ;
#143916=ORIENTED_EDGE ( 'NONE', *, *, #34251, .T. ) ;
#143917=CARTESIAN_POINT ( 'NONE',  ( 0.000000000000000000, 8.499999999999996447, 0.000000000000000000 ) ) ;
#143919=CARTESIAN_POINT ( 'NONE',  ( 6.692885107001518286, 7.837396042037102717, -1.199719254218452047 ) ) ;
#143922=CARTESIAN_POINT ( 'NONE',  ( -5.157723666773176063, 7.780300641499326098, 1.171761296108381201 ) ) ;
#143929=CARTESIAN_POINT ( 'NONE',  ( 5.903649544107831382, 5.852288987739402870, -0.7998128361456481317 ) ) ;
#143937=CARTESIAN_POINT ( 'NONE',  ( 4.773879485787624333, 4.742149952939897162, -0.7216878364870357165 ) ) ;
#143940=CARTESIAN_POINT ( 'NONE',  ( 6.211043768836185031, 6.418841616496599123, 0.7216878364870328300 ) ) ;
#143951=CARTESIAN_POINT ( 'NONE',  ( -4.489158259900630554, 8.251452046610447510, 0.000000000000000000 ) ) ;
#143986=CARTESIAN_POINT ( 'NONE',  ( 5.041653019435334393, 6.975290837464928728, -1.599625672291269396 ) ) ;
#143991=CARTESIAN_POINT ( 'NONE',  ( 5.575758015699216585, 5.849789923344298259, -0.7899890411014517388 ) ) ;
#143999=CARTESIAN_POINT ( 'NONE',  ( -5.790741006812557323, 9.769965251341050205, 0.000000000000000000 ) ) ;
#144002=CARTESIAN_POINT ( 'NONE',  ( 3.065552130021340194, 6.590578228417936835, 0.000000000000000000 ) ) ;
#144018=CARTESIAN_POINT ( 'NONE',  ( -3.933273961740340496, 5.682181936820735579, 1.443375672974065660 ) ) ;
#144020=CARTESIAN_POINT ( 'NONE',  ( -4.858757509019059562, 5.629766575900002401, 2.420000000000000373 ) ) ;
#144055=CARTESIAN_POINT ( 'NONE',  ( -6.129167961829681488, 9.308390501180058507, -1.199719254218452047 ) ) ;
#144056=CARTESIAN_POINT ( 'NONE',  ( -5.289925464687482481, 7.757115612407050165, 1.311310741419260628 ) ) ;
#144061=CARTESIAN_POINT ( 'NONE',  ( -5.000000000000013323, 8.499999999999996447, 0.7750000000000004663 ) ) ;
#144064=CARTESIAN_POINT ( 'NONE',  ( -4.679499295372141709, 5.488445928469455559, 1.199719254218452935 ) ) ;
#144067=CARTESIAN_POINT ( 'NONE',  ( -5.113360211009450040, 5.994616996712990975, -1.199719254218453823 ) ) ;
#144072=ORIENTED_EDGE ( 'NONE', *, *, #213257, .T. ) ;
#144080=CARTESIAN_POINT ( 'NONE',  ( 5.520104819419390907, 6.469152373191302985, 1.199719254218452935 ) ) ;
#144105=CARTESIAN_POINT ( 'NONE',  ( 4.369470645354133431, 8.319742529546998000, 0.7998128361456271485 ) ) ;
#144106=CARTESIAN_POINT ( 'NONE',  ( 3.898851692381625877, 6.706354853490643642, -1.199719254218452047 ) ) ;
#144108=CARTESIAN_POINT ( 'NONE',  ( 3.444653546323793947, 6.176457016423196222, 1.199719254218451159 ) ) ;
#144116=CARTESIAN_POINT ( 'NONE',  ( 0.4663757142498895503, 3.020629270880486494, 1.944911959762657627 ) ) ;
#144121=CARTESIAN_POINT ( 'NONE',  ( 4.650542599771462449, 8.421518672640367242, 0.4769741307986720136 ) ) ;
#144122=CARTESIAN_POINT ( 'NONE',  ( -5.438229012412903352, 6.477593614970734492, -1.082531754730549967 ) ) ;
#144144=CARTESIAN_POINT ( 'NONE',  ( -0.01652817808797454532, 2.595569970836366203, -2.081186177183739883 ) ) ;
#144150=CARTESIAN_POINT ( 'NONE',  ( 3.379725431556547477, 7.165039780116438273, -1.734723475976807094E-15 ) ) ;
#144165=EDGE_CURVE ( 'NONE', #101393, #82918, #3273, .T. ) ;
#144170=CARTESIAN_POINT ( 'NONE',  ( -5.986807348886189040, 9.142303119412650503, -1.199719254218452047 ) ) ;
#144175=CARTESIAN_POINT ( 'NONE',  ( -5.608633734226008194, 5.643391804966442216, 0.4859901473732997079 ) ) ;
#144183=CARTESIAN_POINT ( 'NONE',  ( 4.993145711582793744, 9.047363440147082159, -0.7998128361456481317 ) ) ;
#144188=CARTESIAN_POINT ( 'NONE',  ( 4.929271367020211514, 7.908511140569038922, 1.199719254218452047 ) ) ;
#144198=CARTESIAN_POINT ( 'NONE',  ( 4.739057715201537846, 8.198473722472776615, 0.7146191656044629248 ) ) ;
#144206=DIRECTION ( 'NONE',  ( -0.7592566023653004592, 0.6507913734559639396, 0.000000000000000000 ) ) ;
#144211=CARTESIAN_POINT ( 'NONE',  ( -6.047232192207364854, 7.062196034744411932, 1.031126814801977432 ) ) ;
#144212=CARTESIAN_POINT ( 'NONE',  ( 4.947799714344386146, 4.737130853015369958, -0.7998128361456481317 ) ) ;
#144219=CARTESIAN_POINT ( 'NONE',  ( -6.466312919074983512, 6.508729591867735031, -0.7998128361456362523 ) ) ;
#144221=CARTESIAN_POINT ( 'NONE',  ( 6.737475991348287785, 6.825086509519945999, -0.7998128361456481317 ) ) ;
#144225=CARTESIAN_POINT ( 'NONE',  ( -6.563028877466991595, 9.814561569423593923, 1.199719254218452935 ) ) ;
#144228=CARTESIAN_POINT ( 'NONE',  ( 8.025500584646550806, 8.327781868367935658, 0.000000000000000000 ) ) ;
#144233=CARTESIAN_POINT ( 'NONE',  ( -5.696549332702473656, 7.414053552612095643, -1.332310987329322183 ) ) ;
#144252=CARTESIAN_POINT ( 'NONE',  ( 5.885648082108200896, 6.039213315313952002, 0.7216878364870328300 ) ) ;
#144262=CARTESIAN_POINT ( 'NONE',  ( -3.174173815459254477, 6.085887121384163656, -0.9314628722868825150 ) ) ;
#144272=CARTESIAN_POINT ( 'NONE',  ( 5.061990249855835344, 6.999017606288844284, -1.599625672291273171 ) ) ;
#144291=AXIS2_PLACEMENT_3D ( 'NONE', #97414, #148289, #163469 ) ;
#144308=CARTESIAN_POINT ( 'NONE',  ( 6.966220764712143243, 6.002124920821316323, -2.420000000000000373 ) ) ;
#144310=CARTESIAN_POINT ( 'NONE',  ( 3.919715808126649659, 7.587102519540811940, 0.000000000000000000 ) ) ;
#144320=CARTESIAN_POINT ( 'NONE',  ( -5.777182852754558340, 5.912670547734647286, 0.000000000000000000 ) ) ;
#144325=CARTESIAN_POINT ( 'NONE',  ( -6.120580001926503755, 6.105374521861167914, -0.7998128361456362523 ) ) ;
#144334=CARTESIAN_POINT ( 'NONE',  ( -5.829079699232685208, 5.765290835385048496, 0.000000000000000000 ) ) ;
#144336=CARTESIAN_POINT ( 'NONE',  ( 5.644368669187761256, 7.458116220610145675, 1.329639117314229235 ) ) ;
#144341=CARTESIAN_POINT ( 'NONE',  ( 4.505052181490820651, 8.477920988373101707, -0.7998128361456381397 ) ) ;
#144347=CARTESIAN_POINT ( 'NONE',  ( -6.400331034103001748, 9.624747418832267698, 1.199719254218452935 ) ) ;
#144352=CARTESIAN_POINT ( 'NONE',  ( -5.960744811863571968, 6.983232364376142698, 1.199719254218452935 ) ) ;
#144357=CARTESIAN_POINT ( 'NONE',  ( 6.712695452097489301, 7.964471127936110229, -1.082531754730548412 ) ) ;
#144358=CARTESIAN_POINT ( 'NONE',  ( -6.577113915960849155, 6.845923454808663600, -0.7216878364870338292 ) ) ;
#144365=CARTESIAN_POINT ( 'NONE',  ( 4.016958651398847557, 7.908478536599129249, -0.7998128361456362523 ) ) ;
#144373=EDGE_CURVE ( 'NONE', #41882, #47264, #170889, .T. ) ;
#144375=CARTESIAN_POINT ( 'NONE',  ( -2.299988384273672803, 2.756689234775647979, -2.499999999999998668 ) ) ;
#144395=CARTESIAN_POINT ( 'NONE',  ( 4.746850994788568201, 8.189453717816405742, 0.7312505120831546135 ) ) ;
#144403=CARTESIAN_POINT ( 'NONE',  ( 7.178115983792402233, 7.339166500704784823, 0.7998128361456281477 ) ) ;
#144409=CARTESIAN_POINT ( 'NONE',  ( -4.976059700032323896, 7.958698620104867061, 1.042642055368933285 ) ) ;
#144414=CARTESIAN_POINT ( 'NONE',  ( -4.950135482320929370, 5.908151163196758482, -1.082531754730549967 ) ) ;
#144424=CARTESIAN_POINT ( 'NONE',  ( -4.329849954717889915, 6.144853928627882489, 1.599625672291270506 ) ) ;
#144426=CARTESIAN_POINT ( 'NONE',  ( 7.374709211190586089, 7.568525266002632534, 0.000000000000000000 ) ) ;
#144434=CARTESIAN_POINT ( 'NONE',  ( 4.193214648376505593, 8.114110533073061404, 0.000000000000000000 ) ) ;
#144437=CARTESIAN_POINT ( 'NONE',  ( 6.183927461164522299, 6.387205924212962849, 0.000000000000000000 ) ) ;
#144446=CARTESIAN_POINT ( 'NONE',  ( -6.496151039430258400, 6.761311432142845135, -0.1280508955800782056 ) ) ;
#144447=DIRECTION ( 'NONE',  ( 7.105427357601001859E-15, 0.000000000000000000, 1.000000000000000000 ) ) ;
#144453=CARTESIAN_POINT ( 'NONE',  ( -4.634908411025374875, 6.500755460986618495, 1.599625672291263179 ) ) ;
#144454=CARTESIAN_POINT ( 'NONE',  ( 6.048345925472166762, 10.07050432311064903, 0.7216878364870317197 ) ) ;
#144465=CARTESIAN_POINT ( 'NONE',  ( -6.557303570864871034, 7.679217583210999010, -1.199719254218452047 ) ) ;
#144466=CARTESIAN_POINT ( 'NONE',  ( -4.797606254389363833, 6.690569611577942943, 1.599625672291263179 ) ) ;
#144468=CARTESIAN_POINT ( 'NONE',  ( 6.983858524370772258, 9.241197259889668558, 1.443375672974063439 ) ) ;
#144478=CARTESIAN_POINT ( 'NONE',  ( -5.543397514969483630, 7.443247485022737031, -1.247832777738608678 ) ) ;
#144479=PLANE ( 'NONE',  #91496 ) ;
#144483=EDGE_CURVE ( 'NONE', #89251, #154238, #206397, .T. ) ;
#144487=CARTESIAN_POINT ( 'NONE',  ( -5.759181390754928742, 9.941071732514568993, 0.000000000000000000 ) ) ;
#144494=CARTESIAN_POINT ( 'NONE',  ( 5.736508392357904107, 5.865217010605237924, 0.000000000000000000 ) ) ;
#144504=CARTESIAN_POINT ( 'NONE',  ( 6.180537922983273091, 8.303989891604203422, -1.599625672291281386 ) ) ;
#144538=CARTESIAN_POINT ( 'NONE',  ( 4.848976215542928792, 5.686169002002086970, 1.199719254218452047 ) ) ;
#144567=CARTESIAN_POINT ( 'NONE',  ( -5.468734858265826837, 7.473552982767158070, 1.599625672291263179 ) ) ;
#144569=CARTESIAN_POINT ( 'NONE',  ( 5.682275777458829502, 9.643422483761748154, 0.7216878364870317197 ) ) ;
#144574=CARTESIAN_POINT ( 'NONE',  ( -3.644109427023046521, 7.473487774827342278, 0.000000000000000000 ) ) ;
#144579=CARTESIAN_POINT ( 'NONE',  ( -2.972980823146582186, 6.690504403638126263, 0.000000000000000000 ) ) ;
#144586=CARTESIAN_POINT ( 'NONE',  ( -6.310394152517827315, 6.326824364217716656, 0.7998128361456281477 ) ) ;
#144596=CARTESIAN_POINT ( 'NONE',  ( -5.659602779061863487, 5.567567761852417085, 0.7998128361456281477 ) ) ;
#144599=CARTESIAN_POINT ( 'NONE',  ( -5.153507786970267013, 8.066157280557016307, -1.082531754730549967 ) ) ;
#144600=CARTESIAN_POINT ( 'NONE',  ( -7.282137903871469753, 8.628820655005750240, 1.082531754730549078 ) ) ;
#144601=CARTESIAN_POINT ( 'NONE',  ( 6.873057527484919937, 6.983264968346048818, 0.7998128361456352531 ) ) ;
#144602=CARTESIAN_POINT ( 'NONE',  ( -5.986807348886189040, 9.142303119412650503, -1.199719254218452047 ) ) ;
#144639=CARTESIAN_POINT ( 'NONE',  ( 4.771426152247889796, 8.279957873513081879, -0.8122977234717634332 ) ) ;
#144646=ADVANCED_FACE ( 'NONE', ( #11821 ), #182894, .T. ) ;
#144653=CARTESIAN_POINT ( 'NONE',  ( 7.523848900940885542, 7.742521570711348389, 0.7998128361456291469 ) ) ;
#144656=CARTESIAN_POINT ( 'NONE',  ( -5.438755897737433287, 6.374245297895642537, -1.199719254218453823 ) ) ;
#144660=CARTESIAN_POINT ( 'NONE',  ( -7.905812970100109638, 8.396072351304486148, 0.7216878364870317197 ) ) ;
#144672=CARTESIAN_POINT ( 'NONE',  ( 7.614839552730775729, 8.913009562054615031, 1.199719254218452047 ) ) ;
#144673=CARTESIAN_POINT ( 'NONE',  ( 6.703580607314123085, 6.785541894813420072, 0.000000000000000000 ) ) ;
#144689=CARTESIAN_POINT ( 'NONE',  ( 4.688087255275310561, 8.691461907788344377, -0.7998128361456381397 ) ) ;
#144703=CARTESIAN_POINT ( 'NONE',  ( -4.990809943606273613, 7.876343129965691858, -1.082531754730549967 ) ) ;
#144704=CARTESIAN_POINT ( 'NONE',  ( -7.449279056065764237, 7.655523418356991350, 0.7998128361456341429 ) ) ;
#144706=CARTESIAN_POINT ( 'NONE',  ( -4.815081012084855061, 4.880956980543525781, 0.4525137542755679476 ) ) ;
#144715=CARTESIAN_POINT ( 'NONE',  ( -2.823841133396259639, 6.516508098929413961, -0.7998128361456481317 ) ) ;
#144716=CARTESIAN_POINT ( 'NONE',  ( 6.607619761813720238, 8.802252036906432764, 1.599625672291268286 ) ) ;
#144719=CARTESIAN_POINT ( 'NONE',  ( 3.567203813726958828, 6.215469311773181182, 1.082531754730549078 ) ) ;
#144739=CARTESIAN_POINT ( 'NONE',  ( 6.249382461256315580, 6.255644057745969988, -0.7998128361456481317 ) ) ;
#144741=CARTESIAN_POINT ( 'NONE',  ( -3.156015896931072540, 6.904045323053366268, 0.000000000000000000 ) ) ;
#144744=CARTESIAN_POINT ( 'NONE',  ( 6.412080304620304538, 6.445458208337293549, -0.7998128361456481317 ) ) ;
#144754=CARTESIAN_POINT ( 'NONE',  ( 6.699137298928145690, 8.909022496873262753, 1.443375672974065660 ) ) ;
#144756=CARTESIAN_POINT ( 'NONE',  ( -7.605197822622922210, 7.837428646007010613, -0.7998128361456362523 ) ) ;
#144757=CARTESIAN_POINT ( 'NONE',  ( 4.193214648376505593, 8.114110533073061404, 0.000000000000000000 ) ) ;
#144767=CARTESIAN_POINT ( 'NONE',  ( -5.093022980588950865, 5.970890227889075419, -1.199719254218453823 ) ) ;
#144786=ADVANCED_FACE ( 'NONE', ( #32548 ), #175964, .T. ) ;
#144796=CARTESIAN_POINT ( 'NONE',  ( 5.397554552016226914, 6.430140077841320689, 1.082531754730549078 ) ) ;
#144803=CARTESIAN_POINT ( 'NONE',  ( 5.356880090730872013, 6.382686539675070492, 1.082531754730549078 ) ) ;
#144814=CARTESIAN_POINT ( 'NONE',  ( -6.642568916052639771, 6.714361588341672515, 0.000000000000000000 ) ) ;
#144816=CARTESIAN_POINT ( 'NONE',  ( -8.086512275908061653, 8.398962174839683215, 0.000000000000000000 ) ) ;
#144823=CARTESIAN_POINT ( 'NONE',  ( 7.876360894896227371, 8.153785563659219804, -0.7998128361456341429 ) ) ;
#144828=CARTESIAN_POINT ( 'NONE',  ( -4.776215253764153346, 8.794277906025310898, -0.7998128361456362523 ) ) ;
#144834=CARTESIAN_POINT ( 'NONE',  ( -5.316205630334268406, 6.335233002545657577, -1.082531754730549967 ) ) ;
#144840=CARTESIAN_POINT ( 'NONE',  ( -4.125423880308188629, 8.035021303660014880, -0.7998128361456481317 ) ) ;
#144858=CARTESIAN_POINT ( 'NONE',  ( -5.433785704026946384, 9.561443431331920095, 0.000000000000000000 ) ) ;
#144860=CARTESIAN_POINT ( 'NONE',  ( -4.359828915246279024, 7.244161613499399799, -1.199719254218455378 ) ) ;
#144885=CARTESIAN_POINT ( 'NONE',  ( -7.130662446144611977, 7.283804040115648526, 0.000000000000000000 ) ) ;
#144909=CARTESIAN_POINT ( 'NONE',  ( 5.830888582329017744, 8.960397891762626799, -1.199719254218452047 ) ) ;
#144910=DIRECTION ( 'NONE',  ( 0.000000000000000000, -1.000000000000000000, 0.000000000000000000 ) ) ;
#144923=CARTESIAN_POINT ( 'NONE',  ( 5.840936731490688594, 7.196517624969346549, 1.161314407385056313 ) ) ;
#144925=CARTESIAN_POINT ( 'NONE',  ( 6.617788377246179188, 8.814115421577600529, -1.443375672974078761 ) ) ;
#144930=AXIS2_PLACEMENT_3D ( 'NONE', #96470, #162519, #47714 ) ;
#144931=CARTESIAN_POINT ( 'NONE',  ( -6.296835998904160014, 6.311006518335105397, 0.000000000000000000 ) ) ;
#144938=CARTESIAN_POINT ( 'NONE',  ( -5.275531169048895741, 9.168887107283438809, -0.7216878364870338292 ) ) ;
#144944=CARTESIAN_POINT ( 'NONE',  ( -5.171509248969888617, 4.998125310078441075, 0.7998128361456281477 ) ) ;
#144954=CARTESIAN_POINT ( 'NONE',  ( 7.991605200612358573, 8.288237253661408843, 0.7998128361456281477 ) ) ;
#144958=ORIENTED_EDGE ( 'NONE', *, *, #93445, .T. ) ;
#144968=DIRECTION ( 'NONE',  ( -0.8271092603133229915, -0.5620411653108230432, -0.000000000000000000 ) ) ;
#144976=CARTESIAN_POINT ( 'NONE',  ( 7.340813827156391191, 7.528980651296110160, 0.7998128361456281477 ) ) ;
#144979=CARTESIAN_POINT ( 'NONE',  ( -6.286530415420750195, 6.898050863092263896, 0.7571273896394186131 ) ) ;
#144985=CARTESIAN_POINT ( 'NONE',  ( 4.044074958626150185, 7.940114228364351767, 0.7998128361456271485 ) ) ;
#144994=CARTESIAN_POINT ( 'NONE',  ( 5.072158865288245444, 5.090142562357324429, 0.7216878364870338292 ) ) ;
#144998=CARTESIAN_POINT ( 'NONE',  ( 6.224601922449876312, 6.434659462379210382, 0.000000000000000000 ) ) ;
#145009=CARTESIAN_POINT ( 'NONE',  ( -6.292392690518214593, 7.474117906093608710, -1.082531754730549967 ) ) ;
#145014=CARTESIAN_POINT ( 'NONE',  ( 5.553597010146855695, 5.912075037831448832, 0.6282849591137803502 ) ) ;
#145032=CARTESIAN_POINT ( 'NONE',  ( 3.715983187065167392, 7.557340494876523707, 0.6407673408501418644 ) ) ;
#145042=CARTESIAN_POINT ( 'NONE',  ( 4.518610335104485287, 8.493738834255713854, 0.000000000000000000 ) ) ;
#145045=CARTESIAN_POINT ( 'NONE',  ( 6.496291879603339758, 7.608037276739255006, 1.199719254218452935 ) ) ;
#145050=( NAMED_UNIT ( * ) PLANE_ANGLE_UNIT ( ) SI_UNIT ( $, .RADIAN. ) );
#145056=CARTESIAN_POINT ( 'NONE',  ( -2.823841133396259639, 6.516508098929413961, -0.7998128361456481317 ) ) ;
#145059=CARTESIAN_POINT ( 'NONE',  ( 5.546694241322223107, 5.643767167730274537, -0.7216878364870458196 ) ) ;
#145076=CARTESIAN_POINT ( 'NONE',  ( -4.800995793014949165, 8.615262501910491366, 0.7216878364870267237 ) ) ;
#145078=CARTESIAN_POINT ( 'NONE',  ( -4.502716413514310290, 6.346531463890372926, -1.443375672974066548 ) ) ;
#145079=CARTESIAN_POINT ( 'NONE',  ( 4.271254376947781317, 7.121149023813882373, 1.207541395772090187 ) ) ;
#145112=CARTESIAN_POINT ( 'NONE',  ( -5.915100157312088491, 10.12297696016459092, -0.7998128361456362523 ) ) ;
#145113=CARTESIAN_POINT ( 'NONE',  ( -5.151759543144467379, 7.884679950488731492, 1.249873765817657079 ) ) ;
#145121=CARTESIAN_POINT ( 'NONE',  ( -2.844178363816758814, 6.540234867753325076, -0.7998128361456481317 ) ) ;
#145124=CARTESIAN_POINT ( 'NONE',  ( -3.332271893908731464, 7.109677319527304640, -0.7998128361456481317 ) ) ;
#145129=ORIENTED_EDGE ( 'NONE', *, *, #153640, .T. ) ;
#145138=CARTESIAN_POINT ( 'NONE',  ( 4.712340909201580885, 7.655425606447271214, -1.199719254218452047 ) ) ;
#145161=CARTESIAN_POINT ( 'NONE',  ( 6.364626766972446781, 6.390095747748157251, 0.7998128361456352531 ) ) ;
#145162=CARTESIAN_POINT ( 'NONE',  ( 3.237364818613055473, 6.998952398349030268, -1.734723475976807094E-15 ) ) ;
#145164=CARTESIAN_POINT ( 'NONE',  ( 2.891631901464575272, 6.595597328342462262, 0.000000000000000000 ) ) ;
#145177=CARTESIAN_POINT ( 'NONE',  ( 5.323208952783781811, 7.729862296028469970, 1.309151360253474339 ) ) ;
#145179=CARTESIAN_POINT ( 'NONE',  ( -5.058600711230246461, 7.955432358860325515, 1.082531754730549967 ) ) ;
#145201=CARTESIAN_POINT ( 'NONE',  ( -5.607791805026555387, 5.591516722556655772, -0.3863011750756854545 ) ) ;
#145207=CARTESIAN_POINT ( 'NONE',  ( 6.391743074199808916, 6.421731439513382433, -0.7998128361456481317 ) ) ;
#145209=CARTESIAN_POINT ( 'NONE',  ( 4.329849954717849947, 6.144853928627882489, 1.599625672291262513 ) ) ;
#145226=CARTESIAN_POINT ( 'NONE',  ( -5.935437387732586778, 10.14670372898850381, -0.7998128361456362523 ) ) ;
#145237=CARTESIAN_POINT ( 'NONE',  ( 6.391743074199808916, 6.421731439513382433, -0.7998128361456481317 ) ) ;
#145243=CARTESIAN_POINT ( 'NONE',  ( 6.886615681098613884, 6.999082814228660077, 0.000000000000000000 ) ) ;
#145255=CARTESIAN_POINT ( 'NONE',  ( 4.661274270878652537, 8.290979908523663511, 0.5017903844357074483 ) ) ;
#145268=CARTESIAN_POINT ( 'NONE',  ( -6.282293365727707801, 6.900897561460068275, 0.7630008232915044264 ) ) ;
#145276=CARTESIAN_POINT ( 'NONE',  ( -6.629010762438975135, 6.698543742459062145, -0.7998128361456362523 ) ) ;
#145278=CARTESIAN_POINT ( 'NONE',  ( 4.538947565524982686, 8.517465603079630299, 0.000000000000000000 ) ) ;
#145282=CARTESIAN_POINT ( 'NONE',  ( -7.262327558775498737, 8.501745569106741840, 1.199719254218452047 ) ) ;
#145286=CARTESIAN_POINT ( 'NONE',  ( 6.230854113932139171, 9.427024345299638952, 1.199719254218452047 ) ) ;
#145292=CARTESIAN_POINT ( 'NONE',  ( -0.3989295472767397932, 3.108275709649451102, -2.025156007033537708 ) ) ;
#145309=CARTESIAN_POINT ( 'NONE',  ( 4.882344714696929877, 8.710169577206153591, -0.7216878364870458196 ) ) ;
#145312=EDGE_CURVE ( 'NONE', #44672, #161612, #116769, .T. ) ;
#145314=CARTESIAN_POINT ( 'NONE',  ( -7.075376061485238566, 9.347967719856493218, 1.599625672291269396 ) ) ;
#145326=CARTESIAN_POINT ( 'NONE',  ( -4.828112100242291760, 6.726159765073026264, -1.443375672974066548 ) ) ;
#145330=CARTESIAN_POINT ( 'NONE',  ( 4.199993725183334803, 8.122019456014369254, -0.7998128361456362523 ) ) ;
#145345=ORIENTED_EDGE ( 'NONE', *, *, #145827, .T. ) ;
#145349=CARTESIAN_POINT ( 'NONE',  ( 6.170369307550816806, 9.252495721234380355, 1.082531754730549967 ) ) ;
#145381=CARTESIAN_POINT ( 'NONE',  ( 2.905190055078214595, 6.611415174225076186, 0.7998128361456271485 ) ) ;
#145385=CARTESIAN_POINT ( 'NONE',  ( -3.458738584817664385, 7.049295759013638474, 0.7216878364870338292 ) ) ;
#145391=CARTESIAN_POINT ( 'NONE',  ( -5.906512197408906317, 6.919960980845699439, -1.199719254218453823 ) ) ;
#145400=CARTESIAN_POINT ( 'NONE',  ( -5.167592825464113915, 6.057888380243431570, 1.199719254218452935 ) ) ;
#145402=CARTESIAN_POINT ( 'NONE',  ( 6.344829475870412239, 6.940264737885684987, 0.8615092103797560297 ) ) ;
#145407=CARTESIAN_POINT ( 'NONE',  ( 6.866278450678116485, 6.975356045404744521, 0.000000000000000000 ) ) ;
#145413=LINE ( 'NONE', #195187, #23793 ) ;
#145414=CARTESIAN_POINT ( 'NONE',  ( -3.142457743317409680, 6.888227477170756785, 0.7998128361456352531 ) ) ;
#145419=CARTESIAN_POINT ( 'NONE',  ( -4.664887371553763096, 7.600063145858131364, -1.199719254218453823 ) ) ;
#145423=CARTESIAN_POINT ( 'NONE',  ( 6.333067150914808430, 8.481940657524365434, 1.443375672974063439 ) ) ;
#145425=CARTESIAN_POINT ( 'NONE',  ( -4.597623488365601752, 8.377994813152914944, 0.7216878364870267237 ) ) ;
#145432=CARTESIAN_POINT ( 'NONE',  ( 4.193214648376505593, 8.114110533073061404, 0.000000000000000000 ) ) ;
#145463=CARTESIAN_POINT ( 'NONE',  ( 4.826264338009964128, 8.099924789650724932, 0.8724150771263041726 ) ) ;
#145472=CARTESIAN_POINT ( 'NONE',  ( 7.503511670520385479, 7.718794801887437274, 0.7998128361456281477 ) ) ;
#145477=CARTESIAN_POINT ( 'NONE',  ( -6.190206388764837975, 6.963036634120459922, -0.8879648754220506035 ) ) ;
#145480=ORIENTED_EDGE ( 'NONE', *, *, #157268, .T. ) ;
#145483=CARTESIAN_POINT ( 'NONE',  ( -3.472296738431328134, 7.065113604896248845, 0.000000000000000000 ) ) ;
#145494=CARTESIAN_POINT ( 'NONE',  ( -5.178288325776719603, 5.006034233019745372, 0.000000000000000000 ) ) ;
#145504=CARTESIAN_POINT ( 'NONE',  ( 5.662465432362883355, 6.635239754958710989, 1.199719254218451159 ) ) ;
#145507=CARTESIAN_POINT ( 'NONE',  ( 5.736508391913541338, 6.825586224388162648, -1.082531754730548412 ) ) ;
#145520=CARTESIAN_POINT ( 'NONE',  ( -5.334207092333882017, 5.187939460669764635, 0.7998128361456281477 ) ) ;
#145521=CARTESIAN_POINT ( 'NONE',  ( 4.797606254389322089, 6.690569611577942943, 1.599625672291268286 ) ) ;
#145528=ORIENTED_EDGE ( 'NONE', *, *, #148738, .F. ) ;
#145530=ORIENTED_EDGE ( 'NONE', *, *, #131165, .F. ) ;
#145533=CARTESIAN_POINT ( 'NONE',  ( -6.505933609711270549, 8.683618192786854095, -1.599625672291271394 ) ) ;
#145534=CARTESIAN_POINT ( 'NONE',  ( 6.801350335910821165, 7.963938809097990124, 1.199719254218452047 ) ) ;
#145536=CARTESIAN_POINT ( 'NONE',  ( 4.921594424112039512, 4.706558014410965107, -0.4536484767114294936 ) ) ;
#145541=CARTESIAN_POINT ( 'NONE',  ( 4.146814880933355596, 5.931313009212638931, 1.599625672291261402 ) ) ;
#145548=CARTESIAN_POINT ( 'NONE',  ( -6.429665931644899857, 6.880618766637560668, 0.7446329532827021813 ) ) ;
#145556=CARTESIAN_POINT ( 'NONE',  ( -6.474900878978163021, 9.711745571186627402, -1.199719254218452047 ) ) ;
#145572=CARTESIAN_POINT ( 'NONE',  ( 6.099189001301251523, 8.209082816308541197, 1.599625672291268286 ) ) ;
#145598=VERTEX_POINT ( 'NONE', #92019 ) ;
#145608=CARTESIAN_POINT ( 'NONE',  ( 3.444653546323793947, 6.176457016423196222, 1.199719254218451159 ) ) ;
#145611=DIRECTION ( 'NONE',  ( -0.6507913734559641616, -0.7592566023653004592, 0.000000000000000000 ) ) ;
#145631=( BOUNDED_SURFACE ( )  B_SPLINE_SURFACE ( 1, 2, ( 
 ( #181248, #199619, #331, #114202, #33935, #180200, #149839, #66404, #1409, #32875, #80558, #197496, #98952, #31822, #165003, #196447, #211604, #113129, #81619, #16598, #161827, #166074, #15535, #198548, #212671, #95770, #50196, #100009, #64312, #30759, #116315, #182306, #130457, #48090, #132549, #117389, #147703, #213722, #162887, #183385, #14469, #131492, #67469, #82679, #187647, #135721, #34991, #167150, #202814, #22996, #171406, #39274, #19808, #52327, #203882, #137862, #151969, #3542, #71746, #138930, #53386, #69613, #134675, #122763, #204950, #2471, #89113, #37132, #105369, #201745, #101062, #18737, #54463, #155168, #6751, #56599, #136786, #119522, #72827, #84821, #150909, #186584, #120607, #68548, #200678, #118457, #184443, #36061, #154098, #102142, #168209, #85894, #185509, #103214, #4601, #38212, #104285, #169274, #20860, #86959, #170332, #153027, #70676, #21917, #88026, #5667, #55526, #121681, #194845, #108610, #95244, #12878, #25148, #107544, #161292, #213210, #91249, #64839, #90181, #190842, #78954, #24076, #163428, #13942, #172489, #146128, #40360, #156244, #106463, #140007, #177543, #212141, #47561, #29154, #188722, #7821, #30223, #73914, #42503, #189785, #206030, #57665, #123823, #145076, #41435, #157309, #173578, #211079, #113671, #62702, #179675, #147185, #128863, #15005, #96307, #207099, #129936, #58727, #31295, #162363, #97370, #46478, #8899, #112602, #178613, #124878, #80025, #74980, #141088, #63777, #195924, #81096, #196976, #201226, #133086, #19285, #33411, #130985, #85367, #17140, #99490, #32353, #132026, #199084, #4087, #181778, #180728, #165547, #51816, #151449, #48615, #36606, #168750, #98418, #164483, #149299, #116856, #50730, #200162, #135211, #84296, #114730, #3021, #198036, #34475, #182857, #16069, #100547, #880, #49666, #214247, #69089, #20353, #83217, #66946, #166620, #52867, #119002, #18212, #102692, #150381, #65878, #1952, #68013, #148245, #134154, #117934, #183928, #184980, #86438, #152503, #35540, #82153, #115789, #101617, #167684, #189271, #72297, #136269, #190325, #37689 ),
 ( #123307, #206579, #155713, #55011, #171962, #89660, #88588, #7296, #170884, #120078, #103766, #56078, #23553, #202289, #140567, #138404, #173040, #187129, #70158, #24623, #74462, #121160, #87514, #90730, #156793, #38758, #104839, #107016, #174122, #154645, #22477, #169817, #157861, #25695, #21404, #58208, #204423, #8379, #6227, #53941, #186054, #73374, #124367, #41984, #91803, #139479, #122235, #108093, #153579, #5148, #205509, #57140, #71225, #137340, #203359, #188194, #39830, #40910, #105938, #125422, #191388, #27841, #209770, #143775, #78712, #13710, #177301, #97134, #178374, #10510, #127573, #77653, #9454, #61410, #93938, #76584, #92868, #96068, #47318, #176239, #126493, #193541, #29983, #162121, #110231, #129699, #159979, #158914, #11581, #45183, #26766, #192456, #44110, #111297, #63543, #79783, #113431, #144840, #195681, #75526, #210846, #28915, #128634, #95000, #141637, #179438, #43054, #12642, #207646, #142695, #62472, #145896, #161046, #194600, #46244, #112361, #31058, #109167, #211906, #175180, #59266, #208705, #60332, #65635, #64606, #32108, #67756, #132836, #198840, #116607, #182600, #196740, #80862, #84041, #34224, #33167, #98193, #130746, #131783, #146952, #14771, #181539, #133907, #151194, #35282, #66689, #148002, #150129, #214013, #164241, #48380, #99249, #163187, #114493, #180489, #167436, #199913, #1702, #50486, #212967, #197787, #165297, #16892, #100296, #51560, #166363, #15829, #81915, #49424, #115544, #82973, #149046, #622, #17954, #117685, #183677, #101358, #19028, #36348, #85108, #2765, #68836, #134956, #200964, #52611, #118740, #184724, #38501, #120896, #138148, #139210, #55812, #103502, #20094, #202021, #168495, #136008, #203101, #87248, #54746, #4888, #3824, #169562, #104579, #190076, #153313, #152251, #70966, #23291, #56882, #102426, #8124, #140305, #69897, #53681, #186869, #88323, #22210, #171692, #106755, #121967, #86182, #123057, #21144, #5965, #170624, #119812, #154387, #72035, #137076, #185792, #189011, #206323, #204157, #187933, #39563, #40654, #172783, #105665, #74210, #89401 ) ),
 .UNSPECIFIED., .F., .F., .T. ) 
 B_SPLINE_SURFACE_WITH_KNOTS ( ( 2, 2 ),
 ( 3, 2, 2, 2, 2, 2, 2, 2, 2, 2, 2, 2, 2, 2, 2, 2, 2, 2, 2, 2, 2, 2, 2, 2, 2, 2, 2, 2, 2, 2, 2, 2, 2, 2, 2, 2, 2, 2, 2, 2, 2, 2, 2, 2, 2, 2, 2, 2, 2, 2, 2, 2, 2, 2, 2, 2, 2, 2, 2, 2, 2, 2, 2, 2, 2, 2, 2, 2, 2, 2, 2, 2, 2, 2, 2, 2, 2, 2, 2, 2, 2, 2, 2, 2, 2, 2, 2, 2, 2, 2, 2, 2, 2, 2, 2, 2, 2, 2, 2, 2, 2, 2, 2, 2, 2, 2, 2, 2, 2, 2, 2, 2, 2, 2, 2, 2, 2, 2, 2, 2, 3 ),
 ( 0.000000000000000000, 1.000000000000000000 ),
 ( 0.000000000000000000, 0.008333333333333333218, 0.01666666666666666644, 0.02500000000000000139, 0.03333333333333333287, 0.04166666666666666435, 0.05000000000000000278, 0.05833333333333333426, 0.06666666666666666574, 0.07499999999999999722, 0.08333333333333332871, 0.09166666666666666019, 0.1000000000000000056, 0.1083333333333333370, 0.1166666666666666685, 0.1250000000000000000, 0.1333333333333333315, 0.1416666666666666630, 0.1499999999999999944, 0.1583333333333333259, 0.1666666666666666574, 0.1749999999999999889, 0.1833333333333333204, 0.1916666666666666796, 0.2000000000000000111, 0.2083333333333333426, 0.2166666666666666741, 0.2250000000000000056, 0.2333333333333333370, 0.2416666666666666685, 0.2500000000000000000, 0.2583333333333333592, 0.2666666666666666630, 0.2750000000000000222, 0.2833333333333333259, 0.2916666666666666852, 0.2999999999999999889, 0.3083333333333333481, 0.3166666666666666519, 0.3250000000000000111, 0.3333333333333333148, 0.3416666666666666741, 0.3499999999999999778, 0.3583333333333333370, 0.3666666666666666408, 0.3750000000000000000, 0.3833333333333333592, 0.3916666666666666630, 0.4000000000000000222, 0.4083333333333333259, 0.4166666666666666852, 0.4249999999999999889, 0.4333333333333333481, 0.4416666666666666519, 0.4500000000000000111, 0.4583333333333333148, 0.4666666666666666741, 0.4749999999999999778, 0.4833333333333333370, 0.4916666666666666408, 0.5000000000000000000, 0.5083333333333333037, 0.5166666666666667185, 0.5250000000000000222, 0.5333333333333333259, 0.5416666666666666297, 0.5500000000000000444, 0.5583333333333333481, 0.5666666666666666519, 0.5749999999999999556, 0.5833333333333333703, 0.5916666666666666741, 0.5999999999999999778, 0.6083333333333332815, 0.6166666666666666963, 0.6250000000000000000, 0.6333333333333333037, 0.6416666666666667185, 0.6500000000000000222, 0.6583333333333333259, 0.6666666666666666297, 0.6750000000000000444, 0.6833333333333333481, 0.6916666666666666519, 0.6999999999999999556, 0.7083333333333333703, 0.7166666666666666741, 0.7249999999999999778, 0.7333333333333332815, 0.7416666666666666963, 0.7500000000000000000, 0.7583333333333333037, 0.7666666666666667185, 0.7750000000000000222, 0.7833333333333333259, 0.7916666666666666297, 0.8000000000000000444, 0.8083333333333333481, 0.8166666666666666519, 0.8249999999999999556, 0.8333333333333333703, 0.8416666666666666741, 0.8499999999999999778, 0.8583333333333332815, 0.8666666666666666963, 0.8750000000000000000, 0.8833333333333333037, 0.8916666666666667185, 0.9000000000000000222, 0.9083333333333333259, 0.9166666666666666297, 0.9250000000000000444, 0.9333333333333333481, 0.9416666666666666519, 0.9499999999999999556, 0.9583333333333333703, 0.9666666666666666741, 0.9749999999999999778, 0.9833333333333332815, 0.9916666666666666963, 1.000000000000000000 ),
 .UNSPECIFIED. ) 
 GEOMETRIC_REPRESENTATION_ITEM ( )  RATIONAL_B_SPLINE_SURFACE ( (
 ( 1.000000000000000000, 0.8660254037844387076, 1.000000000000000000, 0.8660254037844387076, 1.000000000000000000, 0.8660254037844387076, 1.000000000000000000, 0.8660254037844387076, 1.000000000000000000, 0.8660254037844387076, 1.000000000000000000, 0.8660254037844387076, 1.000000000000000000, 0.8660254037844387076, 1.000000000000000000, 0.8660254037844387076, 1.000000000000000000, 0.8660254037844387076, 1.000000000000000000, 0.8660254037844387076, 1.000000000000000000, 0.8660254037844387076, 1.000000000000000000, 0.8660254037844387076, 1.000000000000000000, 0.8660254037844387076, 1.000000000000000000, 0.8660254037844387076, 1.000000000000000000, 0.8660254037844387076, 1.000000000000000000, 0.8660254037844387076, 1.000000000000000000, 0.8660254037844387076, 1.000000000000000000, 0.8660254037844387076, 1.000000000000000000, 0.8660254037844387076, 1.000000000000000000, 0.8660254037844387076, 1.000000000000000000, 0.8660254037844387076, 1.000000000000000000, 0.8660254037844387076, 1.000000000000000000, 0.8660254037844387076, 1.000000000000000000, 0.8660254037844387076, 1.000000000000000000, 0.8660254037844387076, 1.000000000000000000, 0.8660254037844387076, 1.000000000000000000, 0.8660254037844387076, 1.000000000000000000, 0.8660254037844387076, 1.000000000000000000, 0.8660254037844387076, 1.000000000000000000, 0.8660254037844387076, 1.000000000000000000, 0.8660254037844387076, 1.000000000000000000, 0.8660254037844387076, 1.000000000000000000, 0.8660254037844387076, 1.000000000000000000, 0.8660254037844387076, 1.000000000000000000, 0.8660254037844387076, 1.000000000000000000, 0.8660254037844387076, 1.000000000000000000, 0.8660254037844387076, 1.000000000000000000, 0.8660254037844387076, 1.000000000000000000, 0.8660254037844387076, 1.000000000000000000, 0.8660254037844387076, 1.000000000000000000, 0.8660254037844387076, 1.000000000000000000, 0.8660254037844387076, 1.000000000000000000, 0.8660254037844387076, 1.000000000000000000, 0.8660254037844387076, 1.000000000000000000, 0.8660254037844387076, 1.000000000000000000, 0.8660254037844387076, 1.000000000000000000, 0.8660254037844387076, 1.000000000000000000, 0.8660254037844387076, 1.000000000000000000, 0.8660254037844387076, 1.000000000000000000, 0.8660254037844387076, 1.000000000000000000, 0.8660254037844387076, 1.000000000000000000, 0.8660254037844387076, 1.000000000000000000, 0.8660254037844387076, 1.000000000000000000, 0.8660254037844387076, 1.000000000000000000, 0.8660254037844387076, 1.000000000000000000, 0.8660254037844387076, 1.000000000000000000, 0.8660254037844387076, 1.000000000000000000, 0.8660254037844387076, 1.000000000000000000, 0.8660254037844387076, 1.000000000000000000, 0.8660254037844387076, 1.000000000000000000, 0.8660254037844387076, 1.000000000000000000, 0.8660254037844387076, 1.000000000000000000, 0.8660254037844387076, 1.000000000000000000, 0.8660254037844387076, 1.000000000000000000, 0.8660254037844387076, 1.000000000000000000, 0.8660254037844387076, 1.000000000000000000, 0.8660254037844387076, 1.000000000000000000, 0.8660254037844387076, 1.000000000000000000, 0.8660254037844387076, 1.000000000000000000, 0.8660254037844387076, 1.000000000000000000, 0.8660254037844387076, 1.000000000000000000, 0.8660254037844387076, 1.000000000000000000, 0.8660254037844387076, 1.000000000000000000, 0.8660254037844387076, 1.000000000000000000, 0.8660254037844387076, 1.000000000000000000, 0.8660254037844387076, 1.000000000000000000, 0.8660254037844387076, 1.000000000000000000, 0.8660254037844387076, 1.000000000000000000, 0.8660254037844387076, 1.000000000000000000, 0.8660254037844387076, 1.000000000000000000, 0.8660254037844387076, 1.000000000000000000, 0.8660254037844387076, 1.000000000000000000, 0.8660254037844387076, 1.000000000000000000, 0.8660254037844387076, 1.000000000000000000, 0.8660254037844387076, 1.000000000000000000, 0.8660254037844387076, 1.000000000000000000, 0.8660254037844387076, 1.000000000000000000, 0.8660254037844387076, 1.000000000000000000, 0.8660254037844387076, 1.000000000000000000, 0.8660254037844387076, 1.000000000000000000, 0.8660254037844387076, 1.000000000000000000, 0.8660254037844387076, 1.000000000000000000, 0.8660254037844387076, 1.000000000000000000, 0.8660254037844387076, 1.000000000000000000, 0.8660254037844387076, 1.000000000000000000, 0.8660254037844387076, 1.000000000000000000, 0.8660254037844387076, 1.000000000000000000, 0.8660254037844387076, 1.000000000000000000, 0.8660254037844387076, 1.000000000000000000, 0.8660254037844387076, 1.000000000000000000, 0.8660254037844387076, 1.000000000000000000, 0.8660254037844387076, 1.000000000000000000, 0.8660254037844387076, 1.000000000000000000, 0.8660254037844387076, 1.000000000000000000, 0.8660254037844387076, 1.000000000000000000, 0.8660254037844387076, 1.000000000000000000, 0.8660254037844387076, 1.000000000000000000, 0.8660254037844387076, 1.000000000000000000, 0.8660254037844387076, 1.000000000000000000, 0.8660254037844387076, 1.000000000000000000, 0.8660254037844387076, 1.000000000000000000, 0.8660254037844387076, 1.000000000000000000, 0.8660254037844387076, 1.000000000000000000, 0.8660254037844387076, 1.000000000000000000, 0.8660254037844387076, 1.000000000000000000, 0.8660254037844387076, 1.000000000000000000, 0.8660254037844387076, 1.000000000000000000, 0.8660254037844387076, 1.000000000000000000, 0.8660254037844387076, 1.000000000000000000, 0.8660254037844387076, 1.000000000000000000),
 ( 1.000000000000000000, 0.8660254037844387076, 1.000000000000000000, 0.8660254037844387076, 1.000000000000000000, 0.8660254037844387076, 1.000000000000000000, 0.8660254037844387076, 1.000000000000000000, 0.8660254037844387076, 1.000000000000000000, 0.8660254037844387076, 1.000000000000000000, 0.8660254037844387076, 1.000000000000000000, 0.8660254037844387076, 1.000000000000000000, 0.8660254037844387076, 1.000000000000000000, 0.8660254037844387076, 1.000000000000000000, 0.8660254037844387076, 1.000000000000000000, 0.8660254037844387076, 1.000000000000000000, 0.8660254037844387076, 1.000000000000000000, 0.8660254037844387076, 1.000000000000000000, 0.8660254037844387076, 1.000000000000000000, 0.8660254037844387076, 1.000000000000000000, 0.8660254037844387076, 1.000000000000000000, 0.8660254037844387076, 1.000000000000000000, 0.8660254037844387076, 1.000000000000000000, 0.8660254037844387076, 1.000000000000000000, 0.8660254037844387076, 1.000000000000000000, 0.8660254037844387076, 1.000000000000000000, 0.8660254037844387076, 1.000000000000000000, 0.8660254037844387076, 1.000000000000000000, 0.8660254037844387076, 1.000000000000000000, 0.8660254037844387076, 1.000000000000000000, 0.8660254037844387076, 1.000000000000000000, 0.8660254037844387076, 1.000000000000000000, 0.8660254037844387076, 1.000000000000000000, 0.8660254037844387076, 1.000000000000000000, 0.8660254037844387076, 1.000000000000000000, 0.8660254037844387076, 1.000000000000000000, 0.8660254037844387076, 1.000000000000000000, 0.8660254037844387076, 1.000000000000000000, 0.8660254037844387076, 1.000000000000000000, 0.8660254037844387076, 1.000000000000000000, 0.8660254037844387076, 1.000000000000000000, 0.8660254037844387076, 1.000000000000000000, 0.8660254037844387076, 1.000000000000000000, 0.8660254037844387076, 1.000000000000000000, 0.8660254037844387076, 1.000000000000000000, 0.8660254037844387076, 1.000000000000000000, 0.8660254037844387076, 1.000000000000000000, 0.8660254037844387076, 1.000000000000000000, 0.8660254037844387076, 1.000000000000000000, 0.8660254037844387076, 1.000000000000000000, 0.8660254037844387076, 1.000000000000000000, 0.8660254037844387076, 1.000000000000000000, 0.8660254037844387076, 1.000000000000000000, 0.8660254037844387076, 1.000000000000000000, 0.8660254037844387076, 1.000000000000000000, 0.8660254037844387076, 1.000000000000000000, 0.8660254037844387076, 1.000000000000000000, 0.8660254037844387076, 1.000000000000000000, 0.8660254037844387076, 1.000000000000000000, 0.8660254037844387076, 1.000000000000000000, 0.8660254037844387076, 1.000000000000000000, 0.8660254037844387076, 1.000000000000000000, 0.8660254037844387076, 1.000000000000000000, 0.8660254037844387076, 1.000000000000000000, 0.8660254037844387076, 1.000000000000000000, 0.8660254037844387076, 1.000000000000000000, 0.8660254037844387076, 1.000000000000000000, 0.8660254037844387076, 1.000000000000000000, 0.8660254037844387076, 1.000000000000000000, 0.8660254037844387076, 1.000000000000000000, 0.8660254037844387076, 1.000000000000000000, 0.8660254037844387076, 1.000000000000000000, 0.8660254037844387076, 1.000000000000000000, 0.8660254037844387076, 1.000000000000000000, 0.8660254037844387076, 1.000000000000000000, 0.8660254037844387076, 1.000000000000000000, 0.8660254037844387076, 1.000000000000000000, 0.8660254037844387076, 1.000000000000000000, 0.8660254037844387076, 1.000000000000000000, 0.8660254037844387076, 1.000000000000000000, 0.8660254037844387076, 1.000000000000000000, 0.8660254037844387076, 1.000000000000000000, 0.8660254037844387076, 1.000000000000000000, 0.8660254037844387076, 1.000000000000000000, 0.8660254037844387076, 1.000000000000000000, 0.8660254037844387076, 1.000000000000000000, 0.8660254037844387076, 1.000000000000000000, 0.8660254037844387076, 1.000000000000000000, 0.8660254037844387076, 1.000000000000000000, 0.8660254037844387076, 1.000000000000000000, 0.8660254037844387076, 1.000000000000000000, 0.8660254037844387076, 1.000000000000000000, 0.8660254037844387076, 1.000000000000000000, 0.8660254037844387076, 1.000000000000000000, 0.8660254037844387076, 1.000000000000000000, 0.8660254037844387076, 1.000000000000000000, 0.8660254037844387076, 1.000000000000000000, 0.8660254037844387076, 1.000000000000000000, 0.8660254037844387076, 1.000000000000000000, 0.8660254037844387076, 1.000000000000000000, 0.8660254037844387076, 1.000000000000000000, 0.8660254037844387076, 1.000000000000000000, 0.8660254037844387076, 1.000000000000000000, 0.8660254037844387076, 1.000000000000000000, 0.8660254037844387076, 1.000000000000000000, 0.8660254037844387076, 1.000000000000000000, 0.8660254037844387076, 1.000000000000000000, 0.8660254037844387076, 1.000000000000000000, 0.8660254037844387076, 1.000000000000000000, 0.8660254037844387076, 1.000000000000000000, 0.8660254037844387076, 1.000000000000000000, 0.8660254037844387076, 1.000000000000000000, 0.8660254037844387076, 1.000000000000000000, 0.8660254037844387076, 1.000000000000000000, 0.8660254037844387076, 1.000000000000000000, 0.8660254037844387076, 1.000000000000000000, 0.8660254037844387076, 1.000000000000000000, 0.8660254037844387076, 1.000000000000000000, 0.8660254037844387076, 1.000000000000000000, 0.8660254037844387076, 1.000000000000000000, 0.8660254037844387076, 1.000000000000000000, 0.8660254037844387076, 1.000000000000000000, 0.8660254037844387076, 1.000000000000000000, 0.8660254037844387076, 1.000000000000000000) ) ) 
 REPRESENTATION_ITEM ( '' )  SURFACE ( )  );
#145639=CARTESIAN_POINT ( 'NONE',  ( -5.712781623311813384, 7.758274208654143855, -1.599625672291271394 ) ) ;
#145641=CARTESIAN_POINT ( 'NONE',  ( 7.146556367734776316, 7.510272981878305387, 0.7216878364870267237 ) ) ;
#145646=CARTESIAN_POINT ( 'NONE',  ( -5.655686355556086120, 6.627330832017406692, 1.199719254218452935 ) ) ;
#145651=CARTESIAN_POINT ( 'NONE',  ( -3.902768115887413014, 5.646591783325653147, -1.599625672291283607 ) ) ;
#145656=CARTESIAN_POINT ( 'NONE',  ( -6.934069218746458318, 7.054445274817795486, -0.7998128361456362523 ) ) ;
#145666=CARTESIAN_POINT ( 'NONE',  ( -4.146814880933400005, 5.931313009212638931, 1.599625672291270506 ) ) ;
#145670=CARTESIAN_POINT ( 'NONE',  ( -4.936577329151611515, 7.813071746435248599, 1.082531754730549967 ) ) ;
#145671=CARTESIAN_POINT ( 'NONE',  ( -7.255021596644144921, 7.636815748939187465, 0.7216878364870317197 ) ) ;
#145672=CARTESIAN_POINT ( 'NONE',  ( 4.895902867866261055, 4.884510565364971413, -0.7216878364870458196 ) ) ;
#145673=CARTESIAN_POINT ( 'NONE',  ( -5.772739544368596043, 9.956889578397179363, -0.7998128361456362523 ) ) ;
#145712=CARTESIAN_POINT ( 'NONE',  ( 4.722521264130603136, 8.336029038342307018, -0.7037175076533495055 ) ) ;
#145725=CARTESIAN_POINT ( 'NONE',  ( 6.658989722967328717, 7.797851427330578566, 1.199719254218452935 ) ) ;
#145728=CARTESIAN_POINT ( 'NONE',  ( -5.061990249855848667, 6.999017606288844284, -1.599625672291271394 ) ) ;
#145732=CARTESIAN_POINT ( 'NONE',  ( -5.926322542504860458, 9.928143709648733051, -0.7216878364870338292 ) ) ;
#145742=CARTESIAN_POINT ( 'NONE',  ( 6.086684617892325733, 6.065829907154645539, -0.7998128361456481317 ) ) ;
#145744=CARTESIAN_POINT ( 'NONE',  ( 5.508355548902068577, 9.648441583686274470, 0.7998128361456331437 ) ) ;
#145753=AXIS2_PLACEMENT_3D ( 'NONE', #170483, #167299, #3686 ) ;
#145759=CARTESIAN_POINT ( 'NONE',  ( 6.886615681098613884, 6.999082814228660077, 0.000000000000000000 ) ) ;
#145769=ORIENTED_EDGE ( 'NONE', *, *, #55665, .F. ) ;
#145771=CARTESIAN_POINT ( 'NONE',  ( -5.478903473698260029, 6.525047153136981137, -1.082531754730549967 ) ) ;
#145772=CARTESIAN_POINT ( 'NONE',  ( 5.560252395380206991, 7.580323442733986283, 1.443375672974065660 ) ) ;
#145774=CARTESIAN_POINT ( 'NONE',  ( -4.826181173005540614, 4.880474388334561375, 0.4619849944318583645 ) ) ;
#145777=ORIENTED_EDGE ( 'NONE', *, *, #136243, .F. ) ;
#145782=CARTESIAN_POINT ( 'NONE',  ( -6.075462232699549325, 9.141770800574526845, 1.082531754730549967 ) ) ;
#145786=CARTESIAN_POINT ( 'NONE',  ( 8.174640274396848483, 8.501778173076651512, 0.7998128361456291469 ) ) ;
#145798=CARTESIAN_POINT ( 'NONE',  ( -5.876342332316932371, 6.610971932319779754, 0.8968535711802629873 ) ) ;
#145800=CARTESIAN_POINT ( 'NONE',  ( 5.520104819419390907, 6.469152373191302985, 1.199719254218452935 ) ) ;
#145802=CARTESIAN_POINT ( 'NONE',  ( -5.978219388983010418, 5.939287140093762574, -0.7998128361456362523 ) ) ;
#145816=CARTESIAN_POINT ( 'NONE',  ( 7.526184669361807522, 7.953172667109813077, 0.000000000000000000 ) ) ;
#145818=CARTESIAN_POINT ( 'NONE',  ( -5.745623237141265882, 9.925253886631958622, 0.7998128361456291469 ) ) ;
#145819=CARTESIAN_POINT ( 'NONE',  ( 6.717138760927786834, 6.801359740696030443, -0.7998128361456481317 ) ) ;
#145827=EDGE_CURVE ( 'NONE', #203624, #78850, #107243, .T. ) ;
#145828=CARTESIAN_POINT ( 'NONE',  ( -5.255720823952942489, 6.160704378480398979, -1.199719254218453823 ) ) ;
#145831=CARTESIAN_POINT ( 'NONE',  ( -0.3866901564497978727, 3.102326550341739875, 2.027579305719746205 ) ) ;
#145850=AXIS2_PLACEMENT_3D ( 'NONE', #25837, #126631, #209907 ) ;
#145856=CARTESIAN_POINT ( 'NONE',  ( 4.529832720741620022, 7.338536369956936589, -1.082531754730548412 ) ) ;
#145862=CARTESIAN_POINT ( 'NONE',  ( 3.879041346841291649, 7.539648981374564407, 1.040834085586084257E-14 ) ) ;
#145873=CARTESIAN_POINT ( 'NONE',  ( -7.117104292530948229, 7.267986194233038155, -0.7998128361456362523 ) ) ;
#145875=CARTESIAN_POINT ( 'NONE',  ( -6.129167961829681488, 9.308390501180058507, -1.199719254218452047 ) ) ;
#145881=CARTESIAN_POINT ( 'NONE',  ( 4.895902867866261055, 4.884510565364971413, -0.7216878364870458196 ) ) ;
#145886=CARTESIAN_POINT ( 'NONE',  ( -4.749098946536820520, 8.762642214260091933, 0.7998128361456281477 ) ) ;
#145892=CARTESIAN_POINT ( 'NONE',  ( -4.001064729808656573, 7.682009594836471500, 1.214306433183764966E-14 ) ) ;
#145896=CARTESIAN_POINT ( 'NONE',  ( -5.367048706163331850, 7.354919138647580290, -1.599625672291271394 ) ) ;
#145916=CARTESIAN_POINT ( 'NONE',  ( -6.420668264523499147, 9.648474187656182366, 1.199719254218452935 ) ) ;
#145917=CARTESIAN_POINT ( 'NONE',  ( 5.246079093845007257, 5.085123462432798114, 0.7998128361456352531 ) ) ;
#145918=CARTESIAN_POINT ( 'NONE',  ( -3.871735385154307263, 6.674719161725423788, -1.199719254218450271 ) ) ;
#145927=DIRECTION ( 'NONE',  ( 0.000000000000000000, 0.000000000000000000, 1.000000000000000000 ) ) ;
#145942=CARTESIAN_POINT ( 'NONE',  ( -6.607619761813764647, 8.802252036906432764, 1.599625672291269396 ) ) ;
#145949=CARTESIAN_POINT ( 'NONE',  ( 3.894033820048787398, 8.999999999999998224, 0.7749999999999996891 ) ) ;
#145967=CARTESIAN_POINT ( 'NONE',  ( 6.668631453075247073, 8.873432343378178544, -1.599625672291281386 ) ) ;
#145979=CARTESIAN_POINT ( 'NONE',  ( 4.798147134389644464, 8.131168186839138556, 0.8272934513729796047 ) ) ;
#145982=CARTESIAN_POINT ( 'NONE',  ( 6.211043768836170820, 9.299949259400630552, 1.082531754730549967 ) ) ;
#145988=CARTESIAN_POINT ( 'NONE',  ( -6.283277845290492714, 6.295188672452495915, -0.7998128361456362523 ) ) ;
#145993=CARTESIAN_POINT ( 'NONE',  ( -6.061904078641520144, 10.08632216847484031, 0.7216878364870267237 ) ) ;
#146002=CARTESIAN_POINT ( 'NONE',  ( -3.962726036944197894, 7.845207153068690431, -0.7998128361456481317 ) ) ;
#146011=CARTESIAN_POINT ( 'NONE',  ( 4.492547798081839794, 6.334668079219206049, 1.599625672291262513 ) ) ;
#146034=CARTESIAN_POINT ( 'NONE',  ( 7.180978637093494044, 8.406838493811077839, -1.199719254218452047 ) ) ;
#146035=CARTESIAN_POINT ( 'NONE',  ( -5.804269833667989431, 7.239147048582937671, 1.181955602297209751 ) ) ;
#146041=CARTESIAN_POINT ( 'NONE',  ( 4.908934136599710563, 7.884784371745123366, 1.199719254218451159 ) ) ;
#146044=CARTESIAN_POINT ( 'NONE',  ( -5.546112223000226216, 5.929839062422638918, -0.8878705470019981894 ) ) ;
#146051=CARTESIAN_POINT ( 'NONE',  ( 4.882344714696929877, 8.710169577206153591, -0.7216878364870458196 ) ) ;
#146062=CARTESIAN_POINT ( 'NONE',  ( -4.475600106286965918, 8.235634200727838916, 0.7216878364870338292 ) ) ;
#146087=CARTESIAN_POINT ( 'NONE',  ( 5.598048612495534648, 5.756137568112394298, 0.6639549446901950036 ) ) ;
#146098=CARTESIAN_POINT ( 'NONE',  ( 6.039231080244466199, 6.010467446565510130, 0.7998128361456352531 ) ) ;
#146100=CARTESIAN_POINT ( 'NONE',  ( 4.712340909201580885, 7.655425606447271214, -1.199719254218452047 ) ) ;
#146111=CARTESIAN_POINT ( 'NONE',  ( -6.563555762791521531, 9.711213252348503744, 1.082531754730549967 ) ) ;
#146114=CARTESIAN_POINT ( 'NONE',  ( 4.489158259456265121, 7.291082831790689056, -1.082531754730548412 ) ) ;
#146128=CARTESIAN_POINT ( 'NONE',  ( -6.455090533882213322, 6.703562842383589349, -0.7216878364870338292 ) ) ;
#146130=CARTESIAN_POINT ( 'NONE',  ( -4.123088112331656951, 6.864000993478624579, 1.082531754730549967 ) ) ;
#146157=CARTESIAN_POINT ( 'NONE',  ( -5.004894982100124068, 5.868074229652107121, 1.199719254218452935 ) ) ;
#146164=CARTESIAN_POINT ( 'NONE',  ( 3.879041346841291649, 7.539648981374564407, 1.040834085586084257E-14 ) ) ;
#146167=CARTESIAN_POINT ( 'NONE',  ( -5.399890319992785237, 9.521898816625391504, 0.7998128361456291469 ) ) ;
#146168=CARTESIAN_POINT ( 'NONE',  ( -5.468737822882341781, 7.600800700804905219, 1.347914668206271038 ) ) ;
#146176=CARTESIAN_POINT ( 'NONE',  ( -4.899292406491858820, 6.809203455697518947, -1.599625672291271394 ) ) ;
#146183=CARTESIAN_POINT ( 'NONE',  ( -6.423886587202998655, 6.778203476158441987, 0.4838116631791135602 ) ) ;
#146190=CARTESIAN_POINT ( 'NONE',  ( 5.387385936583818591, 7.378645907471495846, -1.599625672291283607 ) ) ;
#146196=CARTESIAN_POINT ( 'NONE',  ( -0.04573888721146443515, 3.402170834691579770, -2.080515066271528823 ) ) ;
#146204=CARTESIAN_POINT ( 'NONE',  ( 5.063152511717405879, 4.908155404373435005, -0.2552525419090029835 ) ) ;
#146215=CARTESIAN_POINT ( 'NONE',  ( 4.342354338126830804, 8.288106837781779035, -0.7998128361456381397 ) ) ;
#146216=CARTESIAN_POINT ( 'NONE',  ( 4.923546060418115822, 5.773167154356443120, -1.199719254218452047 ) ) ;
#146230=CARTESIAN_POINT ( 'NONE',  ( 4.690754089986846509, 8.373302309308519042, 0.6171781843518510113 ) ) ;
#146231=CARTESIAN_POINT ( 'NONE',  ( -4.936577328707246082, 8.773440960218172435, 0.000000000000000000 ) ) ;
#146239=ADVANCED_FACE ( 'NONE', ( #214221 ), #20323, .F. ) ;
#146260=CARTESIAN_POINT ( 'NONE',  ( 4.420840606507738357, 7.315341919971147355, 1.199719254218451159 ) ) ;
#146263=CARTESIAN_POINT ( 'NONE',  ( 3.061108821635398769, 6.793320401875094561, -0.7998128361456362523 ) ) ;
#146282=CARTESIAN_POINT ( 'NONE',  ( -6.420668264523499147, 9.648474187656182366, 1.199719254218452935 ) ) ;
#146293=CARTESIAN_POINT ( 'NONE',  ( 6.527324610336440180, 6.579909898339485252, 0.7998128361456331437 ) ) ;
#146297=CARTESIAN_POINT ( 'NONE',  ( 6.412080304620304538, 6.445458208337293549, -0.7998128361456481317 ) ) ;
#146306=CARTESIAN_POINT ( 'NONE',  ( 4.595929827128614420, 8.372548788374160722, -0.07784623617661419470 ) ) ;
#146312=PLANE ( 'NONE',  #184219 ) ;
#146314=CARTESIAN_POINT ( 'NONE',  ( 4.393008644795362905, 7.016788222801661590, 1.284222742053114041 ) ) ;
#146319=CARTESIAN_POINT ( 'NONE',  ( -6.101747606705155924, 7.024000329443246926, 0.9821876679783679842 ) ) ;
#146322=ORIENTED_EDGE ( 'NONE', *, *, #13102, .T. ) ;
#146326=CARTESIAN_POINT ( 'NONE',  ( -6.818824913030298696, 6.919993584815607335, 0.7998128361456341429 ) ) ;
#146328=CARTESIAN_POINT ( 'NONE',  ( 4.227110032410640095, 8.153655147779589996, 0.7998128361456271485 ) ) ;
#146333=CARTESIAN_POINT ( 'NONE',  ( -7.099629715411508890, 8.311931418515415615, 1.199719254218452047 ) ) ;
#146342=CARTESIAN_POINT ( 'NONE',  ( -0.2953305167033711820, 3.289220156445278320, -2.050567765197571113 ) ) ;
#146351=EDGE_CURVE ( 'NONE', #30079, #184155, #112934, .T. ) ;
#146354=DIRECTION ( 'NONE',  ( 0.000000000000000000, 1.000000000000000000, 0.000000000000000000 ) ) ;
#146359=CARTESIAN_POINT ( 'NONE',  ( 6.102578539926878598, 7.252668063737060855, -1.082531754730548412 ) ) ;
#146362=CARTESIAN_POINT ( 'NONE',  ( -8.100070429521727178, 8.414780020722290033, 0.7998128361456341429 ) ) ;
#146373=CARTESIAN_POINT ( 'NONE',  ( -3.363831509966360489, 6.938570838353784076, -0.7216878364870458196 ) ) ;
#146376=CARTESIAN_POINT ( 'NONE',  ( 6.550524494058025837, 7.671308660269694712, -1.199719254218452047 ) ) ;
#146390=EDGE_LOOP ( 'NONE', ( #87361, #188562, #205275 ) ) ;
#146400=EDGE_CURVE ( 'NONE', #90832, #22501, #109530, .T. ) ;
#146431=CARTESIAN_POINT ( 'NONE',  ( -4.407809337774280856, 7.196175756495025055, 1.082531754730549967 ) ) ;
#146438=CARTESIAN_POINT ( 'NONE',  ( -5.367048706163331850, 7.354919138647580290, -1.599625672291271394 ) ) ;
#146445=DIRECTION ( 'NONE',  ( -0.6507913734559641616, -0.7592566023653004592, 0.000000000000000000 ) ) ;
#146446=CARTESIAN_POINT ( 'NONE',  ( -6.005335696210345020, 5.970922831858983315, 0.7998128361456281477 ) ) ;
#146448=CARTESIAN_POINT ( 'NONE',  ( 6.270956187569860063, 6.991113019333711875, 0.9580997929081371822 ) ) ;
#146453=CARTESIAN_POINT ( 'NONE',  ( 5.825163275726873202, 6.825053905550038991, 1.199719254218452047 ) ) ;
#146458=ORIENTED_EDGE ( 'NONE', *, *, #44801, .F. ) ;
#146461=CARTESIAN_POINT ( 'NONE',  ( -5.679940009482361774, 5.591294530676332641, 0.7998128361456281477 ) ) ;
#146465=CARTESIAN_POINT ( 'NONE',  ( -4.749098946536820520, 8.762642214260091933, 0.7998128361456281477 ) ) ;
#146468=CARTESIAN_POINT ( 'NONE',  ( 5.844973620822830895, 8.872867420051733234, 1.082531754730549967 ) ) ;
#146470=CARTESIAN_POINT ( 'NONE',  ( -5.844973620822877969, 7.912498205750389424, 1.443375672974058777 ) ) ;
#146477=CARTESIAN_POINT ( 'NONE',  ( 5.662465432362883355, 6.635239754958710989, 1.199719254218451159 ) ) ;
#146484=DIRECTION ( 'NONE',  ( -0.6507913734559658270, -0.7592566023652989049, 0.000000000000000000 ) ) ;
#146523=CARTESIAN_POINT ( 'NONE',  ( -5.917914848013369422, 7.154962168230770025, -1.123475595150375650 ) ) ;
#146532=CARTESIAN_POINT ( 'NONE',  ( -6.071018923869249129, 10.30488218781460574, 0.7998128361456291469 ) ) ;
#146544=CARTESIAN_POINT ( 'NONE',  ( -5.015590482412729756, 4.816220082428420923, 0.000000000000000000 ) ) ;
#146553=CARTESIAN_POINT ( 'NONE',  ( 4.529305835417093640, 7.441884687032027657, -1.199719254218450271 ) ) ;
#146556=CARTESIAN_POINT ( 'NONE',  ( 6.333067150914808430, 8.481940657524365434, 1.443375672974063439 ) ) ;
#146571=CARTESIAN_POINT ( 'NONE',  ( -4.599959256786493533, 8.588645909551377855, 0.000000000000000000 ) ) ;
#146572=CARTESIAN_POINT ( 'NONE',  ( 3.705121118284530279, 7.544668081299086282, -1.734723475976807094E-15 ) ) ;
#146584=CARTESIAN_POINT ( 'NONE',  ( -6.774234028683526532, 7.932303117332766718, 1.199719254218452047 ) ) ;
#146585=CARTESIAN_POINT ( 'NONE',  ( 4.993145711582793744, 9.047363440147082159, -0.7998128361456481317 ) ) ;
#146590=CARTESIAN_POINT ( 'NONE',  ( 5.174371902270911150, 6.065797303184739420, 1.199719254218452047 ) ) ;
#146592=CARTESIAN_POINT ( 'NONE',  ( -0.1435606456237618622, 2.537783136032443654, 1.995875440081346097 ) ) ;
#146596=CARTESIAN_POINT ( 'NONE',  ( -6.584207447892295839, 6.778236197985048506, 0.3223495580488393575 ) ) ;
#146600=CARTESIAN_POINT ( 'NONE',  ( 2.891631901464575272, 6.595597328342462262, 0.000000000000000000 ) ) ;
#146604=CARTESIAN_POINT ( 'NONE',  ( -6.933015448541747006, 9.181880338089085214, 1.599625672291269396 ) ) ;
#146610=DIRECTION ( 'NONE',  ( 0.000000000000000000, -1.000000000000000000, 0.000000000000000000 ) ) ;
#146656=CARTESIAN_POINT ( 'NONE',  ( 4.686278372178935392, 5.496354851410763409, 1.199719254218452047 ) ) ;
#146686=CARTESIAN_POINT ( 'NONE',  ( -6.493429226302317225, 6.540365283632955773, 0.7998128361456341429 ) ) ;
#146688=CARTESIAN_POINT ( 'NONE',  ( 5.356880090730850696, 9.263794182579101033, 0.7216878364870317197 ) ) ;
#146693=CARTESIAN_POINT ( 'NONE',  ( -4.782994330570982555, 8.802186828966616972, 0.000000000000000000 ) ) ;
#146698=CARTESIAN_POINT ( 'NONE',  ( -3.962726036944197894, 7.845207153068690431, -0.7998128361456481317 ) ) ;
#146703=CARTESIAN_POINT ( 'NONE',  ( -4.827585214917754719, 7.789877296449459365, -1.199719254218453823 ) ) ;
#146714=CARTESIAN_POINT ( 'NONE',  ( -5.581116510680924847, 6.540332679663050541, -1.199719254218453823 ) ) ;
#146719=CARTESIAN_POINT ( 'NONE',  ( -5.885648082108231982, 7.959951743916638733, 1.443375672974058777 ) ) ;
#146720=CARTESIAN_POINT ( 'NONE',  ( -5.099275172071237705, 8.963255110809500437, 0.000000000000000000 ) ) ;
#146721=CARTESIAN_POINT ( 'NONE',  ( 5.851225812749518695, 8.984124660586543243, -1.199719254218452047 ) ) ;
#146722=CARTESIAN_POINT ( 'NONE',  ( -5.745623237141265882, 9.925253886631958622, 0.7998128361456291469 ) ) ;
#146760=CARTESIAN_POINT ( 'NONE',  ( 5.819104682239041537, 7.212836251160942957, -1.171789181936284896 ) ) ;
#146776=CARTESIAN_POINT ( 'NONE',  ( 7.038618024149998043, 8.240751112043669835, -1.199719254218452047 ) ) ;
#146779=CARTESIAN_POINT ( 'NONE',  ( -4.281342646865346602, 8.216926531310035031, 0.7998128361456352531 ) ) ;
#146793=CARTESIAN_POINT ( 'NONE',  ( 3.888156192069020634, 7.758209000714329839, 1.040834085586084257E-14 ) ) ;
#146795=CARTESIAN_POINT ( 'NONE',  ( 5.830888582329017744, 8.960397891762626799, -1.199719254218452047 ) ) ;
#146803=CARTESIAN_POINT ( 'NONE',  ( 3.074666975249065626, 6.809138247757705820, 0.000000000000000000 ) ) ;
#146808=CARTESIAN_POINT ( 'NONE',  ( 5.631432701629774051, 7.663367133358481631, 1.599625672291269396 ) ) ;
#146817=CARTESIAN_POINT ( 'NONE',  ( 4.858757509019037357, 5.629766575900002401, 2.420000000000000373 ) ) ;
#146820=CARTESIAN_POINT ( 'NONE',  ( -4.828112100242283766, 7.686528979374367410, -1.082531754730549967 ) ) ;
#146821=CARTESIAN_POINT ( 'NONE',  ( 5.234856708652233515, 6.240325927249993576, 1.082531754730549078 ) ) ;
#146831=CARTESIAN_POINT ( 'NONE',  ( -3.526002468005825286, 6.271364091718859335, -1.199719254218450271 ) ) ;
#146832=CARTESIAN_POINT ( 'NONE',  ( -5.966997003790221576, 9.015228033513643879, -1.082531754730549967 ) ) ;
#146833=CARTESIAN_POINT ( 'NONE',  ( 8.174640274396848483, 8.501778173076651512, 0.7998128361456291469 ) ) ;
#146836=CARTESIAN_POINT ( 'NONE',  ( 4.217995187182920880, 6.974725914138481642, 1.082531754730549078 ) ) ;
#146851=CARTESIAN_POINT ( 'NONE',  ( -5.829766698406889880, 6.654474238104274519, 0.9546379765748146395 ) ) ;
#146854=CARTESIAN_POINT ( 'NONE',  ( 4.037295881819344956, 7.932205305423046582, -0.7998128361456362523 ) ) ;
#146856=CARTESIAN_POINT ( 'NONE',  ( -4.248501033035892327, 6.049946853332221153, -1.599625672291271394 ) ) ;
#146857=TOROIDAL_SURFACE ( 'NONE', #98434, 3.970406073902761790, 0.08000000000000000167 ) ;
#146869=CARTESIAN_POINT ( 'NONE',  ( 6.861835142292143530, 8.138467433163244280, 1.082531754730549967 ) ) ;
#146871=CARTESIAN_POINT ( 'NONE',  ( -7.144220599758281054, 7.299621885998258897, 0.7998128361456341429 ) ) ;
#146872=CARTESIAN_POINT ( 'NONE',  ( 4.854701522145073334, 7.821512988214679218, -1.199719254218450271 ) ) ;
#146876=AXIS2_PLACEMENT_3D ( 'NONE', #32889, #116329, #182319 ) ;
#146882=CARTESIAN_POINT ( 'NONE',  ( -6.961185525973791144, 7.086080966583015339, 0.7998128361456341429 ) ) ;
#146903=ADVANCED_FACE ( 'NONE', ( #123579 ), #153858, .F. ) ;
#146908=CARTESIAN_POINT ( 'NONE',  ( 6.048345925472191631, 6.229027465905275562, 0.7216878364870328300 ) ) ;
#146909=AXIS2_PLACEMENT_3D ( 'NONE', #81131, #18242, #1979 ) ;
#146915=CARTESIAN_POINT ( 'NONE',  ( 4.706088717274896638, 7.544168365912456764, 1.082531754730548412 ) ) ;
#146928=CARTESIAN_POINT ( 'NONE',  ( -6.629010762438975135, 6.698543742459062145, -0.7998128361456362523 ) ) ;
#146930=CARTESIAN_POINT ( 'NONE',  ( -7.584860592202423035, 7.813701877183096833, -0.7998128361456362523 ) ) ;
#146938=CARTESIAN_POINT ( 'NONE',  ( 4.543390873910913896, 5.433615786718446472, 1.082531754730549078 ) ) ;
#146943=CARTESIAN_POINT ( 'NONE',  ( -6.099189001301292379, 8.209082816308541197, 1.599625672291263179 ) ) ;
#146949=CARTESIAN_POINT ( 'NONE',  ( -4.340018570150306232, 8.077455741901736985, -0.7216878364870338292 ) ) ;
#146952=CARTESIAN_POINT ( 'NONE',  ( -6.798487682609798632, 6.896266815991691779, 0.7998128361456341429 ) ) ;
#146972=CARTESIAN_POINT ( 'NONE',  ( -6.933015448541747006, 9.181880338089085214, 1.599625672291269396 ) ) ;
#146973=CARTESIAN_POINT ( 'NONE',  ( 4.869313445963426190, 5.709895770826003414, 1.199719254218452935 ) ) ;
#146974=CARTESIAN_POINT ( 'NONE',  ( -6.629010762438975135, 6.698543742459062145, -0.7998128361456362523 ) ) ;
#146989=B_SPLINE_CURVE_WITH_KNOTS ( 'NONE', 3,
 ( #27983, #94079, #93011, #11719 ),
 .UNSPECIFIED., .F., .F.,
 ( 4, 4 ),
 ( 2.776912483567743746E-18, 0.0001591530304775611341 ),
 .UNSPECIFIED. ) ;
#146990=CARTESIAN_POINT ( 'NONE',  ( -5.517647459709249524, 5.988123715949840609, -0.9547278355747212952 ) ) ;
#146992=ORIENTED_EDGE ( 'NONE', *, *, #77330, .T. ) ;
#146999=CARTESIAN_POINT ( 'NONE',  ( -5.772739544368596043, 9.956889578397179363, -0.7998128361456362523 ) ) ;
#147023=CARTESIAN_POINT ( 'NONE',  ( 5.657495238652423097, 9.822437888394988548, 0.000000000000000000 ) ) ;
#147036=CARTESIAN_POINT ( 'NONE',  ( 4.743613802917549194, 8.193193991156523026, -0.7244234545457691743 ) ) ;
#147038=CARTESIAN_POINT ( 'NONE',  ( 3.553118775233146120, 6.302999783484076524, -1.199719254218453823 ) ) ;
#147043=CARTESIAN_POINT ( 'NONE',  ( -6.557303570864871034, 7.679217583210999010, -1.199719254218452047 ) ) ;
#147045=ORIENTED_EDGE ( 'NONE', *, *, #88712, .T. ) ;
#147050=CARTESIAN_POINT ( 'NONE',  ( -5.912764388891193157, 9.912325863766124456, 0.000000000000000000 ) ) ;
#147059=CARTESIAN_POINT ( 'NONE',  ( -4.339491684825780737, 7.220434844675483355, -1.199719254218455378 ) ) ;
#147069=CARTESIAN_POINT ( 'NONE',  ( 5.259637247458703868, 5.100941308315409373, 0.000000000000000000 ) ) ;
#147088=CARTESIAN_POINT ( 'NONE',  ( -5.738844160334429567, 9.917344963690652548, 0.000000000000000000 ) ) ;
#147093=AXIS2_PLACEMENT_3D ( 'NONE', #166917, #99779, #81394 ) ;
#147099=CARTESIAN_POINT ( 'NONE',  ( 6.540882763950133238, 6.595727744222092959, 0.000000000000000000 ) ) ;
#147102=CARTESIAN_POINT ( 'NONE',  ( -5.554920708491585479, 5.909662090865936079, -0.8338897427195167689 ) ) ;
#147109=CARTESIAN_POINT ( 'NONE',  ( 6.699137298928153683, 7.948653282571920720, 1.082531754730549967 ) ) ;
#147120=CARTESIAN_POINT ( 'NONE',  ( -6.211043768836215229, 8.339580045099285854, 1.443375672974064550 ) ) ;
#147140=EDGE_CURVE ( 'NONE', #198442, #52032, #132014, .T. ) ;
#147154=CARTESIAN_POINT ( 'NONE',  ( 5.499767588998890844, 6.445425604367387429, 1.199719254218451159 ) ) ;
#147156=CARTESIAN_POINT ( 'NONE',  ( 4.603875680292229156, 7.528882839386387360, 1.199719254218452047 ) ) ;
#147168=CARTESIAN_POINT ( 'NONE',  ( -5.157951095356222204, 4.982307464195829816, 0.000000000000000000 ) ) ;
#147171=CARTESIAN_POINT ( 'NONE',  ( 4.217995187182920880, 6.974725914138481642, 1.082531754730549078 ) ) ;
#147185=CARTESIAN_POINT ( 'NONE',  ( -6.807602527837528505, 7.114826835331461652, 0.7216878364870317197 ) ) ;
#147187=CARTESIAN_POINT ( 'NONE',  ( -3.824808732831001201, 7.476377598362539345, 0.7216878364870338292 ) ) ;
#147188=CARTESIAN_POINT ( 'NONE',  ( 4.221170328939424010, 7.164078207821040323, 1.167600677116547470 ) ) ;
#147194=CARTESIAN_POINT ( 'NONE',  ( -6.274419661981678331, 6.542771797459788097, -0.3271847599185794819 ) ) ;
#147197=CARTESIAN_POINT ( 'NONE',  ( 3.811250579217332568, 5.539821323877241355, 1.214306433183764966E-14 ) ) ;
#147202=CARTESIAN_POINT ( 'NONE',  ( -3.984117037569407938, 5.741498858621315371, 1.599625672291270506 ) ) ;
#147214=CARTESIAN_POINT ( 'NONE',  ( -5.276058054373441664, 6.184431147304315424, -1.199719254218453823 ) ) ;
#147223=DIRECTION ( 'NONE',  ( 0.000000000000000000, 1.000000000000000000, 0.000000000000000000 ) ) ;
#147224=CARTESIAN_POINT ( 'NONE',  ( -7.747558435566414659, 8.003516027774422170, -0.7998128361456362523 ) ) ;
#147225=CARTESIAN_POINT ( 'NONE',  ( -5.621078624820424530, 7.474595091574217420, 1.344519841555512629 ) ) ;
#147228=ORIENTED_EDGE ( 'NONE', *, *, #115159, .F. ) ;
#147243=CARTESIAN_POINT ( 'NONE',  ( 7.212011367826596242, 7.378711115411311638, 0.000000000000000000 ) ) ;
#147263=CARTESIAN_POINT ( 'NONE',  ( 7.178115983792402233, 7.339166500704784823, 0.7998128361456281477 ) ) ;
#147264=CARTESIAN_POINT ( 'NONE',  ( 5.408776937209000657, 5.274937613024121674, 0.7998128361456352531 ) ) ;
#147266=CARTESIAN_POINT ( 'NONE',  ( 2.878073747850912412, 6.579779482459851003, -0.7998128361456362523 ) ) ;
#147269=CARTESIAN_POINT ( 'NONE',  ( -4.895902867866254837, 7.765618208269001066, 1.082531754730549967 ) ) ;
#147278=CARTESIAN_POINT ( 'NONE',  ( 4.607021725950278146, 8.475092030744066918, 0.2235605714990263060 ) ) ;
#147279=CARTESIAN_POINT ( 'NONE',  ( -6.116136693096208887, 6.308116694799912771, 0.7216878364870257245 ) ) ;
#147280=CARTESIAN_POINT ( 'NONE',  ( 3.607878275012302627, 7.223292064240769861, 0.7216878364870257245 ) ) ;
#147308=CARTESIAN_POINT ( 'NONE',  ( 5.367048706163317640, 7.354919138647580290, -1.599625672291281386 ) ) ;
#147310=CARTESIAN_POINT ( 'NONE',  ( 5.273195401072370281, 5.116759154198018855, -0.7998128361456481317 ) ) ;
#147328=CARTESIAN_POINT ( 'NONE',  ( -7.282664789195997912, 8.525472337930658284, 1.199719254218452047 ) ) ;
#147336=DIRECTION ( 'NONE',  ( -1.000000000000000000, 0.000000000000000000, 0.000000000000000000 ) ) ;
#147337=CARTESIAN_POINT ( 'NONE',  ( 4.681308178468477799, 8.683552984847038303, 0.000000000000000000 ) ) ;
#147342=CARTESIAN_POINT ( 'NONE',  ( 6.710359684120930091, 6.793450817754725257, 0.7998128361456352531 ) ) ;
#147353=CARTESIAN_POINT ( 'NONE',  ( 4.594471896879979589, 8.374412622790375238, -0.01639726577711345112 ) ) ;
#147361=DIRECTION ( 'NONE',  ( 0.000000000000000000, 0.000000000000000000, 1.000000000000000000 ) ) ;
#147369=CARTESIAN_POINT ( 'NONE',  ( -3.895996091634230218, 7.334980739573080832, 0.5863762202383783206 ) ) ;
#147377=CARTESIAN_POINT ( 'NONE',  ( -5.094831863685302942, 9.165997284266655498, 0.7998128361456291469 ) ) ;
#147379=CARTESIAN_POINT ( 'NONE',  ( 4.712340909201580885, 7.655425606447271214, -1.199719254218452047 ) ) ;
#147383=CARTESIAN_POINT ( 'NONE',  ( -5.250750630242457362, 9.347902511916677426, 0.000000000000000000 ) ) ;
#147389=CARTESIAN_POINT ( 'NONE',  ( -0.2384352647906655132, 3.429829024941791094, -1.989178028829215350 ) ) ;
#147398=B_SPLINE_CURVE_WITH_KNOTS ( 'NONE', 3,
 ( #67207, #84552, #150641, #3275, #68278, #200415 ),
 .UNSPECIFIED., .F., .F.,
 ( 4, 2, 4 ),
 ( 0.0006551727224218147332, 0.001090474818249038101, 0.001525776914076261252 ),
 .UNSPECIFIED. ) ;
#147406=CARTESIAN_POINT ( 'NONE',  ( 5.221298555038576872, 9.105615724271411082, 0.000000000000000000 ) ) ;
#147415=CARTESIAN_POINT ( 'NONE',  ( -3.096514578442687515, 6.188910745953249304, -0.7944190528704382359 ) ) ;
#147422=CARTESIAN_POINT ( 'NONE',  ( -5.804299160426249493, 5.944306240018289778, -0.7216878364870338292 ) ) ;
#147425=CARTESIAN_POINT ( 'NONE',  ( 6.387826650694035990, 7.481494509678370264, -1.199719254218452047 ) ) ;
#147448=CARTESIAN_POINT ( 'NONE',  ( 5.575758015699216585, 5.849789923344298259, -0.7899890411014517388 ) ) ;
#147477=CARTESIAN_POINT ( 'NONE',  ( 5.065906673361608270, 5.939254536123854677, -1.199719254218450271 ) ) ;
#147480=ORIENTED_EDGE ( 'NONE', *, *, #88206, .F. ) ;
#147481=CARTESIAN_POINT ( 'NONE',  ( -3.797692425159308716, 7.444741906078900406, 0.000000000000000000 ) ) ;
#147487=CARTESIAN_POINT ( 'NONE',  ( -4.288121723672178476, 8.224835454251337552, -0.7998128361456362523 ) ) ;
#147495=CARTESIAN_POINT ( 'NONE',  ( -5.712781623311813384, 7.758274208654143855, -1.599625672291271394 ) ) ;
#147497=CARTESIAN_POINT ( 'NONE',  ( 5.901825473515108555, 7.257632781371366804, 1.250113620240392631 ) ) ;
#147502=CARTESIAN_POINT ( 'NONE',  ( 5.773793314573267388, 7.829454515125894964, 1.599625672291268286 ) ) ;
#147507=ORIENTED_EDGE ( 'NONE', *, *, #381, .F. ) ;
#147510=CARTESIAN_POINT ( 'NONE',  ( 0.000000000000000000, 8.999999999999998224, 0.000000000000000000 ) ) ;
#147511=CARTESIAN_POINT ( 'NONE',  ( -4.899292406491858820, 6.809203455697518947, -1.599625672291271394 ) ) ;
#147515=CARTESIAN_POINT ( 'NONE',  ( -5.261446130555064826, 8.296048364692991228, 1.199719254218452935 ) ) ;
#147518=CARTESIAN_POINT ( 'NONE',  ( -3.707465945607718805, 7.355851012256872323, 0.5743249234583160945 ) ) ;
#147519=CARTESIAN_POINT ( 'NONE',  ( 5.180624093753221970, 9.058162186105164437, 0.000000000000000000 ) ) ;
#147527=CARTESIAN_POINT ( 'NONE',  ( 6.540882763950133238, 6.595727744222092959, 0.000000000000000000 ) ) ;
#147535=EDGE_CURVE ( 'NONE', #29314, #23394, #165496, .T. ) ;
#147563=CARTESIAN_POINT ( 'NONE',  ( 6.373214726875630731, 9.593111727067046957, 1.199719254218452047 ) ) ;
#147568=CARTESIAN_POINT ( 'NONE',  ( -5.178050853460543834, 7.761234873892349562, -1.181743852105126669 ) ) ;
#147588=CARTESIAN_POINT ( 'NONE',  ( -3.817502770699643388, 6.611447778194983194, 1.199719254218452935 ) ) ;
#147590=CARTESIAN_POINT ( 'NONE',  ( 8.039058738260216330, 8.343599714250547805, -0.7998128361456341429 ) ) ;
#147599=CARTESIAN_POINT ( 'NONE',  ( 5.890091390494168522, 5.836471141856793388, 0.000000000000000000 ) ) ;
#147602=CARTESIAN_POINT ( 'NONE',  ( 7.160114521348466710, 7.526090827760914870, 0.000000000000000000 ) ) ;
#147618=CARTESIAN_POINT ( 'NONE',  ( -3.935609729716867289, 7.813571461303467913, 0.7998128361456352531 ) ) ;
#147619=CARTESIAN_POINT ( 'NONE',  ( 5.415556014015861841, 5.282846535965431300, -0.7998128361456481317 ) ) ;
#147629=CARTESIAN_POINT ( 'NONE',  ( -6.237633190739009237, 9.434933268240943249, 1.199719254218452047 ) ) ;
#147630=CARTESIAN_POINT ( 'NONE',  ( 7.530627977747744062, 7.750430493652658015, -0.7998128361456341429 ) ) ;
#147636=CARTESIAN_POINT ( 'NONE',  ( 3.393283585170187688, 7.180857625999046867, 0.7998128361456271485 ) ) ;
#147643=CARTESIAN_POINT ( 'NONE',  ( -6.546709703855362328, 6.802806841334552601, 0.4695730141109008549 ) ) ;
#147654=CARTESIAN_POINT ( 'NONE',  ( -3.485854892044998543, 6.120562236477518070, -1.082531754730546636 ) ) ;
#147655=CARTESIAN_POINT ( 'NONE',  ( -3.919715807682309094, 6.626733304721049933, 1.082531754730549967 ) ) ;
#147664=CARTESIAN_POINT ( 'NONE',  ( -4.688878646772413283, 4.892074522590037056, 0.6607662533205791444 ) ) ;
#147702=CARTESIAN_POINT ( 'NONE',  ( 3.553118775233146120, 6.302999783484076524, -1.199719254218453823 ) ) ;
#147703=CARTESIAN_POINT ( 'NONE',  ( -3.350273356352693188, 6.922752992471175482, 0.000000000000000000 ) ) ;
#147730=TOROIDAL_SURFACE ( 'NONE', #37155, 0.8300000000000010703, 0.08000000000000000167 ) ;
#147734=CARTESIAN_POINT ( 'NONE',  ( -6.479871072688648148, 6.524547437750345402, 0.000000000000000000 ) ) ;
#147736=CARTESIAN_POINT ( 'NONE',  ( 6.007671464186823407, 9.062681570643055906, 1.082531754730549967 ) ) ;
#147741=CARTESIAN_POINT ( 'NONE',  ( -5.661411662158206681, 8.762674818229999829, -1.199719254218452047 ) ) ;
#147749=CARTESIAN_POINT ( 'NONE',  ( -6.771371375382467583, 6.864631124226471037, -0.7998128361456362523 ) ) ;
#147761=CARTESIAN_POINT ( 'NONE',  ( -4.502189528189771472, 7.410248995266807803, -1.199719254218453823 ) ) ;
#147765=CARTESIAN_POINT ( 'NONE',  ( -6.861835142292179057, 9.098836647464588978, 1.443375672974064550 ) ) ;
#147767=CARTESIAN_POINT ( 'NONE',  ( -5.573810548549546162, 9.516879716700865188, 0.7216878364870267237 ) ) ;
#147768=CARTESIAN_POINT ( 'NONE',  ( 5.352436782344940802, 9.466536356036257871, 0.000000000000000000 ) ) ;
#147769=CARTESIAN_POINT ( 'NONE',  ( -4.624739795592948788, 5.528522862014106920, -1.082531754730549967 ) ) ;
#147784=CARTESIAN_POINT ( 'NONE',  ( 0.2829853868402352757, 2.699735994070968204, 1.982489694896476973 ) ) ;
#147789=CARTESIAN_POINT ( 'NONE',  ( 6.489313741793890422, 6.842916442627623219, -0.5960428994750706089 ) ) ;
#147795=CARTESIAN_POINT ( 'NONE',  ( 5.737007114546517350, 7.374902727567925531, -1.359833108435629656 ) ) ;
#147809=CARTESIAN_POINT ( 'NONE',  ( 6.330867959801246059, 6.852818249511213544, -0.6651261847785728820 ) ) ;
#147823=CARTESIAN_POINT ( 'NONE',  ( 6.068156270568149324, 9.237210194708310951, 1.199719254218452047 ) ) ;
#147826=CARTESIAN_POINT ( 'NONE',  ( -5.224688093219839402, 7.188831756880171397, -1.599625672291271394 ) ) ;
#147840=CARTESIAN_POINT ( 'NONE',  ( 5.598591087800349086, 5.496387455380669529, -0.7998128361456481317 ) ) ;
#147842=CARTESIAN_POINT ( 'NONE',  ( 7.340813827156391191, 7.528980651296110160, 0.7998128361456281477 ) ) ;
#147847=CARTESIAN_POINT ( 'NONE',  ( -6.414416072596845986, 8.576847732820027659, -1.443375672974066548 ) ) ;
#147854=CARTESIAN_POINT ( 'NONE',  ( 8.025500584646550806, 8.327781868367935658, 0.000000000000000000 ) ) ;
#147866=DIRECTION ( 'NONE',  ( -0.3321398189114292965, 0.9432301631592805435, 0.000000000000000000 ) ) ;
#147870=CARTESIAN_POINT ( 'NONE',  ( -5.641601317062247212, 7.675230518029648508, -1.443375672974066548 ) ) ;
#147871=CARTESIAN_POINT ( 'NONE',  ( 5.289089323106923146, 6.303597310780433283, -1.082531754730548412 ) ) ;
#147881=FACE_OUTER_BOUND ( 'NONE', #148833, .T. ) ;
#147882=CARTESIAN_POINT ( 'NONE',  ( -6.129694847154211423, 9.205042184104968328, -1.082531754730549967 ) ) ;
#147887=CARTESIAN_POINT ( 'NONE',  ( 4.217995187182915551, 7.935095128439824563, 0.7216878364870257245 ) ) ;
#147904=CARTESIAN_POINT ( 'NONE',  ( -4.197131071882288289, 7.054347462908075350, -1.199719254218455378 ) ) ;
#147908=AXIS2_PLACEMENT_3D ( 'NONE', #198740, #165201, #16793 ) ;
#147916=CARTESIAN_POINT ( 'NONE',  ( 4.577813143269636065, 5.369812084349879555, -1.199719254218450271 ) ) ;
#147920=CARTESIAN_POINT ( 'NONE',  ( 6.690022453700429139, 6.769724048930809701, 0.7998128361456331437 ) ) ;
#147921=EDGE_LOOP ( 'NONE', ( #29155, #188793, #9084, #172503 ) ) ;
#147928=CARTESIAN_POINT ( 'NONE',  ( -6.771371375382467583, 6.864631124226471037, -0.7998128361456362523 ) ) ;
#147951=VECTOR ( 'NONE', #30353, 1000.000000000000000 ) ;
#147957=CARTESIAN_POINT ( 'NONE',  ( 4.909461021924254709, 5.860697626067345567, 1.082531754730549078 ) ) ;
#147963=CARTESIAN_POINT ( 'NONE',  ( 4.353576723319599218, 8.093273587265928271, -0.7216878364870357165 ) ) ;
#147977=CARTESIAN_POINT ( 'NONE',  ( -5.108390017298964914, 9.181815130149269422, 0.000000000000000000 ) ) ;
#147979=CARTESIAN_POINT ( 'NONE',  ( -6.668631453075260396, 8.873432343378178544, -1.599625672291271394 ) ) ;
#147987=CARTESIAN_POINT ( 'NONE',  ( 7.038618024149998043, 8.240751112043669835, -1.199719254218452047 ) ) ;
#147993=CARTESIAN_POINT ( 'NONE',  ( -6.831329296439251131, 9.063246493969506545, -1.599625672291271394 ) ) ;
#147999=CARTESIAN_POINT ( 'NONE',  ( -4.312902262922974295, 8.045820050136510915, 0.7216878364870338292 ) ) ;
#148002=CARTESIAN_POINT ( 'NONE',  ( -5.315678745009726924, 8.359319748223434487, -1.199719254218453823 ) ) ;
#148017=CARTESIAN_POINT ( 'NONE',  ( -6.544399909239620783, 6.796922107324852469, 0.5836599600529659426 ) ) ;
#148020=CARTESIAN_POINT ( 'NONE',  ( -3.634994582239682526, 6.294558541704648569, 1.082531754730549967 ) ) ;
#148022=CARTESIAN_POINT ( 'NONE',  ( -7.095713291905736853, 9.371694488680407886, 1.599625672291269396 ) ) ;
#148023=CARTESIAN_POINT ( 'NONE',  ( 3.410758162289653672, 6.136912401716668519, -1.199719254218453823 ) ) ;
#148024=CARTESIAN_POINT ( 'NONE',  ( -4.932134020321308654, 8.976183133675331050, 0.7998128361456291469 ) ) ;
#148048=CARTESIAN_POINT ( 'NONE',  ( -7.391130018105325661, 8.652015104991543026, -1.199719254218452047 ) ) ;
#148050=EDGE_CURVE ( 'NONE', #103686, #13123, #161418, .T. ) ;
#148076=CARTESIAN_POINT ( 'NONE',  ( 3.464990776744291345, 6.200183785247111778, 1.199719254218452047 ) ) ;
#148089=CARTESIAN_POINT ( 'NONE',  ( 4.620579464570812256, 8.341333509328540785, -0.3192730525469981151 ) ) ;
#148090=EDGE_CURVE ( 'NONE', #138779, #79641, #116463, .T. ) ;
#148092=CARTESIAN_POINT ( 'NONE',  ( 4.415115299905642665, 5.179997933758551554, -1.199719254218450271 ) ) ;
#148098=ORIENTED_EDGE ( 'NONE', *, *, #152381, .F. ) ;
#148099=CARTESIAN_POINT ( 'NONE',  ( -5.424143973919053785, 8.485862515284315677, 1.199719254218454489 ) ) ;
#148106=CARTESIAN_POINT ( 'NONE',  ( -6.983858524370814003, 9.241197259889665006, 1.443375672974064550 ) ) ;
#148116=CARTESIAN_POINT ( 'NONE',  ( -4.797606254389363833, 6.690569611577942943, 1.599625672291263179 ) ) ;
#148123=B_SPLINE_CURVE_WITH_KNOTS ( 'NONE', 3,
 ( #106365, #55428, #90079, #92226, #172389, #140989, #26114, #57566, #9867, #25050, #187551, #23977, #206998, #156142, #91152, #123723, #58629, #107446, #75943, #39181, #124782, #157207, #190741, #42405, #108512, #174539, #44529, #143123, #195026 ),
 .UNSPECIFIED., .F., .F.,
 ( 4, 2, 2, 2, 2, 2, 2, 2, 2, 2, 2, 1, 2, 2, 4 ),
 ( 0.2067929556721437023, 0.2152132502632845279, 0.2236335448544253535, 0.2320538394455661790, 0.2341589130933515450, 0.2362639867411369388, 0.2404741340367071989, 0.2488944286278472751, 0.2531045759234175074, 0.2573147232189876843, 0.2594197968667729670, 0.2615248705145582497, 0.2636299441623435325, 0.2657350178101288707, 0.2741553124012698905 ),
 .UNSPECIFIED. ) ;
#148126=CARTESIAN_POINT ( 'NONE',  ( -6.486624235763164492, 6.835203243035253173, 0.7121179707554707861 ) ) ;
#148128=CARTESIAN_POINT ( 'NONE',  ( 3.888156192069020634, 7.758209000714329839, 1.040834085586084257E-14 ) ) ;
#148147=ORIENTED_EDGE ( 'NONE', *, *, #181711, .T. ) ;
#148148=AXIS2_PLACEMENT_3D ( 'NONE', #106287, #187474, #71575 ) ;
#148149=CARTESIAN_POINT ( 'NONE',  ( -7.370792787684826486, 8.628288336167626582, -1.199719254218452047 ) ) ;
#148158=CARTESIAN_POINT ( 'NONE',  ( 6.703580607314123085, 6.785541894813420072, 0.000000000000000000 ) ) ;
#148165=CARTESIAN_POINT ( 'NONE',  ( 3.933273961740286317, 7.602920365423422311, 0.7216878364870257245 ) ) ;
#148169=CARTESIAN_POINT ( 'NONE',  ( 7.187230829020130329, 7.557726520044554697, 0.7216878364870267237 ) ) ;
#148180=CARTESIAN_POINT ( 'NONE',  ( -7.105881907338169157, 8.423188659050232729, -1.082531754730549967 ) ) ;
#148205=DIRECTION ( 'NONE',  ( 0.7592566023653003482, 0.6507913734559641616, 0.000000000000000000 ) ) ;
#148211=VERTEX_POINT ( 'NONE', #141661 ) ;
#148215=CARTESIAN_POINT ( 'NONE',  ( 6.066347387471824781, 6.042103138330730872, -0.7998128361456481317 ) ) ;
#148217=CARTESIAN_POINT ( 'NONE',  ( 5.387385936583818591, 7.378645907471495846, -1.599625672291283607 ) ) ;
#148224=LINE ( 'NONE', #115765, #6178 ) ;
#148229=CARTESIAN_POINT ( 'NONE',  ( -5.939880696562884310, 9.943961556049767836, 0.7216878364870267237 ) ) ;
#148233=CARTESIAN_POINT ( 'NONE',  ( 4.326460416092276162, 7.101268681199365496, -1.082531754730548412 ) ) ;
#148239=CARTESIAN_POINT ( 'NONE',  ( -4.390861645979385663, 6.216034235099629157, -1.599625672291271394 ) ) ;
#148245=CARTESIAN_POINT ( 'NONE',  ( -7.322812365156824654, 8.676274193172000437, 1.082531754730549078 ) ) ;
#148247=CARTESIAN_POINT ( 'NONE',  ( -4.773879485787619892, 7.623257595843924150, 1.082531754730549967 ) ) ;
#148265=CARTESIAN_POINT ( 'NONE',  ( -4.228163802615396705, 6.026220084508304708, -1.599625672291271394 ) ) ;
#148276=CARTESIAN_POINT ( 'NONE',  ( -3.793249116773374396, 7.647484079536056356, 0.7998128361456352531 ) ) ;
#148286=CARTESIAN_POINT ( 'NONE',  ( -7.587723245503481095, 8.881373870289390737, 1.199719254218452047 ) ) ;
#148287=CARTESIAN_POINT ( 'NONE',  ( -4.712608863230891565, 8.343829661033030476, -0.7091526064728018719 ) ) ;
#148289=DIRECTION ( 'NONE',  ( 0.000000000000000000, 0.000000000000000000, -1.000000000000000000 ) ) ;
#148305=CARTESIAN_POINT ( 'NONE',  ( 4.525389411911321602, 8.501647757197021704, -0.7998128361456381397 ) ) ;
#148327=CARTESIAN_POINT ( 'NONE',  ( 4.993145711582793744, 9.047363440147082159, -0.7998128361456481317 ) ) ;
#148328=CARTESIAN_POINT ( 'NONE',  ( 4.701645408888975197, 8.707279753670952971, 0.000000000000000000 ) ) ;
#148330=CARTESIAN_POINT ( 'NONE',  ( 5.174371902270911150, 6.065797303184739420, 1.199719254218452047 ) ) ;
#148342=CARTESIAN_POINT ( 'NONE',  ( 5.303225773876714122, 7.631601692149430072, -1.229104931163179426 ) ) ;
#148343=CARTESIAN_POINT ( 'NONE',  ( -4.895902867866254837, 7.765618208269001066, 1.082531754730549967 ) ) ;
#148344=CARTESIAN_POINT ( 'NONE',  ( 4.746763178560261309, 5.670883475476017566, 1.082531754730549078 ) ) ;
#148371=CARTESIAN_POINT ( 'NONE',  ( 3.691562964670865199, 7.528850235416478576, -0.7998128361456362523 ) ) ;
#148380=FACE_OUTER_BOUND ( 'NONE', #43223, .T. ) ;
#148382=CARTESIAN_POINT ( 'NONE',  ( -5.608757509019059562, 5.629766575900002401, 2.420000000000000373 ) ) ;
#148402=FACE_OUTER_BOUND ( 'NONE', #178614, .T. ) ;
#148403=CARTESIAN_POINT ( 'NONE',  ( 6.364626766972446781, 6.390095747748157251, 0.7998128361456352531 ) ) ;
#148407=CARTESIAN_POINT ( 'NONE',  ( -5.850575378433040541, 7.204527765336914413, 1.160475518089182811 ) ) ;
#148408=CARTESIAN_POINT ( 'NONE',  ( 5.712781623311797397, 7.758274208654143855, -1.599625672291283607 ) ) ;
#148418=CARTESIAN_POINT ( 'NONE',  ( 4.624009687016504166, 8.337032093926254106, -0.3390773965592456252 ) ) ;
#148439=CARTESIAN_POINT ( 'NONE',  ( -5.745623237141265882, 9.925253886631958622, 0.7998128361456291469 ) ) ;
#148441=CARTESIAN_POINT ( 'NONE',  ( 5.737035277238070385, 6.722237907313067140, -1.199719254218452047 ) ) ;
#148442=CARTESIAN_POINT ( 'NONE',  ( 0.4800000000000000933, 2.999999999999999112, -2.420000000000000373 ) ) ;
#148444=CARTESIAN_POINT ( 'NONE',  ( -4.340018570150322219, 5.196348098997705556, -1.082531754730551743 ) ) ;
#148453=CARTESIAN_POINT ( 'NONE',  ( -0.4139337043657510540, 2.993729876475310636, -1.957981511387787865 ) ) ;
#148472=CARTESIAN_POINT ( 'NONE',  ( 5.831415467653547680, 8.857049574687536619, -1.082531754730548412 ) ) ;
#148484=CARTESIAN_POINT ( 'NONE',  ( -3.851925040058337579, 6.547644075826416277, -1.082531754730546636 ) ) ;
#148487=CARTESIAN_POINT ( 'NONE',  ( 6.574778147984297938, 6.635272358928617997, -0.7998128361456481317 ) ) ;
#148491=CARTESIAN_POINT ( 'NONE',  ( 3.188928480291387313, 8.980740528189222971, 2.451733079074398969 ) ) ;
#148492=CARTESIAN_POINT ( 'NONE',  ( -3.383641855062333281, 6.105276709951447778, -1.199719254218452047 ) ) ;
#148500=ORIENTED_EDGE ( 'NONE', *, *, #76635, .F. ) ;
#148534=CARTESIAN_POINT ( 'NONE',  ( 4.309512724297349884, 6.121127159803966933, 1.599625672291261402 ) ) ;
#148540=CARTESIAN_POINT ( 'NONE',  ( -4.950135482320914271, 8.789258806100786359, -0.7216878364870338292 ) ) ;
#148547=CARTESIAN_POINT ( 'NONE',  ( -6.448838341955544173, 7.552674816150118708, 1.199719254218452047 ) ) ;
#148549=TOROIDAL_SURFACE ( 'NONE', #141626, 2.080000000000000071, 0.08000000000000000167 ) ;
#148555=FACE_OUTER_BOUND ( 'NONE', #32765, .T. ) ;
#148556=CARTESIAN_POINT ( 'NONE',  ( -6.981522756394290319, 7.109807735406931783, 0.7998128361456341429 ) ) ;
#148559=CARTESIAN_POINT ( 'NONE',  ( 5.469253881944042384, 7.602781119232224327, 1.336104631850141944 ) ) ;
#148564=CARTESIAN_POINT ( 'NONE',  ( 7.842465510862060896, 8.114240948952696542, 0.000000000000000000 ) ) ;
#148569=PLANE ( 'NONE',  #23949 ) ;
#148570=CARTESIAN_POINT ( 'NONE',  ( -5.330290668828105538, 6.247702530834755130, 1.199719254218452935 ) ) ;
#148574=CARTESIAN_POINT ( 'NONE',  ( -5.936491157937300756, 8.019268665717216749, 1.599625672291263179 ) ) ;
#148578=CARTESIAN_POINT ( 'NONE',  ( 6.495764994278809823, 7.711385593814346073, 1.082531754730549967 ) ) ;
#148580=CARTESIAN_POINT ( 'NONE',  ( -7.065207446052813367, 8.375735120883982532, -1.082531754730549967 ) ) ;
#148586=CARTESIAN_POINT ( 'NONE',  ( 5.668190738965027897, 8.770583741171307679, -1.199719254218452047 ) ) ;
#148600=CARTESIAN_POINT ( 'NONE',  ( 6.395636025722083673, 6.905704815116233242, -0.7835738547974178125 ) ) ;
#148613=ORIENTED_EDGE ( 'NONE', *, *, #176104, .F. ) ;
#148615=CARTESIAN_POINT ( 'NONE',  ( -5.953438849732211047, 6.118302544208587435, 0.7216878364870287221 ) ) ;
#148626=ADVANCED_FACE ( 'NONE', ( #166386 ), #196814, .T. ) ;
#148630=CARTESIAN_POINT ( 'NONE',  ( -6.171773824192762881, 6.975641918443353795, -0.9092550976456583722 ) ) ;
#148648=CARTESIAN_POINT ( 'NONE',  ( -4.132202957115018727, 8.042930226601317401, 0.000000000000000000 ) ) ;
#148650=CARTESIAN_POINT ( 'NONE',  ( 6.502017186205484300, 9.743381262951846367, -1.199719254218452047 ) ) ;
#148661=CARTESIAN_POINT ( 'NONE',  ( 6.364626766972446781, 6.390095747748157251, 0.7998128361456352531 ) ) ;
#148665=CARTESIAN_POINT ( 'NONE',  ( 5.628043163004202931, 8.619781885929965526, -1.082531754730548412 ) ) ;
#148679=CARTESIAN_POINT ( 'NONE',  ( -4.990283058281743678, 7.979691447040783814, -1.199719254218453823 ) ) ;
#148680=CARTESIAN_POINT ( 'NONE',  ( 4.634908411025333130, 6.500755460986618495, 1.599625672291268286 ) ) ;
#148688=CARTESIAN_POINT ( 'NONE',  ( -5.327428015527048366, 5.180030537728460338, -0.7998128361456362523 ) ) ;
#148689=CARTESIAN_POINT ( 'NONE',  ( 7.018280793729500644, 8.217024343219755167, -1.199719254218452047 ) ) ;
#148691=FACE_OUTER_BOUND ( 'NONE', #184594, .T. ) ;
#148695=CARTESIAN_POINT ( 'NONE',  ( 4.797606254389322089, 6.690569611577942943, 1.599625672291268286 ) ) ;
#148702=CARTESIAN_POINT ( 'NONE',  ( -6.606676129765223671, 6.763588582595081000, -0.1820296311667093936 ) ) ;
#148712=CARTESIAN_POINT ( 'NONE',  ( -2.984203208339354152, 6.495671153122273722, 0.000000000000000000 ) ) ;
#148717=CARTESIAN_POINT ( 'NONE',  ( -1.772846837484827631, 2.502368107626190774, 2.500000000000000444 ) ) ;
#148724=CARTESIAN_POINT ( 'NONE',  ( -3.147653791585948380, 8.919999999999841833, 2.500000000000000444 ) ) ;
#148738=EDGE_CURVE ( 'NONE', #86356, #182295, #140716, .T. ) ;
#148742=CARTESIAN_POINT ( 'NONE',  ( 6.384963997392946844, 6.413822516572072807, 0.7998128361456350310 ) ) ;
#148760=CARTESIAN_POINT ( 'NONE',  ( 0.4461838333975307602, 2.877219473291476426, 1.949594826320503849 ) ) ;
#148761=CARTESIAN_POINT ( 'NONE',  ( 3.718679271898170491, 7.560485927181699317, 0.7998128361456271485 ) ) ;
#148786=CARTESIAN_POINT ( 'NONE',  ( -5.061990249855848667, 6.999017606288844284, -1.599625672291271394 ) ) ;
#148788=CARTESIAN_POINT ( 'NONE',  ( 7.038091138825468107, 8.344099429118761790, -1.082531754730548412 ) ) ;
#148793=CARTESIAN_POINT ( 'NONE',  ( -6.656127069666307072, 6.730179434224282886, 0.7998128361456341429 ) ) ;
#148802=CARTESIAN_POINT ( 'NONE',  ( -5.264308783856126439, 9.363720357799287797, -0.7998128361456362523 ) ) ;
#148809=CARTESIAN_POINT ( 'NONE',  ( 6.533977301828627127, 6.812828965020023553, -0.5176801306737014441 ) ) ;
#148813=CARTESIAN_POINT ( 'NONE',  ( -5.123001941117347080, 7.070197912760590064, 1.599625672291263179 ) ) ;
#148816=CARTESIAN_POINT ( 'NONE',  ( -6.400857919427531684, 9.521399101757175742, 1.082531754730549967 ) ) ;
#148818=CARTESIAN_POINT ( 'NONE',  ( -5.899206235277530297, 9.896508017883515862, 0.7216878364870267237 ) ) ;
#148819=CARTESIAN_POINT ( 'NONE',  ( 6.502017186205484300, 9.743381262951846367, -1.199719254218452047 ) ) ;
#148820=CARTESIAN_POINT ( 'NONE',  ( -8.093291352714894415, 8.406871097780989288, -0.7998128361456362523 ) ) ;
#148833=EDGE_LOOP ( 'NONE', ( #149826, #131740, #33895, #11429 ) ) ;
#148840=CARTESIAN_POINT ( 'NONE',  ( 6.410638904775656677, 6.895589754593423493, 0.7569561588358000304 ) ) ;
#148846=CARTESIAN_POINT ( 'NONE',  ( 5.802484273800978087, 7.324075294900190158, -1.340195914752571271 ) ) ;
#148859=CARTESIAN_POINT ( 'NONE',  ( 5.318333368960210805, 7.618274611128187601, -1.232678415538956518 ) ) ;
#148875=CARTESIAN_POINT ( 'NONE',  ( 7.862802741282558294, 8.137967717776607657, 0.000000000000000000 ) ) ;
#148878=CARTESIAN_POINT ( 'NONE',  ( -4.655245641445871385, 6.524482229810530498, 1.599625672291263179 ) ) ;
#148885=DIRECTION ( 'NONE',  ( -0.6507913734559640506, -0.7592566023653003482, 0.000000000000000000 ) ) ;
#148892=CARTESIAN_POINT ( 'NONE',  ( 3.790386463472274148, 6.579812086429759788, 1.199719254218452047 ) ) ;
#148894=CARTESIAN_POINT ( 'NONE',  ( 5.481239241674765950, 9.616805891921051952, -0.7998128361456481317 ) ) ;
#148900=CARTESIAN_POINT ( 'NONE',  ( -6.251718229232846369, 9.347402796530044355, -1.082531754730549967 ) ) ;
#148906=CARTESIAN_POINT ( 'NONE',  ( 7.700104897918568447, 7.948153567185284096, 0.000000000000000000 ) ) ;
#148920=CARTESIAN_POINT ( 'NONE',  ( -4.990809943606269172, 8.836712344267034780, -0.7216878364870338292 ) ) ;
#148921=CARTESIAN_POINT ( 'NONE',  ( 5.153507786970260796, 7.105788066255672497, -1.443375672974078761 ) ) ;
#148926=ORIENTED_EDGE ( 'NONE', *, *, #161121, .T. ) ;
#148927=LINE ( 'NONE', #153190, #66535 ) ;
#148931=CARTESIAN_POINT ( 'NONE',  ( -5.144392941742557568, 4.966489618313220333, -0.7998128361456362523 ) ) ;
#148932=CARTESIAN_POINT ( 'NONE',  ( -6.292392690518202159, 9.394856334696294553, -1.082531754730549967 ) ) ;
#148937=CARTESIAN_POINT ( 'NONE',  ( 5.356880090730872013, 6.382686539675070492, 1.082531754730549078 ) ) ;
#148956=CARTESIAN_POINT ( 'NONE',  ( -5.330290668828105538, 6.247702530834755130, 1.199719254218452935 ) ) ;
#148966=CARTESIAN_POINT ( 'NONE',  ( 2.891631901464575272, 6.595597328342462262, 0.000000000000000000 ) ) ;
#149002=CARTESIAN_POINT ( 'NONE',  ( 4.963693636378940788, 5.923969009597785274, -1.082531754730548412 ) ) ;
#149007=CARTESIAN_POINT ( 'NONE',  ( 4.657519343637313902, 4.904169560260807970, 0.6806404322877991353 ) ) ;
#149008=CARTESIAN_POINT ( 'NONE',  ( 5.844973620822844218, 5.991759777147701804, 0.7216878364870328300 ) ) ;
#149022=CARTESIAN_POINT ( 'NONE',  ( -7.144220599758281054, 7.299621885998258897, 0.7998128361456341429 ) ) ;
#149030=CARTESIAN_POINT ( 'NONE',  ( 6.016786309414542622, 10.24161080428416426, 0.7998128361456341429 ) ) ;
#149037=CARTESIAN_POINT ( 'NONE',  ( -6.774234028683526532, 7.932303117332766718, 1.199719254218452047 ) ) ;
#149043=CARTESIAN_POINT ( 'NONE',  ( -4.665414256878287702, 8.457084043084382330, -0.7216878364870338292 ) ) ;
#149046=CARTESIAN_POINT ( 'NONE',  ( -6.180537922983287302, 8.303989891604203422, -1.599625672291271394 ) ) ;
#149067=CARTESIAN_POINT ( 'NONE',  ( -4.990809943606294929, 4.995235487061662205, -0.7216878364870338292 ) ) ;
#149069=CARTESIAN_POINT ( 'NONE',  ( -4.217995187182965289, 6.014356699837137832, 1.443375672974065660 ) ) ;
#149070=CARTESIAN_POINT ( 'NONE',  ( 4.061549535745618833, 6.896169004081968090, -1.199719254218452047 ) ) ;
#149071=CARTESIAN_POINT ( 'NONE',  ( -5.119085517611572378, 8.129960982925583224, 1.199719254218452935 ) ) ;
#149094=CARTESIAN_POINT ( 'NONE',  ( -5.908321080505254841, 10.11506803722328129, 0.7998128361456291469 ) ) ;
#149096=CIRCLE ( 'NONE', #45366, 0.7499999999999997780 ) ;
#149115=DIRECTION ( 'NONE',  ( 0.000000000000000000, 1.000000000000000000, 0.000000000000000000 ) ) ;
#149120=EDGE_CURVE ( 'NONE', #26075, #41882, #95551, .T. ) ;
#149123=CARTESIAN_POINT ( 'NONE',  ( 3.790386463472274148, 6.579812086429759788, 1.199719254218452047 ) ) ;
#149125=DIRECTION ( 'NONE',  ( 0.000000000000000000, 0.000000000000000000, -1.000000000000000000 ) ) ;
#149136=CARTESIAN_POINT ( 'NONE',  ( 4.594924845400013780, 8.373833185659544043, 0.04553248676899754321 ) ) ;
#149138=CARTESIAN_POINT ( 'NONE',  ( 3.230585741806197841, 6.991043475407723307, 0.7998128361456271485 ) ) ;
#149145=CARTESIAN_POINT ( 'NONE',  ( -6.099189001301292379, 8.209082816308541197, 1.599625672291263179 ) ) ;
#149147=VERTEX_POINT ( 'NONE', #13764 ) ;
#149153=CARTESIAN_POINT ( 'NONE',  ( -5.518377602441839613, 7.280004618224392487, 1.249996204172974190 ) ) ;
#149159=CARTESIAN_POINT ( 'NONE',  ( 6.048345925472183637, 8.149765894507963182, 1.443375672974065660 ) ) ;
#149163=CARTESIAN_POINT ( 'NONE',  ( -3.447516199624892419, 7.244129009529488350, 0.7998128361456352531 ) ) ;
#149174=CARTESIAN_POINT ( 'NONE',  ( 5.239300017038202917, 5.077214539491492928, 0.000000000000000000 ) ) ;
#149175=CARTESIAN_POINT ( 'NONE',  ( 3.790386463472274148, 6.579812086429759788, 1.199719254218452047 ) ) ;
#149195=CARTESIAN_POINT ( 'NONE',  ( 7.015401035077362124, 6.062865449010541141, -2.437084766375293921 ) ) ;
#149201=CARTESIAN_POINT ( 'NONE',  ( 5.657495238652423097, 9.822437888394988548, 0.000000000000000000 ) ) ;
#149208=CARTESIAN_POINT ( 'NONE',  ( 6.180537922983273091, 8.303989891604203422, -1.599625672291281386 ) ) ;
#149215=CARTESIAN_POINT ( 'NONE',  ( 4.258669648468278446, 7.022179452304728287, 1.082531754730549078 ) ) ;
#149218=CARTESIAN_POINT ( 'NONE',  ( 5.695833931516881776, 9.659240330162777610, -0.7216878364870458196 ) ) ;
#149230=CARTESIAN_POINT ( 'NONE',  ( -6.956742217587851052, 7.288823140040177506, 0.000000000000000000 ) ) ;
#149267=CARTESIAN_POINT ( 'NONE',  ( 5.318541398310776103, 9.426991741329731056, -0.7998128361456481317 ) ) ;
#149269=CARTESIAN_POINT ( 'NONE',  ( 4.875038752565570732, 7.845239757038595663, -1.199719254218452047 ) ) ;
#149281=CARTESIAN_POINT ( 'NONE',  ( -5.469788628470539926, 5.346117919495872783, -0.7998128361456362523 ) ) ;
#149283=CARTESIAN_POINT ( 'NONE',  ( 5.695833931072550094, 5.817763472438987726, 0.000000000000000000 ) ) ;
#149293=CARTESIAN_POINT ( 'NONE',  ( -3.135678666510573365, 6.880318554229450712, 0.000000000000000000 ) ) ;
#149299=CARTESIAN_POINT ( 'NONE',  ( -6.455090533882201775, 8.624301270986276080, -1.443375672974066548 ) ) ;
#149301=CARTESIAN_POINT ( 'NONE',  ( -3.512971199716682591, 7.112567143062499930, 0.000000000000000000 ) ) ;
#149309=DIRECTION ( 'NONE',  ( 0.000000000000000000, 0.000000000000000000, -1.000000000000000000 ) ) ;
#149314=EDGE_CURVE ( 'NONE', #66325, #94850, #44063, .T. ) ;
#149318=CARTESIAN_POINT ( 'NONE',  ( -5.008811405605897882, 4.808311159487113073, 0.7998128361456281477 ) ) ;
#149329=CARTESIAN_POINT ( 'NONE',  ( -2.993318053567081360, 6.714231172462041819, 0.000000000000000000 ) ) ;
#149332=CARTESIAN_POINT ( 'NONE',  ( 4.929342268689171469, 7.989555622611471897, -1.003472558803005565 ) ) ;
#149340=CARTESIAN_POINT ( 'NONE',  ( 4.021723392342543058, 3.853860420242510632, -2.500000000000000444 ) ) ;
#149341=CARTESIAN_POINT ( 'NONE',  ( -5.730308518391983519, 7.387375129167091714, -1.324551712912255486 ) ) ;
#149359=CARTESIAN_POINT ( 'NONE',  ( 5.550083779947807550, 7.568460058062819407, -1.599625672291283607 ) ) ;
#149365=CARTESIAN_POINT ( 'NONE',  ( 2.969872605471105764, 6.605953636083951253, 0.1972538285620730192 ) ) ;
#149382=CARTESIAN_POINT ( 'NONE',  ( 6.017840079619279692, 8.114175741012878973, -1.599625672291281386 ) ) ;
#149383=CARTESIAN_POINT ( 'NONE',  ( 6.059568310664962709, 6.034194215389424798, 0.7998128361456352531 ) ) ;
#149385=CARTESIAN_POINT ( 'NONE',  ( 5.065906673361608270, 5.939254536123854677, -1.199719254218450271 ) ) ;
#149397=CARTESIAN_POINT ( 'NONE',  ( 5.772745519453025054, 7.247817053759448847, -1.191736586928717978 ) ) ;
#149398=CARTESIAN_POINT ( 'NONE',  ( -5.844973620822877969, 7.912498205750389424, 1.443375672974058777 ) ) ;
#149399=CARTESIAN_POINT ( 'NONE',  ( 5.126391479742934187, 6.113783160189109722, -1.082531754730548412 ) ) ;
#149413=ORIENTED_EDGE ( 'NONE', *, *, #176059, .F. ) ;
#149424=CARTESIAN_POINT ( 'NONE',  ( 6.042093733545556233, 7.078139439671806699, -1.199719254218452047 ) ) ;
#149425=CARTESIAN_POINT ( 'NONE',  ( 4.061549535745618833, 6.896169004081968090, -1.199719254218452047 ) ) ;
#149455=CARTESIAN_POINT ( 'NONE',  ( 6.156284269057003655, 9.340026192945279249, -1.199719254218452047 ) ) ;
#149459=CARTESIAN_POINT ( 'NONE',  ( -5.819752210671484960, 7.227523004248635807, 1.175121323085267289 ) ) ;
#149460=CARTESIAN_POINT ( 'NONE',  ( 6.119526231721748033, 8.232809585132461194, 1.599625672291269396 ) ) ;
#149480=DIRECTION ( 'NONE',  ( 0.7592566023653005702, 0.6507913734559639396, 0.000000000000000000 ) ) ;
#149494=CARTESIAN_POINT ( 'NONE',  ( -5.610041701004606196, 9.767075427805856691, -0.7998128361456362523 ) ) ;
#149496=CARTESIAN_POINT ( 'NONE',  ( 7.537407054554579489, 7.758339416593960536, 0.000000000000000000 ) ) ;
#149500=CARTESIAN_POINT ( 'NONE',  ( -6.064239847062411926, 10.29697326487330500, 0.000000000000000000 ) ) ;
#149508=B_SPLINE_CURVE_WITH_KNOTS ( 'NONE', 3,
 ( #119607, #37221, #103295, #169356, #20942, #5751 ),
 .UNSPECIFIED., .F., .F.,
 ( 4, 2, 4 ),
 ( 0.0007479271397814149687, 0.001059363759668584780, 0.001370800379555754591 ),
 .UNSPECIFIED. ) ;
#149510=CARTESIAN_POINT ( 'NONE',  ( -6.285146472706256482, 6.979120928820362835, -0.9578508296879204575 ) ) ;
#149527=CARTESIAN_POINT ( 'NONE',  ( 6.861835142292143530, 8.138467433163244280, 1.082531754730549967 ) ) ;
#149532=CARTESIAN_POINT ( 'NONE',  ( 4.779848517908583894, 4.883929213520019630, -0.7538207499340529028 ) ) ;
#149540=CARTESIAN_POINT ( 'NONE',  ( -3.838366886444665393, 7.492195444245147939, 0.000000000000000000 ) ) ;
#149542=CARTESIAN_POINT ( 'NONE',  ( 7.049313524462606395, 7.188896964819984525, 0.000000000000000000 ) ) ;
#149545=CARTESIAN_POINT ( 'NONE',  ( -7.445362632559989535, 8.715286488521982733, 1.199719254218452047 ) ) ;
#149547=CARTESIAN_POINT ( 'NONE',  ( -3.305155586681401303, 7.078041627762083898, 0.7998128361456352531 ) ) ;
#149563=CARTESIAN_POINT ( 'NONE',  ( 3.799227641567938019, 7.351783938512805427, -0.4255155205789330486 ) ) ;
#149588=CARTESIAN_POINT ( 'NONE',  ( 3.445180431648323882, 6.073108699348104267, 1.082531754730549078 ) ) ;
#149594=CARTESIAN_POINT ( 'NONE',  ( 5.564695703766185275, 5.456842840674144490, 0.000000000000000000 ) ) ;
#149598=CARTESIAN_POINT ( 'NONE',  ( -5.763624699140882157, 7.817591130454727200, -1.443375672974066548 ) ) ;
#149606=CARTESIAN_POINT ( 'NONE',  ( -7.208094944320834863, 8.438474185576302133, -1.199719254218452047 ) ) ;
#149615=CARTESIAN_POINT ( 'NONE',  ( -6.631873415740034083, 7.766215735565355160, 1.199719254218452047 ) ) ;
#149618=CARTESIAN_POINT ( 'NONE',  ( 4.831949485534527966, 8.212610664285437068, 0.9193987405316924599 ) ) ;
#149623=CARTESIAN_POINT ( 'NONE',  ( 8.018721507839716267, 8.319872945426633137, -0.7998128361456341429 ) ) ;
#149629=CARTESIAN_POINT ( 'NONE',  ( -3.969505113751027547, 7.853116076009993840, 1.214306433183764966E-14 ) ) ;
#149635=CARTESIAN_POINT ( 'NONE',  ( -5.088052786878465739, 9.158088361325352977, 0.000000000000000000 ) ) ;
#149637=CARTESIAN_POINT ( 'NONE',  ( 3.903950209304066998, 8.999999999999998224, -0.7749999999999996891 ) ) ;
#149641=CARTESIAN_POINT ( 'NONE',  ( -6.739811759324828344, 8.956476034002674780, -1.443375672974066548 ) ) ;
#149648=CARTESIAN_POINT ( 'NONE',  ( 7.042534447655770080, 7.180988041878682004, -0.7998128361456341429 ) ) ;
#149664=CARTESIAN_POINT ( 'NONE',  ( 5.662876554447811017, 7.443216037249618999, -1.326882488215734845 ) ) ;
#149679=CARTESIAN_POINT ( 'NONE',  ( -4.123088111887291518, 7.824370207261548416, 0.000000000000000000 ) ) ;
#149684=CARTESIAN_POINT ( 'NONE',  ( 3.719872605471109761, 6.605953636083950364, -2.420000000000002149 ) ) ;
#149691=CARTESIAN_POINT ( 'NONE',  ( -5.872679487624441030, 7.188158700483015195, -1.149102218512105145 ) ) ;
#149694=EDGE_CURVE ( 'NONE', #133393, #56668, #121710, .T. ) ;
#149695=VERTEX_POINT ( 'NONE', #209509 ) ;
#149705=EDGE_CURVE ( 'NONE', #23400, #121694, #49116, .T. ) ;
#149711=CARTESIAN_POINT ( 'NONE',  ( -4.736594563127865420, 6.619389305106191834, -1.599625672291271394 ) ) ;
#149726=CARTESIAN_POINT ( 'NONE',  ( 7.354371980770088690, 7.544798497178720531, 0.000000000000000000 ) ) ;
#149729=CARTESIAN_POINT ( 'NONE',  ( 7.038091138825468107, 8.344099429118761790, -1.082531754730548412 ) ) ;
#149746=CARTESIAN_POINT ( 'NONE',  ( -4.586401103172829785, 8.572828063668767484, 0.7998128361456281477 ) ) ;
#149747=CARTESIAN_POINT ( 'NONE',  ( 4.692003678781083487, 7.631698837623355658, -1.199719254218450271 ) ) ;
#149756=CARTESIAN_POINT ( 'NONE',  ( -6.454563648557663846, 9.688018802362710957, -1.199719254218452047 ) ) ;
#149757=CARTESIAN_POINT ( 'NONE',  ( 5.657495238652423097, 9.822437888394988548, 0.000000000000000000 ) ) ;
#149759=CARTESIAN_POINT ( 'NONE',  ( -6.966220764712169000, 6.002124920821316323, -2.500000000000000444 ) ) ;
#149763=LINE ( 'NONE', #1340, #125833 ) ;
#149764=CARTESIAN_POINT ( 'NONE',  ( 4.903208829997618423, 5.749440385532527564, -1.199719254218450271 ) ) ;
#149769=CARTESIAN_POINT ( 'NONE',  ( -1.886825320689270225, 2.480000000000016858, -2.459652456995881753 ) ) ;
#149771=CARTESIAN_POINT ( 'NONE',  ( -5.823544721894389653, 7.314923355733134791, 1.295626528688619272 ) ) ;
#149780=CARTESIAN_POINT ( 'NONE',  ( -5.921879234118920365, 10.13088588310589699, 0.000000000000000000 ) ) ;
#149786=CARTESIAN_POINT ( 'NONE',  ( -2.281615103654124344, 2.664038801896170483, 2.456549816139032227 ) ) ;
#149792=CARTESIAN_POINT ( 'NONE',  ( 0.1054570145121072472, 2.614151819895196738, -2.076146791065091701 ) ) ;
#149804=DIRECTION ( 'NONE',  ( -0.6507913734559640506, -0.7592566023653003482, 0.000000000000000000 ) ) ;
#149814=CARTESIAN_POINT ( 'NONE',  ( 4.098537063712264228, 7.253343185014818673, 1.055677455976588686 ) ) ;
#149826=ORIENTED_EDGE ( 'NONE', *, *, #32673, .F. ) ;
#149838=CARTESIAN_POINT ( 'NONE',  ( 3.881377115262159894, 7.750300077773022878, 0.7998128361456271485 ) ) ;
#149839=CARTESIAN_POINT ( 'NONE',  ( -4.841670253855968831, 4.821239182352949904, 0.000000000000000000 ) ) ;
#149865=CARTESIAN_POINT ( 'NONE',  ( -6.631873415740034083, 7.766215735565355160, 1.199719254218452047 ) ) ;
#149877=AXIS2_PLACEMENT_3D ( 'NONE', #159670, #78414, #25394 ) ;
#149881=CARTESIAN_POINT ( 'NONE',  ( -5.725286006720766707, 9.901527117808042178, 0.7998128361456291469 ) ) ;
#149883=CARTESIAN_POINT ( 'NONE',  ( 5.364607279338250656, 7.693244595681929532, -1.319704323257679057 ) ) ;
#149888=CARTESIAN_POINT ( 'NONE',  ( 5.063044020060520900, 4.871582543017558109, 0.7998128361456352531 ) ) ;
#149892=CARTESIAN_POINT ( 'NONE',  ( -3.962726036944197894, 7.845207153068690431, -0.7998128361456481317 ) ) ;
#149895=CARTESIAN_POINT ( 'NONE',  ( -5.641601317062233001, 9.595968946632336127, -0.7216878364870338292 ) ) ;
#149897=CARTESIAN_POINT ( 'NONE',  ( -8.054952659850432184, 8.570068656013202002, 0.000000000000000000 ) ) ;
#149898=CARTESIAN_POINT ( 'NONE',  ( 3.051993976407674225, 6.574760382535328240, -0.7216878364870338292 ) ) ;
#149899=CARTESIAN_POINT ( 'NONE',  ( -4.841670253411603397, 5.781608396135871075, 1.082531754730549078 ) ) ;
#149918=CARTESIAN_POINT ( 'NONE',  ( 6.546060204425600659, 6.805396270974036987, -0.4351356575816138772 ) ) ;
#149936=CARTESIAN_POINT ( 'NONE',  ( 5.504185490526544378, 7.460110003252303557, -1.249659907641489820 ) ) ;
#149955=CARTESIAN_POINT ( 'NONE',  ( -5.550083779947821760, 7.568460058062819407, -1.599625672291271394 ) ) ;
#149969=CARTESIAN_POINT ( 'NONE',  ( 5.357406976055401948, 6.279338222599979424, 1.199719254218452935 ) ) ;
#149971=CARTESIAN_POINT ( 'NONE',  ( 7.666209513884374438, 7.908608952478760834, 0.7998128361456281477 ) ) ;
#149976=CARTESIAN_POINT ( 'NONE',  ( -5.763624699140868834, 9.738329559057408602, -0.7216878364870338292 ) ) ;
#149981=CARTESIAN_POINT ( 'NONE',  ( 7.713663051532233972, 7.963971413067895355, -0.7998128361456341429 ) ) ;
#149986=CARTESIAN_POINT ( 'NONE',  ( 1.930226670627029684, 8.999999999999998224, 0.7750000000000004663 ) ) ;
#149994=CARTESIAN_POINT ( 'NONE',  ( -4.977251789992602760, 8.820894498384422633, 0.000000000000000000 ) ) ;
#149995=CARTESIAN_POINT ( 'NONE',  ( 4.746763178560254204, 6.631252689777363152, 1.443375672974065660 ) ) ;
#150006=CARTESIAN_POINT ( 'NONE',  ( -3.797165540279144214, 6.587721009371067638, 1.199719254218452935 ) ) ;
#150007=CARTESIAN_POINT ( 'NONE',  ( -5.777182853198894463, 9.754147405458438058, 0.7216878364870267237 ) ) ;
#150008=CARTESIAN_POINT ( 'NONE',  ( 1.838377265450863440, 2.505607861886320897, -2.496072963307877313 ) ) ;
#150011=CARTESIAN_POINT ( 'NONE',  ( 4.055297343818923039, 7.745280977848496562, 0.7216878364870257245 ) ) ;
#150022=CARTESIAN_POINT ( 'NONE',  ( -6.197060558222979409, 6.958367536249086882, 0.8797177744420351386 ) ) ;
#150028=CARTESIAN_POINT ( 'NONE',  ( 4.095971805104288599, 5.871996087412059140, 1.443375672974058777 ) ) ;
#150031=CARTESIAN_POINT ( 'NONE',  ( -4.847922445338252118, 7.813604065273374921, -1.199719254218453823 ) ) ;
#150043=CARTESIAN_POINT ( 'NONE',  ( 5.388439706788500594, 5.251210844200210559, 0.7998128361456352531 ) ) ;
#150081=CIRCLE ( 'NONE', #46345, 4.583333333333340143 ) ;
#150082=CARTESIAN_POINT ( 'NONE',  ( 5.722950238744209273, 6.809768379023969587, 1.082531754730549967 ) ) ;
#150088=CARTESIAN_POINT ( 'NONE',  ( 5.167065940139554669, 9.042344340222555843, -0.7216878364870458196 ) ) ;
#150103=CARTESIAN_POINT ( 'NONE',  ( -6.071018923869249129, 10.30488218781460574, 0.7998128361456291469 ) ) ;
#150105=CARTESIAN_POINT ( 'NONE',  ( -7.587723245503481095, 8.881373870289390737, 1.199719254218452047 ) ) ;
#150112=CARTESIAN_POINT ( 'NONE',  ( -3.923105346307911745, 5.670318552149568703, -1.599625672291283607 ) ) ;
#150114=CARTESIAN_POINT ( 'NONE',  ( 5.058600711230250013, 5.074324715956299414, -0.7216878364870458196 ) ) ;
#150120=CARTESIAN_POINT ( 'NONE',  ( -6.129167961829681488, 9.308390501180058507, -1.199719254218452047 ) ) ;
#150126=CARTESIAN_POINT ( 'NONE',  ( -4.773879485787619892, 7.623257595843924150, 1.082531754730549967 ) ) ;
#150129=CARTESIAN_POINT ( 'NONE',  ( -5.855142236255304944, 7.924361590421551860, -1.599625672291271394 ) ) ;
#150147=EDGE_CURVE ( 'NONE', #22322, #204026, #186039, .T. ) ;
#150151=CARTESIAN_POINT ( 'NONE',  ( -4.828112100242303306, 4.805421336470338645, -0.7216878364870338292 ) ) ;
#150153=CARTESIAN_POINT ( 'NONE',  ( -5.921879234118920365, 10.13088588310589699, 0.000000000000000000 ) ) ;
#150155=CARTESIAN_POINT ( 'NONE',  ( 4.947799714344386146, 4.737130853015369958, -0.7998128361456481317 ) ) ;
#150156=CARTESIAN_POINT ( 'NONE',  ( -3.332271893908731464, 7.109677319527304640, -0.7998128361456481317 ) ) ;
#150157=CARTESIAN_POINT ( 'NONE',  ( -6.252245114557387851, 7.323316050852266557, -1.199719254218453823 ) ) ;
#150164=VERTEX_POINT ( 'NONE', #175457 ) ;
#150178=DIRECTION ( 'NONE',  ( 0.000000000000000000, 0.000000000000000000, 1.000000000000000000 ) ) ;
#150183=CARTESIAN_POINT ( 'NONE',  ( -5.921879234118920365, 10.13088588310589699, 0.000000000000000000 ) ) ;
#150210=CARTESIAN_POINT ( 'NONE',  ( 4.655245641445829641, 6.524482229810530498, 1.599625672291269396 ) ) ;
#150212=CARTESIAN_POINT ( 'NONE',  ( -3.939566984407580907, 8.987080315575658673, -0.7749999999999979128 ) ) ;
#150225=CARTESIAN_POINT ( 'NONE',  ( 4.637820276784100137, 8.319831082953612622, -0.4078742439591088731 ) ) ;
#150227=CARTESIAN_POINT ( 'NONE',  ( 8.014278199453778839, 8.522615118883788199, 0.000000000000000000 ) ) ;
#150231=CARTESIAN_POINT ( 'NONE',  ( -5.855142236255304944, 7.924361590421551860, -1.599625672291271394 ) ) ;
#150238=CARTESIAN_POINT ( 'NONE',  ( -6.495764994278840021, 8.671754808115688107, 1.443375672974064550 ) ) ;
#150243=B_SPLINE_CURVE_WITH_KNOTS ( 'NONE', 3,
 ( #122018, #154438, #71014, #105715 ),
 .UNSPECIFIED., .F., .F.,
 ( 4, 4 ),
 ( 0.000000000000000000, 1.000000000000000000 ),
 .UNSPECIFIED. ) ;
#150246=CARTESIAN_POINT ( 'NONE',  ( 5.722950238744200391, 7.770137593325314285, 1.443375672974065660 ) ) ;
#150250=CARTESIAN_POINT ( 'NONE',  ( -5.743814354044916470, 6.730146830254374990, -1.199719254218453823 ) ) ;
#150257=EDGE_LOOP ( 'NONE', ( #108385, #209610, #180067, #3390, #141415 ) ) ;
#150262=CARTESIAN_POINT ( 'NONE',  ( 5.337069745634900997, 6.255611453776062980, 1.199719254218452047 ) ) ;
#150263=CARTESIAN_POINT ( 'NONE',  ( 5.923986774528332333, 5.876015756563318426, -0.7998128361456481317 ) ) ;
#150264=VERTEX_POINT ( 'NONE', #180768 ) ;
#150287=CARTESIAN_POINT ( 'NONE',  ( 7.452141709366786770, 8.723195411463290583, 1.199719254218452047 ) ) ;
#150295=CARTESIAN_POINT ( 'NONE',  ( 5.773793314573267388, 7.829454515125894964, 1.599625672291268286 ) ) ;
#150301=CARTESIAN_POINT ( 'NONE',  ( 3.919715808126649659, 7.587102519540811940, 0.000000000000000000 ) ) ;
#150304=CARTESIAN_POINT ( 'NONE',  ( 5.831415467653547680, 8.857049574687536619, -1.082531754730548412 ) ) ;
#150305=EDGE_LOOP ( 'NONE', ( #120378, #111802, #87614 ) ) ;
#150316=CARTESIAN_POINT ( 'NONE',  ( 6.326190869690321961, 6.855918622363850190, 0.6739092513716876676 ) ) ;
#150317=CARTESIAN_POINT ( 'NONE',  ( -5.153507786970262572, 9.026526494858359229, -0.7216878364870338292 ) ) ;
#150332=B_SPLINE_CURVE_WITH_KNOTS ( 'NONE', 3,
 ( #125775, #112706, #59619, #110576, #11928, #210117, #113775, #79061 ),
 .UNSPECIFIED., .F., .F.,
 ( 4, 2, 2, 4 ),
 ( 0.000000000000000000, 0.0002889198933005425896, 0.0005778397866010851792, 0.001155679573202170358 ),
 .UNSPECIFIED. ) ;
#150350=CARTESIAN_POINT ( 'NONE',  ( 7.679767667498067496, 7.924426798361372093, 0.000000000000000000 ) ) ;
#150352=CARTESIAN_POINT ( 'NONE',  ( 6.363572996767764778, 8.517530811019446091, -1.599625672291283607 ) ) ;
#150366=CARTESIAN_POINT ( 'NONE',  ( -4.664887371553763096, 7.600063145858131364, -1.199719254218453823 ) ) ;
#150368=CARTESIAN_POINT ( 'NONE',  ( 6.007671464186834065, 7.141943142040370063, 1.082531754730549967 ) ) ;
#150376=CARTESIAN_POINT ( 'NONE',  ( -3.902768115887413014, 5.646591783325653147, -1.599625672291283607 ) ) ;
#150381=CARTESIAN_POINT ( 'NONE',  ( -7.268579750702160780, 8.613002809641560731, -1.082531754730549967 ) ) ;
#150383=CARTESIAN_POINT ( 'NONE',  ( -4.638297949650955765, 8.425448351319163365, 0.7216878364870267237 ) ) ;
#150409=CARTESIAN_POINT ( 'NONE',  ( -4.142898457427624415, 6.991076079377632091, 1.199719254218452935 ) ) ;
#150410=ADVANCED_FACE ( 'NONE', ( #65921 ), #1990, .F. ) ;
#150421=PLANE ( 'NONE',  #107890 ) ;
#150423=CARTESIAN_POINT ( 'NONE',  ( -5.297016005617503076, 7.750740434075895635, -1.313619143682826396 ) ) ;
#150443=CARTESIAN_POINT ( 'NONE',  ( 5.189738938980948291, 9.276722205444929870, 0.000000000000000000 ) ) ;
#150465=CARTESIAN_POINT ( 'NONE',  ( 6.879836604291781121, 6.991173891287354003, -0.7998128361456341429 ) ) ;
#150466=CARTESIAN_POINT ( 'NONE',  ( 4.376249722160992839, 8.327651452488305850, 0.000000000000000000 ) ) ;
#150468=CARTESIAN_POINT ( 'NONE',  ( 4.193214648376505593, 8.114110533073061404, 0.000000000000000000 ) ) ;
#150472=CARTESIAN_POINT ( 'NONE',  ( -6.135297098026184948, 5.374196335731616259, -2.500000000000000444 ) ) ;
#150481=CARTESIAN_POINT ( 'NONE',  ( 4.868750418105482147, 8.172599172502351905, -0.9747704861028365642 ) ) ;
#150482=CARTESIAN_POINT ( 'NONE',  ( -5.844973620822877969, 7.912498205750389424, 1.443375672974058777 ) ) ;
#150483=CARTESIAN_POINT ( 'NONE',  ( 4.909461021924244051, 6.821066840368686712, 1.443375672974065660 ) ) ;
#150496=ORIENTED_EDGE ( 'NONE', *, *, #189724, .F. ) ;
#150505=CARTESIAN_POINT ( 'NONE',  ( -4.678972410047611774, 5.591794245544547515, 1.082531754730549078 ) ) ;
#150510=CARTESIAN_POINT ( 'NONE',  ( 6.099189001301251523, 8.209082816308541197, 1.599625672291268286 ) ) ;
#150525=CARTESIAN_POINT ( 'NONE',  ( -6.189669738297100210, 5.317594965474102153, -2.438128856460784366 ) ) ;
#150536=CARTESIAN_POINT ( 'NONE',  ( 5.668190738965027897, 8.770583741171307679, -1.199719254218452047 ) ) ;
#150540=CARTESIAN_POINT ( 'NONE',  ( -5.258916259484140099, 7.686978671390940043, 1.214082833407425621 ) ) ;
#150541=CARTESIAN_POINT ( 'NONE',  ( 7.309781096423290769, 8.557108029695882578, 1.199719254218452935 ) ) ;
#150546=EDGE_CURVE ( 'NONE', #113379, #109831, #192601, .T. ) ;
#150569=CARTESIAN_POINT ( 'NONE',  ( 4.421367491832282504, 5.291255174293369556, 1.082531754730549078 ) ) ;
#150573=CARTESIAN_POINT ( 'NONE',  ( -6.095272577795516789, 9.268845886473535245, 1.199719254218452047 ) ) ;
#150575=CARTESIAN_POINT ( 'NONE',  ( 6.821687566331318564, 7.987665577921906568, 1.199719254218452935 ) ) ;
#150596=CARTESIAN_POINT ( 'NONE',  ( 6.668631453075247073, 8.873432343378178544, -1.599625672291281386 ) ) ;
#150601=CARTESIAN_POINT ( 'NONE',  ( 2.276625743944757474, 2.743370740431589017, 2.499999999999998668 ) ) ;
#150607=CARTESIAN_POINT ( 'NONE',  ( 5.533136088152891929, 9.469426179571447832, -0.7216878364870458196 ) ) ;
#150610=ORIENTED_EDGE ( 'NONE', *, *, #36937, .F. ) ;
#150621=CARTESIAN_POINT ( 'NONE',  ( -4.638297949650955765, 8.425448351319163365, 0.7216878364870267237 ) ) ;
#150624=CARTESIAN_POINT ( 'NONE',  ( 4.929271367020211514, 7.908511140569038922, 1.199719254218452047 ) ) ;
#150629=CARTESIAN_POINT ( 'NONE',  ( -5.327428015527048366, 5.180030537728460338, -0.7998128361456362523 ) ) ;
#150631=EDGE_CURVE ( 'NONE', #82918, #80427, #4470, .T. ) ;
#150640=CARTESIAN_POINT ( 'NONE',  ( -7.013428937081412684, 5.939655416065874327, 2.436399677959149468 ) ) ;
#150641=CARTESIAN_POINT ( 'NONE',  ( 3.733245760708456817, 7.355895828392214675, 0.2085371205484687906 ) ) ;
#150655=EDGE_LOOP ( 'NONE', ( #20758, #58750, #112097, #159497 ) ) ;
#150670=CARTESIAN_POINT ( 'NONE',  ( 4.340018570150304456, 6.156717313299049366, -1.443375672974068769 ) ) ;
#150675=CARTESIAN_POINT ( 'NONE',  ( 3.705121118284530279, 7.544668081299086282, -1.734723475976807094E-15 ) ) ;
#150678=CARTESIAN_POINT ( 'NONE',  ( -3.786470039966538970, 7.639575156594750283, 0.000000000000000000 ) ) ;
#150682=CARTESIAN_POINT ( 'NONE',  ( -6.265276382846530545, 6.482112999508623297, 0.000000000000000000 ) ) ;
#150688=CARTESIAN_POINT ( 'NONE',  ( -5.562588163356775972, 9.711712967216715953, 0.7998128361456291469 ) ) ;
#150696=CARTESIAN_POINT ( 'NONE',  ( -7.293360289508603600, 7.473618190706972086, 0.000000000000000000 ) ) ;
#150698=CARTESIAN_POINT ( 'NONE',  ( 5.084740326411086642, 7.951855545768795608, 1.193092838546747414 ) ) ;
#150703=CARTESIAN_POINT ( 'NONE',  ( 7.530627977747744062, 7.750430493652658015, -0.7998128361456341429 ) ) ;
#150710=CARTESIAN_POINT ( 'NONE',  ( -4.197131071882288289, 7.054347462908075350, -1.199719254218455378 ) ) ;
#150716=CARTESIAN_POINT ( 'NONE',  ( -5.478376588373717659, 8.549133898814758936, -1.199719254218452047 ) ) ;
#150722=CARTESIAN_POINT ( 'NONE',  ( -6.495764994278840021, 8.671754808115688107, 1.443375672974064550 ) ) ;
#150728=CARTESIAN_POINT ( 'NONE',  ( 6.475954649182838807, 7.584310507915338562, 1.199719254218452047 ) ) ;
#150742=CARTESIAN_POINT ( 'NONE',  ( 5.269423316188119877, 7.778230059001682406, -1.291559732514224068 ) ) ;
#150763=CARTESIAN_POINT ( 'NONE',  ( 4.421367491832268293, 7.211993602896056288, 1.082531754730549078 ) ) ;
#150771=CARTESIAN_POINT ( 'NONE',  ( -6.483603504774570148, 6.769331023298949646, -0.2299166613418425487 ) ) ;
#150789=CARTESIAN_POINT ( 'NONE',  ( -3.969505113751027547, 7.853116076009993840, 1.214306433183764966E-14 ) ) ;
#150793=CARTESIAN_POINT ( 'NONE',  ( 3.947104627881218963, 8.980740528189222971, -0.7749999999999996891 ) ) ;
#150803=CARTESIAN_POINT ( 'NONE',  ( 5.722423353419669567, 8.833855124701747386, 1.199719254218451159 ) ) ;
#150804=CARTESIAN_POINT ( 'NONE',  ( 2.898410978271408922, 6.603506251283770112, -0.7998128361456362523 ) ) ;
#150806=CARTESIAN_POINT ( 'NONE',  ( 7.010974831598141499, 7.352094523052197239, -0.7216878364870317197 ) ) ;
#150813=CARTESIAN_POINT ( 'NONE',  ( 4.367134877377630175, 7.148722219365612141, -1.082531754730548412 ) ) ;
#150821=CARTESIAN_POINT ( 'NONE',  ( -5.152980901645737077, 8.169505597632108262, -1.199719254218453823 ) ) ;
#150822=CARTESIAN_POINT ( 'NONE',  ( 5.204350862799327793, 7.165104988056252289, -1.599625672291281386 ) ) ;
#150831=CARTESIAN_POINT ( 'NONE',  ( -7.910256278930404505, 8.193330178365746619, -0.7998128361456362523 ) ) ;
#150832=CARTESIAN_POINT ( 'NONE',  ( 6.749980374757213575, 8.968339418673846097, 1.599625672291268286 ) ) ;
#150840=CARTESIAN_POINT ( 'NONE',  ( 4.715203562502613188, 8.723097599553565118, 0.7998128361456341429 ) ) ;
#150845=CARTESIAN_POINT ( 'NONE',  ( -4.758546912290684716, 8.291040531757728260, 0.8107885835855069834 ) ) ;
#150850=CARTESIAN_POINT ( 'NONE',  ( 2.977454500823585093, 6.499579965040511276, -0.5808385047149626779 ) ) ;
#150855=CARTESIAN_POINT ( 'NONE',  ( -6.084577077482911101, 10.32070003369722144, 0.000000000000000000 ) ) ;
#150865=CARTESIAN_POINT ( 'NONE',  ( 3.268924434670684498, 6.827845917175511481, -1.734723475976807094E-15 ) ) ;
#150886=CARTESIAN_POINT ( 'NONE',  ( 4.213551878797002992, 8.137837301896977849, 0.000000000000000000 ) ) ;
#150906=CARTESIAN_POINT ( 'NONE',  ( 0.2344991881673083867, 3.432054146482980794, 1.989640237496114850 ) ) ;
#150908=CARTESIAN_POINT ( 'NONE',  ( 4.044074958626150185, 7.940114228364351767, 0.7998128361456271485 ) ) ;
#150909=CARTESIAN_POINT ( 'NONE',  ( -5.370438244788932280, 6.398504386076097283, 1.082531754730549078 ) ) ;
#150936=CARTESIAN_POINT ( 'NONE',  ( -5.420227550413282636, 9.545625585449309725, 0.7998128361456291469 ) ) ;
#150942=CARTESIAN_POINT ( 'NONE',  ( -5.144392941742557568, 4.966489618313220333, -0.7998128361456362523 ) ) ;
#150948=CARTESIAN_POINT ( 'NONE',  ( -6.074935347375019390, 9.245119117649618801, 1.199719254218452047 ) ) ;
#150955=CARTESIAN_POINT ( 'NONE',  ( 4.927462483923885195, 4.713404084191450849, -0.7998128361456481317 ) ) ;
#150959=CARTESIAN_POINT ( 'NONE',  ( -6.147696309153835692, 6.137010213626392208, 0.7998128361456281477 ) ) ;
#150963=CARTESIAN_POINT ( 'NONE',  ( -7.282137904315833410, 7.668451441222825515, 0.000000000000000000 ) ) ;
#150967=CARTESIAN_POINT ( 'NONE',  ( 4.299344108864946890, 6.109263775132799168, -1.443375672974068769 ) ) ;
#150968=CARTESIAN_POINT ( 'NONE',  ( -6.583366107887490770, 9.838288338247510367, 1.199719254218452935 ) ) ;
#150982=CARTESIAN_POINT ( 'NONE',  ( -0.2036233647782254297, 2.640173713333016536, 2.069169101323902193 ) ) ;
#150987=CARTESIAN_POINT ( 'NONE',  ( 6.463557619869761517, 6.860074278669063830, -0.6545079704341187909 ) ) ;
#151006=CARTESIAN_POINT ( 'NONE',  ( 5.551963943121584144, 7.421064284658021037, -1.246246109899084020 ) ) ;
#151008=AXIS2_PLACEMENT_3D ( 'NONE', #105751, #171778, #136088 ) ;
#151026=CARTESIAN_POINT ( 'NONE',  ( -5.956828388357799042, 8.042995434541133193, 1.599625672291263179 ) ) ;
#151039=CARTESIAN_POINT ( 'NONE',  ( 5.682802662783380754, 6.658966523782627434, 1.199719254218452935 ) ) ;
#151042=CARTESIAN_POINT ( 'NONE',  ( -5.593777659986292505, 7.397990072842402398, -1.241664499109219166 ) ) ;
#151046=AXIS2_PLACEMENT_3D ( 'NONE', #192587, #42120, #45306 ) ;
#151047=CARTESIAN_POINT ( 'NONE',  ( -6.916067756302494374, 7.241369601873926420, 0.000000000000000000 ) ) ;
#151053=CARTESIAN_POINT ( 'NONE',  ( 8.011942431032855083, 8.311964022485323511, 0.7998128361456291469 ) ) ;
#151062=CARTESIAN_POINT ( 'NONE',  ( 1.872340672757953906, 8.979957301293506333, 0.7750000000000004663 ) ) ;
#151063=CARTESIAN_POINT ( 'NONE',  ( 0.000000000000000000, 8.999999999999998224, 0.000000000000000000 ) ) ;
#151069=CARTESIAN_POINT ( 'NONE',  ( -6.956742217587851052, 7.288823140040177506, 0.000000000000000000 ) ) ;
#151070=CARTESIAN_POINT ( 'NONE',  ( 5.560252395380206103, 8.540692657035327429, 1.082531754730547524 ) ) ;
#151079=CARTESIAN_POINT ( 'NONE',  ( -5.795184315198522285, 5.725746220678519904, -0.7998128361456362523 ) ) ;
#151080=CARTESIAN_POINT ( 'NONE',  ( -5.939880696562884310, 9.943961556049767836, 0.7216878364870267237 ) ) ;
#151083=CARTESIAN_POINT ( 'NONE',  ( 6.346625304528514810, 6.577020074804287297, 0.000000000000000000 ) ) ;
#151096=CARTESIAN_POINT ( 'NONE',  ( -4.976059700032323896, 7.958698620104867061, 1.042642055368933285 ) ) ;
#151101=CARTESIAN_POINT ( 'NONE',  ( 3.092668437693027794, 6.622213920701574885, -0.7216878364870338292 ) ) ;
#151104=CARTESIAN_POINT ( 'NONE',  ( -6.466312919074983512, 6.508729591867735031, -0.7998128361456362523 ) ) ;
#151115=CARTESIAN_POINT ( 'NONE',  ( 4.390861645979372341, 6.216034235099629157, -1.599625672291269396 ) ) ;
#151149=CARTESIAN_POINT ( 'NONE',  ( 6.699137298928158124, 6.988284068270579574, 0.7216878364870328300 ) ) ;
#151154=CARTESIAN_POINT ( 'NONE',  ( 4.892487020634524342, 4.880525410245029505, -1.277330582746047388E-09 ) ) ;
#151155=CARTESIAN_POINT ( 'NONE',  ( 5.519577934094851202, 8.493239118869080784, 1.082531754730547524 ) ) ;
#151168=CARTESIAN_POINT ( 'NONE',  ( -6.607619761813764647, 8.802252036906432764, 1.599625672291269396 ) ) ;
#151180=CARTESIAN_POINT ( 'NONE',  ( 4.462041952228939401, 6.299077925724123617, -1.443375672974068769 ) ) ;
#151185=CARTESIAN_POINT ( 'NONE',  ( -6.424584688029276514, 8.588711117491191871, 1.599625672291269396 ) ) ;
#151190=CARTESIAN_POINT ( 'NONE',  ( -5.804299160426242388, 6.904675454319632699, -1.082531754730549967 ) ) ;
#151194=CARTESIAN_POINT ( 'NONE',  ( -4.749098946536820520, 8.762642214260091933, 0.7998128361456281477 ) ) ;
#151215=CARTESIAN_POINT ( 'NONE',  ( -3.201133666602369310, 6.748756687762456963, -0.7216878364870458196 ) ) ;
#151218=CARTESIAN_POINT ( 'NONE',  ( -5.777182852754558340, 5.912670547734647286, 0.000000000000000000 ) ) ;
#151220=CARTESIAN_POINT ( 'NONE',  ( 5.194709132691408549, 6.089524072008651423, 1.199719254218452935 ) ) ;
#151221=CARTESIAN_POINT ( 'NONE',  ( -5.679940009482361774, 5.591294530676332641, 0.7998128361456281477 ) ) ;
#151222=CARTESIAN_POINT ( 'NONE',  ( -4.281342646865346602, 8.216926531310035031, 0.7998128361456352531 ) ) ;
#151234=ORIENTED_EDGE ( 'NONE', *, *, #200488, .F. ) ;
#151265=CARTESIAN_POINT ( 'NONE',  ( 5.526144005543697446, 7.442112546579989996, -1.248357989223557452 ) ) ;
#151272=CARTESIAN_POINT ( 'NONE',  ( 5.194709132691408549, 6.089524072008651423, 1.199719254218452935 ) ) ;
#151287=CARTESIAN_POINT ( 'NONE',  ( 4.612778539632031105, 8.351152097327862123, 0.2683542610703564812 ) ) ;
#151290=CARTESIAN_POINT ( 'NONE',  ( 4.390861645979372341, 6.216034235099629157, -1.599625672291269396 ) ) ;
#151296=CARTESIAN_POINT ( 'NONE',  ( -5.285699784481336927, 7.260012063351913625, 1.599625672291263179 ) ) ;
#151311=CARTESIAN_POINT ( 'NONE',  ( 6.536439455564164724, 7.758839131980592718, 1.082531754730549967 ) ) ;
#151314=CARTESIAN_POINT ( 'NONE',  ( -5.285699784481336927, 7.260012063351913625, 1.599625672291263179 ) ) ;
#151325=CARTESIAN_POINT ( 'NONE',  ( 5.174371902270911150, 6.065797303184739420, 1.199719254218452047 ) ) ;
#151326=CARTESIAN_POINT ( 'NONE',  ( 6.561219994370630637, 6.619454513046008515, 0.000000000000000000 ) ) ;
#151351=CARTESIAN_POINT ( 'NONE',  ( 5.806634928402749196, 9.996434193103704402, -0.7998128361456481317 ) ) ;
#151355=CARTESIAN_POINT ( 'NONE',  ( 3.410758162289653672, 6.136912401716668519, -1.199719254218453823 ) ) ;
#151358=ADVANCED_FACE ( 'NONE', ( #23070 ), #43643, .T. ) ;
#151361=CARTESIAN_POINT ( 'NONE',  ( 5.155843554946782703, 9.237177590738404831, -0.7998128361456481317 ) ) ;
#151366=CARTESIAN_POINT ( 'NONE',  ( 5.072158865288233009, 7.010880990960010273, 1.443375672974065660 ) ) ;
#151369=CARTESIAN_POINT ( 'NONE',  ( 6.482206841109512396, 9.616306177052839743, -1.082531754730548412 ) ) ;
#151381=CARTESIAN_POINT ( 'NONE',  ( 5.954584599377941601, 7.113081392617206511, -1.094866876611422235 ) ) ;
#151382=CARTESIAN_POINT ( 'NONE',  ( -6.373741612200205076, 8.529394195690610303, 1.443375672974064550 ) ) ;
#151411=ORIENTED_EDGE ( 'NONE', *, *, #200741, .F. ) ;
#151415=CARTESIAN_POINT ( 'NONE',  ( 6.017840079619279692, 8.114175741012878973, -1.599625672291281386 ) ) ;
#151417=CARTESIAN_POINT ( 'NONE',  ( 5.189738938980948291, 9.276722205444929870, 0.000000000000000000 ) ) ;
#151430=CARTESIAN_POINT ( 'NONE',  ( -6.147696309153835692, 6.137010213626392208, 0.7998128361456281477 ) ) ;
#151432=CARTESIAN_POINT ( 'NONE',  ( 6.821160681006788629, 8.091013894996997635, 1.082531754730549967 ) ) ;
#151435=EDGE_CURVE ( 'NONE', #150164, #96695, #87447, .T. ) ;
#151442=CARTESIAN_POINT ( 'NONE',  ( -3.363304624641834106, 6.081549941127532222, -1.199719254218452047 ) ) ;
#151449=CARTESIAN_POINT ( 'NONE',  ( -6.373741612200205076, 8.529394195690610303, 1.443375672974064550 ) ) ;
#151451=CARTESIAN_POINT ( 'NONE',  ( -4.651856103264620401, 8.441266197201775512, 0.000000000000000000 ) ) ;
#151475=CARTESIAN_POINT ( 'NONE',  ( -6.154475385960665790, 6.144919136567696505, 0.000000000000000000 ) ) ;
#151487=CARTESIAN_POINT ( 'NONE',  ( -4.941402330188276792, 8.092876352253616901, -1.081280284042404727 ) ) ;
#151495=DIRECTION ( 'NONE',  ( 0.6507913734559641616, -0.7592566023653004592, 0.000000000000000000 ) ) ;
#151503=CARTESIAN_POINT ( 'NONE',  ( 6.062430963966053632, 7.101866208495718702, -1.199719254218452047 ) ) ;
#151512=CARTESIAN_POINT ( 'NONE',  ( 1.853667714121303600, 8.957164077253494838, -0.7749999999999996891 ) ) ;
#151526=CARTESIAN_POINT ( 'NONE',  ( 5.169401708560450004, 9.252995436621013425, 0.000000000000000000 ) ) ;
#151527=CARTESIAN_POINT ( 'NONE',  ( 4.538947565524982686, 8.517465603079630299, 0.000000000000000000 ) ) ;
#151529=CARTESIAN_POINT ( 'NONE',  ( 4.797606254389322089, 6.690569611577942943, 1.599625672291268286 ) ) ;
#151533=CARTESIAN_POINT ( 'NONE',  ( -7.005397802120338469, 5.950282834973755541, -2.500000000000000000 ) ) ;
#151543=CARTESIAN_POINT ( 'NONE',  ( 5.273189713885392926, 7.658326211947664497, -1.220946906274408494 ) ) ;
#151545=CARTESIAN_POINT ( 'NONE',  ( -5.085717018457573957, 8.947437264926888290, 0.7216878364870267237 ) ) ;
#151546=CARTESIAN_POINT ( 'NONE',  ( 4.258669648468281110, 6.061810238003387141, 1.443375672974058777 ) ) ;
#151567=CARTESIAN_POINT ( 'NONE',  ( -5.112833325684928987, 5.137596099486740897, -0.7216878364870338292 ) ) ;
#151572=CARTESIAN_POINT ( 'NONE',  ( 5.885121196783658526, 9.023669275293071834, 1.199719254218452047 ) ) ;
#151593=EDGE_LOOP ( 'NONE', ( #213358, #94490, #177696, #40095 ) ) ;
#151599=CARTESIAN_POINT ( 'NONE',  ( 7.289443866002793371, 8.533381260871966134, 1.199719254218452047 ) ) ;
#151603=CARTESIAN_POINT ( 'NONE',  ( 6.526270840131753737, 8.707344961610770540, -1.599625672291283607 ) ) ;
#151612=AXIS2_PLACEMENT_3D ( 'NONE', #33502, #113765, #99574 ) ;
#151614=CARTESIAN_POINT ( 'NONE',  ( 1.817552723627605671, 2.511586290612293659, 2.499391979724956414 ) ) ;
#151632=CARTESIAN_POINT ( 'NONE',  ( 5.411112705629925301, 5.485588709422586362, 0.000000000000000000 ) ) ;
#151637=CARTESIAN_POINT ( 'NONE',  ( -5.271087860662956537, 9.371629280740593870, 0.000000000000000000 ) ) ;
#151639=CARTESIAN_POINT ( 'NONE',  ( 6.607619761813720238, 8.802252036906432764, 1.599625672291268286 ) ) ;
#151642=CARTESIAN_POINT ( 'NONE',  ( -3.933273961740340496, 5.682181936820735579, 1.443375672974065660 ) ) ;
#151661=CARTESIAN_POINT ( 'NONE',  ( 7.506374323821472849, 8.786466794993730289, -1.199719254218452047 ) ) ;
#151662=FACE_OUTER_BOUND ( 'NONE', #24206, .T. ) ;
#151671=CARTESIAN_POINT ( 'NONE',  ( 7.349928672384120176, 7.747540670635879145, 0.7216878364870267237 ) ) ;
#151674=DIRECTION ( 'NONE',  ( -0.7592566023653016805, -0.6507913734559627184, 0.000000000000000000 ) ) ;
#151683=CARTESIAN_POINT ( 'NONE',  ( -6.183927461608886844, 7.347575139032721303, 1.082531754730548412 ) ) ;
#151686=CARTESIAN_POINT ( 'NONE',  ( 6.068156270568149324, 9.237210194708310951, 1.199719254218452047 ) ) ;
#151692=CARTESIAN_POINT ( 'NONE',  ( -6.050681693448748177, 10.28115541899069463, 0.7998128361456291469 ) ) ;
#151705=DIRECTION ( 'NONE',  ( -0.000000000000000000, 1.000000000000000000, -0.000000000000000000 ) ) ;
#151706=CARTESIAN_POINT ( 'NONE',  ( -5.655159470231558849, 6.730679149092498648, 1.082531754730549078 ) ) ;
#151709=CARTESIAN_POINT ( 'NONE',  ( 3.832672171918658943, 7.347512574185182110, -0.5939728463272093695 ) ) ;
#151733=CARTESIAN_POINT ( 'NONE',  ( 4.502716413514295191, 6.346531463890372926, -1.443375672974068769 ) ) ;
#151740=CARTESIAN_POINT ( 'NONE',  ( -6.134138155540168391, 6.121192367743780949, 0.000000000000000000 ) ) ;
#151741=CARTESIAN_POINT ( 'NONE',  ( -4.359828915246279024, 7.244161613499399799, -1.199719254218455378 ) ) ;
#151744=CARTESIAN_POINT ( 'NONE',  ( -4.760321331729590710, 8.567808963744235839, 0.7216878364870267237 ) ) ;
#151750=CARTESIAN_POINT ( 'NONE',  ( -7.422162748838431412, 7.623887726591770608, -0.7998128361456362523 ) ) ;
#151758=( BOUNDED_CURVE ( )  B_SPLINE_CURVE ( 2, ( #113880, #15213, #33609, #179875, #197174 ),
 .UNSPECIFIED., .F., .T. ) 
 B_SPLINE_CURVE_WITH_KNOTS ( ( 3, 2, 3 ),
 ( 0.2725899390149210122, 0.2750000000000000222, 0.2781713664827957233 ),
 .UNSPECIFIED. ) 
 CURVE ( )  GEOMETRIC_REPRESENTATION_ITEM ( )  RATIONAL_B_SPLINE_CURVE ( ( 0.9449186369899742477, 0.9612535663202994574, 1.000000000000000000, 0.9490140947219055656, 0.9368349873063581690 ) ) 
 REPRESENTATION_ITEM ( '' )  );
#151760=CARTESIAN_POINT ( 'NONE',  ( -6.805266759416629618, 6.904175738932996964, 0.000000000000000000 ) ) ;
#151762=CARTESIAN_POINT ( 'NONE',  ( 4.634937608369048334, 8.440560775401745985, -0.4060563726728562139 ) ) ;
#151767=CARTESIAN_POINT ( 'NONE',  ( 7.856023664475727308, 8.130058794835305136, -0.7998128361456341429 ) ) ;
#151779=CARTESIAN_POINT ( 'NONE',  ( 5.899206235277530297, 7.015400374979486209, -1.082531754730548412 ) ) ;
#151782=CARTESIAN_POINT ( 'NONE',  ( -6.238160075619175515, 10.29195416494877513, 0.000000000000000000 ) ) ;
#151788=CARTESIAN_POINT ( 'NONE',  ( 5.020262018810099924, 9.078999131912302900, 0.7998128361456331437 ) ) ;
#151798=DIRECTION ( 'NONE',  ( 0.000000000000000000, 0.000000000000000000, -1.000000000000000000 ) ) ;
#151803=CARTESIAN_POINT ( 'NONE',  ( 5.461903044330952639, 7.609029316319980474, -1.335476589331906494 ) ) ;
#151825=CARTESIAN_POINT ( 'NONE',  ( 5.397554552016226914, 6.430140077841320689, 1.082531754730549078 ) ) ;
#151832=CARTESIAN_POINT ( 'NONE',  ( -6.472689817967896886, 6.776322833669464529, -0.2902398332882798471 ) ) ;
#151849=CARTESIAN_POINT ( 'NONE',  ( -4.444040490229335560, 8.406740681901359480, 0.7998128361456352531 ) ) ;
#151862=ORIENTED_EDGE ( 'NONE', *, *, #28043, .T. ) ;
#151865=CARTESIAN_POINT ( 'NONE',  ( 6.852720297064418986, 6.959538199522133262, 0.7998128361456331437 ) ) ;
#151868=CARTESIAN_POINT ( 'NONE',  ( 8.136301581532414673, 8.664975731308866003, 0.000000000000000000 ) ) ;
#151877=CARTESIAN_POINT ( 'NONE',  ( 4.380693030546900957, 8.124909279031152565, 0.7216878364870219498 ) ) ;
#151882=CARTESIAN_POINT ( 'NONE',  ( -5.237192476628793614, 9.332084666034067055, 0.7998128361456291469 ) ) ;
#151883=CARTESIAN_POINT ( 'NONE',  ( 6.527324610336440180, 6.579909898339485252, 0.7998128361456331437 ) ) ;
#151891=CARTESIAN_POINT ( 'NONE',  ( -3.142457743317409680, 6.888227477170756785, 0.7998128361456352531 ) ) ;
#151892=CARTESIAN_POINT ( 'NONE',  ( 7.452141709366786770, 8.723195411463290583, 1.199719254218452047 ) ) ;
#151899=CARTESIAN_POINT ( 'NONE',  ( 7.049313524462606395, 7.188896964819984525, 0.000000000000000000 ) ) ;
#151905=CARTESIAN_POINT ( 'NONE',  ( -4.948302019123040019, 8.085739352127342627, 1.088677458455259650 ) ) ;
#151915=CARTESIAN_POINT ( 'NONE',  ( -3.485854892044998543, 6.120562236477518070, -1.082531754730546636 ) ) ;
#151924=CARTESIAN_POINT ( 'NONE',  ( 4.095971805104285934, 6.832365301713403838, 1.082531754730549078 ) ) ;
#151927=CARTESIAN_POINT ( 'NONE',  ( -5.367048706163331850, 7.354919138647580290, -1.599625672291271394 ) ) ;
#151938=CARTESIAN_POINT ( 'NONE',  ( 4.194756697597139983, 7.186718463257284917, 1.144634955760708950 ) ) ;
#151945=CARTESIAN_POINT ( 'NONE',  ( 4.227110032410640095, 8.153655147779589996, 0.7998128361456271485 ) ) ;
#151968=CARTESIAN_POINT ( 'NONE',  ( 6.201928923608456046, 6.200281597156833691, 0.7998128361456352531 ) ) ;
#151969=CARTESIAN_POINT ( 'NONE',  ( -5.045042558060949034, 6.018876084893449274, 1.082531754730549078 ) ) ;
#151991=CARTESIAN_POINT ( 'NONE',  ( -5.610041701004606196, 9.767075427805856691, -0.7998128361456362523 ) ) ;
#152002=ORIENTED_EDGE ( 'NONE', *, *, #159680, .T. ) ;
#152006=CARTESIAN_POINT ( 'NONE',  ( -5.399890319992785237, 9.521898816625391504, 0.7998128361456291469 ) ) ;
#152014=CARTESIAN_POINT ( 'NONE',  ( 5.401997860402196316, 5.267028690082820930, 0.000000000000000000 ) ) ;
#152021=CARTESIAN_POINT ( 'NONE',  ( -6.934069218746458318, 7.054445274817795486, -0.7998128361456362523 ) ) ;
#152024=CARTESIAN_POINT ( 'NONE',  ( -6.699137298928187434, 8.909022496873262753, 1.443375672974064550 ) ) ;
#152027=CARTESIAN_POINT ( 'NONE',  ( -6.685579144870156476, 9.853573864773576219, 1.082531754730549967 ) ) ;
#152028=CARTESIAN_POINT ( 'NONE',  ( 4.380693030546913391, 7.164540064729805202, 1.082531754730549078 ) ) ;
#152029=CARTESIAN_POINT ( 'NONE',  ( -3.648552735408985725, 7.270745601370182776, -0.7216878364870458196 ) ) ;
#152041=CARTESIAN_POINT ( 'NONE',  ( 0.3866926556112013635, 2.897682894409562060, 2.027578619373314073 ) ) ;
#152045=CARTESIAN_POINT ( 'NONE',  ( 1.878856644857516578, 2.480000000000016858, 2.465765312203895387 ) ) ;
#152046=CARTESIAN_POINT ( 'NONE',  ( 6.367678427751853221, 6.924687757192571347, 0.8275186136274095272 ) ) ;
#152047=ORIENTED_EDGE ( 'NONE', *, *, #128773, .F. ) ;
#152066=CARTESIAN_POINT ( 'NONE',  ( 5.931307043615195340, 7.129970210930432373, 1.110187140972586306 ) ) ;
#152079=CARTESIAN_POINT ( 'NONE',  ( 4.889022008684530185, 4.879516615612172536, -0.08706862575298174312 ) ) ;
#152084=CARTESIAN_POINT ( 'NONE',  ( -6.791708605802965870, 6.888357893050385705, -0.7998128361456362523 ) ) ;
#152095=CARTESIAN_POINT ( 'NONE',  ( 4.688087255275310561, 8.691461907788344377, -0.7998128361456381397 ) ) ;
#152103=CARTESIAN_POINT ( 'NONE',  ( -7.119440060507479018, 8.439006504414422238, 1.082531754730549078 ) ) ;
#152108=CARTESIAN_POINT ( 'NONE',  ( 5.851225812749518695, 8.984124660586543243, -1.199719254218452047 ) ) ;
#152123=CARTESIAN_POINT ( 'NONE',  ( -6.292392690518209264, 8.434487120394948079, -1.443375672974066548 ) ) ;
#152124=CARTESIAN_POINT ( 'NONE',  ( 6.427974226654860956, 7.632296364919712417, -1.082531754730548412 ) ) ;
#152126=EDGE_CURVE ( 'NONE', #121694, #78339, #98540, .T. ) ;
#152136=CARTESIAN_POINT ( 'NONE',  ( -4.146814880933400005, 5.931313009212638931, 1.599625672291270506 ) ) ;
#152137=CARTESIAN_POINT ( 'NONE',  ( -3.122120512896910505, 6.864500708346841229, 0.7998128361456352531 ) ) ;
#152139=CARTESIAN_POINT ( 'NONE',  ( 6.997416677984476863, 7.336276677169590421, 0.000000000000000000 ) ) ;
#152147=CARTESIAN_POINT ( 'NONE',  ( -6.004825442174102967, 7.178221627660431814, 1.212153120240029969 ) ) ;
#152150=CARTESIAN_POINT ( 'NONE',  ( -4.712247760717829692, 8.249883430950177399, 0.6303846594760522670 ) ) ;
#152155=CARTESIAN_POINT ( 'NONE',  ( 3.119784744920330422, 6.653849612466795627, 0.7216878364870257245 ) ) ;
#152159=CARTESIAN_POINT ( 'NONE',  ( -4.633854640820660009, 8.628190524257904670, -0.7998128361456362523 ) ) ;
#152171=CARTESIAN_POINT ( 'NONE',  ( 4.041212305325117882, 6.872442235258051646, -1.199719254218448494 ) ) ;
#152198=ORIENTED_EDGE ( 'NONE', *, *, #172187, .T. ) ;
#152207=CARTESIAN_POINT ( 'NONE',  ( 4.231553341240963384, 7.950912974840849579, -0.7216878364870357165 ) ) ;
#152211=CARTESIAN_POINT ( 'NONE',  ( 4.831500990369687720, 4.877271539032528302, 0.3436843597541731632 ) ) ;
#152212=CARTESIAN_POINT ( 'NONE',  ( 6.333067150914820864, 6.561202228921677815, 0.7216878364870328300 ) ) ;
#152226=CARTESIAN_POINT ( 'NONE',  ( -6.257970421159510188, 9.458660037064859694, 1.199719254218452047 ) ) ;
#152228=CARTESIAN_POINT ( 'NONE',  ( -7.075376061485238566, 9.347967719856493218, 1.599625672291269396 ) ) ;
#152237=CARTESIAN_POINT ( 'NONE',  ( 4.706088717274895750, 6.583799151611112954, 1.443375672974065660 ) ) ;
#152243=CARTESIAN_POINT ( 'NONE',  ( -7.584860592202423035, 7.813701877183096833, -0.7998128361456362523 ) ) ;
#152248=CARTESIAN_POINT ( 'NONE',  ( -6.834718835064852449, 8.106831741398025315, 1.082531754730549078 ) ) ;
#152251=CARTESIAN_POINT ( 'NONE',  ( -6.129167961829681488, 9.308390501180058507, -1.199719254218452047 ) ) ;
#152272=CARTESIAN_POINT ( 'NONE',  ( -5.017926250833627755, 5.026871178826882947, 0.7216878364870257245 ) ) ;
#152274=CARTESIAN_POINT ( 'NONE',  ( -3.458738584817664385, 7.049295759013638474, 0.7216878364870338292 ) ) ;
#152275=CARTESIAN_POINT ( 'NONE',  ( 4.655245641445829641, 6.524482229810530498, 1.599625672291269396 ) ) ;
#152276=CARTESIAN_POINT ( 'NONE',  ( -4.132202957115018727, 8.042930226601317401, 0.000000000000000000 ) ) ;
#152277=CARTESIAN_POINT ( 'NONE',  ( -5.271087860662956537, 9.371629280740593870, 0.000000000000000000 ) ) ;
#152331=CARTESIAN_POINT ( 'NONE',  ( 5.747730777550676073, 5.670383760089384495, 0.000000000000000000 ) ) ;
#152333=CARTESIAN_POINT ( 'NONE',  ( -3.930720324626924000, 8.992102070998189589, -0.7749999999999979128 ) ) ;
#152344=CARTESIAN_POINT ( 'NONE',  ( 1.843739406749204335, 8.499999999999996447, 0.7750000000000004663 ) ) ;
#152347=CARTESIAN_POINT ( 'NONE',  ( 5.876533236880477240, 5.820653295974182129, 0.7998128361456352531 ) ) ;
#152355=CARTESIAN_POINT ( 'NONE',  ( -6.831329296439251131, 9.063246493969506545, -1.599625672291271394 ) ) ;
#152365=DIRECTION ( 'NONE',  ( -0.8271092603120230313, 0.5620411653127359575, 0.000000000000000000 ) ) ;
#152369=CARTESIAN_POINT ( 'NONE',  ( 4.570507181582611267, 8.346359121906111511, 0.000000000000000000 ) ) ;
#152371=CARTESIAN_POINT ( 'NONE',  ( 1.930226670627054109, 8.999999999999998224, -0.7749999999999996891 ) ) ;
#152372=CARTESIAN_POINT ( 'NONE',  ( -5.906512197408906317, 6.919960980845699439, -1.199719254218453823 ) ) ;
#152381=EDGE_CURVE ( 'NONE', #95167, #138779, #34877, .T. ) ;
#152383=CARTESIAN_POINT ( 'NONE',  ( 3.040771591214902259, 6.769593633051179005, -0.7998128361456362523 ) ) ;
#152384=CARTESIAN_POINT ( 'NONE',  ( 5.574337433874081427, 6.532423756721743580, -1.199719254218452047 ) ) ;
#152404=CARTESIAN_POINT ( 'NONE',  ( 5.796475149741596056, 7.337953333587568849, -1.293683646293428913 ) ) ;
#152413=CARTESIAN_POINT ( 'NONE',  ( 3.576318658954677598, 7.394398545414291313, 0.7998128361456281477 ) ) ;
#152418=CARTESIAN_POINT ( 'NONE',  ( 4.681308178468477799, 8.683552984847038303, 0.000000000000000000 ) ) ;
#152423=CARTESIAN_POINT ( 'NONE',  ( 5.722950238744209273, 6.809768379023969587, 1.082531754730549967 ) ) ;
#152426=CARTESIAN_POINT ( 'NONE',  ( 6.943184063974162434, 9.193743722760251202, -1.443375672974064550 ) ) ;
#152435=CARTESIAN_POINT ( 'NONE',  ( 2.969872605471084448, 6.605953636083950364, 2.420000000000000373 ) ) ;
#152438=CARTESIAN_POINT ( 'NONE',  ( 6.463930056324285189, 6.765849701160138174, -0.2895399612845122039 ) ) ;
#152439=CARTESIAN_POINT ( 'NONE',  ( -3.902768115887413014, 5.646591783325653147, -1.599625672291283607 ) ) ;
#152464=CARTESIAN_POINT ( 'NONE',  ( 3.892599500454932304, 7.555466827257172113, 0.7216878364870257245 ) ) ;
#152472=CARTESIAN_POINT ( 'NONE',  ( 5.332099551924443404, 9.442809587212341427, 0.000000000000000000 ) ) ;
#152474=CARTESIAN_POINT ( 'NONE',  ( 7.523848900940885542, 7.742521570711348389, 0.7998128361456291469 ) ) ;
#152487=CARTESIAN_POINT ( 'NONE',  ( -4.176793841461789114, 7.030620694084159794, -1.199719254218455378 ) ) ;
#152489=CARTESIAN_POINT ( 'NONE',  ( 5.302647476276220573, 8.240153584747313076, -1.082531754730548412 ) ) ;
#152503=CARTESIAN_POINT ( 'NONE',  ( -6.455090533882193782, 9.584670485287619002, -1.082531754730549967 ) ) ;
#152505=CARTESIAN_POINT ( 'NONE',  ( -5.804299160426237059, 7.865044668620976509, -1.443375672974066548 ) ) ;
#152528=CARTESIAN_POINT ( 'NONE',  ( -4.468294144155606773, 7.370704380560280100, 1.199719254218452935 ) ) ;
#152530=CARTESIAN_POINT ( 'NONE',  ( -3.817502770699643388, 6.611447778194983194, 1.199719254218452935 ) ) ;
#152538=CARTESIAN_POINT ( 'NONE',  ( -5.249610431062532889, 7.793670086080374482, -1.296690129572550365 ) ) ;
#152552=CARTESIAN_POINT ( 'NONE',  ( 2.246985366953961449, 2.726529103553876787, 2.500000000000000444 ) ) ;
#152558=CARTESIAN_POINT ( 'NONE',  ( 4.629897721447052028, 8.429254678175810866, 0.5782609040035974202 ) ) ;
#152565=CARTESIAN_POINT ( 'NONE',  ( 0.000000000000000000, 2.999999999999999112, -2.420000000000000373 ) ) ;
#152569=CARTESIAN_POINT ( 'NONE',  ( 4.899292406491845497, 6.809203455697518947, -1.599625672291273171 ) ) ;
#152571=CARTESIAN_POINT ( 'NONE',  ( 3.840479349152599919, 7.346192795665340114, 0.4818892653144311033 ) ) ;
#152577=CARTESIAN_POINT ( 'NONE',  ( 6.526270840131753737, 8.707344961610770540, -1.599625672291283607 ) ) ;
#152579=CARTESIAN_POINT ( 'NONE',  ( 4.854701522145073334, 7.821512988214679218, -1.199719254218450271 ) ) ;
#152583=CARTESIAN_POINT ( 'NONE',  ( -2.744871144686030107, 2.962149295542713112, -2.500000000000111022 ) ) ;
#152592=CARTESIAN_POINT ( 'NONE',  ( 4.626831674679969808, 8.450518883791096059, -0.3637425496919588497 ) ) ;
#152595=CARTESIAN_POINT ( 'NONE',  ( -6.414416072596857532, 6.656109304217339151, -0.7216878364870338292 ) ) ;
#152596=CARTESIAN_POINT ( 'NONE',  ( 4.719646871332936477, 8.520355426614829142, -0.7216878364870357165 ) ) ;
#152604=CARTESIAN_POINT ( 'NONE',  ( -5.144392941742557568, 4.966489618313220333, -0.7998128361456362523 ) ) ;
#152616=CARTESIAN_POINT ( 'NONE',  ( -5.329763783503577379, 6.351050847909847086, 1.082531754730549078 ) ) ;
#152620=CARTESIAN_POINT ( 'NONE',  ( 5.692444392891300886, 7.734547439830227411, -1.599625672291281386 ) ) ;
#152644=CARTESIAN_POINT ( 'NONE',  ( -3.895996091634230218, 7.334980739573080832, 0.5863762202383783206 ) ) ;
#152650=CARTESIAN_POINT ( 'NONE',  ( 7.530627977747744062, 7.750430493652658015, -0.7998128361456341429 ) ) ;
#152655=VECTOR ( 'NONE', #135870, 1000.000000000000114 ) ;
#152659=ORIENTED_EDGE ( 'NONE', *, *, #35597, .T. ) ;
#152673=DIRECTION ( 'NONE',  ( 1.000000000000000000, 0.000000000000000000, 0.000000000000000000 ) ) ;
#152680=CARTESIAN_POINT ( 'NONE',  ( 5.248414862265931902, 5.295774558831261913, 0.000000000000000000 ) ) ;
#152686=CARTESIAN_POINT ( 'NONE',  ( -4.517335436343488553, 8.499999999999996447, -0.7750000000000013545 ) ) ;
#152688=CARTESIAN_POINT ( 'NONE',  ( 7.700104897918568447, 7.948153567185284096, 0.000000000000000000 ) ) ;
#152692=CARTESIAN_POINT ( 'NONE',  ( -4.502716413514313842, 5.386162249589033557, -1.082531754730549967 ) ) ;
#152701=CARTESIAN_POINT ( 'NONE',  ( -4.448483798615272100, 8.203998508444197313, 0.000000000000000000 ) ) ;
#152710=CARTESIAN_POINT ( 'NONE',  ( 8.154303043976348420, 8.478051404252736845, 0.7998128361456281477 ) ) ;
#152717=ORIENTED_EDGE ( 'NONE', *, *, #203130, .F. ) ;
#152720=CARTESIAN_POINT ( 'NONE',  ( 5.063044020060520900, 4.871582543017558109, 0.7998128361456352531 ) ) ;
#152723=ORIENTED_EDGE ( 'NONE', *, *, #17759, .T. ) ;
#152732=CARTESIAN_POINT ( 'NONE',  ( -4.977251789992602760, 8.820894498384422633, 0.000000000000000000 ) ) ;
#152733=ORIENTED_EDGE ( 'NONE', *, *, #28043, .F. ) ;
#152735=CARTESIAN_POINT ( 'NONE',  ( 5.840530312436913007, 10.03597880781023299, 0.000000000000000000 ) ) ;
#152738=CARTESIAN_POINT ( 'NONE',  ( -7.957709816578236506, 8.248692638954882028, 0.7998128361456341429 ) ) ;
#152741=CARTESIAN_POINT ( 'NONE',  ( -4.950662367645459305, 5.804802846121667415, -1.199719254218453823 ) ) ;
#152787=CARTESIAN_POINT ( 'NONE',  ( -5.119085517611572378, 8.129960982925583224, 1.199719254218452935 ) ) ;
#152791=CARTESIAN_POINT ( 'NONE',  ( -4.960304097753355457, 6.880383762169266504, 1.599625672291263179 ) ) ;
#152795=CARTESIAN_POINT ( 'NONE',  ( -6.143253000323532831, 7.300121600866474658, 1.082531754730548412 ) ) ;
#152802=CARTESIAN_POINT ( 'NONE',  ( -7.584860592202423035, 7.813701877183096833, -0.7998128361456362523 ) ) ;
#152806=ORIENTED_EDGE ( 'NONE', *, *, #103174, .T. ) ;
#152807=ORIENTED_EDGE ( 'NONE', *, *, #125818, .T. ) ;
#152811=CARTESIAN_POINT ( 'NONE',  ( -6.444921918449773024, 8.612437886315108315, 1.599625672291269396 ) ) ;
#152813=CARTESIAN_POINT ( 'NONE',  ( 5.214490215732396017, 7.828485850976955263, 1.269369371331245500 ) ) ;
#152818=CARTESIAN_POINT ( 'NONE',  ( 3.855102659574559443, 8.506872032338398171, 2.500000000000000444 ) ) ;
#152820=CARTESIAN_POINT ( 'NONE',  ( 6.343235766347262938, 8.493804042195527870, -1.599625672291281386 ) ) ;
#152845=CARTESIAN_POINT ( 'NONE',  ( 5.342795052237045539, 8.390955439988655229, -1.199719254218450271 ) ) ;
#152856=CARTESIAN_POINT ( 'NONE',  ( 0.3866926556111174862, 2.897682894409570054, 2.027578619373079594 ) ) ;
#152857=CARTESIAN_POINT ( 'NONE',  ( 5.845834525830363226, 7.300097092180095615, -1.274846751706928849 ) ) ;
#152863=DIRECTION ( 'NONE',  ( -0.6507913734559650498, 0.7592566023652995710, 0.000000000000000000 ) ) ;
#152869=ORIENTED_EDGE ( 'NONE', *, *, #146351, .T. ) ;
#152883=CARTESIAN_POINT ( 'NONE',  ( -6.564228937702958788, 6.791309396811020527, 0.4070866938790471679 ) ) ;
#152890=CARTESIAN_POINT ( 'NONE',  ( -3.231779075379147770, 6.036511184309971689, 7.500000000000000000 ) ) ;
#152901=CARTESIAN_POINT ( 'NONE',  ( -5.492988512192097161, 6.437516681426083132, 1.199719254218452935 ) ) ;
#152915=ORIENTED_EDGE ( 'NONE', *, *, #190788, .F. ) ;
#152919=CARTESIAN_POINT ( 'NONE',  ( 3.074666975249065626, 6.809138247757705820, 0.000000000000000000 ) ) ;
#152921=CARTESIAN_POINT ( 'NONE',  ( 6.902509602688803980, 9.146290184594002781, -1.443375672974064550 ) ) ;
#152935=CARTESIAN_POINT ( 'NONE',  ( -5.586841817283045408, 8.675676665875643678, 1.199719254218454489 ) ) ;
#152937=CARTESIAN_POINT ( 'NONE',  ( 5.180097208873055692, 8.201141289397330780, -1.199719254218450271 ) ) ;
#152947=DIRECTION ( 'NONE',  ( -0.7592566023652995710, 0.6507913734559650498, -0.000000000000000000 ) ) ;
#152948=CARTESIAN_POINT ( 'NONE',  ( -5.652823702255029836, 5.559658838911111900, -0.7998128361456362523 ) ) ;
#152949=CARTESIAN_POINT ( 'NONE',  ( 4.706615602599436343, 5.520081620234675412, 1.199719254218452935 ) ) ;
#152955=CARTESIAN_POINT ( 'NONE',  ( 5.501576472095266901, 9.640532660744973725, -0.7998128361456481317 ) ) ;
#152962=CARTESIAN_POINT ( 'NONE',  ( -5.196461137543813891, 7.842688287721260032, 1.273345793684066862 ) ) ;
#152974=CARTESIAN_POINT ( 'NONE',  ( -4.787437638956935082, 6.678706226906775179, -1.443375672974066548 ) ) ;
#152983=CARTESIAN_POINT ( 'NONE',  ( 3.431622278034673901, 7.017660067766835930, -1.734723475976807094E-15 ) ) ;
#152987=CARTESIAN_POINT ( 'NONE',  ( -5.773793314573309132, 7.829454515125894964, 1.599625672291263179 ) ) ;
#153024=CARTESIAN_POINT ( 'NONE',  ( -0.001208985763515336336, 3.412797577246581060, 2.002358321876673397 ) ) ;
#153027=CARTESIAN_POINT ( 'NONE',  ( -6.129694847154231852, 6.323934541200937787, -0.7216878364870338292 ) ) ;
#153051=CARTESIAN_POINT ( 'NONE',  ( -6.200875153403786477, 8.327716660428123419, -1.599625672291271394 ) ) ;
#153057=CARTESIAN_POINT ( 'NONE',  ( -4.604929450496978660, 5.401447776115099408, -1.199719254218453823 ) ) ;
#153060=CARTESIAN_POINT ( 'NONE',  ( 2.972033609136344623, 6.549060441754430251, -0.4946758370507742253 ) ) ;
#153066=CARTESIAN_POINT ( 'NONE',  ( -5.427006627220116286, 9.553534508390610469, -0.7998128361456362523 ) ) ;
#153068=CARTESIAN_POINT ( 'NONE',  ( 5.178155719255617129, 7.862379301422712352, -1.251444257556088457 ) ) ;
#153072=CARTESIAN_POINT ( 'NONE',  ( 4.065465959251388206, 5.836405933916976707, -1.599625672291269396 ) ) ;
#153077=CARTESIAN_POINT ( 'NONE',  ( -7.286581212701773502, 7.465709267765667789, 0.7998128361456341429 ) ) ;
#153080=CARTESIAN_POINT ( 'NONE',  ( -5.008811405605897882, 4.808311159487113073, 0.7998128361456281477 ) ) ;
#153084=CARTESIAN_POINT ( 'NONE',  ( -7.553300976144787349, 8.945177572657957654, -1.082531754730549967 ) ) ;
#153085=CARTESIAN_POINT ( 'NONE',  ( 4.543390873910913896, 5.433615786718446472, 1.082531754730549078 ) ) ;
#153086=CARTESIAN_POINT ( 'NONE',  ( -5.275531169048911728, 6.287779464379406491, -1.082531754730549967 ) ) ;
#153092=CARTESIAN_POINT ( 'NONE',  ( -5.635349125135588721, 6.603604063193491136, 1.199719254218452935 ) ) ;
#153101=CARTESIAN_POINT ( 'NONE',  ( 4.366607992053101128, 7.252070536440704096, -1.199719254218448494 ) ) ;
#153105=CARTESIAN_POINT ( 'NONE',  ( 1.870725386045717142, 2.481143736744112704, 2.471938233550914354 ) ) ;
#153106=CARTESIAN_POINT ( 'NONE',  ( 6.090086331970060662, 7.118959255344424086, 1.132899493623270359 ) ) ;
#153116=CARTESIAN_POINT ( 'NONE',  ( 6.875920180786008196, 8.050936961452347163, -1.199719254218452047 ) ) ;
#153120=CARTESIAN_POINT ( 'NONE',  ( -6.486624235763164492, 6.835203243035253173, 0.7121179707554707861 ) ) ;
#153127=CARTESIAN_POINT ( 'NONE',  ( 5.590372323399994237, 7.390087136190794936, 1.241407824010079652 ) ) ;
#153143=CARTESIAN_POINT ( 'NONE',  ( -4.457598643843001973, 8.422558527783969851, 0.000000000000000000 ) ) ;
#153156=CARTESIAN_POINT ( 'NONE',  ( 4.701645408888975197, 8.707279753670952971, 0.000000000000000000 ) ) ;
#153158=CARTESIAN_POINT ( 'NONE',  ( 5.969332771766739931, 10.18624834369502885, -0.7998128361456481317 ) ) ;
#153167=CARTESIAN_POINT ( 'NONE',  ( 3.079110283634975964, 6.606396074300548982, 0.7216878364870257245 ) ) ;
#153175=CARTESIAN_POINT ( 'NONE',  ( 1.921775512840651956, 9.000000000008071765, 0.7750000000000004663 ) ) ;
#153182=CARTESIAN_POINT ( 'NONE',  ( -6.400857919427531684, 9.521399101757175742, 1.082531754730549967 ) ) ;
#153183=CARTESIAN_POINT ( 'NONE',  ( 5.722950238744198614, 8.730506807626655430, 1.082531754730549967 ) ) ;
#153189=ORIENTED_EDGE ( 'NONE', *, *, #30238, .F. ) ;
#153190=CARTESIAN_POINT ( 'NONE',  ( -4.370663978927099791, 5.060324124126027279, 7.500000000000000000 ) ) ;
#153194=CARTESIAN_POINT ( 'NONE',  ( -4.659162064951642535, 5.464719159645540003, 1.199719254218452935 ) ) ;
#153195=CARTESIAN_POINT ( 'NONE',  ( -6.116136693540540570, 10.14959355252370266, 0.000000000000000000 ) ) ;
#153198=CARTESIAN_POINT ( 'NONE',  ( 5.194182247366868843, 8.113610817686430110, 1.082531754730548412 ) ) ;
#153204=CARTESIAN_POINT ( 'NONE',  ( -5.570361349191150779, 5.866663122702686195, 0.5491554309224304653 ) ) ;
#153211=CARTESIAN_POINT ( 'NONE',  ( -4.624779211906307808, 8.357533986720639518, 0.2900094174717957607 ) ) ;
#153219=CARTESIAN_POINT ( 'NONE',  ( -5.926849427829407269, 6.943687749669614995, -1.199719254218453823 ) ) ;
#153230=CARTESIAN_POINT ( 'NONE',  ( 4.206772801990143584, 8.129928378955675328, 0.7998128361456271485 ) ) ;
#153264=CARTESIAN_POINT ( 'NONE',  ( 6.373741612200171325, 7.569024981389272710, 1.082531754730549967 ) ) ;
#153269=CARTESIAN_POINT ( 'NONE',  ( 4.855228407025239612, 8.678533884922511987, 0.000000000000000000 ) ) ;
#153285=CARTESIAN_POINT ( 'NONE',  ( -7.469616286486262524, 7.679250187180907794, 0.7998128361456341429 ) ) ;
#153297=CARTESIAN_POINT ( 'NONE',  ( 5.356880090730874677, 5.422317325373725794, 0.7216878364870328300 ) ) ;
#153304=CARTESIAN_POINT ( 'NONE',  ( -5.517242166118370150, 5.401480380085008193, 0.7998128361456281477 ) ) ;
#153310=CARTESIAN_POINT ( 'NONE',  ( -5.451787166470911217, 9.374519104275787384, 0.7216878364870267237 ) ) ;
#153313=CARTESIAN_POINT ( 'NONE',  ( -5.589704470584107909, 9.743348658981940247, -0.7998128361456362523 ) ) ;
#153329=CIRCLE ( 'NONE', #115365, 0.08000000000000012657 ) ;
#153334=CARTESIAN_POINT ( 'NONE',  ( -3.662110889467009578, 7.286563447771212232, 0.7216878364870338292 ) ) ;
#153337=CARTESIAN_POINT ( 'NONE',  ( -4.624739795592936353, 7.449261290616792763, -1.082531754730549967 ) ) ;
#153339=CARTESIAN_POINT ( 'NONE',  ( 4.441177836928239309, 7.339068688795062911, 1.199719254218452047 ) ) ;
#153340=CARTESIAN_POINT ( 'NONE',  ( -5.167592825464113915, 6.057888380243431570, 1.199719254218452935 ) ) ;
#153341=CARTESIAN_POINT ( 'NONE',  ( -5.094831863685302942, 9.165997284266655498, 0.7998128361456291469 ) ) ;
#153358=CARTESIAN_POINT ( 'NONE',  ( 7.013428937081386927, 5.939655416065874327, 2.436399677959149468 ) ) ;
#153393=CARTESIAN_POINT ( 'NONE',  ( 6.387299765813869712, 6.624473612970537495, 0.000000000000000000 ) ) ;
#153398=CARTESIAN_POINT ( 'NONE',  ( 4.875038752565570732, 7.845239757038595663, -1.199719254218452047 ) ) ;
#153400=CARTESIAN_POINT ( 'NONE',  ( -3.947104627881522720, 8.980740528188976057, -0.7749999999999979128 ) ) ;
#153401=CARTESIAN_POINT ( 'NONE',  ( -3.719872605471121751, 6.605953636083950364, 2.420000000000000373 ) ) ;
#153416=CARTESIAN_POINT ( 'NONE',  ( 4.206772801990143584, 8.129928378955675328, 0.7998128361456271485 ) ) ;
#153424=CARTESIAN_POINT ( 'NONE',  ( -6.882699257592852504, 8.058845884393651460, -1.199719254218452047 ) ) ;
#153429=CARTESIAN_POINT ( 'NONE',  ( 6.249382461256315580, 6.255644057745969988, -0.7998128361456481317 ) ) ;
#153441=CARTESIAN_POINT ( 'NONE',  ( 5.072158865288222351, 8.931619419562697004, 0.7216878364870317197 ) ) ;
#153443=CARTESIAN_POINT ( 'NONE',  ( -3.675669043080673770, 7.302381293653823491, 0.000000000000000000 ) ) ;
#153444=CARTESIAN_POINT ( 'NONE',  ( -5.692444392891315097, 7.734547439830227411, -1.599625672291271394 ) ) ;
#153454=CARTESIAN_POINT ( 'NONE',  ( 4.878955176071345434, 6.785476686873604280, -1.599625672291269396 ) ) ;
#153455=CARTESIAN_POINT ( 'NONE',  ( 5.899733120602060232, 6.912052057904395141, -1.199719254218452047 ) ) ;
#153473=CARTESIAN_POINT ( 'NONE',  ( 5.991454128980707949, 7.190850779781567503, -1.201235417510186254 ) ) ;
#153476=ADVANCED_FACE ( 'NONE', ( #148402 ), #75426, .T. ) ;
#153481=AXIS2_PLACEMENT_3D ( 'NONE', #136616, #199447, #201572 ) ;
#153484=CARTESIAN_POINT ( 'NONE',  ( 5.747730777550676073, 5.670383760089384495, 0.000000000000000000 ) ) ;
#153489=CARTESIAN_POINT ( 'NONE',  ( 7.842465510862060896, 8.114240948952696542, 0.000000000000000000 ) ) ;
#153494=CARTESIAN_POINT ( 'NONE',  ( 5.506019780925567986, 8.477421273504887722, -1.082531754730548412 ) ) ;
#153498=CARTESIAN_POINT ( 'NONE',  ( 4.927462483923885195, 4.713404084191450849, -0.7998128361456481317 ) ) ;
#153510=CARTESIAN_POINT ( 'NONE',  ( 6.465908158583062892, 6.764574590967027845, 0.2795716154820517829 ) ) ;
#153511=CARTESIAN_POINT ( 'NONE',  ( -7.756673280794142755, 8.222076047114187602, -0.7216878364870338292 ) ) ;
#153520=CARTESIAN_POINT ( 'NONE',  ( 0.4132722983370792913, 3.247815196129578919, -1.957108758695520923 ) ) ;
#153527=LINE ( 'NONE', #88534, #76385 ) ;
#153529=EDGE_LOOP ( 'NONE', ( #115564, #70053, #176403, #72215 ) ) ;
#153544=CARTESIAN_POINT ( 'NONE',  ( 7.354371980770088690, 7.544798497178720531, 0.000000000000000000 ) ) ;
#153546=CARTESIAN_POINT ( 'NONE',  ( 7.537407054554579489, 7.758339416593960536, 0.000000000000000000 ) ) ;
#153560=CARTESIAN_POINT ( 'NONE',  ( -4.960304097753355457, 6.880383762169266504, 1.599625672291263179 ) ) ;
#153562=CARTESIAN_POINT ( 'NONE',  ( 6.522881301506172846, 6.782652071278222117, -0.7216878364870458196 ) ) ;
#153572=CARTESIAN_POINT ( 'NONE',  ( -4.014095998097799267, 6.840806543492835345, -1.199719254218450271 ) ) ;
#153575=CARTESIAN_POINT ( 'NONE',  ( -2.875737979874388284, 6.369128386579808954, -0.7216878364870458196 ) ) ;
#153579=CARTESIAN_POINT ( 'NONE',  ( -3.461074353238556167, 7.259946855412102273, 0.000000000000000000 ) ) ;
#153581=CARTESIAN_POINT ( 'NONE',  ( -5.316205630334255972, 8.255971431148344308, -1.082531754730549967 ) ) ;
#153605=CARTESIAN_POINT ( 'NONE',  ( -5.601453741101424022, 6.564059448486966986, -1.199719254218453823 ) ) ;
#153615=CARTESIAN_POINT ( 'NONE',  ( -6.514548575684607989, 6.824011503973982151, -0.5624163230865379948 ) ) ;
#153623=CARTESIAN_POINT ( 'NONE',  ( -3.810548893104181101, 8.469546410357015276, 2.500000000000000000 ) ) ;
#153630=CARTESIAN_POINT ( 'NONE',  ( 1.772846837484799210, 2.502368107626177451, 2.500000000000000444 ) ) ;
#153640=EDGE_CURVE ( 'NONE', #138803, #68330, #18400, .T. ) ;
#153649=CARTESIAN_POINT ( 'NONE',  ( 5.248941747146098180, 6.152795455539095570, -1.199719254218452047 ) ) ;
#153651=CARTESIAN_POINT ( 'NONE',  ( 3.901829752285186803, 7.334923791204486676, 0.6872182573793610416 ) ) ;
#153658=CARTESIAN_POINT ( 'NONE',  ( 5.338878628731272613, 9.450718510153643948, -0.7998128361456481317 ) ) ;
#153660=CARTESIAN_POINT ( 'NONE',  ( 5.020262018810099924, 9.078999131912302900, 0.7998128361456331437 ) ) ;
#153673=CARTESIAN_POINT ( 'NONE',  ( 6.476386945563378461, 6.757828299745357370, 0.2189195654383000456 ) ) ;
#153675=CARTESIAN_POINT ( 'NONE',  ( 5.722950238744209273, 6.809768379023969587, 1.082531754730549967 ) ) ;
#153692=CARTESIAN_POINT ( 'NONE',  ( -4.611181641979265500, 8.393812659035525314, 0.000000000000000000 ) ) ;
#153697=CARTESIAN_POINT ( 'NONE',  ( 5.169401708560450004, 9.252995436621013425, 0.000000000000000000 ) ) ;
#153714=CARTESIAN_POINT ( 'NONE',  ( -7.013428937081434000, 5.939655416065874327, -2.436399677959149468 ) ) ;
#153743=CARTESIAN_POINT ( 'NONE',  ( -5.602498012743508227, 5.726462300312828546, -0.1687859242097844992 ) ) ;
#153752=CARTESIAN_POINT ( 'NONE',  ( 4.258669648468278446, 7.022179452304728287, 1.082531754730549078 ) ) ;
#153757=CARTESIAN_POINT ( 'NONE',  ( -7.095713291905736853, 9.371694488680407886, 1.599625672291269396 ) ) ;
#153759=CARTESIAN_POINT ( 'NONE',  ( 5.851225812749518695, 8.984124660586543243, -1.199719254218452047 ) ) ;
#153764=CARTESIAN_POINT ( 'NONE',  ( -5.316205630334268406, 6.335233002545657577, -1.082531754730549967 ) ) ;
#153767=EDGE_LOOP ( 'NONE', ( #122902, #139230, #206175, #75381, #142261, #66710, #151862, #50442, #174557, #160633, #187800, #10255, #53715, #56565, #169437, #193563 ) ) ;
#153768=DIRECTION ( 'NONE',  ( -1.000000000000000000, 0.000000000000000000, 0.000000000000000000 ) ) ;
#153794=CARTESIAN_POINT ( 'NONE',  ( 5.546694241766559230, 9.485244025454063532, 0.000000000000000000 ) ) ;
#153808=CARTESIAN_POINT ( 'NONE',  ( -4.177320726786315497, 7.887641591310407208, -0.7216878364870458196 ) ) ;
#153809=ORIENTED_EDGE ( 'NONE', *, *, #150631, .F. ) ;
#153811=CARTESIAN_POINT ( 'NONE',  ( 7.537407054554579489, 7.758339416593960536, 0.000000000000000000 ) ) ;
#153813=B_SPLINE_CURVE_WITH_KNOTS ( 'NONE', 3,
 ( #77295, #90358, #74102, #10151, #57842, #158554 ),
 .UNSPECIFIED., .F., .F.,
 ( 4, 2, 4 ),
 ( 0.000000000000000000, 0.002406600572792975002, 0.004813201145585950871 ),
 .UNSPECIFIED. ) ;
#153817=CARTESIAN_POINT ( 'NONE',  ( -5.224688093219839402, 7.188831756880171397, -1.599625672291271394 ) ) ;
#153825=AXIS2_PLACEMENT_3D ( 'NONE', #73273, #8282, #25596 ) ;
#153827=CYLINDRICAL_SURFACE ( 'NONE', #175202, 0.7499999999999997780 ) ;
#153847=VERTEX_POINT ( 'NONE', #130092 ) ;
#153858=PLANE ( 'NONE',  #12960 ) ;
#153859=CARTESIAN_POINT ( 'NONE',  ( 5.411112705629925301, 5.485588709422586362, 0.000000000000000000 ) ) ;
#153863=CARTESIAN_POINT ( 'NONE',  ( -5.094831863685302942, 9.165997284266655498, 0.7998128361456291469 ) ) ;
#153867=CARTESIAN_POINT ( 'NONE',  ( -5.448397627845328550, 7.449826213943242514, 1.599625672291263179 ) ) ;
#153868=CARTESIAN_POINT ( 'NONE',  ( -6.140917232347002042, 6.129101290685087911, -0.7998128361456361413 ) ) ;
#153872=CARTESIAN_POINT ( 'NONE',  ( -6.739811759324831897, 7.996106819701333634, -1.082531754730549967 ) ) ;
#153878=ORIENTED_EDGE ( 'NONE', *, *, #195731, .F. ) ;
#153879=CARTESIAN_POINT ( 'NONE',  ( -6.454563648557663846, 9.688018802362710957, -1.199719254218452047 ) ) ;
#153886=CARTESIAN_POINT ( 'NONE',  ( -6.583366107887490770, 9.838288338247510367, 1.199719254218452935 ) ) ;
#153887=ORIENTED_EDGE ( 'NONE', *, *, #163618, .F. ) ;
#153888=CARTESIAN_POINT ( 'NONE',  ( 5.260375520412221562, 7.786458765878076171, 1.288147692060326532 ) ) ;
#153893=CARTESIAN_POINT ( 'NONE',  ( 3.237364818613055473, 6.998952398349030268, -1.734723475976807094E-15 ) ) ;
#153904=CARTESIAN_POINT ( 'NONE',  ( -5.966470118465691641, 9.118576350588734059, -1.199719254218452047 ) ) ;
#153916=CARTESIAN_POINT ( 'NONE',  ( 6.481679955784983349, 9.719654494127929922, -1.199719254218452047 ) ) ;
#153931=CARTESIAN_POINT ( 'NONE',  ( 5.950060389077887812, 7.221515259811701171, 1.225279837341096689 ) ) ;
#153959=CARTESIAN_POINT ( 'NONE',  ( -5.971735067414164710, 7.203215006737162085, 1.225879040106806706 ) ) ;
#153977=CARTESIAN_POINT ( 'NONE',  ( -6.791708605802965870, 6.888357893050385705, -0.7998128361456362523 ) ) ;
#153993=CARTESIAN_POINT ( 'NONE',  ( 3.573456005653643519, 6.326726552307992080, -1.199719254218453823 ) ) ;
#153995=CARTESIAN_POINT ( 'NONE',  ( 6.170369307550816806, 9.252495721234380355, 1.082531754730549967 ) ) ;
#153998=EDGE_CURVE ( 'NONE', #179867, #40807, #40569, .T. ) ;
#154012=CARTESIAN_POINT ( 'NONE',  ( 6.039231080244466199, 6.010467446565510130, 0.7998128361456352531 ) ) ;
#154022=CARTESIAN_POINT ( 'NONE',  ( -4.359828915246279024, 7.244161613499399799, -1.199719254218455378 ) ) ;
#154023=CARTESIAN_POINT ( 'NONE',  ( 5.969332771766739931, 10.18624834369502885, -0.7998128361456481317 ) ) ;
#154027=CARTESIAN_POINT ( 'NONE',  ( -6.557303570864871034, 7.679217583210999010, -1.199719254218452047 ) ) ;
#154029=ORIENTED_EDGE ( 'NONE', *, *, #35597, .F. ) ;
#154030=CARTESIAN_POINT ( 'NONE',  ( 6.119526231721748033, 8.232809585132461194, 1.599625672291269396 ) ) ;
#154035=CARTESIAN_POINT ( 'NONE',  ( -4.584908210271880336, 8.498668195373706880, -0.01721603403951645073 ) ) ;
#154045=CARTESIAN_POINT ( 'NONE',  ( -5.614485009390564940, 5.722856397143323726, 0.000000000000000000 ) ) ;
#154056=CARTESIAN_POINT ( 'NONE',  ( 3.607878275012313285, 6.262922849939428716, 1.082531754730549078 ) ) ;
#154059=CARTESIAN_POINT ( 'NONE',  ( 5.063152511717405879, 4.908155404373435005, -0.2552525419090029835 ) ) ;
#154060=CARTESIAN_POINT ( 'NONE',  ( -7.123883369337781879, 7.275895117174344229, 0.7998128361456341429 ) ) ;
#154061=ADVANCED_FACE ( 'NONE', ( #42941 ), #176131, .T. ) ;
#154077=CARTESIAN_POINT ( 'NONE',  ( -4.869786032514803686, 4.879826965026095031, -0.6311548526560835093 ) ) ;
#154098=CARTESIAN_POINT ( 'NONE',  ( -5.478903473698260029, 6.525047153136981137, -1.082531754730549967 ) ) ;
#154123=CARTESIAN_POINT ( 'NONE',  ( -6.095272577795516789, 9.268845886473535245, 1.199719254218452047 ) ) ;
#154130=CARTESIAN_POINT ( 'NONE',  ( -3.634467696915153034, 6.397906858779740524, 1.199719254218452935 ) ) ;
#154134=EDGE_LOOP ( 'NONE', ( #106893, #58358, #89032, #3564 ) ) ;
#154140=CARTESIAN_POINT ( 'NONE',  ( -5.015590482412729756, 4.816220082428420923, 0.000000000000000000 ) ) ;
#154142=CARTESIAN_POINT ( 'NONE',  ( 5.269423316188119877, 7.778230059001682406, -1.291559732514224068 ) ) ;
#154147=CARTESIAN_POINT ( 'NONE',  ( 5.662465432362883355, 6.635239754958710989, 1.199719254218451159 ) ) ;
#154152=CARTESIAN_POINT ( 'NONE',  ( -6.180537922983287302, 8.303989891604203422, -1.599625672291271394 ) ) ;
#154156=CARTESIAN_POINT ( 'NONE',  ( -3.797165540279144214, 6.587721009371067638, 1.199719254218452935 ) ) ;
#154159=CARTESIAN_POINT ( 'NONE',  ( 5.153507786970260796, 7.105788066255672497, -1.443375672974078316 ) ) ;
#154160=CARTESIAN_POINT ( 'NONE',  ( 5.031484404002889654, 6.003058238492422483, 1.082531754730549078 ) ) ;
#154162=CARTESIAN_POINT ( 'NONE',  ( -4.706088717274938382, 6.583799151611112954, 1.443375672974058777 ) ) ;
#154164=ADVANCED_FACE ( 'NONE', ( #23440 ), #113530, .T. ) ;
#154169=CARTESIAN_POINT ( 'NONE',  ( 4.634908411025333130, 6.500755460986618495, 1.599625672291268286 ) ) ;
#154175=CARTESIAN_POINT ( 'NONE',  ( 6.039231080244466199, 6.010467446565509242, 0.7998128361456350310 ) ) ;
#154179=CARTESIAN_POINT ( 'NONE',  ( 0.3999999999999758193, 3.000000000029069636, -2.023857702507768419 ) ) ;
#154180=CARTESIAN_POINT ( 'NONE',  ( 5.770588788983777917, 7.358121641400980018, 1.301467365913897112 ) ) ;
#154189=CARTESIAN_POINT ( 'NONE',  ( 5.338878628731272613, 9.450718510153643948, -0.7998128361456481317 ) ) ;
#154200=CARTESIAN_POINT ( 'NONE',  ( 6.335378924966214242, 6.849830188997488634, 0.6565068261209184852 ) ) ;
#154214=CARTESIAN_POINT ( 'NONE',  ( -4.847922445338252118, 7.813604065273374921, -1.199719254218453823 ) ) ;
#154218=DIRECTION ( 'NONE',  ( 0.000000000000000000, 0.000000000000000000, -1.000000000000000000 ) ) ;
#154228=CARTESIAN_POINT ( 'NONE',  ( 5.899733120602060232, 6.912052057904395141, -1.199719254218452047 ) ) ;
#154235=CARTESIAN_POINT ( 'NONE',  ( -4.138282870000122848, 7.235124601197615135, 0.9996976134348694032 ) ) ;
#154237=CARTESIAN_POINT ( 'NONE',  ( -8.068510813464099485, 8.585886501895810596, 0.7216878364870317197 ) ) ;
#154238=VERTEX_POINT ( 'NONE', #110119 ) ;
#154243=CARTESIAN_POINT ( 'NONE',  ( 4.868786560638896255, 5.813244087901094481, 1.082531754730549078 ) ) ;
#154259=CARTESIAN_POINT ( 'NONE',  ( -7.485510208520816278, 8.866088343763324886, 1.082531754730549078 ) ) ;
#154261=CARTESIAN_POINT ( 'NONE',  ( 6.211043768836173484, 8.339580045099285854, 1.443375672974065660 ) ) ;
#154266=VERTEX_POINT ( 'NONE', #92757 ) ;
#154271=CARTESIAN_POINT ( 'NONE',  ( -5.285699784481336927, 7.260012063351913625, 1.599625672291263179 ) ) ;
#154272=CARTESIAN_POINT ( 'NONE',  ( -4.309512724297390740, 6.121127159803966933, 1.599625672291270506 ) ) ;
#154274=CARTESIAN_POINT ( 'NONE',  ( 5.017926250389229459, 8.868348035513836436, 0.000000000000000000 ) ) ;
#154278=DIRECTION ( 'NONE',  ( -0.000000000000000000, -1.000000000000000000, -0.000000000000000000 ) ) ;
#154285=CARTESIAN_POINT ( 'NONE',  ( -4.613315975161869531, 8.372148359400446438, -0.1986654441144524719 ) ) ;
#154288=CARTESIAN_POINT ( 'NONE',  ( 4.584065335196261692, 7.401807753487379848, 1.082531754730549078 ) ) ;
#154292=CARTESIAN_POINT ( 'NONE',  ( -4.118644803501354978, 8.027112380718707030, 0.7998128361456352531 ) ) ;
#154304=VECTOR ( 'NONE', #31797, 1000.000000000000114 ) ;
#154306=CARTESIAN_POINT ( 'NONE',  ( 3.691562964670865199, 7.528850235416478576, -0.7998128361456362523 ) ) ;
#154320=CARTESIAN_POINT ( 'NONE',  ( -5.763624699140887486, 5.896852701852046685, -0.7216878364870392693 ) ) ;
#154331=EDGE_LOOP ( 'NONE', ( #204281, #142869, #107857, #63939, #134833 ) ) ;
#154340=CARTESIAN_POINT ( 'NONE',  ( 6.726253606155519371, 7.019919760035800316, -0.7216878364870458196 ) ) ;
#154345=CARTESIAN_POINT ( 'NONE',  ( 6.061904078641523697, 7.205214525570814210, -1.082531754730548412 ) ) ;
#154359=CARTESIAN_POINT ( 'NONE',  ( -8.120407659942227241, 8.438506789546210030, 0.7998128361456341429 ) ) ;
#154373=CARTESIAN_POINT ( 'NONE',  ( 3.390947816749319443, 6.970206529600588397, -1.734723475976807094E-15 ) ) ;
#154379=CARTESIAN_POINT ( 'NONE',  ( -6.064239847062411926, 10.29697326487330500, 0.000000000000000000 ) ) ;
#154384=CARTESIAN_POINT ( 'NONE',  ( -5.804299160426229953, 8.825413882922319431, -1.082531754730549967 ) ) ;
#154387=CARTESIAN_POINT ( 'NONE',  ( -5.887983850084758330, 10.09134126839936840, 0.7998128361456291469 ) ) ;
#154392=CARTESIAN_POINT ( 'NONE',  ( -5.418418667316934112, 6.350518529071726981, -1.199719254218453823 ) ) ;
#154406=CARTESIAN_POINT ( 'NONE',  ( -4.584065335196305213, 6.441438539186039591, 1.443375672974058777 ) ) ;
#154408=CARTESIAN_POINT ( 'NONE',  ( -5.112833325684920993, 6.097965313788082931, -1.082531754730549967 ) ) ;
#154410=CARTESIAN_POINT ( 'NONE',  ( 4.362691568547328202, 8.311833606605697256, -0.7998128361456381397 ) ) ;
#154411=CARTESIAN_POINT ( 'NONE',  ( -5.875479466675803231, 7.948088359245467416, -1.599625672291271394 ) ) ;
#154412=CARTESIAN_POINT ( 'NONE',  ( -6.149505192250180663, 9.332117270003974951, -1.199719254218452047 ) ) ;
#154438=CARTESIAN_POINT ( 'NONE',  ( -5.574622267388016361, 7.504663849841638701, -1.387123747601160639 ) ) ;
#154461=CARTESIAN_POINT ( 'NONE',  ( 5.071913926361915514, 4.910694714577345188, 0.2269669051133595961 ) ) ;
#154473=CARTESIAN_POINT ( 'NONE',  ( 4.712340909201580885, 7.655425606447271214, -1.199719254218452047 ) ) ;
#154490=CARTESIAN_POINT ( 'NONE',  ( 3.705121118284530279, 7.544668081299086282, -1.734723475976807094E-15 ) ) ;
#154495=CARTESIAN_POINT ( 'NONE',  ( -5.738844160334429567, 9.917344963690652548, 0.000000000000000000 ) ) ;
#154500=CARTESIAN_POINT ( 'NONE',  ( 3.888156192069020634, 7.758209000714329839, 1.040834085586084257E-14 ) ) ;
#154509=CARTESIAN_POINT ( 'NONE',  ( 6.211043768836173484, 8.339580045099285854, 1.443375672974065660 ) ) ;
#154510=CARTESIAN_POINT ( 'NONE',  ( -5.153507786970285665, 5.185049637652990207, -0.7216878364870338292 ) ) ;
#154511=ADVANCED_FACE ( 'NONE', ( #178263 ), #128524, .F. ) ;
#154512=CARTESIAN_POINT ( 'NONE',  ( -4.827585214917754719, 7.789877296449459365, -1.199719254218453823 ) ) ;
#154524=CARTESIAN_POINT ( 'NONE',  ( 5.825163275726873202, 6.825053905550038991, 1.199719254218452047 ) ) ;
#154525=CARTESIAN_POINT ( 'NONE',  ( 5.468734858265785093, 7.473552982767158070, 1.599625672291269396 ) ) ;
#154546=CARTESIAN_POINT ( 'NONE',  ( 0.3999999999999758193, 3.000000000000047518, 2.023857702507768419 ) ) ;
#154552=AXIS2_PLACEMENT_3D ( 'NONE', #160166, #159097, #59461 ) ;
#154553=CARTESIAN_POINT ( 'NONE',  ( 5.435893244436359240, 5.306573304789342416, -0.7998128361456481317 ) ) ;
#154557=CARTESIAN_POINT ( 'NONE',  ( 4.004454267989866700, 5.765225627445230927, 1.599625672291262513 ) ) ;
#154564=CARTESIAN_POINT ( 'NONE',  ( 4.394251184604957672, 8.140727125432173139, -0.7216878364870357165 ) ) ;
#154566=CARTESIAN_POINT ( 'NONE',  ( -4.685224601974262271, 7.623789914682047808, -1.199719254218453823 ) ) ;
#154568=CARTESIAN_POINT ( 'NONE',  ( 4.740510986633625024, 5.559626234941203116, -1.199719254218450271 ) ) ;
#154579=CARTESIAN_POINT ( 'NONE',  ( 6.385878362533466301, 6.816559200039058020, 0.5486352003098924346 ) ) ;
#154580=CARTESIAN_POINT ( 'NONE',  ( -7.431277594066152403, 8.802816960232885179, -1.082531754730549967 ) ) ;
#154613=CARTESIAN_POINT ( 'NONE',  ( 5.657495238652423097, 9.822437888394988548, 0.000000000000000000 ) ) ;
#154615=CARTESIAN_POINT ( 'NONE',  ( 6.200875153403774043, 8.327716660428123419, -1.599625672291283607 ) ) ;
#154628=CARTESIAN_POINT ( 'NONE',  ( -3.474632506852224356, 7.275764701294714420, -0.7998128361456481317 ) ) ;
#154630=CARTESIAN_POINT ( 'NONE',  ( 6.672020991256494504, 6.956648375986938859, 0.000000000000000000 ) ) ;
#154639=CARTESIAN_POINT ( 'NONE',  ( -5.581116510680924847, 6.540332679663050541, -1.199719254218453823 ) ) ;
#154642=CARTESIAN_POINT ( 'NONE',  ( -4.394251184604987870, 5.259619482528146150, 1.082531754730549078 ) ) ;
#154645=CARTESIAN_POINT ( 'NONE',  ( -5.307090785106547415, 5.156303768904543894, -0.7998128361456362523 ) ) ;
#154667=CARTESIAN_POINT ( 'NONE',  ( -4.118644803501354978, 8.027112380718707030, 0.7998128361456352531 ) ) ;
#154679=CARTESIAN_POINT ( 'NONE',  ( -6.117836340636773507, 7.096790560477957754, -1.125390141808879196 ) ) ;
#154695=CARTESIAN_POINT ( 'NONE',  ( -5.631432701629818460, 7.663367133358481631, 1.599625672291263179 ) ) ;
#154703=CARTESIAN_POINT ( 'NONE',  ( 6.441532379824158383, 9.568852638886589546, -1.082531754730548412 ) ) ;
#154712=CARTESIAN_POINT ( 'NONE',  ( -3.231779075379149546, 6.036511184309971689, -2.419999999999998597 ) ) ;
#154716=CARTESIAN_POINT ( 'NONE',  ( 4.278479993564246797, 7.149254538203735798, 1.199719254218452047 ) ) ;
#154724=CARTESIAN_POINT ( 'NONE',  ( 6.200875153403774043, 8.327716660428123419, -1.599625672291283607 ) ) ;
#154726=CARTESIAN_POINT ( 'NONE',  ( 5.017399365509065845, 8.011327138806002779, -1.199719254218450271 ) ) ;
#154739=CARTESIAN_POINT ( 'NONE',  ( 6.450676980830294838, 6.774405823990504949, -0.3487213023658369826 ) ) ;
#154741=CARTESIAN_POINT ( 'NONE',  ( 4.909461021924240498, 7.781436054670031410, 1.082531754730549078 ) ) ;
#154749=CARTESIAN_POINT ( 'NONE',  ( -4.604929450496978660, 5.401447776115099408, -1.199719254218453823 ) ) ;
#154759=CARTESIAN_POINT ( 'NONE',  ( -5.980555156959541208, 7.110307450275150210, 1.082531754730549078 ) ) ;
#154764=CARTESIAN_POINT ( 'NONE',  ( 5.318541398310776103, 9.426991741329731056, -0.7998128361456481317 ) ) ;
#154790=CARTESIAN_POINT ( 'NONE',  ( 5.704304454332028484, 5.827645749575025569, -0.4508780309788811835 ) ) ;
#154820=EDGE_LOOP ( 'NONE', ( #24035, #183776, #168522, #6047 ) ) ;
#154821=CARTESIAN_POINT ( 'NONE',  ( 4.204437034013637664, 6.958908068774287692, -1.082531754730548412 ) ) ;
#154826=CARTESIAN_POINT ( 'NONE',  ( -8.093291352714894415, 8.406871097780989288, -0.7998128361456362523 ) ) ;
#154828=CARTESIAN_POINT ( 'NONE',  ( 7.014364370223726830, 9.276787413384745662, -1.599625672291269396 ) ) ;
#154833=CARTESIAN_POINT ( 'NONE',  ( -3.336715202739028552, 6.906935146588564223, 0.7216878364870338292 ) ) ;
#154864=CARTESIAN_POINT ( 'NONE',  ( 5.709392085130549077, 9.675058176045386205, 0.000000000000000000 ) ) ;
#154876=CARTESIAN_POINT ( 'NONE',  ( -4.814553946628611136, 8.631080347793099961, 0.000000000000000000 ) ) ;
#154879=CARTESIAN_POINT ( 'NONE',  ( 5.338878628731272613, 9.450718510153643948, -0.7998128361456481317 ) ) ;
#154884=CARTESIAN_POINT ( 'NONE',  ( -3.983063267364693960, 7.868933921892603323, -0.7998128361456481317 ) ) ;
#154927=CARTESIAN_POINT ( 'NONE',  ( -7.930593509350902792, 8.217056947189661287, -0.7998128361456362523 ) ) ;
#154930=CARTESIAN_POINT ( 'NONE',  ( -5.101610940492132151, 9.173906207207963348, -0.7998128361456362523 ) ) ;
#154931=CARTESIAN_POINT ( 'NONE',  ( -6.005335696210345020, 5.970922831858983315, 0.7998128361456282587 ) ) ;
#154935=CARTESIAN_POINT ( 'NONE',  ( -5.912764388891193157, 9.912325863766124456, 0.000000000000000000 ) ) ;
#154937=CARTESIAN_POINT ( 'NONE',  ( 6.441532379824158383, 9.568852638886589546, -1.082531754730548412 ) ) ;
#154943=CARTESIAN_POINT ( 'NONE',  ( -4.085803189671902480, 5.860132702740892263, -1.599625672291271394 ) ) ;
#154950=CARTESIAN_POINT ( 'NONE',  ( -7.119966945832006289, 8.335658187339330283, 1.199719254218452047 ) ) ;
#154952=CARTESIAN_POINT ( 'NONE',  ( 4.780342502845265074, 8.269896785439653897, -0.8296954209953393278 ) ) ;
#154956=CARTESIAN_POINT ( 'NONE',  ( 3.923105346307896202, 5.670318552149568703, -1.599625672291269396 ) ) ;
#154967=CARTESIAN_POINT ( 'NONE',  ( -5.562588163356775972, 9.711712967216715953, 0.7998128361456291469 ) ) ;
#154970=CARTESIAN_POINT ( 'NONE',  ( -3.805626687661477270, 7.453998545664736852, -0.4223333724091842267 ) ) ;
#154980=CARTESIAN_POINT ( 'NONE',  ( 7.506374323821472849, 8.786466794993730289, -1.199719254218452047 ) ) ;
#154989=CARTESIAN_POINT ( 'NONE',  ( 4.570728514692611100, 8.499999999999511502, -0.1921259283747507873 ) ) ;
#154994=CARTESIAN_POINT ( 'NONE',  ( 6.569431593124095414, 6.790062804044275424, 0.3413723397009699734 ) ) ;
#155001=CARTESIAN_POINT ( 'NONE',  ( -5.595925273716217951, 5.773232080116717846, -0.3509683264134528247 ) ) ;
#155017=AXIS2_PLACEMENT_3D ( 'NONE', #132241, #146354, #129101 ) ;
#155023=CARTESIAN_POINT ( 'NONE',  ( -6.617491849531519144, 6.756558277422160863, -0.006230766683231955816 ) ) ;
#155037=CARTESIAN_POINT ( 'NONE',  ( -6.265276382846530545, 6.482112999508623297, 0.000000000000000000 ) ) ;
#155041=CARTESIAN_POINT ( 'NONE',  ( -5.173318132066234476, 8.193232366456022930, -1.199719254218453823 ) ) ;
#155060=CARTESIAN_POINT ( 'NONE',  ( 6.143253000323500856, 10.18122924377050609, -0.7216878364870458196 ) ) ;
#155061=CARTESIAN_POINT ( 'NONE',  ( -4.370663978927087356, 5.060324124126027279, 2.420000000000000373 ) ) ;
#155069=CARTESIAN_POINT ( 'NONE',  ( 5.187768293964614585, 7.852886447769140688, 1.258803494560766678 ) ) ;
#155077=CARTESIAN_POINT ( 'NONE',  ( 7.178115983792402233, 7.339166500704784823, 0.7998128361456281477 ) ) ;
#155083=( BOUNDED_CURVE ( )  B_SPLINE_CURVE ( 2, ( #44384, #138689, #172249, #81135, #146164 ),
 .UNSPECIFIED., .F., .T. ) 
 B_SPLINE_CURVE_WITH_KNOTS ( ( 3, 2, 3 ),
 ( 0.2625000001274112593, 0.2666666666666666630, 0.2750000000000000222 ),
 .UNSPECIFIED. ) 
 CURVE ( )  GEOMETRIC_REPRESENTATION_ITEM ( )  RATIONAL_B_SPLINE_CURVE ( ( 0.9330127018922194093, 0.9330127039406037603, 1.000000000000000000, 0.8660254037844387076, 1.000000000000000000 ) ) 
 REPRESENTATION_ITEM ( '' )  );
#155084=EDGE_CURVE ( 'NONE', #824, #123208, #203652, .T. ) ;
#155089=CARTESIAN_POINT ( 'NONE',  ( -4.468294144155606773, 7.370704380560280100, 1.199719254218452935 ) ) ;
#155091=CARTESIAN_POINT ( 'NONE',  ( 4.115782150200256950, 6.959440387612411349, 1.199719254218452047 ) ) ;
#155093=EDGE_CURVE ( 'NONE', #195055, #198620, #61661, .T. ) ;
#155095=CARTESIAN_POINT ( 'NONE',  ( -5.088052786878465739, 9.158088361325352977, 0.000000000000000000 ) ) ;
#155099=CARTESIAN_POINT ( 'NONE',  ( 5.365994935958575240, 9.482354201918870018, 0.7998128361456341429 ) ) ;
#155105=CARTESIAN_POINT ( 'NONE',  ( -4.662743238902972820, 8.402825839448235357, 0.5650157067484343765 ) ) ;
#155115=CARTESIAN_POINT ( 'NONE',  ( -5.790741006368224753, 5.928488393617260321, 0.7216878364870257245 ) ) ;
#155125=CARTESIAN_POINT ( 'NONE',  ( 3.092668437693027794, 6.622213920701574885, -0.7216878364870338292 ) ) ;
#155129=CARTESIAN_POINT ( 'NONE',  ( -6.074935347375019390, 9.245119117649618801, 1.199719254218452047 ) ) ;
#155168=CARTESIAN_POINT ( 'NONE',  ( -3.851925040058333582, 7.508013290127760087, -0.7216878364870458196 ) ) ;
#155192=CARTESIAN_POINT ( 'NONE',  ( -4.299344108864961989, 6.109263775132799168, -1.443375672974066548 ) ) ;
#155198=CARTESIAN_POINT ( 'NONE',  ( -5.334207092333882017, 5.187939460669764635, 0.7998128361456281477 ) ) ;
#155202=CYLINDRICAL_SURFACE ( 'NONE', #105891, 2.000000000000000000 ) ;
#155206=CARTESIAN_POINT ( 'NONE',  ( -6.994027139803241866, 9.253060644560830994, -1.599625672291271394 ) ) ;
#155208=CARTESIAN_POINT ( 'NONE',  ( 5.763319317650291040, 7.363698819737331647, -1.304181885133362195 ) ) ;
#155212=CARTESIAN_POINT ( 'NONE',  ( 5.903649544107831382, 5.852288987739402870, -0.7998128361456481317 ) ) ;
#155218=CARTESIAN_POINT ( 'NONE',  ( -7.584860592202423035, 7.813701877183096833, -0.7998128361456362523 ) ) ;
#155221=CARTESIAN_POINT ( 'NONE',  ( -6.116136693540540570, 10.14959355252370266, 0.000000000000000000 ) ) ;
#155226=CARTESIAN_POINT ( 'NONE',  ( 3.865483193227626124, 7.523831135491951372, -0.7216878364870338292 ) ) ;
#155227=CARTESIAN_POINT ( 'NONE',  ( -4.285785955251283141, 8.014184357852876417, 0.000000000000000000 ) ) ;
#155231=CARTESIAN_POINT ( 'NONE',  ( -5.957882158562513908, 5.915560371269844353, -0.7998128361456361413 ) ) ;
#155234=CARTESIAN_POINT ( 'NONE',  ( 4.203910148689107729, 7.062256385849379647, -1.199719254218448494 ) ) ;
#155245=CARTESIAN_POINT ( 'NONE',  ( 4.941988244637107286, 8.095350367992509177, 1.064974588601754757 ) ) ;
#155255=CARTESIAN_POINT ( 'NONE',  ( 4.877901405866606588, 8.912911750144889567, 0.7998128361456341429 ) ) ;
#155266=CARTESIAN_POINT ( 'NONE',  ( 5.794989345469916842, 7.230977472937116346, 1.182549002416101835 ) ) ;
#155279=CARTESIAN_POINT ( 'NONE',  ( 6.224601922449876312, 6.434659462379210382, 0.000000000000000000 ) ) ;
#155283=CARTESIAN_POINT ( 'NONE',  ( -7.014364370223741929, 9.276787413384745662, -1.599625672291271394 ) ) ;
#155295=CARTESIAN_POINT ( 'NONE',  ( 5.468734858265785093, 7.473552982767158070, 1.599625672291269396 ) ) ;
#155299=CARTESIAN_POINT ( 'NONE',  ( 4.570507181582611267, 8.346359121906111511, 0.000000000000000000 ) ) ;
#155302=CARTESIAN_POINT ( 'NONE',  ( -5.899206235277530297, 9.896508017883515862, 0.7216878364870267237 ) ) ;
#155304=CARTESIAN_POINT ( 'NONE',  ( 5.090160327287878594, 4.903218234782778850, -0.7998128361456481317 ) ) ;
#155307=CARTESIAN_POINT ( 'NONE',  ( 3.567203813726958828, 6.215469311773181182, 1.082531754730549078 ) ) ;
#155308=CARTESIAN_POINT ( 'NONE',  ( 6.116136693540529912, 10.14959355252369910, 1.530808498934192557E-16 ) ) ;
#155313=CIRCLE ( 'NONE', #37645, 0.08000000000000061229 ) ;
#155314=FACE_OUTER_BOUND ( 'NONE', #166442, .T. ) ;
#155320=CARTESIAN_POINT ( 'NONE',  ( -4.442231607132987925, 5.211633625523774960, -1.199719254218453823 ) ) ;
#155321=CARTESIAN_POINT ( 'NONE',  ( 7.363486825997814123, 7.763358516518489516, 0.000000000000000000 ) ) ;
#155331=CARTESIAN_POINT ( 'NONE',  ( -4.599959256786493533, 8.588645909551377855, 0.000000000000000000 ) ) ;
#155332=CARTESIAN_POINT ( 'NONE',  ( -2.959422669532919326, 6.674686557755516780, 0.7998128361456352531 ) ) ;
#155334=CARTESIAN_POINT ( 'NONE',  ( 5.682275777458846377, 7.722684055159064975, 1.443375672974064550 ) ) ;
#155339=AXIS2_PLACEMENT_3D ( 'NONE', #27363, #30587, #146484 ) ;
#155343=CARTESIAN_POINT ( 'NONE',  ( -6.326802395788107880, 6.950450678040672514, 0.9045734915664763731 ) ) ;
#155347=CARTESIAN_POINT ( 'NONE',  ( -4.820236115778962827, 8.125194398966316456, -0.8510355349711593576 ) ) ;
#155349=CARTESIAN_POINT ( 'NONE',  ( 5.072158865288233009, 7.010880990960010273, 1.443375672974065660 ) ) ;
#155353=CARTESIAN_POINT ( 'NONE',  ( -5.336015975430226099, 8.383046517047350932, -1.199719254218453823 ) ) ;
#155365=CARTESIAN_POINT ( 'NONE',  ( 3.854260808034858155, 7.718664386007802136, -0.7998128361456362523 ) ) ;
#155403=CARTESIAN_POINT ( 'NONE',  ( 5.370438244788902971, 9.279612028980123384, -0.7216878364870458196 ) ) ;
#155408=CARTESIAN_POINT ( 'NONE',  ( 7.309254211098767051, 7.700087132469628948, 0.7216878364870267237 ) ) ;
#155433=CARTESIAN_POINT ( 'NONE',  ( -3.709037541790315640, 6.484905011134099340, -1.199719254218450271 ) ) ;
#155435=CARTESIAN_POINT ( 'NONE',  ( 6.360183458142179447, 6.592837920686898556, -0.7216878364870458196 ) ) ;
#155441=CARTESIAN_POINT ( 'NONE',  ( -4.787964524281469458, 5.614988695530339413, -1.199719254218453823 ) ) ;
#155446=CARTESIAN_POINT ( 'NONE',  ( -7.593975437430151132, 8.032261896522864930, -0.7216878364870338292 ) ) ;
#155450=LINE ( 'NONE', #7033, #185372 ) ;
#155455=CARTESIAN_POINT ( 'NONE',  ( -5.496904935697871863, 5.377753611261092637, 0.7998128361456281477 ) ) ;
#155464=CARTESIAN_POINT ( 'NONE',  ( -7.015401035077384329, 6.062865449010541141, -2.437084766375293921 ) ) ;
#155469=CARTESIAN_POINT ( 'NONE',  ( -3.499413046103020175, 7.096749297179887783, 0.7216878364870338292 ) ) ;
#155470=ORIENTED_EDGE ( 'NONE', *, *, #50541, .T. ) ;
#155471=CARTESIAN_POINT ( 'NONE',  ( -6.251718229232857915, 7.426664367927358512, -1.082531754730549967 ) ) ;
#155473=CARTESIAN_POINT ( 'NONE',  ( 6.235824307642648279, 6.239826211863360506, 0.000000000000000000 ) ) ;
#155475=CARTESIAN_POINT ( 'NONE',  ( -4.782994330570982555, 8.802186828966616972, 0.000000000000000000 ) ) ;
#155476=CARTESIAN_POINT ( 'NONE',  ( -7.228432174741334038, 8.462200954400218578, -1.199719254218452047 ) ) ;
#155496=CARTESIAN_POINT ( 'NONE',  ( 7.876360894896227371, 8.153785563659219804, -0.7998128361456341429 ) ) ;
#155503=( BOUNDED_CURVE ( )  B_SPLINE_CURVE ( 2, ( #159453, #160522, #25181, #24795, #171053, #203529, #121329 ),
 .UNSPECIFIED., .F., .T. ) 
 B_SPLINE_CURVE_WITH_KNOTS ( ( 3, 2, 2, 3 ),
 ( 0.4499999999999995115, 0.4583333333333330373, 0.4666666666666666741, 0.4750000000000001998 ),
 .UNSPECIFIED. ) 
 CURVE ( )  GEOMETRIC_REPRESENTATION_ITEM ( )  RATIONAL_B_SPLINE_CURVE ( ( 1.000000000000007994, 0.8660254037844307140, 1.000000000000000000, 0.8660254037844387076, 1.000000000000000000, 0.8660254037844351549, 1.000000000000003553 ) ) 
 REPRESENTATION_ITEM ( '' )  );
#155525=ADVANCED_FACE ( 'NONE', ( #83407 ), #158244, .T. ) ;
#155529=CARTESIAN_POINT ( 'NONE',  ( -1.850900803405209905, 8.952907405788534945, -0.7749999999999996891 ) ) ;
#155531=CARTESIAN_POINT ( 'NONE',  ( 2.989549312115233004, 6.434947971831853408, -0.5153606499832382726 ) ) ;
#155540=CARTESIAN_POINT ( 'NONE',  ( 5.896870467300973750, 5.844380064798101237, 0.7998128361456352531 ) ) ;
#155543=CARTESIAN_POINT ( 'NONE',  ( -3.156015896931072540, 6.904045323053366268, 0.000000000000000000 ) ) ;
#155557=CARTESIAN_POINT ( 'NONE',  ( 5.499767588998890844, 6.445425604367387429, 1.199719254218451159 ) ) ;
#155563=CARTESIAN_POINT ( 'NONE',  ( -5.725286006720766707, 9.901527117808042178, 0.7998128361456291469 ) ) ;
#155568=CARTESIAN_POINT ( 'NONE',  ( 5.737035277238070385, 6.722237907313067140, -1.199719254218452047 ) ) ;
#155572=CARTESIAN_POINT ( 'NONE',  ( -5.000000000000013323, 11.39843543023555661, -0.7749999999999996891 ) ) ;
#155578=CARTESIAN_POINT ( 'NONE',  ( 6.861835142292143530, 8.138467433163244280, 1.082531754730549967 ) ) ;
#155579=CARTESIAN_POINT ( 'NONE',  ( -5.004368097219957789, 5.011053332944274352, 0.000000000000000000 ) ) ;
#155580=CARTESIAN_POINT ( 'NONE',  ( -5.261446130555064826, 8.296048364692991228, 1.199719254218452935 ) ) ;
#155590=CARTESIAN_POINT ( 'NONE',  ( 4.583538449871731757, 7.505156070562471804, 1.199719254218451159 ) ) ;
#155591=CARTESIAN_POINT ( 'NONE',  ( 4.538947565524982686, 8.517465603079630299, 0.000000000000000000 ) ) ;
#155594=CARTESIAN_POINT ( 'NONE',  ( 5.352436782344940802, 9.466536356036257871, 0.000000000000000000 ) ) ;
#155609=CARTESIAN_POINT ( 'NONE',  ( 5.595231165798738360, 7.497995327707586810, -1.335214257040851615 ) ) ;
#155613=CARTESIAN_POINT ( 'NONE',  ( 5.896870467300973750, 5.844380064798101237, 0.7998128361456352531 ) ) ;
#155617=CARTESIAN_POINT ( 'NONE',  ( 5.761288931164342486, 5.686201605971993978, -0.7998128361456481317 ) ) ;
#155622=CARTESIAN_POINT ( 'NONE',  ( 6.047819040147648373, 9.213483425884394507, 1.199719254218452047 ) ) ;
#155626=CARTESIAN_POINT ( 'NONE',  ( 6.211043768836181478, 7.379210830797944709, 1.082531754730549967 ) ) ;
#155628=CARTESIAN_POINT ( 'NONE',  ( -6.493429226302317225, 6.540365283632955773, 0.7998128361456341429 ) ) ;
#155630=CARTESIAN_POINT ( 'NONE',  ( 7.865138509703455405, 8.348618814175074121, -0.7216878364870317197 ) ) ;
#155641=CARTESIAN_POINT ( 'NONE',  ( -4.659162064951642535, 5.464719159645540003, 1.199719254218452935 ) ) ;
#155649=TOROIDAL_SURFACE ( 'NONE', #210967, 7.374593666277937665, 0.08000000000000000167 ) ;
#155652=CARTESIAN_POINT ( 'NONE',  ( 0.1054570145121071778, 2.614151819895196294, -2.076146791065092145 ) ) ;
#155673=CARTESIAN_POINT ( 'NONE',  ( 4.584065335196271462, 5.481069324884694005, 1.082531754730549078 ) ) ;
#155678=CARTESIAN_POINT ( 'NONE',  ( 5.643937085038755797, 9.806620042512378177, -0.7998128361456481317 ) ) ;
#155680=CARTESIAN_POINT ( 'NONE',  ( 6.003228155800906407, 10.22579295840155744, 0.000000000000000000 ) ) ;
#155692=CARTESIAN_POINT ( 'NONE',  ( -5.529746549527323474, 7.544733289238903851, -1.599625672291271394 ) ) ;
#155695=CARTESIAN_POINT ( 'NONE',  ( 7.010974831598141499, 7.352094523052197239, -0.7216878364870317197 ) ) ;
#155706=CARTESIAN_POINT ( 'NONE',  ( -5.798046968499580345, 6.793418213784815585, 1.199719254218452935 ) ) ;
#155713=CARTESIAN_POINT ( 'NONE',  ( -3.363304624641834106, 6.081549941127532222, -1.199719254218452047 ) ) ;
#155736=CARTESIAN_POINT ( 'NONE',  ( -4.633854640820660009, 8.628190524257904670, -0.7998128361456362523 ) ) ;
#155739=CARTESIAN_POINT ( 'NONE',  ( -3.709037541790315640, 6.484905011134099340, -1.199719254218450271 ) ) ;
#155740=EDGE_LOOP ( 'NONE', ( #38271, #152723, #6188 ) ) ;
#155750=CARTESIAN_POINT ( 'NONE',  ( -4.072997184480262156, 7.271224798513709509, -0.8443910950608760624 ) ) ;
#155751=CARTESIAN_POINT ( 'NONE',  ( 4.529832720297257254, 8.298905583739861314, 0.000000000000000000 ) ) ;
#155761=CARTESIAN_POINT ( 'NONE',  ( -4.318600669050610463, 4.999583595936801572, 2.420000000000000373 ) ) ;
#155764=CARTESIAN_POINT ( 'NONE',  ( -5.010620288702242853, 8.003418215864698482, -1.199719254218453823 ) ) ;
#155765=CARTESIAN_POINT ( 'NONE',  ( 6.132223229334005765, 5.371873414694337434, 2.500000000000000444 ) ) ;
#155773=CARTESIAN_POINT ( 'NONE',  ( -2.428612866367529932E-14, 2.999999999999999112, 2.500000000000000444 ) ) ;
#155779=CARTESIAN_POINT ( 'NONE',  ( -5.865261586769421776, 6.278966368068457093, 0.6541898161073615992 ) ) ;
#155784=CARTESIAN_POINT ( 'NONE',  ( 4.736594563127852098, 6.619389305106191834, -1.599625672291273171 ) ) ;
#155792=CARTESIAN_POINT ( 'NONE',  ( 5.515134625708930649, 9.656350506627580543, 0.000000000000000000 ) ) ;
#155794=CARTESIAN_POINT ( 'NONE',  ( 7.178115983792402233, 7.339166500704784823, 0.7998128361456281477 ) ) ;
#155808=CARTESIAN_POINT ( 'NONE',  ( 6.463930056324285189, 6.765849701160138174, -0.2895399612845122039 ) ) ;
#155810=CARTESIAN_POINT ( 'NONE',  ( 6.211043768836181478, 7.379210830797944709, 1.082531754730549967 ) ) ;
#155820=VERTEX_POINT ( 'NONE', #87370 ) ;
#155827=CARTESIAN_POINT ( 'NONE',  ( -5.926322542504884439, 6.086666852443364029, -0.7216878364870338292 ) ) ;
#155847=CARTESIAN_POINT ( 'NONE',  ( 6.261886844665240481, 8.398896966899865646, 1.599625672291268286 ) ) ;
#155871=B_SPLINE_CURVE_WITH_KNOTS ( 'NONE', 3,
 ( #94528, #196272, #47919, #131329, #114031, #180025, #48963, #199441, #169088, #35887 ),
 .UNSPECIFIED., .F., .F.,
 ( 4, 3, 3, 4 ),
 ( 2.434915676126017810E-15, 3.125147921016584851E-05, 5.470111457697502723E-05, 7.815590336363350394E-05 ),
 .UNSPECIFIED. ) ;
#155888=CARTESIAN_POINT ( 'NONE',  ( 5.397554552016226914, 6.430140077841320689, 1.082531754730549078 ) ) ;
#155899=CARTESIAN_POINT ( 'NONE',  ( -4.340018570150318666, 6.156717313299049366, -1.443375672974066548 ) ) ;
#155905=CARTESIAN_POINT ( 'NONE',  ( 4.760662214969796580, 8.263722922863950160, 0.7838479752697187219 ) ) ;
#155932=CARTESIAN_POINT ( 'NONE',  ( 4.797606254389322089, 6.690569611577942943, 1.599625672291268286 ) ) ;
#155944=CARTESIAN_POINT ( 'NONE',  ( -5.478903473698247595, 8.445785581739666981, -1.082531754730549967 ) ) ;
#155947=CARTESIAN_POINT ( 'NONE',  ( 6.282224075085741433, 8.422623735723785643, 1.599625672291268286 ) ) ;
#155964=CARTESIAN_POINT ( 'NONE',  ( -4.095971805104331231, 5.871996087412059140, 1.443375672974065660 ) ) ;
#155968=CARTESIAN_POINT ( 'NONE',  ( 5.346851039111029991, 6.199209027673978412, 7.500000000000000000 ) ) ;
#155978=EDGE_LOOP ( 'NONE', ( #98384, #32650 ) ) ;
#155994=CARTESIAN_POINT ( 'NONE',  ( -5.582925393777276035, 9.735439736040634173, 0.7998128361456291469 ) ) ;
#155997=CARTESIAN_POINT ( 'NONE',  ( -5.692444392891315097, 7.734547439830227411, -1.599625672291271394 ) ) ;
#156002=CARTESIAN_POINT ( 'NONE',  ( -5.736508391913536897, 9.706693867292189637, 0.7216878364870267237 ) ) ;
#156003=CARTESIAN_POINT ( 'NONE',  ( 7.065207446052794715, 9.336104335185329006, -1.443375672974064550 ) ) ;
#156008=CARTESIAN_POINT ( 'NONE',  ( -2.844178363816758814, 6.540234867753325076, -0.7998128361456481317 ) ) ;
#156014=ORIENTED_EDGE ( 'NONE', *, *, #104484, .T. ) ;
#156017=CARTESIAN_POINT ( 'NONE',  ( -7.014364370223741929, 9.276787413384745662, -1.599625672291271394 ) ) ;
#156019=CARTESIAN_POINT ( 'NONE',  ( 5.273189713885392926, 7.658326211947664497, -1.220946906274408494 ) ) ;
#156022=CARTESIAN_POINT ( 'NONE',  ( 6.343417644181545967, 6.506394916570013898, 2.500000000000000444 ) ) ;
#156024=CARTESIAN_POINT ( 'NONE',  ( 4.543917759235442944, 5.330267469643351852, 1.199719254218452935 ) ) ;
#156045=CARTESIAN_POINT ( 'NONE',  ( 7.842465510862060896, 8.114240948952696542, 0.000000000000000000 ) ) ;
#156062=CARTESIAN_POINT ( 'NONE',  ( 6.589288424369031283, 6.777081280454712697, 0.2339771526987007022 ) ) ;
#156063=CARTESIAN_POINT ( 'NONE',  ( -3.973948422136968084, 7.650373902552835226, -0.7216878364870458196 ) ) ;
#156094=CARTESIAN_POINT ( 'NONE',  ( 7.512626515748109135, 8.897724035528543851, 1.082531754730549967 ) ) ;
#156115=CARTESIAN_POINT ( 'NONE',  ( -6.089547271193396227, 7.133501900260939443, -1.199719254218453823 ) ) ;
#156124=CARTESIAN_POINT ( 'NONE',  ( 5.591005849568446706, 5.791977450266268868, -0.7139200525481930182 ) ) ;
#156131=VERTEX_POINT ( 'NONE', #42914 ) ;
#156133=CARTESIAN_POINT ( 'NONE',  ( 3.400062661977048428, 7.188766548940353829, -1.734723475976807094E-15 ) ) ;
#156135=CARTESIAN_POINT ( 'NONE',  ( 7.824464048418096951, 8.301165276008827476, -0.7216878364870317197 ) ) ;
#156142=CARTESIAN_POINT ( 'NONE',  ( 4.754915986029614849, 8.180161719226850536, 0.7478464228280010673 ) ) ;
#156145=CARTESIAN_POINT ( 'NONE',  ( 5.654245663017247736, 7.339362581565530341, 1.229167601055790815 ) ) ;
#156147=CARTESIAN_POINT ( 'NONE',  ( -3.704603422706345572, 7.358260162494655532, -0.4639270913322328105 ) ) ;
#156164=CARTESIAN_POINT ( 'NONE',  ( -5.666381855868691808, 5.575476684793721383, 0.000000000000000000 ) ) ;
#156166=CARTESIAN_POINT ( 'NONE',  ( 4.064412189046650248, 7.963840997188264659, 0.7998128361456271485 ) ) ;
#156169=CARTESIAN_POINT ( 'NONE',  ( -6.961185525973791144, 7.086080966583015339, 0.7998128361456341429 ) ) ;
#156174=CARTESIAN_POINT ( 'NONE',  ( 5.027041095616958444, 9.086908054853605421, 0.000000000000000000 ) ) ;
#156175=CARTESIAN_POINT ( 'NONE',  ( -7.065207446497166366, 9.336104335703744539, 0.000000000000000000 ) ) ;
#156179=( BOUNDED_CURVE ( )  B_SPLINE_CURVE ( 2, ( #163261, #194675, #112435, #14843, #100377 ),
 .UNSPECIFIED., .F., .T. ) 
 B_SPLINE_CURVE_WITH_KNOTS ( ( 3, 2, 3 ),
 ( 0.5171743412319206312, 0.5250000000000000222, 0.5287935031110296835 ),
 .UNSPECIFIED. ) 
 CURVE ( )  GEOMETRIC_REPRESENTATION_ITEM ( )  RATIONAL_B_SPLINE_CURVE ( ( 0.9846707376464753914, 0.8741872631710951858, 1.000000000000000000, 0.9390120342948788945, 0.9335499976228173180 ) ) 
 REPRESENTATION_ITEM ( '' )  );
#156180=CARTESIAN_POINT ( 'NONE',  ( -4.839158742459761520, 8.201312040681516535, -0.9517655008395020655 ) ) ;
#156189=CARTESIAN_POINT ( 'NONE',  ( -6.102578539482539810, 6.292298848917299736, 0.000000000000000000 ) ) ;
#156199=CARTESIAN_POINT ( 'NONE',  ( 5.750066545971570520, 5.881034856487848295, -0.7216878364870458196 ) ) ;
#156203=CARTESIAN_POINT ( 'NONE',  ( -7.747558435566414659, 8.003516027774422170, -0.7998128361456362523 ) ) ;
#156207=EDGE_CURVE ( 'NONE', #69840, #26075, #70789, .T. ) ;
#156234=ORIENTED_EDGE ( 'NONE', *, *, #61552, .F. ) ;
#156244=CARTESIAN_POINT ( 'NONE',  ( -6.482206841109545259, 6.735198534148810090, 0.7216878364870257245 ) ) ;
#156259=EDGE_CURVE ( 'NONE', #135468, #71711, #56367, .T. ) ;
#156267=CARTESIAN_POINT ( 'NONE',  ( -4.217995187182965289, 6.014356699837137832, 1.443375672974065660 ) ) ;
#156268=CARTESIAN_POINT ( 'NONE',  ( -3.923105346307911745, 5.670318552149568703, -1.599625672291283607 ) ) ;
#156272=CARTESIAN_POINT ( 'NONE',  ( -4.176793841461789114, 7.030620694084159794, -1.199719254218455378 ) ) ;
#156280=CARTESIAN_POINT ( 'NONE',  ( -3.006876207180748217, 6.730049018344652190, -0.7998128361456481317 ) ) ;
#156282=CARTESIAN_POINT ( 'NONE',  ( 6.374094191309353619, 6.920300110170956032, -0.8184029421815092187 ) ) ;
#156286=CARTESIAN_POINT ( 'NONE',  ( 3.366167277942881064, 7.149221934233827014, -0.7998128361456362523 ) ) ;
#156291=CARTESIAN_POINT ( 'NONE',  ( -5.399890319992785237, 9.521898816625391504, 0.7998128361456291469 ) ) ;
#156293=B_SPLINE_CURVE_WITH_KNOTS ( 'NONE', 3,
 ( #95303, #161352, #146183, #63835 ),
 .UNSPECIFIED., .F., .F.,
 ( 4, 4 ),
 ( 0.7146167707638562128, 1.000000000000000000 ),
 .UNSPECIFIED. ) ;
#156295=CARTESIAN_POINT ( 'NONE',  ( -4.767627293860968507, 5.591261926706423857, -1.199719254218453823 ) ) ;
#156301=CARTESIAN_POINT ( 'NONE',  ( 4.706088717274885092, 8.504537580213796133, 0.7216878364870317197 ) ) ;
#156302=CARTESIAN_POINT ( 'NONE',  ( -5.926322542504884439, 6.086666852443364029, -0.7216878364870338292 ) ) ;
#156308=CARTESIAN_POINT ( 'NONE',  ( 2.905190055078214595, 6.611415174225076186, 0.7998128361456271485 ) ) ;
#156315=CARTESIAN_POINT ( 'NONE',  ( 3.811250579217332568, 5.539821323877241355, 1.214306433183764966E-14 ) ) ;
#156320=CARTESIAN_POINT ( 'NONE',  ( 5.950060389077887812, 7.221515259811701171, 1.225279837341096689 ) ) ;
#156330=CARTESIAN_POINT ( 'NONE',  ( 6.886615681098613884, 6.999082814228660077, 0.000000000000000000 ) ) ;
#156341=CARTESIAN_POINT ( 'NONE',  ( 6.491225937077876651, 6.748298437306541331, 0.07656069123261090292 ) ) ;
#156358=CARTESIAN_POINT ( 'NONE',  ( -6.257970421159510188, 9.458660037064859694, 1.199719254218452047 ) ) ;
#156364=CARTESIAN_POINT ( 'NONE',  ( -4.036671995544492297, 7.285761072467114019, 0.7944190476826870073 ) ) ;
#156371=CARTESIAN_POINT ( 'NONE',  ( 7.201315867513990554, 8.430565262634994284, -1.199719254218452047 ) ) ;
#156375=CARTESIAN_POINT ( 'NONE',  ( 4.575498903167257936, 8.352182797088220312, 0.2657046714051370384 ) ) ;
#156378=CARTESIAN_POINT ( 'NONE',  ( -7.878696662872776812, 8.364436659539265406, -0.7216878364870338292 ) ) ;
#156381=CARTESIAN_POINT ( 'NONE',  ( 5.063044020060520900, 4.871582543017558109, 0.7998128361456352531 ) ) ;
#156384=CARTESIAN_POINT ( 'NONE',  ( 3.729901657090938460, 7.365652676665848553, 0.7216878364870257245 ) ) ;
#156396=CARTESIAN_POINT ( 'NONE',  ( -7.946487431385463651, 8.443525889470736345, 0.7216878364870317197 ) ) ;
#156397=CARTESIAN_POINT ( 'NONE',  ( 3.040771591214902259, 6.769593633051179005, -0.7998128361456362523 ) ) ;
#156408=CARTESIAN_POINT ( 'NONE',  ( -5.906512197408906317, 6.919960980845699439, -1.199719254218453823 ) ) ;
#156409=CARTESIAN_POINT ( 'NONE',  ( -3.610214042988883598, 7.433943160120816351, 0.7998128361456352531 ) ) ;
#156411=CARTESIAN_POINT ( 'NONE',  ( 6.333067150914816423, 7.521571443223021625, 1.082531754730549967 ) ) ;
#156424=CARTESIAN_POINT ( 'NONE',  ( -4.733264021794758136, 8.224961065399975624, 0.6825151564062783560 ) ) ;
#156428=CARTESIAN_POINT ( 'NONE',  ( 5.912764389335563919, 6.070849007079172743, -0.7216878364870458196 ) ) ;
#156434=CARTESIAN_POINT ( 'NONE',  ( -6.740338644649361832, 7.892758502626242567, -1.199719254218452047 ) ) ;
#156449=CARTESIAN_POINT ( 'NONE',  ( 4.203910148689107729, 7.062256385849379647, -1.199719254218448494 ) ) ;
#156464=DIRECTION ( 'NONE',  ( -0.7771862570881792331, -0.6292706268317843632, -6.822565806923340619E-15 ) ) ;
#156470=CARTESIAN_POINT ( 'NONE',  ( 5.456087663318581527, 6.086207979321623718, 0.9243867668097293100 ) ) ;
#156486=CARTESIAN_POINT ( 'NONE',  ( 6.373741612200162443, 8.529394195690610303, 1.443375672974065660 ) ) ;
#156491=CARTESIAN_POINT ( 'NONE',  ( 6.116136693096175136, 9.189224337703940648, -1.082531754730548412 ) ) ;
#156516=CARTESIAN_POINT ( 'NONE',  ( -5.490125858891038213, 5.369844688319787451, -0.7998128361456362523 ) ) ;
#156518=CARTESIAN_POINT ( 'NONE',  ( 5.519577934094861860, 6.572500690266394940, 1.082531754730549078 ) ) ;
#156524=CARTESIAN_POINT ( 'NONE',  ( -5.002032328799064231, 4.800402236545811441, -0.7998128361456362523 ) ) ;
#156529=CARTESIAN_POINT ( 'NONE',  ( -7.621091744657483069, 8.063897588288083895, 0.7216878364870317197 ) ) ;
#156538=CARTESIAN_POINT ( 'NONE',  ( -3.772911886352873445, 7.623757310712140800, 0.7998128361456352531 ) ) ;
#156549=CARTESIAN_POINT ( 'NONE',  ( -5.641601317062259646, 5.754492089426966217, -0.7216878364870338292 ) ) ;
#156551=CARTESIAN_POINT ( 'NONE',  ( -6.278834536460198734, 6.497930845391236332, 0.7216878364870257245 ) ) ;
#156552=CARTESIAN_POINT ( 'NONE',  ( 6.574778147984297938, 6.635272358928617997, -0.7998128361456481317 ) ) ;
#156553=CARTESIAN_POINT ( 'NONE',  ( -6.330731382938325602, 6.350551133041632212, 0.7998128361456281477 ) ) ;
#156557=DIRECTION ( 'NONE',  ( -0.6095094443598249034, 0.000000000000000000, -0.7927788072572181655 ) ) ;
#156574=CARTESIAN_POINT ( 'NONE',  ( 7.364013710877980401, 8.620379413226322285, -1.199719254218452047 ) ) ;
#156600=ADVANCED_FACE ( 'NONE', ( #79651 ), #94967, .T. ) ;
#156612=CARTESIAN_POINT ( 'NONE',  ( 5.091969210384201361, 8.098325291160362482, 1.199719254218452047 ) ) ;
#156615=DIRECTION ( 'NONE',  ( 0.000000000000000000, 0.000000000000000000, 1.000000000000000000 ) ) ;
#156618=CARTESIAN_POINT ( 'NONE',  ( -6.007671464186866928, 8.102312356341712984, 1.443375672974058777 ) ) ;
#156626=CARTESIAN_POINT ( 'NONE',  ( 3.147653791585693028, 8.920000000000001705, 2.499999999999999556 ) ) ;
#156630=CARTESIAN_POINT ( 'NONE',  ( 7.075376061485196821, 9.347967719856493218, 1.599625672291268286 ) ) ;
#156631=CARTESIAN_POINT ( 'NONE',  ( 3.528865121306874464, 7.339036084825155015, -0.7998128361456362523 ) ) ;
#156637=CARTESIAN_POINT ( 'NONE',  ( -7.533490631048818109, 8.818102486758951031, -1.199719254218452047 ) ) ;
#156642=CARTESIAN_POINT ( 'NONE',  ( 4.549643065837591038, 7.465611455855944101, -1.199719254218452047 ) ) ;
#156651=CARTESIAN_POINT ( 'NONE',  ( 6.536439455564155843, 8.719208346281938304, 1.443375672974065660 ) ) ;
#156652=CARTESIAN_POINT ( 'NONE',  ( -4.502716413514313842, 5.386162249589033557, -1.082531754730549967 ) ) ;
#156653=CARTESIAN_POINT ( 'NONE',  ( -6.180537922983287302, 8.303989891604203422, -1.599625672291271394 ) ) ;
#156665=CARTESIAN_POINT ( 'NONE',  ( 7.354371980770088690, 7.544798497178720531, 0.000000000000000000 ) ) ;
#156666=CARTESIAN_POINT ( 'NONE',  ( 5.529746549527311039, 7.544733289238903851, -1.599625672291281386 ) ) ;
#156667=CARTESIAN_POINT ( 'NONE',  ( 7.713663051532233972, 7.963971413067895355, -0.7998128361456341429 ) ) ;
#156670=CARTESIAN_POINT ( 'NONE',  ( 6.200875153403774043, 8.327716660428123419, -1.599625672291283607 ) ) ;
#156691=CARTESIAN_POINT ( 'NONE',  ( 5.248941747146098180, 6.152795455539095570, -1.199719254218452047 ) ) ;
#156693=SPHERICAL_SURFACE ( 'NONE', #153825, 0.08000000000000000167 ) ;
#156695=CARTESIAN_POINT ( 'NONE',  ( 3.400062661977048428, 7.188766548940353829, -1.734723475976807094E-15 ) ) ;
#156700=CARTESIAN_POINT ( 'NONE',  ( 4.543917759235442944, 5.330267469643351852, 1.199719254218452935 ) ) ;
#156704=EDGE_CURVE ( 'NONE', #160443, #185175, #211768, .T. ) ;
#156705=CARTESIAN_POINT ( 'NONE',  ( 5.072158865288233898, 7.971250205261355859, 1.082531754730549078 ) ) ;
#156707=CARTESIAN_POINT ( 'NONE',  ( -6.967964602780620353, 7.093989889524320525, 0.000000000000000000 ) ) ;
#156709=CARTESIAN_POINT ( 'NONE',  ( 5.713835393516482952, 5.630839145382857680, 0.7998128361456352531 ) ) ;
#156719=CARTESIAN_POINT ( 'NONE',  ( -2.986538976760251263, 6.706322249520737522, -0.7998128361456481317 ) ) ;
#156724=VERTEX_POINT ( 'NONE', #127432 ) ;
#156751=CARTESIAN_POINT ( 'NONE',  ( 3.851925040058331806, 5.587274861525073355, -1.443375672974066548 ) ) ;
#156752=EDGE_LOOP ( 'NONE', ( #134599, #68276, #178297, #211255 ) ) ;
#156756=CARTESIAN_POINT ( 'NONE',  ( 6.994027139803230320, 9.253060644560830994, -1.599625672291267398 ) ) ;
#156759=CARTESIAN_POINT ( 'NONE',  ( 6.502017186205484300, 9.743381262951846367, -1.199719254218452047 ) ) ;
#156768=AXIS2_PLACEMENT_3D ( 'NONE', #207880, #125660, #191622 ) ;
#156772=CARTESIAN_POINT ( 'NONE',  ( -6.784929528996132220, 6.880448970109080520, 0.000000000000000000 ) ) ;
#156774=CARTESIAN_POINT ( 'NONE',  ( 6.658462837642789012, 9.821938173008357253, 1.082531754730549078 ) ) ;
#156784=CARTESIAN_POINT ( 'NONE',  ( -5.971440312176176768, 5.931378217152456500, 0.000000000000000000 ) ) ;
#156793=CARTESIAN_POINT ( 'NONE',  ( -3.135678666510573365, 6.880318554229450712, 0.000000000000000000 ) ) ;
#156813=CARTESIAN_POINT ( 'NONE',  ( -5.794130544993808307, 7.853181283949808744, 1.599625672291263179 ) ) ;
#156815=CARTESIAN_POINT ( 'NONE',  ( -5.015590482412729756, 4.816220082428420923, 0.000000000000000000 ) ) ;
#156840=CARTESIAN_POINT ( 'NONE',  ( -6.967964602780620353, 7.093989889524320525, 0.000000000000000000 ) ) ;
#156841=CARTESIAN_POINT ( 'NONE',  ( 2.734094378161750605, 2.930569811600769459, 2.453211638583554954 ) ) ;
#156856=CARTESIAN_POINT ( 'NONE',  ( -4.339333680283728789, 7.686373885219706992, 0.7730735768287697596 ) ) ;
#156860=CARTESIAN_POINT ( 'NONE',  ( 3.790386463472274148, 6.579812086429759788, 1.199719254218452047 ) ) ;
#156867=CARTESIAN_POINT ( 'NONE',  ( 7.713663051532233972, 7.963971413067895355, -0.7998128361456341429 ) ) ;
#156869=CARTESIAN_POINT ( 'NONE',  ( 4.993145711582793744, 9.047363440147082159, -0.7998128361456481317 ) ) ;
#156882=CARTESIAN_POINT ( 'NONE',  ( 6.157602363183391603, 6.969851231138187941, -0.9158007892692658913 ) ) ;
#156884=CARTESIAN_POINT ( 'NONE',  ( 4.082413651490639062, 7.776916670132135501, 0.000000000000000000 ) ) ;
#156891=CARTESIAN_POINT ( 'NONE',  ( -3.298376509874564988, 7.070132704820777825, 0.000000000000000000 ) ) ;
#156899=CIRCLE ( 'NONE', #153481, 0.07999999999999984901 ) ;
#156902=CARTESIAN_POINT ( 'NONE',  ( -7.227905289416814760, 7.605180057173966723, -0.7216878364870338292 ) ) ;
#156906=CARTESIAN_POINT ( 'NONE',  ( 6.318982112420993502, 9.529840343536603697, -1.199719254218452047 ) ) ;
#156924=CARTESIAN_POINT ( 'NONE',  ( 5.234329823327693809, 8.264412672927770487, 1.199719254218451159 ) ) ;
#156941=CARTESIAN_POINT ( 'NONE',  ( -6.099189001301292379, 8.209082816308541197, 1.599625672291263179 ) ) ;
#156963=CARTESIAN_POINT ( 'NONE',  ( 6.387299765813869712, 6.624473612970537495, 0.000000000000000000 ) ) ;
#156975=CARTESIAN_POINT ( 'NONE',  ( -4.448483799059637533, 7.243629294661272588, 1.082531754730549967 ) ) ;
#156980=FACE_OUTER_BOUND ( 'NONE', #55917, .T. ) ;
#157008=CARTESIAN_POINT ( 'NONE',  ( 3.932747076415766596, 6.745899468197171345, 1.199719254218451159 ) ) ;
#157020=CARTESIAN_POINT ( 'NONE',  ( -6.699137298928187434, 8.909022496873262753, 1.443375672974064550 ) ) ;
#157022=CARTESIAN_POINT ( 'NONE',  ( 6.502017186205484300, 9.743381262951846367, -1.199719254218452047 ) ) ;
#157039=CARTESIAN_POINT ( 'NONE',  ( -4.841670253855968831, 4.821239182352949904, 0.000000000000000000 ) ) ;
#157040=CARTESIAN_POINT ( 'NONE',  ( 4.850610703097786747, 8.175460293138137047, -1.048226046837946512 ) ) ;
#157042=DIRECTION ( 'NONE',  ( 0.000000000000000000, 0.000000000000000000, 1.000000000000000000 ) ) ;
#157043=CARTESIAN_POINT ( 'NONE',  ( 3.894326384698054255, 7.335661066667313435, -0.8064731704051804062 ) ) ;
#157071=CARTESIAN_POINT ( 'NONE',  ( -7.014364370223741929, 9.276787413384745662, -1.599625672291271394 ) ) ;
#157074=CARTESIAN_POINT ( 'NONE',  ( -5.152980901645737077, 8.169505597632108262, -1.199719254218453823 ) ) ;
#157079=CARTESIAN_POINT ( 'NONE',  ( -5.248414861821563804, 9.137251415518218067, 0.7216878364870267237 ) ) ;
#157085=CARTESIAN_POINT ( 'NONE',  ( -6.563028877466991595, 9.814561569423593923, 1.199719254218452935 ) ) ;
#157093=CARTESIAN_POINT ( 'NONE',  ( -7.442499979258930587, 7.647614495415686164, -0.7998128361456362523 ) ) ;
#157095=CARTESIAN_POINT ( 'NONE',  ( 5.583942420111207561, 7.395222456726187943, -1.242479836444350783 ) ) ;
#157099=CARTESIAN_POINT ( 'NONE',  ( 5.996449078994045223, 10.21788403546024782, 0.7998128361456331437 ) ) ;
#157122=CARTESIAN_POINT ( 'NONE',  ( 5.806634928402749196, 9.996434193103704402, -0.7998128361456481317 ) ) ;
#157134=CARTESIAN_POINT ( 'NONE',  ( 0.2847049989426675976, 3.404688149418213960, 1.981472963502264317 ) ) ;
#157137=CARTESIAN_POINT ( 'NONE',  ( -2.974142338115852269, 6.685868392857900133, 0.1038623869373533903 ) ) ;
#157138=CARTESIAN_POINT ( 'NONE',  ( 6.400241882075590638, 6.902609158730609096, 0.7749192096189911894 ) ) ;
#157139=CARTESIAN_POINT ( 'NONE',  ( -4.109529958273628658, 7.808552361378938045, 0.7216878364870338292 ) ) ;
#157164=ORIENTED_EDGE ( 'NONE', *, *, #34519, .F. ) ;
#157168=CARTESIAN_POINT ( 'NONE',  ( 3.444653546323793947, 6.176457016423196222, 1.199719254218451159 ) ) ;
#157182=CARTESIAN_POINT ( 'NONE',  ( -5.444481204339554736, 8.509589284108232121, 1.199719254218454489 ) ) ;
#157189=CARTESIAN_POINT ( 'NONE',  ( 5.602074566136501232, 5.729665287594564838, 0.6253354971682704155 ) ) ;
#157197=CARTESIAN_POINT ( 'NONE',  ( 5.357406976055401948, 6.279338222599979424, 1.199719254218452935 ) ) ;
#157207=CARTESIAN_POINT ( 'NONE',  ( 4.816680029521997142, 8.110538062004499338, 0.8573938582591574820 ) ) ;
#157209=CARTESIAN_POINT ( 'NONE',  ( 6.017777097630443883, 7.067734144800174256, 1.048426327298467742 ) ) ;
#157230=ORIENTED_EDGE ( 'NONE', *, *, #187873, .F. ) ;
#157232=CARTESIAN_POINT ( 'NONE',  ( -6.154475385960665790, 6.144919136567696505, 0.000000000000000000 ) ) ;
#157234=CARTESIAN_POINT ( 'NONE',  ( 5.761288931164342486, 5.686201605971993978, -0.7998128361456481317 ) ) ;
#157237=CARTESIAN_POINT ( 'NONE',  ( -6.123442655227560927, 7.173046514967467147, 1.199719254218452047 ) ) ;
#157245=CARTESIAN_POINT ( 'NONE',  ( -4.992018142146231519, 8.041046192835899831, -1.132135330316372590 ) ) ;
#157253=CARTESIAN_POINT ( 'NONE',  ( -5.926322542504884439, 6.086666852443364029, -0.7216878364870338292 ) ) ;
#157264=CARTESIAN_POINT ( 'NONE',  ( 5.017926250833595780, 7.907978821730911712, -1.082531754730548412 ) ) ;
#157268=EDGE_CURVE ( 'NONE', #111968, #117552, #202465, .T. ) ;
#157269=CARTESIAN_POINT ( 'NONE',  ( -6.180537922983287302, 8.303989891604203422, -1.599625672291271394 ) ) ;
#157271=VERTEX_POINT ( 'NONE', #20551 ) ;
#157279=CARTESIAN_POINT ( 'NONE',  ( -3.689227196694346400, 6.357829925235092716, -1.082531754730546636 ) ) ;
#157284=CARTESIAN_POINT ( 'NONE',  ( 3.223806664999388172, 6.983134552466421674, -0.7998128361456362523 ) ) ;
#157287=CARTESIAN_POINT ( 'NONE',  ( 5.984665970559388093, 7.172686677051047788, -1.260417782354812832 ) ) ;
#157309=CARTESIAN_POINT ( 'NONE',  ( -4.828112100242279325, 8.646898193675708555, -0.7216878364870338292 ) ) ;
#157334=CARTESIAN_POINT ( 'NONE',  ( -7.930593509350902792, 8.217056947189661287, -0.7998128361456362523 ) ) ;
#157337=CARTESIAN_POINT ( 'NONE',  ( -4.004454267989906668, 5.765225627445230927, 1.599625672291270506 ) ) ;
#157342=CARTESIAN_POINT ( 'NONE',  ( -4.797606254389363833, 6.690569611577942943, 1.599625672291263179 ) ) ;
#157351=CARTESIAN_POINT ( 'NONE',  ( -4.679499295372141709, 5.488445928469455559, 1.199719254218452935 ) ) ;
#157353=CARTESIAN_POINT ( 'NONE',  ( 6.184762415132515123, 7.051423785172313607, -1.050594063207562545 ) ) ;
#157357=CARTESIAN_POINT ( 'NONE',  ( 3.705121118284530279, 7.544668081299086282, -1.734723475976807094E-15 ) ) ;
#157361=CARTESIAN_POINT ( 'NONE',  ( -5.015590482412729756, 4.816220082428420923, 0.000000000000000000 ) ) ;
#157365=CARTESIAN_POINT ( 'NONE',  ( -5.320648938720212051, 5.172121614787156929, 0.000000000000000000 ) ) ;
#157371=CARTESIAN_POINT ( 'NONE',  ( 6.170369307550831017, 6.371388078330353366, 0.7216878364870328300 ) ) ;
#157372=CARTESIAN_POINT ( 'NONE',  ( -4.245111494410291897, 7.006361605903701495, 1.082531754730549967 ) ) ;
#157375=CARTESIAN_POINT ( 'NONE',  ( -4.960304097753355457, 6.880383762169266504, 1.599625672291263401 ) ) ;
#157379=CARTESIAN_POINT ( 'NONE',  ( 4.686278372178935392, 5.496354851410763409, 1.199719254218452047 ) ) ;
#157380=VERTEX_POINT ( 'NONE', #171079 ) ;
#157389=CARTESIAN_POINT ( 'NONE',  ( 5.337069745634900997, 6.255611453776062980, 1.199719254218452047 ) ) ;
#157390=CARTESIAN_POINT ( 'NONE',  ( 4.774898309648160755, 8.276035162536045320, 0.8191430224755236189 ) ) ;
#157396=( BOUNDED_CURVE ( )  B_SPLINE_CURVE ( 2, ( #157189, #206980, #90062, #22880, #156124 ),
 .UNSPECIFIED., .F., .T. ) 
 B_SPLINE_CURVE_WITH_KNOTS ( ( 3, 2, 3 ),
 ( 0.2462631119352014508, 0.2500000000000000000, 0.2543051829449332057 ),
 .UNSPECIFIED. ) 
 CURVE ( )  GEOMETRIC_REPRESENTATION_ITEM ( )  RATIONAL_B_SPLINE_CURVE ( ( 0.9337253982215369952, 0.9399222316499036278, 1.000000000000000000, 0.9307857823982145229, 0.9330867333962934440 ) ) 
 REPRESENTATION_ITEM ( '' )  );
#157401=CARTESIAN_POINT ( 'NONE',  ( 5.794130544993763898, 7.853181283949808744, 1.599625672291269396 ) ) ;
#157412=CARTESIAN_POINT ( 'NONE',  ( 4.990887655837901171, 7.926359819171765686, 1.063311220390166234 ) ) ;
#157419=CARTESIAN_POINT ( 'NONE',  ( 7.354371980770088690, 7.544798497178720531, 0.000000000000000000 ) ) ;
#157423=CARTESIAN_POINT ( 'NONE',  ( -4.733264021794758136, 8.224961065399975624, 0.6825151564062783560 ) ) ;
#157431=CARTESIAN_POINT ( 'NONE',  ( -7.442499979258930587, 7.647614495415686164, -0.7998128361456362523 ) ) ;
#157444=CARTESIAN_POINT ( 'NONE',  ( 7.364013710877980401, 8.620379413226322285, -1.199719254218452047 ) ) ;
#157453=CARTESIAN_POINT ( 'NONE',  ( 5.740951700743842423, 5.662474837148078421, -0.7998128361456481317 ) ) ;
#157456=CARTESIAN_POINT ( 'NONE',  ( 4.760321331729593375, 5.686701320840210627, -1.082531754730548412 ) ) ;
#157470=CARTESIAN_POINT ( 'NONE',  ( -4.604929450496978660, 5.401447776115099408, -1.199719254218453823 ) ) ;
#157471=CARTESIAN_POINT ( 'NONE',  ( 5.994113311017540191, 9.046863725278862844, -1.082531754730548412 ) ) ;
#157478=VERTEX_POINT ( 'NONE', #42176 ) ;
#157484=CARTESIAN_POINT ( 'NONE',  ( -4.610654757099099221, 7.536791762327691657, 1.199719254218452935 ) ) ;
#157485=CARTESIAN_POINT ( 'NONE',  ( -4.176793841461789114, 7.030620694084159794, -1.199719254218455378 ) ) ;
#157487=CARTESIAN_POINT ( 'NONE',  ( 6.441532379824158383, 9.568852638886589546, -1.082531754730548412 ) ) ;
#157494=CARTESIAN_POINT ( 'NONE',  ( -6.966220764712169000, 6.002124920821316323, -2.420000000000000373 ) ) ;
#157498=CARTESIAN_POINT ( 'NONE',  ( -5.575295409310188965, 7.417394932307940003, -1.244639187630245170 ) ) ;
#157503=CARTESIAN_POINT ( 'NONE',  ( 3.594320121398666856, 7.207474218358159490, -1.734723475976807094E-15 ) ) ;
#157506=CARTESIAN_POINT ( 'NONE',  ( -7.442499979258930587, 7.647614495415686164, -0.7998128361456362523 ) ) ;
#157513=DIRECTION ( 'NONE',  ( 0.6507913734559658270, -0.7592566023652989049, 0.000000000000000000 ) ) ;
#157521=CARTESIAN_POINT ( 'NONE',  ( 5.337069745634900997, 6.255611453776062980, 1.199719254218452047 ) ) ;
#157532=CARTESIAN_POINT ( 'NONE',  ( -5.346851039111035320, 6.199209027673978412, 2.420000000000001261 ) ) ;
#157540=CARTESIAN_POINT ( 'NONE',  ( 5.484430959185961463, 6.043327615839654499, 0.8208683321978844649 ) ) ;
#157556=EDGE_CURVE ( 'NONE', #158833, #179029, #198662, .T. ) ;
#157557=CARTESIAN_POINT ( 'NONE',  ( 5.546694241766559230, 9.485244025454063532, 0.000000000000000000 ) ) ;
#157563=CARTESIAN_POINT ( 'NONE',  ( 6.577113915960825175, 8.766661883411348555, -1.443375672974078761 ) ) ;
#157588=CARTESIAN_POINT ( 'NONE',  ( -3.793249116773374396, 7.647484079536056356, 0.7998128361456352531 ) ) ;
#157590=CARTESIAN_POINT ( 'NONE',  ( 4.706088717274885092, 8.504537580213796133, 0.7216878364870317197 ) ) ;
#157596=CARTESIAN_POINT ( 'NONE',  ( -5.652823702255029836, 5.559658838911111900, -0.7998128361456362523 ) ) ;
#157601=CARTESIAN_POINT ( 'NONE',  ( -4.065465959251405081, 5.836405933916976707, -1.599625672291271394 ) ) ;
#157607=CARTESIAN_POINT ( 'NONE',  ( -3.284818356260900796, 7.054314858938165678, 0.7998128361456352531 ) ) ;
#157616=CARTESIAN_POINT ( 'NONE',  ( -2.972980823146582186, 6.690504403638126263, 0.000000000000000000 ) ) ;
#157619=CARTESIAN_POINT ( 'NONE',  ( -5.966997003790240228, 6.134120390609613338, -0.7216878364870338292 ) ) ;
#157620=CARTESIAN_POINT ( 'NONE',  ( -4.448483798615272100, 8.203998508444197313, 0.000000000000000000 ) ) ;
#157621=CARTESIAN_POINT ( 'NONE',  ( 6.038177310039780643, 8.137902509836795417, -1.599625672291283607 ) ) ;
#157622=CARTESIAN_POINT ( 'NONE',  ( -5.119085517611572378, 8.129960982925583224, 1.199719254218452935 ) ) ;
#157642=CARTESIAN_POINT ( 'NONE',  ( 6.013923656113508542, 9.173938811177871244, -1.199719254218452047 ) ) ;
#157671=CARTESIAN_POINT ( 'NONE',  ( -1.865749732055444365, 8.973930515401084662, -0.7749999999999996891 ) ) ;
#157679=CARTESIAN_POINT ( 'NONE',  ( 5.254667053748194760, 8.288139441751686931, 1.199719254218452047 ) ) ;
#157685=CARTESIAN_POINT ( 'NONE',  ( -6.577113915960849155, 6.845923454808663600, -0.7216878364870338292 ) ) ;
#157697=CARTESIAN_POINT ( 'NONE',  ( 5.110497557708379546, 4.926945003606695295, -0.7998128361456481317 ) ) ;
#157698=CARTESIAN_POINT ( 'NONE',  ( 5.879395890181562834, 6.888325289080478697, -1.199719254218452047 ) ) ;
#157710=CARTESIAN_POINT ( 'NONE',  ( 6.222266154028957885, 6.224008365980749247, 0.7998128361456352531 ) ) ;
#157724=CARTESIAN_POINT ( 'NONE',  ( 5.885648082108177803, 9.880690172519326353, 0.7216878364870317197 ) ) ;
#157725=CARTESIAN_POINT ( 'NONE',  ( -3.512971199716682591, 7.112567143062499930, 0.000000000000000000 ) ) ;
#157726=CARTESIAN_POINT ( 'NONE',  ( -6.129167961829681488, 9.308390501180058507, -1.199719254218452047 ) ) ;
#157734=DIRECTION ( 'NONE',  ( 0.000000000000000000, 0.000000000000000000, 1.000000000000000000 ) ) ;
#157737=CARTESIAN_POINT ( 'NONE',  ( 5.692444392891300886, 7.734547439830227411, -1.599625672291281386 ) ) ;
#157738=CARTESIAN_POINT ( 'NONE',  ( 4.864343252252968597, 8.897093904262280972, 0.000000000000000000 ) ) ;
#157741=CARTESIAN_POINT ( 'NONE',  ( 4.868786560638896255, 5.813244087901094481, 1.082531754730549078 ) ) ;
#157758=CARTESIAN_POINT ( 'NONE',  ( 5.032011289327418702, 5.899709921417326974, 1.199719254218452935 ) ) ;
#157761=CARTESIAN_POINT ( 'NONE',  ( 4.441177836928239309, 7.339068688795062911, 1.199719254218452047 ) ) ;
#157765=CARTESIAN_POINT ( 'NONE',  ( 4.580100504995564314, 8.463430921191662293, -0.5085073561186970181 ) ) ;
#157766=CARTESIAN_POINT ( 'NONE',  ( 6.505933609711257226, 8.683618192786854095, -1.599625672291281386 ) ) ;
#157769=B_SPLINE_CURVE_WITH_KNOTS ( 'NONE', 3,
 ( #6681, #107477, #74911, #120533 ),
 .UNSPECIFIED., .F., .F.,
 ( 4, 4 ),
 ( 1.788112030672750545E-18, 0.0006551727224232820924 ),
 .UNSPECIFIED. ) ;
#157773=CARTESIAN_POINT ( 'NONE',  ( 4.746763178560241769, 8.551991118380046331, 0.7216878364870328300 ) ) ;
#157775=CARTESIAN_POINT ( 'NONE',  ( -5.550083779947821760, 7.568460058062819407, -1.599625672291271394 ) ) ;
#157776=CARTESIAN_POINT ( 'NONE',  ( 4.529305835417093640, 7.441884687032027657, -1.199719254218450271 ) ) ;
#157783=CARTESIAN_POINT ( 'NONE',  ( -4.244597871138700462, 7.508646359881505639, -0.8219154050654879917 ) ) ;
#157788=CARTESIAN_POINT ( 'NONE',  ( -4.122561227007127016, 6.967349310553715647, 1.199719254218452935 ) ) ;
#157817=CARTESIAN_POINT ( 'NONE',  ( 3.282482588284323821, 6.843663763058119187, 0.7216878364870257245 ) ) ;
#157823=CARTESIAN_POINT ( 'NONE',  ( 6.210516883511641772, 9.403297576475722508, 1.199719254218452047 ) ) ;
#157824=CARTESIAN_POINT ( 'NONE',  ( 6.393551957296131683, 9.616838495890963401, 1.199719254218452047 ) ) ;
#157836=CARTESIAN_POINT ( 'NONE',  ( -6.961185525973791144, 7.086080966583015339, 0.7998128361456341429 ) ) ;
#157838=CARTESIAN_POINT ( 'NONE',  ( 7.499068361690118145, 7.921536974826172361, -0.7216878364870317197 ) ) ;
#157849=CARTESIAN_POINT ( 'NONE',  ( -5.147255595043616516, 6.034161611419515125, 1.199719254218452935 ) ) ;
#157859=ORIENTED_EDGE ( 'NONE', *, *, #73531, .T. ) ;
#157861=CARTESIAN_POINT ( 'NONE',  ( -4.821859908315634158, 5.654533310236863564, 1.199719254218452935 ) ) ;
#157885=CARTESIAN_POINT ( 'NONE',  ( -5.824109505522200081, 8.952488968821326054, -1.199719254218452047 ) ) ;
#157887=CARTESIAN_POINT ( 'NONE',  ( -3.332271893908731464, 7.109677319527304640, -0.7998128361456481317 ) ) ;
#157895=CARTESIAN_POINT ( 'NONE',  ( -6.297925439369929101, 6.970297724909739756, -0.9421744322617598977 ) ) ;
#157910=CARTESIAN_POINT ( 'NONE',  ( -5.030313335769911021, 7.996221790701172338, -1.198669363888727357 ) ) ;
#157911=CARTESIAN_POINT ( 'NONE',  ( -5.550083779947821760, 7.568460058062819407, -1.599625672291271394 ) ) ;
#157937=CARTESIAN_POINT ( 'NONE',  ( 7.309781096423290769, 8.557108029695882578, 1.199719254218452935 ) ) ;
#157939=CARTESIAN_POINT ( 'NONE',  ( 5.006703865196457492, 9.063181286029688977, 0.000000000000000000 ) ) ;
#157949=CARTESIAN_POINT ( 'NONE',  ( 6.483881968795301098, 6.767627347268279969, 0.2992266196225811803 ) ) ;
#157953=CARTESIAN_POINT ( 'NONE',  ( 6.266472554743693912, 6.895788939045927712, 0.7740814723603481884 ) ) ;
#157955=CARTESIAN_POINT ( 'NONE',  ( 6.916067756746836714, 8.201738816693689316, -1.082531754730548412 ) ) ;
#157963=CARTESIAN_POINT ( 'NONE',  ( -4.502189528189771472, 7.410248995266807803, -1.199719254218453823 ) ) ;
#157973=CARTESIAN_POINT ( 'NONE',  ( -6.753369912938502750, 7.051555451282599307, 0.000000000000000000 ) ) ;
#157984=CARTESIAN_POINT ( 'NONE',  ( -3.902768115887413014, 5.646591783325653147, -1.599625672291283607 ) ) ;
#157993=CARTESIAN_POINT ( 'NONE',  ( 5.110497557708379546, 4.926945003606695295, -0.7998128361456481317 ) ) ;
#158004=CIRCLE ( 'NONE', #50833, 0.8300000000000008482 ) ;
#158012=CARTESIAN_POINT ( 'NONE',  ( -5.413448473606448985, 9.537716662508005427, 0.000000000000000000 ) ) ;
#158014=DIRECTION ( 'NONE',  ( 0.000000000000000000, 0.000000000000000000, -1.000000000000000000 ) ) ;
#158016=CARTESIAN_POINT ( 'NONE',  ( -6.488192154978348114, 6.766396236290696642, 0.1981293719705672085 ) ) ;
#158031=DIRECTION ( 'NONE',  ( -1.000000000000000000, 0.000000000000000000, 0.000000000000000000 ) ) ;
#158032=CARTESIAN_POINT ( 'NONE',  ( 5.804299160426222848, 7.865044668620976509, -1.443375672974078761 ) ) ;
#158044=CARTESIAN_POINT ( 'NONE',  ( -4.828112100242291760, 6.726159765073026264, -1.443375672974066548 ) ) ;
#158075=CARTESIAN_POINT ( 'NONE',  ( 3.393283585170187688, 7.180857625999046867, 0.7998128361456271485 ) ) ;
#158086=CARTESIAN_POINT ( 'NONE',  ( -6.373741612200205076, 8.529394195690610303, 1.443375672974064550 ) ) ;
#158089=CARTESIAN_POINT ( 'NONE',  ( 3.675669042636310557, 6.342012078834061484, -1.082531754730549967 ) ) ;
#158106=CARTESIAN_POINT ( 'NONE',  ( -3.851925040058337579, 6.547644075826416277, -1.082531754730546636 ) ) ;
#158107=CARTESIAN_POINT ( 'NONE',  ( 4.689424523294686509, 8.358602041046323095, -0.7454045323363467368 ) ) ;
#158136=CARTESIAN_POINT ( 'NONE',  ( -7.095713291905736853, 9.371694488680407886, 1.599625672291269396 ) ) ;
#158139=CARTESIAN_POINT ( 'NONE',  ( -6.123442655227560927, 7.173046514967467147, 1.199719254218452047 ) ) ;
#158140=CARTESIAN_POINT ( 'NONE',  ( -5.601338601481473667, 5.735503837863156207, 0.2797457239998907275 ) ) ;
#158142=ORIENTED_EDGE ( 'NONE', *, *, #123715, .T. ) ;
#158144=CARTESIAN_POINT ( 'NONE',  ( -7.715998819508785189, 8.174622508947939181, -0.7216878364870338292 ) ) ;
#158150=CARTESIAN_POINT ( 'NONE',  ( -6.064239847062411926, 10.29697326487330500, 0.000000000000000000 ) ) ;
#158155=ORIENTED_EDGE ( 'NONE', *, *, #105692, .F. ) ;
#158161=CARTESIAN_POINT ( 'NONE',  ( 5.694759483343039719, 7.307619849039811655, -1.219011658351103478 ) ) ;
#158165=CARTESIAN_POINT ( 'NONE',  ( 4.441177836928239309, 7.339068688795062911, 1.199719254218452047 ) ) ;
#158170=VERTEX_POINT ( 'NONE', #142893 ) ;
#158171=DIRECTION ( 'NONE',  ( -0.6507913734559640506, -0.7592566023653003482, 0.000000000000000000 ) ) ;
#158189=CARTESIAN_POINT ( 'NONE',  ( 5.508355548902068577, 9.648441583686274470, 0.7998128361456331437 ) ) ;
#158204=CARTESIAN_POINT ( 'NONE',  ( -3.231779075379149546, 6.036511184309971689, -0.9899555337401846344 ) ) ;
#158205=CARTESIAN_POINT ( 'NONE',  ( 6.493754380866193721, 6.839952184459461293, 0.5864284347954504817 ) ) ;
#158206=CARTESIAN_POINT ( 'NONE',  ( -4.787437638956939523, 5.718337012605431369, -1.082531754730549967 ) ) ;
#158233=CARTESIAN_POINT ( 'NONE',  ( 2.905190055078214595, 6.611415174225076186, 0.7998128361456271485 ) ) ;
#158244=( BOUNDED_SURFACE ( )  B_SPLINE_SURFACE ( 1, 2, ( 
 ( #133271, #199279, #18402, #134337, #127201, #50921, #183044, #179866, #15204, #213398, #150569, #200342, #118118, #193168, #184103, #35723, #101799, #47757, #31490, #97566, #163623, #20531, #123481, #119175, #53041, #105016, #72478, #5321, #137514, #69268, #120255, #139660, #103944, #102869, #122410, #107194, #152680, #23734, #19466, #185160, #36785, #168927, #85542, #203531, #86613, #106118, #70333, #41087, #151632, #21573, #4263, #136450, #7476, #22653, #171056, #202467, #201403, #3198, #87679, #38933, #169986, #55185, #186232, #54120, #154821, #37865, #205680, #88765, #153752, #71402, #135382, #121331, #138578, #187307, #6406, #204601, #56253, #188368, #189444, #40008, #172141, #89839, #155888, #73558, #57317, #44277, #24798, #191558, #77819, #161215, #45343, #76747, #75696, #176402, #174289, #177468, #25864, #28008, #190495, #78875, #193699, #94106, #11744, #12802, #140740, #43222, #95166, #143940, #144998, #93037, #141810, #160147, #90901, #109339, #110398, #59441, #8554, #206752, #159079, #60500, #156963, #29082, #175349, #61574, #207813, #26929, #74633, #125598, #111462, #58382, #10676, #128786, #173219, #142868, #209936, #62626, #208870, #126660, #124538, #46404, #194767, #42153, #108268, #192625, #211003, #127742, #91974, #158032, #9620, #146051, #34392, #99411, #98342, #81021, #100464, #166539, #30143, #97292, #162282, #163350, #179597, #18127, #84216, #195843, #17060, #178533, #212065, #134075, #50651, #200083, #82076, #49585, #181699, #79948, #13870, #199006, #47484, #63703, #147109, #148169, #129860, #164407, #112520, #1870, #150304, #32276, #15991, #214171, #14926, #182774, #213134, #64765, #165465, #96232, #113594, #114657, #65797, #115709, #130907, #67930, #131945, #31218, #196899, #197956, #48538, #180651, #33329, #133006, #83140, #149218, #793, #116777, #66861, #87430, #187046, #89581, #103685, #201144, #138321, #35459, #117855, #86355, #72214, #167606, #70075, #7215, #51732, #20271, #88506, #155630, #136189, #152426, #151369, #139392, #73289, #19204, #183847, #4005, #101537, #37604, #168667 ),
 ( #202207, #153498, #53861, #36525, #184901, #119994, #2938, #85283, #69010, #185971, #102612, #169734, #21323, #135127, #52782, #5068, #118921, #71143, #137260, #203280, #54927, #121079, #204337, #39745, #38678, #104757, #154568, #170806, #22397, #6144, #55995, #122146, #188114, #105850, #171877, #23473, #75445, #143695, #205425, #59187, #141558, #206496, #94919, #90648, #24540, #76501, #44029, #191305, #109083, #40829, #91725, #111215, #207565, #74384, #93856, #78632, #124286, #209687, #57063, #156709, #8299, #140485, #123227, #175098, #125342, #58127, #208620, #190245, #61331, #41903, #60254, #108014, #177217, #11501, #126411, #110147, #193461, #172961, #9374, #127490, #176160, #45105, #42973, #174040, #192373, #189192, #26685, #142612, #157776, #106938, #25613, #92787, #158832, #10429, #28831, #27760, #159894, #77572, #160968, #12558, #165218, #194518, #144757, #113352, #16809, #14688, #129615, #80784, #97054, #112280, #115469, #98115, #146872, #195602, #49350, #181461, #62388, #211824, #46166, #63461, #79704, #33091, #99165, #95988, #164166, #128553, #178296, #82894, #197708, #210768, #32029, #147920, #213936, #145819, #47237, #29903, #179357, #30979, #212894, #15752, #163108, #81836, #162040, #13631, #64526, #130671, #196659, #48300, #114411, #180411, #65557, #131703, #110848, #211467, #25258, #126048, #159533, #60967, #10072, #177930, #143326, #45809, #161686, #209320, #124988, #75085, #43675, #144403, #194162, #9010, #127122, #128201, #111929, #11131, #44742, #13281, #175801, #29544, #192012, #59897, #157419, #193093, #190947, #95636, #42611, #176855, #141198, #79354, #210404, #28468, #94560, #145472, #91358, #142252, #123929, #160602, #189897, #109793, #92432, #12205, #41539, #208264, #78276, #76148, #173682, #207209, #27393, #77208, #107652, #58833, #93493, #62046, #26320, #108720, #174746, #158472, #83605, #179002, #81486, #18599, #63101, #31682, #99869, #167007, #147563, #97758, #162755, #65208, #96706, #199473, #50053, #48998, #163816, #51115, #117240, #195241, #47952, #112990, #114067, #130318, #183240 ) ),
 .UNSPECIFIED., .F., .F., .T. ) 
 B_SPLINE_SURFACE_WITH_KNOTS ( ( 2, 2 ),
 ( 3, 2, 2, 2, 2, 2, 2, 2, 2, 2, 2, 2, 2, 2, 2, 2, 2, 2, 2, 2, 2, 2, 2, 2, 2, 2, 2, 2, 2, 2, 2, 2, 2, 2, 2, 2, 2, 2, 2, 2, 2, 2, 2, 2, 2, 2, 2, 2, 2, 2, 2, 2, 2, 2, 2, 2, 2, 2, 2, 2, 2, 2, 2, 2, 2, 2, 2, 2, 2, 2, 2, 2, 2, 2, 2, 2, 2, 2, 2, 2, 2, 2, 2, 2, 2, 2, 2, 2, 2, 2, 2, 2, 2, 2, 2, 2, 2, 2, 2, 2, 2, 2, 2, 2, 2, 2, 2, 2, 2, 2, 2, 2, 2, 2, 2, 2, 2, 2, 2, 2, 3 ),
 ( 0.000000000000000000, 1.000000000000000000 ),
 ( 0.000000000000000000, 0.008333333333333333218, 0.01666666666666666644, 0.02500000000000000139, 0.03333333333333333287, 0.04166666666666666435, 0.05000000000000000278, 0.05833333333333333426, 0.06666666666666666574, 0.07499999999999999722, 0.08333333333333332871, 0.09166666666666666019, 0.1000000000000000056, 0.1083333333333333370, 0.1166666666666666685, 0.1250000000000000000, 0.1333333333333333315, 0.1416666666666666630, 0.1499999999999999944, 0.1583333333333333259, 0.1666666666666666574, 0.1749999999999999889, 0.1833333333333333204, 0.1916666666666666796, 0.2000000000000000111, 0.2083333333333333426, 0.2166666666666666741, 0.2250000000000000056, 0.2333333333333333370, 0.2416666666666666685, 0.2500000000000000000, 0.2583333333333333592, 0.2666666666666666630, 0.2750000000000000222, 0.2833333333333333259, 0.2916666666666666852, 0.2999999999999999889, 0.3083333333333333481, 0.3166666666666666519, 0.3250000000000000111, 0.3333333333333333148, 0.3416666666666666741, 0.3499999999999999778, 0.3583333333333333370, 0.3666666666666666408, 0.3750000000000000000, 0.3833333333333333592, 0.3916666666666666630, 0.4000000000000000222, 0.4083333333333333259, 0.4166666666666666852, 0.4249999999999999889, 0.4333333333333333481, 0.4416666666666666519, 0.4500000000000000111, 0.4583333333333333148, 0.4666666666666666741, 0.4749999999999999778, 0.4833333333333333370, 0.4916666666666666408, 0.5000000000000000000, 0.5083333333333333037, 0.5166666666666667185, 0.5250000000000000222, 0.5333333333333333259, 0.5416666666666666297, 0.5500000000000000444, 0.5583333333333333481, 0.5666666666666666519, 0.5749999999999999556, 0.5833333333333333703, 0.5916666666666666741, 0.5999999999999999778, 0.6083333333333332815, 0.6166666666666666963, 0.6250000000000000000, 0.6333333333333333037, 0.6416666666666667185, 0.6500000000000000222, 0.6583333333333333259, 0.6666666666666666297, 0.6750000000000000444, 0.6833333333333333481, 0.6916666666666666519, 0.6999999999999999556, 0.7083333333333333703, 0.7166666666666666741, 0.7249999999999999778, 0.7333333333333332815, 0.7416666666666666963, 0.7500000000000000000, 0.7583333333333333037, 0.7666666666666667185, 0.7750000000000000222, 0.7833333333333333259, 0.7916666666666666297, 0.8000000000000000444, 0.8083333333333333481, 0.8166666666666666519, 0.8249999999999999556, 0.8333333333333333703, 0.8416666666666666741, 0.8499999999999999778, 0.8583333333333332815, 0.8666666666666666963, 0.8750000000000000000, 0.8833333333333333037, 0.8916666666666667185, 0.9000000000000000222, 0.9083333333333333259, 0.9166666666666666297, 0.9250000000000000444, 0.9333333333333333481, 0.9416666666666666519, 0.9499999999999999556, 0.9583333333333333703, 0.9666666666666666741, 0.9749999999999999778, 0.9833333333333332815, 0.9916666666666666963, 1.000000000000000000 ),
 .UNSPECIFIED. ) 
 GEOMETRIC_REPRESENTATION_ITEM ( )  RATIONAL_B_SPLINE_SURFACE ( (
 ( 1.000000000000000000, 0.8660254037844387076, 1.000000000000000000, 0.8660254037844387076, 1.000000000000000000, 0.8660254037844387076, 1.000000000000000000, 0.8660254037844387076, 1.000000000000000000, 0.8660254037844387076, 1.000000000000000000, 0.8660254037844387076, 1.000000000000000000, 0.8660254037844387076, 1.000000000000000000, 0.8660254037844387076, 1.000000000000000000, 0.8660254037844387076, 1.000000000000000000, 0.8660254037844387076, 1.000000000000000000, 0.8660254037844387076, 1.000000000000000000, 0.8660254037844387076, 1.000000000000000000, 0.8660254037844387076, 1.000000000000000000, 0.8660254037844387076, 1.000000000000000000, 0.8660254037844387076, 1.000000000000000000, 0.8660254037844387076, 1.000000000000000000, 0.8660254037844387076, 1.000000000000000000, 0.8660254037844387076, 1.000000000000000000, 0.8660254037844387076, 1.000000000000000000, 0.8660254037844387076, 1.000000000000000000, 0.8660254037844387076, 1.000000000000000000, 0.8660254037844387076, 1.000000000000000000, 0.8660254037844387076, 1.000000000000000000, 0.8660254037844387076, 1.000000000000000000, 0.8660254037844387076, 1.000000000000000000, 0.8660254037844387076, 1.000000000000000000, 0.8660254037844387076, 1.000000000000000000, 0.8660254037844387076, 1.000000000000000000, 0.8660254037844387076, 1.000000000000000000, 0.8660254037844387076, 1.000000000000000000, 0.8660254037844387076, 1.000000000000000000, 0.8660254037844387076, 1.000000000000000000, 0.8660254037844387076, 1.000000000000000000, 0.8660254037844387076, 1.000000000000000000, 0.8660254037844387076, 1.000000000000000000, 0.8660254037844387076, 1.000000000000000000, 0.8660254037844387076, 1.000000000000000000, 0.8660254037844387076, 1.000000000000000000, 0.8660254037844387076, 1.000000000000000000, 0.8660254037844387076, 1.000000000000000000, 0.8660254037844387076, 1.000000000000000000, 0.8660254037844387076, 1.000000000000000000, 0.8660254037844387076, 1.000000000000000000, 0.8660254037844387076, 1.000000000000000000, 0.8660254037844387076, 1.000000000000000000, 0.8660254037844387076, 1.000000000000000000, 0.8660254037844387076, 1.000000000000000000, 0.8660254037844387076, 1.000000000000000000, 0.8660254037844387076, 1.000000000000000000, 0.8660254037844387076, 1.000000000000000000, 0.8660254037844387076, 1.000000000000000000, 0.8660254037844387076, 1.000000000000000000, 0.8660254037844387076, 1.000000000000000000, 0.8660254037844387076, 1.000000000000000000, 0.8660254037844387076, 1.000000000000000000, 0.8660254037844387076, 1.000000000000000000, 0.8660254037844387076, 1.000000000000000000, 0.8660254037844387076, 1.000000000000000000, 0.8660254037844387076, 1.000000000000000000, 0.8660254037844387076, 1.000000000000000000, 0.8660254037844387076, 1.000000000000000000, 0.8660254037844387076, 1.000000000000000000, 0.8660254037844387076, 1.000000000000000000, 0.8660254037844387076, 1.000000000000000000, 0.8660254037844387076, 1.000000000000000000, 0.8660254037844387076, 1.000000000000000000, 0.8660254037844387076, 1.000000000000000000, 0.8660254037844387076, 1.000000000000000000, 0.8660254037844387076, 1.000000000000000000, 0.8660254037844387076, 1.000000000000000000, 0.8660254037844387076, 1.000000000000000000, 0.8660254037844387076, 1.000000000000000000, 0.8660254037844387076, 1.000000000000000000, 0.8660254037844387076, 1.000000000000000000, 0.8660254037844387076, 1.000000000000000000, 0.8660254037844387076, 1.000000000000000000, 0.8660254037844387076, 1.000000000000000000, 0.8660254037844387076, 1.000000000000000000, 0.8660254037844387076, 1.000000000000000000, 0.8660254037844387076, 1.000000000000000000, 0.8660254037844387076, 1.000000000000000000, 0.8660254037844387076, 1.000000000000000000, 0.8660254037844387076, 1.000000000000000000, 0.8660254037844387076, 1.000000000000000000, 0.8660254037844387076, 1.000000000000000000, 0.8660254037844387076, 1.000000000000000000, 0.8660254037844387076, 1.000000000000000000, 0.8660254037844387076, 1.000000000000000000, 0.8660254037844387076, 1.000000000000000000, 0.8660254037844387076, 1.000000000000000000, 0.8660254037844387076, 1.000000000000000000, 0.8660254037844387076, 1.000000000000000000, 0.8660254037844387076, 1.000000000000000000, 0.8660254037844387076, 1.000000000000000000, 0.8660254037844387076, 1.000000000000000000, 0.8660254037844387076, 1.000000000000000000, 0.8660254037844387076, 1.000000000000000000, 0.8660254037844387076, 1.000000000000000000, 0.8660254037844387076, 1.000000000000000000, 0.8660254037844387076, 1.000000000000000000, 0.8660254037844387076, 1.000000000000000000, 0.8660254037844387076, 1.000000000000000000, 0.8660254037844387076, 1.000000000000000000, 0.8660254037844387076, 1.000000000000000000, 0.8660254037844387076, 1.000000000000000000, 0.8660254037844387076, 1.000000000000000000, 0.8660254037844387076, 1.000000000000000000, 0.8660254037844387076, 1.000000000000000000, 0.8660254037844387076, 1.000000000000000000, 0.8660254037844387076, 1.000000000000000000, 0.8660254037844387076, 1.000000000000000000, 0.8660254037844387076, 1.000000000000000000, 0.8660254037844387076, 1.000000000000000000, 0.8660254037844387076, 1.000000000000000000, 0.8660254037844387076, 1.000000000000000000, 0.8660254037844387076, 1.000000000000000000, 0.8660254037844387076, 1.000000000000000000, 0.8660254037844387076, 1.000000000000000000, 0.8660254037844387076, 1.000000000000000000, 0.8660254037844387076, 1.000000000000000000),
 ( 1.000000000000000000, 0.8660254037844387076, 1.000000000000000000, 0.8660254037844387076, 1.000000000000000000, 0.8660254037844387076, 1.000000000000000000, 0.8660254037844387076, 1.000000000000000000, 0.8660254037844387076, 1.000000000000000000, 0.8660254037844387076, 1.000000000000000000, 0.8660254037844387076, 1.000000000000000000, 0.8660254037844387076, 1.000000000000000000, 0.8660254037844387076, 1.000000000000000000, 0.8660254037844387076, 1.000000000000000000, 0.8660254037844387076, 1.000000000000000000, 0.8660254037844387076, 1.000000000000000000, 0.8660254037844387076, 1.000000000000000000, 0.8660254037844387076, 1.000000000000000000, 0.8660254037844387076, 1.000000000000000000, 0.8660254037844387076, 1.000000000000000000, 0.8660254037844387076, 1.000000000000000000, 0.8660254037844387076, 1.000000000000000000, 0.8660254037844387076, 1.000000000000000000, 0.8660254037844387076, 1.000000000000000000, 0.8660254037844387076, 1.000000000000000000, 0.8660254037844387076, 1.000000000000000000, 0.8660254037844387076, 1.000000000000000000, 0.8660254037844387076, 1.000000000000000000, 0.8660254037844387076, 1.000000000000000000, 0.8660254037844387076, 1.000000000000000000, 0.8660254037844387076, 1.000000000000000000, 0.8660254037844387076, 1.000000000000000000, 0.8660254037844387076, 1.000000000000000000, 0.8660254037844387076, 1.000000000000000000, 0.8660254037844387076, 1.000000000000000000, 0.8660254037844387076, 1.000000000000000000, 0.8660254037844387076, 1.000000000000000000, 0.8660254037844387076, 1.000000000000000000, 0.8660254037844387076, 1.000000000000000000, 0.8660254037844387076, 1.000000000000000000, 0.8660254037844387076, 1.000000000000000000, 0.8660254037844387076, 1.000000000000000000, 0.8660254037844387076, 1.000000000000000000, 0.8660254037844387076, 1.000000000000000000, 0.8660254037844387076, 1.000000000000000000, 0.8660254037844387076, 1.000000000000000000, 0.8660254037844387076, 1.000000000000000000, 0.8660254037844387076, 1.000000000000000000, 0.8660254037844387076, 1.000000000000000000, 0.8660254037844387076, 1.000000000000000000, 0.8660254037844387076, 1.000000000000000000, 0.8660254037844387076, 1.000000000000000000, 0.8660254037844387076, 1.000000000000000000, 0.8660254037844387076, 1.000000000000000000, 0.8660254037844387076, 1.000000000000000000, 0.8660254037844387076, 1.000000000000000000, 0.8660254037844387076, 1.000000000000000000, 0.8660254037844387076, 1.000000000000000000, 0.8660254037844387076, 1.000000000000000000, 0.8660254037844387076, 1.000000000000000000, 0.8660254037844387076, 1.000000000000000000, 0.8660254037844387076, 1.000000000000000000, 0.8660254037844387076, 1.000000000000000000, 0.8660254037844387076, 1.000000000000000000, 0.8660254037844387076, 1.000000000000000000, 0.8660254037844387076, 1.000000000000000000, 0.8660254037844387076, 1.000000000000000000, 0.8660254037844387076, 1.000000000000000000, 0.8660254037844387076, 1.000000000000000000, 0.8660254037844387076, 1.000000000000000000, 0.8660254037844387076, 1.000000000000000000, 0.8660254037844387076, 1.000000000000000000, 0.8660254037844387076, 1.000000000000000000, 0.8660254037844387076, 1.000000000000000000, 0.8660254037844387076, 1.000000000000000000, 0.8660254037844387076, 1.000000000000000000, 0.8660254037844387076, 1.000000000000000000, 0.8660254037844387076, 1.000000000000000000, 0.8660254037844387076, 1.000000000000000000, 0.8660254037844387076, 1.000000000000000000, 0.8660254037844387076, 1.000000000000000000, 0.8660254037844387076, 1.000000000000000000, 0.8660254037844387076, 1.000000000000000000, 0.8660254037844387076, 1.000000000000000000, 0.8660254037844387076, 1.000000000000000000, 0.8660254037844387076, 1.000000000000000000, 0.8660254037844387076, 1.000000000000000000, 0.8660254037844387076, 1.000000000000000000, 0.8660254037844387076, 1.000000000000000000, 0.8660254037844387076, 1.000000000000000000, 0.8660254037844387076, 1.000000000000000000, 0.8660254037844387076, 1.000000000000000000, 0.8660254037844387076, 1.000000000000000000, 0.8660254037844387076, 1.000000000000000000, 0.8660254037844387076, 1.000000000000000000, 0.8660254037844387076, 1.000000000000000000, 0.8660254037844387076, 1.000000000000000000, 0.8660254037844387076, 1.000000000000000000, 0.8660254037844387076, 1.000000000000000000, 0.8660254037844387076, 1.000000000000000000, 0.8660254037844387076, 1.000000000000000000, 0.8660254037844387076, 1.000000000000000000, 0.8660254037844387076, 1.000000000000000000, 0.8660254037844387076, 1.000000000000000000, 0.8660254037844387076, 1.000000000000000000, 0.8660254037844387076, 1.000000000000000000, 0.8660254037844387076, 1.000000000000000000, 0.8660254037844387076, 1.000000000000000000, 0.8660254037844387076, 1.000000000000000000, 0.8660254037844387076, 1.000000000000000000, 0.8660254037844387076, 1.000000000000000000, 0.8660254037844387076, 1.000000000000000000, 0.8660254037844387076, 1.000000000000000000, 0.8660254037844387076, 1.000000000000000000, 0.8660254037844387076, 1.000000000000000000, 0.8660254037844387076, 1.000000000000000000, 0.8660254037844387076, 1.000000000000000000, 0.8660254037844387076, 1.000000000000000000, 0.8660254037844387076, 1.000000000000000000, 0.8660254037844387076, 1.000000000000000000, 0.8660254037844387076, 1.000000000000000000, 0.8660254037844387076, 1.000000000000000000, 0.8660254037844387076, 1.000000000000000000, 0.8660254037844387076, 1.000000000000000000) ) ) 
 REPRESENTATION_ITEM ( '' )  SURFACE ( )  );
#158247=CIRCLE ( 'NONE', #138033, 0.08000000000000020983 ) ;
#158255=CARTESIAN_POINT ( 'NONE',  ( -6.967964602780620353, 7.093989889524320525, 0.000000000000000000 ) ) ;
#158269=CARTESIAN_POINT ( 'NONE',  ( 5.248941747146098180, 6.152795455539095570, -1.199719254218452047 ) ) ;
#158277=DIRECTION ( 'NONE',  ( -0.6292706268317891372, -0.7771862570881751253, 0.000000000000000000 ) ) ;
#158279=CARTESIAN_POINT ( 'NONE',  ( 4.826264338009964128, 8.099924789650724932, 0.8724150771263041726 ) ) ;
#158280=CARTESIAN_POINT ( 'NONE',  ( 4.968759571299464994, 8.067260998001806627, 1.096838584164006924 ) ) ;
#158281=CARTESIAN_POINT ( 'NONE',  ( -3.707465945607718805, 7.355851012256872323, 0.5743249234583160945 ) ) ;
#158298=CARTESIAN_POINT ( 'NONE',  ( -4.793689830883590020, 7.750332681742931662, 1.199719254218452935 ) ) ;
#158300=CARTESIAN_POINT ( 'NONE',  ( 3.576318658954677598, 7.394398545414291313, 0.7998128361456281477 ) ) ;
#158304=CARTESIAN_POINT ( 'NONE',  ( -5.152980901645737077, 8.169505597632108262, -1.199719254218453823 ) ) ;
#158307=CARTESIAN_POINT ( 'NONE',  ( 5.691390622686558487, 9.861982503101517139, 0.7998128361456341429 ) ) ;
#158313=CARTESIAN_POINT ( 'NONE',  ( -4.600441534204600558, 8.479163753367195966, -0.2584006677722027745 ) ) ;
#158330=CARTESIAN_POINT ( 'NONE',  ( 3.933273961740286317, 7.602920365423422311, 0.7216878364870257245 ) ) ;
#158333=CARTESIAN_POINT ( 'NONE',  ( -5.399890319992785237, 9.521898816625391504, 0.7998128361456291469 ) ) ;
#158342=CARTESIAN_POINT ( 'NONE',  ( -3.024877669624710386, 6.543124691288523920, 0.000000000000000000 ) ) ;
#158347=CARTESIAN_POINT ( 'NONE',  ( 5.923986774528332333, 5.876015756563318426, -0.7998128361456481317 ) ) ;
#158376=ORIENTED_EDGE ( 'NONE', *, *, #115282, .F. ) ;
#158392=CARTESIAN_POINT ( 'NONE',  ( -4.516274566683622815, 5.401980094953223066, 1.082531754730549078 ) ) ;
#158398=CARTESIAN_POINT ( 'NONE',  ( -4.716257332707368910, 6.595662536282280719, -1.599625672291271394 ) ) ;
#158406=CARTESIAN_POINT ( 'NONE',  ( -4.462568837553487100, 5.235360394347691404, -1.199719254218453823 ) ) ;
#158407=CARTESIAN_POINT ( 'NONE',  ( 5.461903044330952639, 7.609029316319980474, -1.335476589331906494 ) ) ;
#158411=CARTESIAN_POINT ( 'NONE',  ( 4.960304097753311936, 6.880383762169266504, 1.599625672291268286 ) ) ;
#158416=CARTESIAN_POINT ( 'NONE',  ( -3.492107083971660586, 6.231819477012331632, 1.199719254218452935 ) ) ;
#158422=CARTESIAN_POINT ( 'NONE',  ( -5.255720823952942489, 6.160704378480398979, -1.199719254218453823 ) ) ;
#158426=CARTESIAN_POINT ( 'NONE',  ( 6.021229617800532452, 6.197391773621639288, 0.000000000000000000 ) ) ;
#158427=CARTESIAN_POINT ( 'NONE',  ( -5.546694241322218666, 8.524874810634301525, 1.082531754730550855 ) ) ;
#158435=CARTESIAN_POINT ( 'NONE',  ( 5.065906673361608270, 5.939254536123854677, -1.199719254218450271 ) ) ;
#158443=FILL_AREA_STYLE_COLOUR ( '', #107007 ) ;
#158465=CARTESIAN_POINT ( 'NONE',  ( 4.604167169973131912, 8.362045362587558373, -0.1994984680026238300 ) ) ;
#158472=CARTESIAN_POINT ( 'NONE',  ( 7.828907357248368726, 8.098423103070084395, 0.7998128361456281477 ) ) ;
#158477=CARTESIAN_POINT ( 'NONE',  ( -4.900660301121059881, 8.037431844279481652, -0.9627648694432132670 ) ) ;
#158486=CARTESIAN_POINT ( 'NONE',  ( -6.933015448541747006, 9.181880338089085214, 1.599625672291269396 ) ) ;
#158498=CARTESIAN_POINT ( 'NONE',  ( 6.821687566331318564, 7.987665577921906568, 1.199719254218452935 ) ) ;
#158507=CARTESIAN_POINT ( 'NONE',  ( 3.067887898442204442, 6.801229324816399746, 0.7998128361456271485 ) ) ;
#158510=CARTESIAN_POINT ( 'NONE',  ( 5.600926855776875435, 7.627776979863398310, -1.443375672974078761 ) ) ;
#158525=CARTESIAN_POINT ( 'NONE',  ( -5.307090785106547415, 5.156303768904543894, -0.7998128361456362523 ) ) ;
#158526=CARTESIAN_POINT ( 'NONE',  ( 6.373741612200160667, 9.489763409991955001, 1.082531754730549078 ) ) ;
#158532=ORIENTED_EDGE ( 'NONE', *, *, #137043, .F. ) ;
#158538=CARTESIAN_POINT ( 'NONE',  ( -5.773793314573309132, 7.829454515125894964, 1.599625672291263179 ) ) ;
#158539=CARTESIAN_POINT ( 'NONE',  ( -5.971440312176176768, 5.931378217152456500, 0.000000000000000000 ) ) ;
#158541=CARTESIAN_POINT ( 'NONE',  ( 6.821160681006788629, 8.091013894996997635, 1.082531754730549967 ) ) ;
#158544=CARTESIAN_POINT ( 'NONE',  ( 2.905190055078214595, 6.611415174225076186, 0.7998128361456271485 ) ) ;
#158547=DIRECTION ( 'NONE',  ( 1.000000000000000000, 0.000000000000000000, 0.000000000000000000 ) ) ;
#158553=CARTESIAN_POINT ( 'NONE',  ( -5.056216892478136771, 7.878110338051091510, -1.109312559570382550 ) ) ;
#158554=CARTESIAN_POINT ( 'NONE',  ( -7.015401035077384329, 6.062865449010541141, -2.437084766375293921 ) ) ;
#158558=CARTESIAN_POINT ( 'NONE',  ( 4.082413651490639062, 7.776916670132135501, 0.000000000000000000 ) ) ;
#158563=CARTESIAN_POINT ( 'NONE',  ( -5.108390017298964914, 9.181815130149269422, 0.000000000000000000 ) ) ;
#158566=TOROIDAL_SURFACE ( 'NONE', #99815, 0.4800000000000000933, 0.08000000000000000167 ) ;
#158578=CARTESIAN_POINT ( 'NONE',  ( 6.261886844665240481, 8.398896966899865646, 1.599625672291268286 ) ) ;
#158615=CARTESIAN_POINT ( 'NONE',  ( 7.078765600110826561, 8.391552967285011988, -1.082531754730548412 ) ) ;
#158621=CARTESIAN_POINT ( 'NONE',  ( 7.471952054462754234, 8.850270497362297206, 1.082531754730549078 ) ) ;
#158622=CARTESIAN_POINT ( 'NONE',  ( -3.059665831784952651E-14, 3.479999999999999538, 2.000000000000000000 ) ) ;
#158644=CARTESIAN_POINT ( 'NONE',  ( -5.679940009482361774, 5.591294530676332641, 0.7998128361456281477 ) ) ;
#158646=CARTESIAN_POINT ( 'NONE',  ( 5.573810548549551491, 6.635772073796838200, -1.082531754730548412 ) ) ;
#158651=CARTESIAN_POINT ( 'NONE',  ( -6.168033539574333979, 6.160736982450306876, 0.7998128361456281477 ) ) ;
#158657=CARTESIAN_POINT ( 'NONE',  ( -4.014095998097799267, 6.840806543492835345, -1.199719254218450271 ) ) ;
#158664=CARTESIAN_POINT ( 'NONE',  ( -3.637330350216213759, 7.465578851886037093, -0.7998128361456481317 ) ) ;
#158673=CARTESIAN_POINT ( 'NONE',  ( -3.851398154733808088, 6.650992392901508232, -1.199719254218450271 ) ) ;
#158676=CARTESIAN_POINT ( 'NONE',  ( -4.963693636378939011, 8.805076652501815815, 0.7216878364870267237 ) ) ;
#158677=CARTESIAN_POINT ( 'NONE',  ( -5.980555156959541208, 7.110307450275150210, 1.082531754730549078 ) ) ;
#158678=CARTESIAN_POINT ( 'NONE',  ( 4.701645408888975197, 8.707279753670952971, 0.000000000000000000 ) ) ;
#158679=CARTESIAN_POINT ( 'NONE',  ( -6.038177310039794854, 8.137902509836795417, -1.599625672291271394 ) ) ;
#158698=CARTESIAN_POINT ( 'NONE',  ( 7.700104897918568447, 7.948153567185284096, 0.000000000000000000 ) ) ;
#158718=CARTESIAN_POINT ( 'NONE',  ( 4.595652554671352696, 8.489339133230261680, -0.03962354257190832396 ) ) ;
#158733=CARTESIAN_POINT ( 'NONE',  ( 6.886615681098613884, 6.999082814228660077, 0.000000000000000000 ) ) ;
#158736=CARTESIAN_POINT ( 'NONE',  ( -4.248501033035892327, 6.049946853332221153, -1.599625672291271394 ) ) ;
#158739=CARTESIAN_POINT ( 'NONE',  ( -7.715998819508785189, 8.174622508947939181, -0.7216878364870338292 ) ) ;
#158750=CARTESIAN_POINT ( 'NONE',  ( 6.749980374757213575, 8.968339418673846097, 1.599625672291268286 ) ) ;
#158751=CARTESIAN_POINT ( 'NONE',  ( 4.505052181490820651, 8.477920988373101707, -0.7998128361456381397 ) ) ;
#158766=CARTESIAN_POINT ( 'NONE',  ( 5.712781623311797397, 7.758274208654143855, -1.599625672291283607 ) ) ;
#158769=EDGE_CURVE ( 'NONE', #49308, #139590, #16993, .T. ) ;
#158776=CARTESIAN_POINT ( 'NONE',  ( 7.024532985656128936, 9.288650798055913427, 1.443375672974065660 ) ) ;
#158777=CARTESIAN_POINT ( 'NONE',  ( -4.502716413514296079, 8.267269892493059658, -0.7216878364870338292 ) ) ;
#158778=CARTESIAN_POINT ( 'NONE',  ( -5.641074431737709283, 8.738948049406083385, -1.199719254218452047 ) ) ;
#158790=CARTESIAN_POINT ( 'NONE',  ( 4.355912491740495440, 8.303924683664389406, 0.000000000000000000 ) ) ;
#158791=CARTESIAN_POINT ( 'NONE',  ( 5.189738938980948291, 9.276722205444929870, 0.000000000000000000 ) ) ;
#158794=CARTESIAN_POINT ( 'NONE',  ( 4.136646265500957043, 5.919449624541475607, -1.443375672974068769 ) ) ;
#158812=DIRECTION ( 'NONE',  ( 1.000000000000000000, 0.000000000000000000, 0.000000000000000000 ) ) ;
#158815=CARTESIAN_POINT ( 'NONE',  ( 3.736153849017632922, 6.516540702899320081, -1.199719254218453823 ) ) ;
#158817=FACE_OUTER_BOUND ( 'NONE', #13908, .T. ) ;
#158819=CARTESIAN_POINT ( 'NONE',  ( 5.037736595929563244, 8.035053907629919223, -1.199719254218452047 ) ) ;
#158825=CARTESIAN_POINT ( 'NONE',  ( 5.346851039111033543, 6.199209027673978412, -1.009771797811720884 ) ) ;
#158829=CARTESIAN_POINT ( 'NONE',  ( 7.539742822975472158, 7.968990512992423447, -0.7216878364870317197 ) ) ;
#158831=CARTESIAN_POINT ( 'NONE',  ( -5.655686355556086120, 6.627330832017406692, 1.199719254218452935 ) ) ;
#158832=CARTESIAN_POINT ( 'NONE',  ( 4.583538449871731757, 7.505156070562471804, 1.199719254218451159 ) ) ;
#158833=VERTEX_POINT ( 'NONE', #30891 ) ;
#158839=CARTESIAN_POINT ( 'NONE',  ( -5.977437402589944604, 6.146301162042552058, -0.1694826866821088351 ) ) ;
#158842=CARTESIAN_POINT ( 'NONE',  ( -5.632486471834530661, 5.535932070087196344, -0.7998128361456362523 ) ) ;
#158860=ORIENTED_EDGE ( 'NONE', *, *, #33468, .T. ) ;
#158870=CARTESIAN_POINT ( 'NONE',  ( 3.607878275012313285, 6.262922849939428716, 1.082531754730549078 ) ) ;
#158875=CARTESIAN_POINT ( 'NONE',  ( 7.180978637093494044, 8.406838493811077839, -1.199719254218452047 ) ) ;
#158876=CARTESIAN_POINT ( 'NONE',  ( 3.553645660113312399, 7.160020680191912845, -1.734723475976807094E-15 ) ) ;
#158888=CARTESIAN_POINT ( 'NONE',  ( -5.818384198920079520, 6.817144982608731141, 1.199719254218452935 ) ) ;
#158890=CARTESIAN_POINT ( 'NONE',  ( -6.557303570864871034, 7.679217583210999010, -1.199719254218452047 ) ) ;
#158892=CARTESIAN_POINT ( 'NONE',  ( 7.146556367734764770, 9.431011410480991231, 1.443375672974063439 ) ) ;
#158896=CARTESIAN_POINT ( 'NONE',  ( -3.824766175154623582, 7.348582304423016964, -0.7466790275774716212 ) ) ;
#158902=CARTESIAN_POINT ( 'NONE',  ( -4.936050443827081580, 7.916420063510339666, 1.199719254218452935 ) ) ;
#158910=CARTESIAN_POINT ( 'NONE',  ( -4.177320726786319049, 6.927272377009067839, -1.082531754730551743 ) ) ;
#158914=CARTESIAN_POINT ( 'NONE',  ( -5.041653019435350380, 6.975290837464928728, -1.599625672291271394 ) ) ;
#158929=DIRECTION ( 'NONE',  ( -2.168404344971003188E-14, 0.000000000000000000, 1.000000000000000000 ) ) ;
#158935=CARTESIAN_POINT ( 'NONE',  ( -5.956828388357799042, 8.042995434541133193, 1.599625672291263179 ) ) ;
#158937=CARTESIAN_POINT ( 'NONE',  ( -5.438755897737433287, 6.374245297895642537, -1.199719254218453823 ) ) ;
#158950=ORIENTED_EDGE ( 'NONE', *, *, #65893, .F. ) ;
#158963=CARTESIAN_POINT ( 'NONE',  ( -4.796552484184649856, 8.818004674849227342, -0.7998128361456362523 ) ) ;
#158964=B_SPLINE_CURVE_WITH_KNOTS ( 'NONE', 3,
 ( #15471, #80495, #116252, #197431, #115192, #146592, #182240, #212610 ),
 .UNSPECIFIED., .F., .F.,
 ( 4, 2, 2, 4 ),
 ( 0.002867044791237291414, 0.003303366235547880534, 0.003521526957703175094, 0.003739687679858470087 ),
 .UNSPECIFIED. ) ;
#158990=CARTESIAN_POINT ( 'NONE',  ( 7.614839552730775729, 8.913009562054615031, 1.199719254218452047 ) ) ;
#159005=CARTESIAN_POINT ( 'NONE',  ( 5.606371582794006159, 7.377293116531995487, 1.238817421570908905 ) ) ;
#159007=CARTESIAN_POINT ( 'NONE',  ( 6.129694847154206983, 8.244672969803623630, -1.443375672974078761 ) ) ;
#159013=CARTESIAN_POINT ( 'NONE',  ( -3.623772196602547346, 7.449761006003425834, 0.000000000000000000 ) ) ;
#159021=CARTESIAN_POINT ( 'NONE',  ( -6.251718229232857915, 7.426664367927358512, -1.082531754730549967 ) ) ;
#159025=CARTESIAN_POINT ( 'NONE',  ( 6.156284269057003655, 9.340026192945279249, -1.199719254218452047 ) ) ;
#159030=CARTESIAN_POINT ( 'NONE',  ( -4.604929450496978660, 5.401447776115099408, -1.199719254218453823 ) ) ;
#159039=CARTESIAN_POINT ( 'NONE',  ( 5.982890925380405456, 10.20206618957764100, 0.000000000000000000 ) ) ;
#159045=CYLINDRICAL_SURFACE ( 'NONE', #81912, 0.7499999999999997780 ) ;
#159057=CARTESIAN_POINT ( 'NONE',  ( -6.343235766347277149, 8.493804042195527870, -1.599625672291271394 ) ) ;
#159060=CARTESIAN_POINT ( 'NONE',  ( 7.191674137406095291, 7.354984346587396082, 0.000000000000000000 ) ) ;
#159079=CARTESIAN_POINT ( 'NONE',  ( 5.885648082108199119, 6.999582529615296700, 1.082531754730549967 ) ) ;
#159089=CARTESIAN_POINT ( 'NONE',  ( -6.644904684473536882, 6.925012684740138980, 0.7216878364870317197 ) ) ;
#159097=DIRECTION ( 'NONE',  ( 0.000000000000000000, 1.000000000000000000, 0.000000000000000000 ) ) ;
#159104=LINE ( 'NONE', #61602, #172001 ) ;
#159121=CARTESIAN_POINT ( 'NONE',  ( 5.388439706788500594, 5.251210844200210559, 0.7998128361456352531 ) ) ;
#159132=CARTESIAN_POINT ( 'NONE',  ( -7.621091744657483069, 8.063897588288083895, 0.7216878364870317197 ) ) ;
#159134=CARTESIAN_POINT ( 'NONE',  ( 3.540087506499646874, 7.144202834309300698, -0.7216878364870338292 ) ) ;
#159148=LINE ( 'NONE', #118998, #137583 ) ;
#159152=CARTESIAN_POINT ( 'NONE',  ( 4.327421620524169121, 8.660439266295391292, 0.7750000000000001332 ) ) ;
#159153=DIRECTION ( 'NONE',  ( -1.000000000000000000, 0.000000000000000000, 0.000000000000000000 ) ) ;
#159181=CARTESIAN_POINT ( 'NONE',  ( -6.957269102468015554, 8.145844036748005834, 1.199719254218452047 ) ) ;
#159184=CARTESIAN_POINT ( 'NONE',  ( -6.774234028683526532, 7.932303117332766718, 1.199719254218452047 ) ) ;
#159185=CARTESIAN_POINT ( 'NONE',  ( -5.274058703912462676, 7.771439464937274444, 1.305864451146660388 ) ) ;
#159186=CARTESIAN_POINT ( 'NONE',  ( -5.010620288702242853, 8.003418215864698482, -1.199719254218453823 ) ) ;
#159194=CARTESIAN_POINT ( 'NONE',  ( -3.006876207180748217, 6.730049018344652190, -0.7998128361456481317 ) ) ;
#159197=CARTESIAN_POINT ( 'NONE',  ( -5.438755897737433287, 6.374245297895642537, -1.199719254218453823 ) ) ;
#159210=CARTESIAN_POINT ( 'NONE',  ( 4.213551878797002992, 8.137837301896977849, 0.000000000000000000 ) ) ;
#159214=ORIENTED_EDGE ( 'NONE', *, *, #182569, .T. ) ;
#159231=CARTESIAN_POINT ( 'NONE',  ( 4.854701522145073334, 7.821512988214679218, -1.199719254218450271 ) ) ;
#159232=CARTESIAN_POINT ( 'NONE',  ( 5.411639590510088027, 6.342609606130419131, -1.199719254218452047 ) ) ;
#159247=CARTESIAN_POINT ( 'NONE',  ( 4.873468316212648865, 8.167532512703042258, 0.9812947938723035612 ) ) ;
#159248=CARTESIAN_POINT ( 'NONE',  ( -3.784134271545645412, 7.428924060196286483, 0.7216878364870338292 ) ) ;
#159249=CARTESIAN_POINT ( 'NONE',  ( 3.092668437693027794, 6.622213920701574885, -0.7216878364870338292 ) ) ;
#159272=EDGE_CURVE ( 'NONE', #108645, #128754, #143088, .T. ) ;
#159278=CARTESIAN_POINT ( 'NONE',  ( 4.228163802615382494, 6.026220084508304708, -1.599625672291269396 ) ) ;
#159297=CARTESIAN_POINT ( 'NONE',  ( -5.772739544368596043, 9.956889578397179363, -0.7998128361456362523 ) ) ;
#159299=ORIENTED_EDGE ( 'NONE', *, *, #173426, .F. ) ;
#159315=CARTESIAN_POINT ( 'NONE',  ( 5.061990249855835344, 6.999017606288844284, -1.599625672291273171 ) ) ;
#159326=CARTESIAN_POINT ( 'NONE',  ( 5.886377668569586774, 7.162856863344262415, 1.137212067324339104 ) ) ;
#159327=CARTESIAN_POINT ( 'NONE',  ( 6.095239321792044862, 7.114357098804711121, 1.141570887979098448 ) ) ;
#159346=CARTESIAN_POINT ( 'NONE',  ( -6.143779885648060102, 7.196773283791382703, 1.199719254218452047 ) ) ;
#159348=CARTESIAN_POINT ( 'NONE',  ( 4.655245641445829641, 6.524482229810530498, 1.599625672291269396 ) ) ;
#159352=CARTESIAN_POINT ( 'NONE',  ( -5.237192476628793614, 9.332084666034067055, 0.7998128361456291469 ) ) ;
#159355=CARTESIAN_POINT ( 'NONE',  ( 7.014364370223726830, 9.276787413384745662, -1.599625672291269396 ) ) ;
#159360=CARTESIAN_POINT ( 'NONE',  ( -5.880564528862151974, 7.271459349814712425, -1.272365726499018246 ) ) ;
#159378=CARTESIAN_POINT ( 'NONE',  ( 6.373741612200174878, 6.608655767087927124, 0.7216878364870328300 ) ) ;
#159381=CARTESIAN_POINT ( 'NONE',  ( -5.901542003698421190, 10.10715911428198055, 0.000000000000000000 ) ) ;
#159391=FACE_OUTER_BOUND ( 'NONE', #3526, .T. ) ;
#159396=CARTESIAN_POINT ( 'NONE',  ( 4.573896719763862251, 6.429575154514868274, -1.599625672291273171 ) ) ;
#159414=EDGE_CURVE ( 'NONE', #37959, #182199, #9542, .T. ) ;
#159446=EDGE_LOOP ( 'NONE', ( #211783, #25842, #208081, #40652, #130884 ) ) ;
#159447=CARTESIAN_POINT ( 'NONE',  ( -6.312203035614172286, 9.521931420595302953, -1.199719254218452047 ) ) ;
#159453=CARTESIAN_POINT ( 'NONE',  ( 6.224601922449876312, 6.434659462379210382, 0.000000000000000000 ) ) ;
#159454=CARTESIAN_POINT ( 'NONE',  ( -6.147696309153835692, 6.137010213626392208, 0.7998128361456281477 ) ) ;
#159459=EDGE_LOOP ( 'NONE', ( #17525, #192713, #205797, #37556, #74400, #179721 ) ) ;
#159464=CARTESIAN_POINT ( 'NONE',  ( -5.330290668828105538, 6.247702530834755130, 1.199719254218452935 ) ) ;
#159466=CARTESIAN_POINT ( 'NONE',  ( 6.265786130652515773, 6.994708711910199384, -0.9640221254198673151 ) ) ;
#159470=CARTESIAN_POINT ( 'NONE',  ( 2.979005374030806230, 6.489267109963819280, 0.4299785398500996503 ) ) ;
#159472=CARTESIAN_POINT ( 'NONE',  ( 6.703580607314123085, 6.785541894813420072, 0.000000000000000000 ) ) ;
#159478=CARTESIAN_POINT ( 'NONE',  ( -4.516801452008150086, 5.298631777878131111, 1.199719254218452935 ) ) ;
#159483=CARTESIAN_POINT ( 'NONE',  ( -6.310394152517827315, 6.326824364217716656, 0.7998128361456281477 ) ) ;
#159487=CARTESIAN_POINT ( 'NONE',  ( 4.529832720297257254, 8.298905583739861314, 0.000000000000000000 ) ) ;
#159488=CARTESIAN_POINT ( 'NONE',  ( -5.275531169048901958, 8.208517892982092334, -1.082531754730549967 ) ) ;
#159496=CARTESIAN_POINT ( 'NONE',  ( 4.583538449871731757, 7.505156070562471804, 1.199719254218451159 ) ) ;
#159497=ORIENTED_EDGE ( 'NONE', *, *, #84476, .F. ) ;
#159503=CARTESIAN_POINT ( 'NONE',  ( 6.042093733545556233, 7.078139439671806699, -1.199719254218452047 ) ) ;
#159524=CARTESIAN_POINT ( 'NONE',  ( 5.015976829175539109, 7.901154160799176651, 1.084432410706299477 ) ) ;
#159533=CARTESIAN_POINT ( 'NONE',  ( 7.028976294042106332, 7.165170195996068969, 0.000000000000000000 ) ) ;
#159538=CARTESIAN_POINT ( 'NONE',  ( -4.693116838625758014, 8.272874032808440248, 0.5769273507626712094 ) ) ;
#159545=CARTESIAN_POINT ( 'NONE',  ( -7.293360289508603600, 7.473618190706972086, 0.000000000000000000 ) ) ;
#159558=CARTESIAN_POINT ( 'NONE',  ( 5.580062740476173566, 8.667767742934335828, 1.199719254218451159 ) ) ;
#159561=CARTESIAN_POINT ( 'NONE',  ( 1.806654366501771136, 2.480000000000016858, 2.499999999999998668 ) ) ;
#159568=CARTESIAN_POINT ( 'NONE',  ( 3.691562964670865199, 7.528850235416478576, -0.7998128361456362523 ) ) ;
#159571=CARTESIAN_POINT ( 'NONE',  ( 4.204437033569277560, 7.919277282557212416, 0.000000000000000000 ) ) ;
#159580=CARTESIAN_POINT ( 'NONE',  ( -5.488562097922137895, 7.488332829134150437, 1.250156803814896245 ) ) ;
#159586=CARTESIAN_POINT ( 'NONE',  ( -4.821859908315634158, 5.654533310236863564, 1.199719254218452935 ) ) ;
#159587=CARTESIAN_POINT ( 'NONE',  ( 6.699137298928145690, 8.909022496873262753, 1.443375672974065660 ) ) ;
#159599=CARTESIAN_POINT ( 'NONE',  ( -6.343235766347277149, 8.493804042195527870, -1.599625672291271394 ) ) ;
#159600=CARTESIAN_POINT ( 'NONE',  ( -3.474632506852224356, 7.275764701294714420, -0.7998128361456481317 ) ) ;
#159602=CARTESIAN_POINT ( 'NONE',  ( 6.007671464186823407, 9.062681570643055906, 1.082531754730549967 ) ) ;
#159608=CARTESIAN_POINT ( 'NONE',  ( 3.444653546323793947, 6.176457016423196222, 1.199719254218451159 ) ) ;
#159616=CARTESIAN_POINT ( 'NONE',  ( -5.591215426272092337, 7.404592667505576209, -1.242541652263975172 ) ) ;
#159623=CARTESIAN_POINT ( 'NONE',  ( 6.238160076063542725, 6.450477308261824305, -0.7216878364870458196 ) ) ;
#159628=CARTESIAN_POINT ( 'NONE',  ( -7.605197822622922210, 7.837428646007010613, -0.7998128361456362523 ) ) ;
#159643=CARTESIAN_POINT ( 'NONE',  ( 5.773793314573267388, 7.829454515125894964, 1.599625672291268286 ) ) ;
#159670=CARTESIAN_POINT ( 'NONE',  ( 0.000000000000000000, 0.000000000000000000, 0.000000000000000000 ) ) ;
#159673=CARTESIAN_POINT ( 'NONE',  ( 6.780486220610169035, 9.003929572168926754, -1.443375672974078761 ) ) ;
#159680=EDGE_CURVE ( 'NONE', #203624, #69840, #17153, .T. ) ;
#159705=CARTESIAN_POINT ( 'NONE',  ( -3.142457743317409680, 6.888227477170756785, 0.7998128361456352531 ) ) ;
#159707=CARTESIAN_POINT ( 'NONE',  ( 6.658462837642799670, 6.940830530104329377, 0.7216878364870328300 ) ) ;
#159713=CARTESIAN_POINT ( 'NONE',  ( -4.308458954092677651, 8.248562223075252220, -0.7998128361456362523 ) ) ;
#159718=CARTESIAN_POINT ( 'NONE',  ( -3.474632506852224356, 7.275764701294714420, -0.7998128361456481317 ) ) ;
#159725=CARTESIAN_POINT ( 'NONE',  ( -4.938913097128142304, 8.984092056616635347, -0.7998128361456362523 ) ) ;
#159735=CARTESIAN_POINT ( 'NONE',  ( -4.984557751679625781, 5.844347460828191565, 1.199719254218452935 ) ) ;
#159738=CARTESIAN_POINT ( 'NONE',  ( -4.814553946628611136, 8.631080347793099961, 0.000000000000000000 ) ) ;
#159739=CARTESIAN_POINT ( 'NONE',  ( -4.299344108864949554, 8.030002203735486788, -0.7216878364870338292 ) ) ;
#159740=CARTESIAN_POINT ( 'NONE',  ( 5.631432701629774051, 7.663367133358481631, 1.599625672291269396 ) ) ;
#159741=CARTESIAN_POINT ( 'NONE',  ( -7.469616286486262524, 7.679250187180907794, 0.7998128361456341429 ) ) ;
#159766=AXIS2_PLACEMENT_3D ( 'NONE', #165814, #85621, #35799 ) ;
#159778=CARTESIAN_POINT ( 'NONE',  ( 4.655672573246532941, 8.415299432525721102, 0.4976263304441782553 ) ) ;
#159790=CARTESIAN_POINT ( 'NONE',  ( 5.712781623311797397, 7.758274208654143855, -1.599625672291283607 ) ) ;
#159793=CARTESIAN_POINT ( 'NONE',  ( -2.844178363816758814, 6.540234867753325076, -0.7998128361456481317 ) ) ;
#159797=CARTESIAN_POINT ( 'NONE',  ( -7.553300976144794454, 7.984808358356614733, -0.7216878364870338292 ) ) ;
#159798=CARTESIAN_POINT ( 'NONE',  ( 7.015401035077338143, 6.062865449010541141, 2.437084766375292144 ) ) ;
#159810=CARTESIAN_POINT ( 'NONE',  ( 8.018721507839716267, 8.319872945426633137, -0.7998128361456341429 ) ) ;
#159811=CARTESIAN_POINT ( 'NONE',  ( 6.367489420273535039, 7.457767740854454708, -1.199719254218452047 ) ) ;
#159812=CARTESIAN_POINT ( 'NONE',  ( 0.2304661401069136861, 2.567903733459023119, -1.989664166560570324 ) ) ;
#159825=CARTESIAN_POINT ( 'NONE',  ( 6.561219994370630637, 6.619454513046008515, 0.000000000000000000 ) ) ;
#159829=ADVANCED_FACE ( 'NONE', ( #118613 ), #72511, .T. ) ;
#159835=DIRECTION ( 'NONE',  ( -0.6507913734559627184, 0.7592566023653016805, 0.000000000000000000 ) ) ;
#159841=CARTESIAN_POINT ( 'NONE',  ( -3.838366886444665393, 7.492195444245147939, 0.000000000000000000 ) ) ;
#159842=CARTESIAN_POINT ( 'NONE',  ( -6.587282531393266360, 8.778525268082516320, 1.599625672291269396 ) ) ;
#159854=CARTESIAN_POINT ( 'NONE',  ( -3.363304624641834106, 6.081549941127532222, -1.199719254218452047 ) ) ;
#159855=CARTESIAN_POINT ( 'NONE',  ( 6.013923656113508542, 9.173938811177871244, -1.199719254218452047 ) ) ;
#159858=CARTESIAN_POINT ( 'NONE',  ( 5.546694241322223107, 5.643767167730274537, -0.7216878364870458196 ) ) ;
#159876=CARTESIAN_POINT ( 'NONE',  ( 3.790386463472274148, 6.579812086429759788, 1.199719254218452047 ) ) ;
#159878=CARTESIAN_POINT ( 'NONE',  ( -4.085803189671902480, 5.860132702740892263, -1.599625672291271394 ) ) ;
#159881=CARTESIAN_POINT ( 'NONE',  ( 5.910428620914669473, 5.860197910680708944, 0.000000000000000000 ) ) ;
#159890=CARTESIAN_POINT ( 'NONE',  ( 6.699137298928153683, 7.948653282571920720, 1.082531754730549967 ) ) ;
#159893=CARTESIAN_POINT ( 'NONE',  ( -5.610041701004606196, 9.767075427805856691, -0.7998128361456362523 ) ) ;
#159894=CARTESIAN_POINT ( 'NONE',  ( 6.215487077222150880, 6.216099443039444949, 0.000000000000000000 ) ) ;
#159904=CARTESIAN_POINT ( 'NONE',  ( -4.878955176071358757, 6.785476686873604280, -1.599625672291271394 ) ) ;
#159941=CARTESIAN_POINT ( 'NONE',  ( 4.217995187182922656, 6.014356699837137832, 1.443375672974058777 ) ) ;
#159954=CARTESIAN_POINT ( 'NONE',  ( -4.197131071882288289, 7.054347462908075350, -1.199719254218455378 ) ) ;
#159956=CARTESIAN_POINT ( 'NONE',  ( -5.074494633264801990, 9.142270515442742607, 0.7998128361456291469 ) ) ;
#159958=CARTESIAN_POINT ( 'NONE',  ( 6.278834536460164983, 9.379038488295265097, -1.082531754730548412 ) ) ;
#159967=CARTESIAN_POINT ( 'NONE',  ( -6.961185525973791144, 7.086080966583015339, 0.7998128361456341429 ) ) ;
#159974=CARTESIAN_POINT ( 'NONE',  ( -5.343321937561608337, 5.406499480009534508, 0.7216878364870257245 ) ) ;
#159979=CARTESIAN_POINT ( 'NONE',  ( -4.502189528189771472, 7.410248995266807803, -1.199719254218453823 ) ) ;
#159999=CARTESIAN_POINT ( 'NONE',  ( -6.119526231721793330, 8.232809585132461194, 1.599625672291263179 ) ) ;
#160001=CARTESIAN_POINT ( 'NONE',  ( -5.829079699232685208, 5.765290835385048496, 0.000000000000000000 ) ) ;
#160010=CYLINDRICAL_SURFACE ( 'NONE', #31709, 1.250000000000000000 ) ;
#160028=CARTESIAN_POINT ( 'NONE',  ( -5.824109505522200081, 8.952488968821326054, -1.199719254218452047 ) ) ;
#160051=CARTESIAN_POINT ( 'NONE',  ( 7.526711554241970248, 8.810193563817646734, -1.199719254218452047 ) ) ;
#160053=CARTESIAN_POINT ( 'NONE',  ( 7.679767667498067496, 7.924426798361372093, 0.000000000000000000 ) ) ;
#160061=CARTESIAN_POINT ( 'NONE',  ( 6.507146750061663099, 6.764461114227863447, -0.3103342489862369602 ) ) ;
#160065=CARTESIAN_POINT ( 'NONE',  ( 5.015976829175539109, 7.901154160799176651, 1.084432410706299477 ) ) ;
#160067=CARTESIAN_POINT ( 'NONE',  ( 7.539742822975472158, 7.968990512992423447, -0.7216878364870317197 ) ) ;
#160075=CARTESIAN_POINT ( 'NONE',  ( -4.285259070371116863, 7.157163461145040095, 1.199719254218452935 ) ) ;
#160082=CARTESIAN_POINT ( 'NONE',  ( -6.902509602688821744, 8.185920970292658083, -1.082531754730549967 ) ) ;
#160086=CARTESIAN_POINT ( 'NONE',  ( 7.842465510862060896, 8.114240948952696542, 0.000000000000000000 ) ) ;
#160087=CARTESIAN_POINT ( 'NONE',  ( 5.081545378421249204, 4.913620246396115832, -0.1915759117748269125 ) ) ;
#160102=CARTESIAN_POINT ( 'NONE',  ( 7.842465510862060896, 8.114240948952696542, 0.000000000000000000 ) ) ;
#160123=CARTESIAN_POINT ( 'NONE',  ( 5.481239241674765950, 9.616805891921051952, -0.7998128361456481317 ) ) ;
#160127=CARTESIAN_POINT ( 'NONE',  ( -6.081925898509194184, 7.037820769655190212, 1.000852813763454252 ) ) ;
#160133=CARTESIAN_POINT ( 'NONE',  ( 6.554440917563797875, 6.611545590104705994, -0.7998128361456481317 ) ) ;
#160136=LINE ( 'NONE', #161207, #36420 ) ;
#160147=CARTESIAN_POINT ( 'NONE',  ( 5.316205630334249754, 7.295602216847000498, -1.443375672974078761 ) ) ;
#160158=CARTESIAN_POINT ( 'NONE',  ( -6.143253000767895600, 6.339752387083549934, 0.000000000000000000 ) ) ;
#160166=CARTESIAN_POINT ( 'NONE',  ( 0.000000000000000000, 0.08000000000000020983, 0.000000000000000000 ) ) ;
#160188=CARTESIAN_POINT ( 'NONE',  ( 5.180097208873055692, 8.201141289397330780, -1.199719254218450271 ) ) ;
#160199=CARTESIAN_POINT ( 'NONE',  ( -6.617788377246193399, 8.814115421577600529, -1.443375672974066548 ) ) ;
#160203=CARTESIAN_POINT ( 'NONE',  ( 4.624739795592929248, 6.488892076315451618, -1.443375672974068769 ) ) ;
#160221=CARTESIAN_POINT ( 'NONE',  ( 4.248158675776232407, 7.140945339103782707, 1.189375853805716643 ) ) ;
#160227=CARTESIAN_POINT ( 'NONE',  ( -4.326460414921602826, 8.061637894134911164, 8.322892513849239118E-08 ) ) ;
#160255=CARTESIAN_POINT ( 'NONE',  ( -7.262327558775498737, 8.501745569106741840, 1.199719254218452047 ) ) ;
#160256=CARTESIAN_POINT ( 'NONE',  ( -5.181409149560055383, 7.856748536063159705, 1.265847179423916335 ) ) ;
#160258=CARTESIAN_POINT ( 'NONE',  ( -4.859018323670466266, 8.113919647779686883, 0.9376688295712337640 ) ) ;
#160264=CARTESIAN_POINT ( 'NONE',  ( -5.191846479390389568, 5.021852078902356631, 0.7998128361456281477 ) ) ;
#160267=CARTESIAN_POINT ( 'NONE',  ( -3.793249116773374396, 7.647484079536056356, 0.7998128361456352531 ) ) ;
#160281=CARTESIAN_POINT ( 'NONE',  ( 5.910428620914669473, 5.860197910680708944, 0.000000000000000000 ) ) ;
#160305=CARTESIAN_POINT ( 'NONE',  ( 4.694866332082116678, 8.699370830729650450, 0.7998128361456341429 ) ) ;
#160306=CARTESIAN_POINT ( 'NONE',  ( 5.910428620914669473, 5.860197910680708944, 0.000000000000000000 ) ) ;
#160311=CARTESIAN_POINT ( 'NONE',  ( -7.065207446497166366, 9.336104335703744539, 0.000000000000000000 ) ) ;
#160322=CARTESIAN_POINT ( 'NONE',  ( 5.260375520412221562, 7.786458765878076171, 1.288147692060326532 ) ) ;
#160323=CARTESIAN_POINT ( 'NONE',  ( -4.624739795592943459, 6.488892076315448065, -1.443375672974066548 ) ) ;
#160324=CARTESIAN_POINT ( 'NONE',  ( 3.119784744920330422, 6.653849612466795627, 0.7216878364870257245 ) ) ;
#160344=CARTESIAN_POINT ( 'NONE',  ( 0.04629450404499204502, 2.597981984072172512, -2.080474185699523026 ) ) ;
#160351=CARTESIAN_POINT ( 'NONE',  ( 3.054329744828568227, 6.785411478933790264, 0.000000000000000000 ) ) ;
#160354=ORIENTED_EDGE ( 'NONE', *, *, #44751, .T. ) ;
#160370=CARTESIAN_POINT ( 'NONE',  ( -7.632314129850253259, 7.869064337772231355, 0.7998128361456341429 ) ) ;
#160372=VERTEX_POINT ( 'NONE', #98337 ) ;
#160387=CARTESIAN_POINT ( 'NONE',  ( 5.737035277238070385, 6.722237907313067140, -1.199719254218452047 ) ) ;
#160394=DIRECTION ( 'NONE',  ( 0.000000000000000000, 0.000000000000000000, 1.000000000000000000 ) ) ;
#160395=CARTESIAN_POINT ( 'NONE',  ( -0.2046361996433256059, 3.442961633857401171, 1.991136556534453206 ) ) ;
#160397=CARTESIAN_POINT ( 'NONE',  ( 5.370783296855561773, 7.572579728427998091, 1.242435897699250891 ) ) ;
#160415=CARTESIAN_POINT ( 'NONE',  ( -6.252245114557387851, 7.323316050852266557, -1.199719254218453823 ) ) ;
#160417=CARTESIAN_POINT ( 'NONE',  ( 4.525389411911321602, 8.501647757197021704, -0.7998128361456381397 ) ) ;
#160421=CARTESIAN_POINT ( 'NONE',  ( -6.261886844665283114, 8.398896966899865646, 1.599625672291269396 ) ) ;
#160425=FACE_OUTER_BOUND ( 'NONE', #475, .T. ) ;
#160427=DIRECTION ( 'NONE',  ( 0.3281536732072464768, -0.000000000000000000, -0.9446243521954066358 ) ) ;
#160429=CARTESIAN_POINT ( 'NONE',  ( -4.624683998644739447, 8.449116153850892985, -0.4091045222319161234 ) ) ;
#160430=DIRECTION ( 'NONE',  ( 0.000000000000000000, 0.000000000000000000, 1.000000000000000000 ) ) ;
#160443=VERTEX_POINT ( 'NONE', #30138 ) ;
#160447=CARTESIAN_POINT ( 'NONE',  ( 4.584065335196261692, 7.401807753487379848, 1.082531754730549078 ) ) ;
#160449=CARTESIAN_POINT ( 'NONE',  ( -4.858757509019083543, 5.629766575900002401, -2.420000000000000373 ) ) ;
#160454=ORIENTED_EDGE ( 'NONE', *, *, #19832, .T. ) ;
#160460=CARTESIAN_POINT ( 'NONE',  ( -3.970504344535652486, 7.404204864921184459, -0.6292205879280321490 ) ) ;
#160461=CARTESIAN_POINT ( 'NONE',  ( -4.990809943606294929, 4.995235487061662205, -0.7216878364870338292 ) ) ;
#160466=CARTESIAN_POINT ( 'NONE',  ( 5.143339171537801846, 7.093924681584509173, 1.599625672291269396 ) ) ;
#160509=CARTESIAN_POINT ( 'NONE',  ( -5.608478439449225306, 5.609308656285654671, -0.4224404339892348093 ) ) ;
#160517=CARTESIAN_POINT ( 'NONE',  ( -5.614485009390564940, 5.722856397143323726, 0.000000000000000000 ) ) ;
#160522=CARTESIAN_POINT ( 'NONE',  ( 6.238160076063574699, 6.450477308261794107, -0.7216878364870207285 ) ) ;
#160523=CARTESIAN_POINT ( 'NONE',  ( -6.784929528996132220, 6.880448970109080520, 0.000000000000000000 ) ) ;
#160529=ORIENTED_EDGE ( 'NONE', *, *, #91370, .T. ) ;
#160532=CARTESIAN_POINT ( 'NONE',  ( -5.113360211009450040, 5.994616996712990975, -1.199719254218453823 ) ) ;
#160534=CARTESIAN_POINT ( 'NONE',  ( 5.753927575595171540, 7.371122731025397279, 1.306365966420112601 ) ) ;
#160539=CARTESIAN_POINT ( 'NONE',  ( 4.355912491740495440, 8.303924683664389406, 0.000000000000000000 ) ) ;
#160546=CARTESIAN_POINT ( 'NONE',  ( -5.029148636026397945, 4.832037928311032182, 0.7998128361456281477 ) ) ;
#160551=CARTESIAN_POINT ( 'NONE',  ( -3.935609729716867289, 7.813571461303467913, 0.7998128361456352531 ) ) ;
#160555=CARTESIAN_POINT ( 'NONE',  ( 5.519577934094851202, 8.493239118869080784, 1.082531754730547524 ) ) ;
#160556=CARTESIAN_POINT ( 'NONE',  ( -6.577113915960841162, 7.806292669110006521, -1.082531754730549967 ) ) ;
#160560=CARTESIAN_POINT ( 'NONE',  ( -4.423703259808839938, 8.383013913077439483, 0.7998128361456350310 ) ) ;
#160563=CARTESIAN_POINT ( 'NONE',  ( 6.554440917563797875, 6.611545590104705994, -0.7998128361456481317 ) ) ;
#160569=CARTESIAN_POINT ( 'NONE',  ( 6.215487077222150880, 6.216099443039444949, 0.000000000000000000 ) ) ;
#160588=LINE ( 'NONE', #94550, #189714 ) ;
#160592=CARTESIAN_POINT ( 'NONE',  ( 4.684024595049480766, 8.263433789595206136, 0.5754648794667740486 ) ) ;
#160602=CARTESIAN_POINT ( 'NONE',  ( 6.505933609711257226, 8.683618192786854095, -1.599625672291281386 ) ) ;
#160608=CARTESIAN_POINT ( 'NONE',  ( -4.626128544448885549, 8.355821839108529048, -0.2988314032242797569 ) ) ;
#160615=CARTESIAN_POINT ( 'NONE',  ( -2.984203208339354152, 6.495671153122273722, 0.000000000000000000 ) ) ;
#160625=CARTESIAN_POINT ( 'NONE',  ( -3.169574050544739841, 6.919863168935977527, -0.7998128361456481317 ) ) ;
#160627=CARTESIAN_POINT ( 'NONE',  ( 6.658989722967328717, 7.797851427330578566, 1.199719254218452935 ) ) ;
#160630=CYLINDRICAL_SURFACE ( 'NONE', #133826, 1.250000000000000000 ) ;
#160633=ORIENTED_EDGE ( 'NONE', *, *, #150631, .T. ) ;
#160635=CARTESIAN_POINT ( 'NONE',  ( 6.527324610336440180, 6.579909898339485252, 0.7998128361456331437 ) ) ;
#160639=CARTESIAN_POINT ( 'NONE',  ( 5.031484404002878996, 7.923796667095108326, 1.082531754730548412 ) ) ;
#160647=CARTESIAN_POINT ( 'NONE',  ( -6.220586654761008027, 6.942393398233093649, 0.8502372543972673835 ) ) ;
#160653=ORIENTED_EDGE ( 'NONE', *, *, #103129, .T. ) ;
#160657=CARTESIAN_POINT ( 'NONE',  ( -3.526002468005825286, 6.271364091718859335, -1.199719254218450271 ) ) ;
#160659=CARTESIAN_POINT ( 'NONE',  ( 5.872089928494542477, 9.864872326636710653, 0.000000000000000000 ) ) ;
#160670=CARTESIAN_POINT ( 'NONE',  ( -4.776215253764153346, 8.794277906025310898, -0.7998128361456362523 ) ) ;
#160671=CARTESIAN_POINT ( 'NONE',  ( -3.461074353238556167, 7.259946855412102273, 0.000000000000000000 ) ) ;
#160673=CARTESIAN_POINT ( 'NONE',  ( 5.980555156959511898, 9.991415093179179863, -0.7216878364870458196 ) ) ;
#160677=CARTESIAN_POINT ( 'NONE',  ( 3.902768115887398803, 5.646591783325653147, -1.599625672291269396 ) ) ;
#160680=PLANE ( 'NONE',  #23872 ) ;
#160684=CARTESIAN_POINT ( 'NONE',  ( -6.419388467533182485, 6.810688026658763938, -0.4840902626340077841 ) ) ;
#160685=FACE_OUTER_BOUND ( 'NONE', #25321, .T. ) ;
#160693=CARTESIAN_POINT ( 'NONE',  ( -3.973948422136981407, 5.729635473950147606, -1.443375672974066548 ) ) ;
#160709=CARTESIAN_POINT ( 'NONE',  ( 7.042534447655770080, 7.180988041878682004, -0.7998128361456341429 ) ) ;
#160720=EDGE_CURVE ( 'NONE', #512, #198714, #105561, .T. ) ;
#160743=CARTESIAN_POINT ( 'NONE',  ( 2.891631901464575272, 6.595597328342462262, 0.000000000000000000 ) ) ;
#160768=AXIS2_PLACEMENT_3D ( 'NONE', #193979, #191838, #9899 ) ;
#160776=CARTESIAN_POINT ( 'NONE',  ( -4.796552484184649856, 8.818004674849227342, -0.7998128361456362523 ) ) ;
#160778=CARTESIAN_POINT ( 'NONE',  ( 6.251718229232841928, 8.387033582228703210, -1.443375672974078761 ) ) ;
#160783=CARTESIAN_POINT ( 'NONE',  ( -5.842637852846353397, 5.781108681267656202, 0.7998128361456281477 ) ) ;
#160789=CARTESIAN_POINT ( 'NONE',  ( -7.485510208520816278, 8.866088343763324886, 1.082531754730549078 ) ) ;
#160797=CARTESIAN_POINT ( 'NONE',  ( -6.017840079619296567, 8.114175741012878973, -1.599625672291271394 ) ) ;
#160804=EDGE_CURVE ( 'NONE', #96867, #92970, #59985, .T. ) ;
#160807=CARTESIAN_POINT ( 'NONE',  ( -4.122561227007127016, 6.967349310553715647, 1.199719254218452935 ) ) ;
#160810=CARTESIAN_POINT ( 'NONE',  ( -6.455090533882213322, 6.703562842383589349, -0.7216878364870338292 ) ) ;
#160811=CARTESIAN_POINT ( 'NONE',  ( -5.709392084686210289, 8.714688961225625974, 1.082531754730550855 ) ) ;
#160812=CARTESIAN_POINT ( 'NONE',  ( 4.552505719138623341, 8.533283448962240669, 0.7998128361456341429 ) ) ;
#160814=CARTESIAN_POINT ( 'NONE',  ( -7.442499979258930587, 7.647614495415686164, -0.7998128361456362523 ) ) ;
#160831=B_SPLINE_CURVE_WITH_KNOTS ( 'NONE', 3,
 ( #47713, #45576, #11977, #144175 ),
 .UNSPECIFIED., .F., .F.,
 ( 4, 4 ),
 ( 6.656384948891156620E-05, 9.470887020559977376E-05 ),
 .UNSPECIFIED. ) ;
#160851=CARTESIAN_POINT ( 'NONE',  ( 4.641544345285703699, 8.432478572106539616, -0.4375188090333537727 ) ) ;
#160859=B_SPLINE_CURVE_WITH_KNOTS ( 'NONE', 3,
 ( #203133, #54775, #104604, #205268, #120922, #38527, #22238, #55839 ),
 .UNSPECIFIED., .F., .F.,
 ( 4, 2, 2, 4 ),
 ( 4.412020206058498508E-14, 0.0006900569950749766085, 0.001035085492590404922, 0.001380113990105833128 ),
 .UNSPECIFIED. ) ;
#160867=CARTESIAN_POINT ( 'NONE',  ( 6.444921918449731280, 8.612437886315108315, 1.599625672291268286 ) ) ;
#160870=CARTESIAN_POINT ( 'NONE',  ( -5.652823702255029836, 5.559658838911111900, -0.7998128361456362523 ) ) ;
#160874=CARTESIAN_POINT ( 'NONE',  ( -6.034787771414192648, 9.094317262408276648, 1.082531754730549967 ) ) ;
#160885=CARTESIAN_POINT ( 'NONE',  ( 8.167861197590044142, 8.493869250135347215, 0.000000000000000000 ) ) ;
#160886=CARTESIAN_POINT ( 'NONE',  ( 6.364626766972446781, 6.390095747748157251, 0.7998128361456352531 ) ) ;
#160887=CARTESIAN_POINT ( 'NONE',  ( 0.4458543674108841337, 2.831572362596164627, -1.950633739370720487 ) ) ;
#160894=CARTESIAN_POINT ( 'NONE',  ( 4.598150373690133463, 5.393538853173795111, -1.199719254218452047 ) ) ;
#160899=ORIENTED_EDGE ( 'NONE', *, *, #28879, .F. ) ;
#160900=CARTESIAN_POINT ( 'NONE',  ( 4.701645408888975197, 8.707279753670952971, 0.000000000000000000 ) ) ;
#160913=VERTEX_POINT ( 'NONE', #76236 ) ;
#160916=CARTESIAN_POINT ( 'NONE',  ( -4.489158259900630554, 8.251452046610447510, 0.000000000000000000 ) ) ;
#160917=CARTESIAN_POINT ( 'NONE',  ( -7.099629715411508890, 8.311931418515415615, 1.199719254218452047 ) ) ;
#160927=ORIENTED_EDGE ( 'NONE', *, *, #163868, .F. ) ;
#160929=CARTESIAN_POINT ( 'NONE',  ( 5.528692779322568640, 9.672168352510192690, 0.7998128361456341429 ) ) ;
#160932=CARTESIAN_POINT ( 'NONE',  ( 4.299344108864946890, 6.109263775132799168, -1.443375672974068769 ) ) ;
#160950=CARTESIAN_POINT ( 'NONE',  ( 4.552505719138623341, 8.533283448962240669, 0.7998128361456341429 ) ) ;
#160951=CARTESIAN_POINT ( 'NONE',  ( -3.644109427023046521, 7.473487774827342278, 0.000000000000000000 ) ) ;
#160955=CARTESIAN_POINT ( 'NONE',  ( 4.064412189046650248, 7.963840997188264659, 0.7998128361456271485 ) ) ;
#160965=CARTESIAN_POINT ( 'NONE',  ( 7.214347136247488912, 7.589362211809770997, -0.7216878364870317197 ) ) ;
#160967=CARTESIAN_POINT ( 'NONE',  ( -7.767895665986912057, 8.027242796598338614, -0.7998128361456362523 ) ) ;
#160968=CARTESIAN_POINT ( 'NONE',  ( 5.716698046817569434, 6.698511138489155137, -1.199719254218452047 ) ) ;
#160978=CARTESIAN_POINT ( 'NONE',  ( -3.786470039966538970, 7.639575156594750283, 0.000000000000000000 ) ) ;
#160997=CARTESIAN_POINT ( 'NONE',  ( -3.838364070418780027, 7.492192144726518954, 0.0001517565043702621237 ) ) ;
#161003=CARTESIAN_POINT ( 'NONE',  ( 5.750066545971570520, 5.881034856487848295, -0.7216878364870458196 ) ) ;
#161009=CARTESIAN_POINT ( 'NONE',  ( 3.729901657090938460, 7.365652676665848553, 0.7216878364870257245 ) ) ;
#161021=CARTESIAN_POINT ( 'NONE',  ( -6.493429226302317225, 6.540365283632955773, 0.7998128361456341429 ) ) ;
#161023=CARTESIAN_POINT ( 'NONE',  ( -5.887983850084758330, 10.09134126839936840, 0.7998128361456291469 ) ) ;
#161036=CARTESIAN_POINT ( 'NONE',  ( -6.180537922983287302, 8.303989891604203422, -1.599625672291271394 ) ) ;
#161042=CARTESIAN_POINT ( 'NONE',  ( -4.285785955695645910, 7.053815144069948140, 1.082531754730549967 ) ) ;
#161046=CARTESIAN_POINT ( 'NONE',  ( -5.906512197408906317, 6.919960980845699439, -1.199719254218453823 ) ) ;
#161069=CARTESIAN_POINT ( 'NONE',  ( -7.065734331377342414, 8.272386803808890576, -1.199719254218452047 ) ) ;
#161071=CARTESIAN_POINT ( 'NONE',  ( -4.655245641445871385, 6.524482229810530498, 1.599625672291263179 ) ) ;
#161096=CARTESIAN_POINT ( 'NONE',  ( -6.957269102468015554, 8.145844036748005834, 1.199719254218452047 ) ) ;
#161105=CARTESIAN_POINT ( 'NONE',  ( 3.939566984407675498, 8.987080315575580514, 0.7749999999999996891 ) ) ;
#161110=AXIS2_PLACEMENT_3D ( 'NONE', #184085, #168907, #103925 ) ;
#161121=EDGE_CURVE ( 'NONE', #10691, #75117, #38207, .T. ) ;
#161123=CARTESIAN_POINT ( 'NONE',  ( 5.989670002187236442, 10.20997511251894529, -0.7998128361456481317 ) ) ;
#161125=CARTESIAN_POINT ( 'NONE',  ( 7.856023664475727308, 8.130058794835305136, -0.7998128361456341429 ) ) ;
#161138=CARTESIAN_POINT ( 'NONE',  ( 4.876420697298537554, 8.045338245374718866, 0.9427337716215690167 ) ) ;
#161140=CARTESIAN_POINT ( 'NONE',  ( 6.536439455564164724, 7.758839131980592718, 1.082531754730549967 ) ) ;
#161146=CARTESIAN_POINT ( 'NONE',  ( -4.960304097753355457, 6.880383762169266504, 1.599625672291263179 ) ) ;
#161152=CARTESIAN_POINT ( 'NONE',  ( -5.112833325684904118, 8.979072956692109031, -0.7216878364870338292 ) ) ;
#161161=ADVANCED_FACE ( 'NONE', ( #76480 ), #94895, .F. ) ;
#161163=CARTESIAN_POINT ( 'NONE',  ( -3.471769853551161411, 6.208092708188416076, 1.199719254218452935 ) ) ;
#161173=CARTESIAN_POINT ( 'NONE',  ( 2.925527285498711549, 6.635141943048991742, 0.7998128361456281477 ) ) ;
#161191=CARTESIAN_POINT ( 'NONE',  ( -8.086512275908061653, 8.398962174839683215, 0.000000000000000000 ) ) ;
#161194=CARTESIAN_POINT ( 'NONE',  ( 7.042534447655770080, 7.180988041878682004, -0.7998128361456341429 ) ) ;
#161197=CARTESIAN_POINT ( 'NONE',  ( -5.955741603288206676, 7.127506980570093020, 1.099513196254948699 ) ) ;
#161204=CARTESIAN_POINT ( 'NONE',  ( 5.890091390494168522, 5.836471141856793388, 0.000000000000000000 ) ) ;
#161207=CARTESIAN_POINT ( 'NONE',  ( 0.000000000000000000, 9.999999999999998224, -2.000000000000000000 ) ) ;
#161211=CARTESIAN_POINT ( 'NONE',  ( 3.607878275012313285, 6.262922849939428716, 1.082531754730549078 ) ) ;
#161215=CARTESIAN_POINT ( 'NONE',  ( 4.068855497876973537, 7.761098824249525130, -0.7216878364870338292 ) ) ;
#161226=CARTESIAN_POINT ( 'NONE',  ( -5.994113311017573054, 6.165756082374834079, 0.7216878364870257245 ) ) ;
#161249=CARTESIAN_POINT ( 'NONE',  ( 3.913815762669449416, 7.330443837381343641, -0.8582294057540799104 ) ) ;
#161259=CARTESIAN_POINT ( 'NONE',  ( 5.367048706163317640, 7.354919138647580290, -1.599625672291281386 ) ) ;
#161261=CARTESIAN_POINT ( 'NONE',  ( 4.877901405866606588, 8.912911750144889567, 0.7998128361456341429 ) ) ;
#161266=DIRECTION ( 'NONE',  ( 1.000000000000000000, 0.000000000000000000, 0.000000000000000000 ) ) ;
#161273=CARTESIAN_POINT ( 'NONE',  ( -7.485510208520816278, 8.866088343763324886, 1.082531754730549078 ) ) ;
#161276=CARTESIAN_POINT ( 'NONE',  ( 6.016786309414542622, 10.24161080428416426, 0.7998128361456341429 ) ) ;
#161286=CARTESIAN_POINT ( 'NONE',  ( 5.413285142218079216, 7.534467834982624623, -1.255836820238024121 ) ) ;
#161292=CARTESIAN_POINT ( 'NONE',  ( -6.305950844131887223, 6.529566537674873494, 0.000000000000000000 ) ) ;
#161294=CARTESIAN_POINT ( 'NONE',  ( -5.817857314039913241, 5.960124085900898372, 0.000000000000000000 ) ) ;
#161304=EDGE_CURVE ( 'NONE', #77529, #157380, #99681, .T. ) ;
#161311=ORIENTED_EDGE ( 'NONE', *, *, #160720, .F. ) ;
#161332=CARTESIAN_POINT ( 'NONE',  ( -6.064239847062411926, 10.29697326487330500, 0.000000000000000000 ) ) ;
#161333=CARTESIAN_POINT ( 'NONE',  ( -5.739830873228516595, 7.379802178037835780, 1.322642659050039970 ) ) ;
#161339=CARTESIAN_POINT ( 'NONE',  ( -6.685579144870156476, 9.853573864773576219, 1.082531754730549967 ) ) ;
#161346=CARTESIAN_POINT ( 'NONE',  ( -3.871735385154307263, 6.674719161725423788, -1.199719254218450271 ) ) ;
#161352=CARTESIAN_POINT ( 'NONE',  ( -6.473746350531913940, 6.725327903095910109, 0.2421321588450163209 ) ) ;
#161359=CARTESIAN_POINT ( 'NONE',  ( 5.845500506147374153, 6.848780674373954547, 1.199719254218453823 ) ) ;
#161384=EDGE_CURVE ( 'NONE', #154266, #19980, #197299, .T. ) ;
#161385=CARTESIAN_POINT ( 'NONE',  ( 4.193214648376505593, 8.114110533073061404, 0.000000000000000000 ) ) ;
#161386=CARTESIAN_POINT ( 'NONE',  ( 3.088225128862704949, 6.824956093640315302, 0.7998128361456281477 ) ) ;
#161389=CARTESIAN_POINT ( 'NONE',  ( 4.065465959251388206, 5.836405933916976707, -1.599625672291269396 ) ) ;
#161401=CARTESIAN_POINT ( 'NONE',  ( 5.214490215732396017, 7.828485850976955263, 1.269369371331245500 ) ) ;
#161402=CARTESIAN_POINT ( 'NONE',  ( -4.733205024502264102, 7.575804057677677505, 1.082531754730549967 ) ) ;
#161403=CARTESIAN_POINT ( 'NONE',  ( 5.072158865288245444, 5.090142562357324429, 0.7216878364870338292 ) ) ;
#161418=CIRCLE ( 'NONE', #189074, 0.08000000000000041800 ) ;
#161429=CARTESIAN_POINT ( 'NONE',  ( 6.052789233858158369, 6.026285292448116948, 0.000000000000000000 ) ) ;
#161451=CARTESIAN_POINT ( 'NONE',  ( -5.420227550413282636, 9.545625585449309725, 0.7998128361456291469 ) ) ;
#161462=CARTESIAN_POINT ( 'NONE',  ( 4.179656494762836516, 8.098292687190454586, -0.7998128361456362523 ) ) ;
#161467=ORIENTED_EDGE ( 'NONE', *, *, #68466, .F. ) ;
#161468=CARTESIAN_POINT ( 'NONE',  ( 6.225128807330042591, 7.291680359087043151, -1.199719254218452047 ) ) ;
#161479=CARTESIAN_POINT ( 'NONE',  ( -3.059665831784952651E-14, 3.479999999999999538, 2.000000000000000000 ) ) ;
#161500=CARTESIAN_POINT ( 'NONE',  ( -5.498713818794216834, 8.572860667638675380, -1.199719254218452047 ) ) ;
#161502=CARTESIAN_POINT ( 'NONE',  ( 5.037736595929563244, 8.035053907629919223, -1.199719254218452047 ) ) ;
#161503=CARTESIAN_POINT ( 'NONE',  ( -2.723004532691724489, 3.009022671084740974, 2.500000000000000444 ) ) ;
#161506=CARTESIAN_POINT ( 'NONE',  ( -5.749539660647037032, 8.865490816466966351, 1.199719254218454489 ) ) ;
#161509=CARTESIAN_POINT ( 'NONE',  ( 7.095713291905693332, 9.371694488680407886, 1.599625672291268286 ) ) ;
#161514=CARTESIAN_POINT ( 'NONE',  ( -6.423891471114925977, 6.884501071190606503, -0.7550301924055674574 ) ) ;
#161531=CARTESIAN_POINT ( 'NONE',  ( 6.699137298928158124, 6.988284068270579574, 0.7216878364870328300 ) ) ;
#161544=CARTESIAN_POINT ( 'NONE',  ( -5.343321937561608337, 5.406499480009534508, 0.7216878364870257245 ) ) ;
#161548=CARTESIAN_POINT ( 'NONE',  ( 5.737035277238070385, 6.722237907313067140, -1.199719254218452047 ) ) ;
#161571=EDGE_CURVE ( 'NONE', #22501, #136572, #19476, .T. ) ;
#161597=CARTESIAN_POINT ( 'NONE',  ( 3.902768115887398803, 5.646591783325653147, -1.599625672291269396 ) ) ;
#161601=CARTESIAN_POINT ( 'NONE',  ( -5.329763783503577379, 6.351050847909847086, 1.082531754730549078 ) ) ;
#161607=CARTESIAN_POINT ( 'NONE',  ( -4.610654757099099221, 7.536791762327691657, 1.199719254218452935 ) ) ;
#161612=VERTEX_POINT ( 'NONE', #1596 ) ;
#161616=CARTESIAN_POINT ( 'NONE',  ( -5.842637852846353397, 5.781108681267656202, 0.7998128361456281477 ) ) ;
#161618=CARTESIAN_POINT ( 'NONE',  ( 6.548892101489681927, 6.803534504848940401, 0.4251794856353352525 ) ) ;
#161623=CARTESIAN_POINT ( 'NONE',  ( 6.313256805818848960, 7.394496357324014113, 1.199719254218452047 ) ) ;
#161630=CARTESIAN_POINT ( 'NONE',  ( -6.237633190739009237, 9.434933268240943249, 1.199719254218452047 ) ) ;
#161632=ORIENTED_EDGE ( 'NONE', *, *, #90176, .T. ) ;
#161635=CARTESIAN_POINT ( 'NONE',  ( -5.529746549527323474, 7.544733289238903851, -1.599625672291271394 ) ) ;
#161639=CARTESIAN_POINT ( 'NONE',  ( 5.329763783503544516, 9.232158490813878515, -0.7216878364870458196 ) ) ;
#161641=CARTESIAN_POINT ( 'NONE',  ( -5.221298554594238084, 8.145246509451649075, 1.082531754730549967 ) ) ;
#161648=CARTESIAN_POINT ( 'NONE',  ( 4.878955176071345434, 6.785476686873604280, -1.599625672291269396 ) ) ;
#161655=CARTESIAN_POINT ( 'NONE',  ( 4.355912491740495440, 8.303924683664389406, 0.000000000000000000 ) ) ;
#161656=DIRECTION ( 'NONE',  ( -0.6507913734559658270, -0.7592566023652989049, 0.000000000000000000 ) ) ;
#161678=CARTESIAN_POINT ( 'NONE',  ( 4.594924845400013780, 8.373833185659544043, 0.04553248676899754321 ) ) ;
#161686=CARTESIAN_POINT ( 'NONE',  ( 5.006703865196457492, 9.063181286029688977, 0.000000000000000000 ) ) ;
#161692=CARTESIAN_POINT ( 'NONE',  ( -4.789308618567226006, 8.160042084799258078, 0.7984581689710170682 ) ) ;
#161699=CARTESIAN_POINT ( 'NONE',  ( -4.299344108864961989, 6.109263775132799168, -1.443375672974066548 ) ) ;
#161710=CARTESIAN_POINT ( 'NONE',  ( -4.842197138736131556, 5.678260079060780008, 1.199719254218452935 ) ) ;
#161720=CARTESIAN_POINT ( 'NONE',  ( 5.716698046817569434, 6.698511138489155137, -1.199719254218452047 ) ) ;
#161723=CARTESIAN_POINT ( 'NONE',  ( 6.197485614778188712, 6.403023770095574108, -0.7216878364870458196 ) ) ;
#161738=CARTESIAN_POINT ( 'NONE',  ( -5.632486471834530661, 5.535932070087196344, -0.7998128361456362523 ) ) ;
#161739=CARTESIAN_POINT ( 'NONE',  ( 4.878955176071345434, 6.785476686873604280, -1.599625672291269396 ) ) ;
#161750=CARTESIAN_POINT ( 'NONE',  ( -6.261886844665283114, 8.398896966899865646, 1.599625672291269396 ) ) ;
#161751=CARTESIAN_POINT ( 'NONE',  ( 5.020262018810099924, 9.078999131912302900, 0.7998128361456331437 ) ) ;
#161753=CARTESIAN_POINT ( 'NONE',  ( 6.875393295461478260, 8.154285278527437342, -1.082531754730548412 ) ) ;
#161758=CARTESIAN_POINT ( 'NONE',  ( 4.065465959251388206, 5.836405933916976707, -1.599625672291269396 ) ) ;
#161764=CARTESIAN_POINT ( 'NONE',  ( -5.947459870766462764, 7.133493745255431229, -1.104964307564069603 ) ) ;
#161772=CARTESIAN_POINT ( 'NONE',  ( -7.014364370223741929, 9.276787413384745662, -1.599625672291271394 ) ) ;
#161789=CARTESIAN_POINT ( 'NONE',  ( 6.313256805818848960, 7.394496357324014113, 1.199719254218452047 ) ) ;
#161824=CARTESIAN_POINT ( 'NONE',  ( 5.388439706788500594, 5.251210844200210559, 0.7998128361456352531 ) ) ;
#161827=CARTESIAN_POINT ( 'NONE',  ( -4.556949027968976829, 5.449433633119473264, 1.082531754730549078 ) ) ;
#161855=CARTESIAN_POINT ( 'NONE',  ( -6.629010762438975135, 6.698543742459062145, -0.7998128361456362523 ) ) ;
#161857=CARTESIAN_POINT ( 'NONE',  ( 5.682275777458841048, 8.683053269460405232, 1.082531754730547524 ) ) ;
#161862=CARTESIAN_POINT ( 'NONE',  ( -4.847922445338252118, 7.813604065273374921, -1.199719254218453823 ) ) ;
#161867=CARTESIAN_POINT ( 'NONE',  ( -5.469788628470539926, 5.346117919495872783, -0.7998128361456362523 ) ) ;
#161875=CARTESIAN_POINT ( 'NONE',  ( -4.749098946536820520, 8.762642214260091933, 0.7998128361456281477 ) ) ;
#161885=CARTESIAN_POINT ( 'NONE',  ( -4.285259070371116863, 7.157163461145040095, 1.199719254218452935 ) ) ;
#161889=CARTESIAN_POINT ( 'NONE',  ( -5.478903473698255588, 7.485416367438324059, -1.443375672974066548 ) ) ;
#161890=CARTESIAN_POINT ( 'NONE',  ( -5.736508391913536897, 9.706693867292189637, 0.7216878364870267237 ) ) ;
#161891=CARTESIAN_POINT ( 'NONE',  ( 7.537407054554579489, 7.758339416593960536, 0.000000000000000000 ) ) ;
#161892=CARTESIAN_POINT ( 'NONE',  ( -5.759181390754928742, 9.941071732514568993, 0.000000000000000000 ) ) ;
#161930=CARTESIAN_POINT ( 'NONE',  ( 4.681345713234763117, 8.384430392927429310, -0.5894114041281351968 ) ) ;
#161944=CARTESIAN_POINT ( 'NONE',  ( 7.049313524462606395, 7.188896964819984525, 0.000000000000000000 ) ) ;
#161947=CARTESIAN_POINT ( 'NONE',  ( -4.899292406491858820, 6.809203455697518947, -1.599625672291271394 ) ) ;
#161951=CARTESIAN_POINT ( 'NONE',  ( -6.577113915960836721, 8.766661883411348555, -1.443375672974066548 ) ) ;
#161961=CARTESIAN_POINT ( 'NONE',  ( 3.901714345682657292, 7.774026846596938434, 0.7998128361456271485 ) ) ;
#161963=CARTESIAN_POINT ( 'NONE',  ( 5.020262018810099924, 9.078999131912302900, 0.7998128361456331437 ) ) ;
#161978=CARTESIAN_POINT ( 'NONE',  ( 6.821687566331318564, 7.987665577921906568, 1.199719254218452935 ) ) ;
#161991=CARTESIAN_POINT ( 'NONE',  ( -3.987506576194992824, 7.666191748953863794, 0.7216878364870338292 ) ) ;
#161992=CARTESIAN_POINT ( 'NONE',  ( 5.750066545971570520, 5.881034856487848295, -0.7216878364870458196 ) ) ;
#162004=CARTESIAN_POINT ( 'NONE',  ( -6.617788377246193399, 8.814115421577600529, -1.443375672974066548 ) ) ;
#162005=CARTESIAN_POINT ( 'NONE',  ( 6.502017186205484300, 9.743381262951846367, -1.199719254218452047 ) ) ;
#162008=CARTESIAN_POINT ( 'NONE',  ( 5.221298554594243413, 5.264138866547622975, -0.7216878364870458196 ) ) ;
#162024=CARTESIAN_POINT ( 'NONE',  ( 6.235824307642648279, 6.239826211863360506, 0.000000000000000000 ) ) ;
#162026=CARTESIAN_POINT ( 'NONE',  ( -5.438755897737433287, 6.374245297895642537, -1.199719254218453823 ) ) ;
#162037=CARTESIAN_POINT ( 'NONE',  ( 7.675324359112103423, 8.127168971818530707, 0.7216878364870267237 ) ) ;
#162039=CARTESIAN_POINT ( 'NONE',  ( -6.526270840131767059, 8.707344961610770540, -1.599625672291271394 ) ) ;
#162040=CARTESIAN_POINT ( 'NONE',  ( 6.313256805818848960, 7.394496357324014113, 1.199719254218452047 ) ) ;
#162050=CARTESIAN_POINT ( 'NONE',  ( -5.743814354044916470, 6.730146830254374990, -1.199719254218453823 ) ) ;
#162063=LINE ( 'NONE', #13652, #63953 ) ;
#162078=CARTESIAN_POINT ( 'NONE',  ( 4.204437034013637664, 6.958908068774287692, -1.082531754730548412 ) ) ;
#162079=VERTEX_POINT ( 'NONE', #90361 ) ;
#162084=CARTESIAN_POINT ( 'NONE',  ( 6.021229617800532452, 6.197391773621639288, 0.000000000000000000 ) ) ;
#162098=CARTESIAN_POINT ( 'NONE',  ( -6.119526231721793330, 8.232809585132461194, 1.599625672291263179 ) ) ;
#162100=CARTESIAN_POINT ( 'NONE',  ( -5.399890319992785237, 9.521898816625391504, 0.7998128361456291469 ) ) ;
#162106=CARTESIAN_POINT ( 'NONE',  ( 7.635176783151273128, 8.936736330878529699, 1.199719254218452935 ) ) ;
#162111=CARTESIAN_POINT ( 'NONE',  ( -6.771371375382467583, 6.864631124226471037, -0.7998128361456362523 ) ) ;
#162117=CARTESIAN_POINT ( 'NONE',  ( -4.909461021924285795, 6.821066840368686712, 1.443375672974058777 ) ) ;
#162121=CARTESIAN_POINT ( 'NONE',  ( -3.935609729716867289, 7.813571461303467913, 0.7998128361456352531 ) ) ;
#162143=CARTESIAN_POINT ( 'NONE',  ( -5.112833325684928987, 5.137596099486740897, -0.7216878364870338292 ) ) ;
#162146=CARTESIAN_POINT ( 'NONE',  ( -4.899292406491858820, 6.809203455697518947, -1.599625672291271394 ) ) ;
#162171=CARTESIAN_POINT ( 'NONE',  ( -7.632314129850253259, 7.869064337772231355, 0.7998128361456341429 ) ) ;
#162178=CARTESIAN_POINT ( 'NONE',  ( 3.912682303000288631, 8.998411203033816363, 0.7749999999999996891 ) ) ;
#162195=CARTESIAN_POINT ( 'NONE',  ( 6.003228155800906407, 10.22579295840155744, 0.000000000000000000 ) ) ;
#162196=CARTESIAN_POINT ( 'NONE',  ( 5.993586425693011144, 9.150212042353954800, -1.199719254218452047 ) ) ;
#162211=CARTESIAN_POINT ( 'NONE',  ( 5.370783296855561773, 7.572579728427998091, 1.242435897699250891 ) ) ;
#162213=CARTESIAN_POINT ( 'NONE',  ( 5.709392085130549077, 9.675058176045386205, 0.000000000000000000 ) ) ;
#162219=CARTESIAN_POINT ( 'NONE',  ( -5.798046968499580345, 6.793418213784815585, 1.199719254218452935 ) ) ;
#162222=B_SPLINE_CURVE_WITH_KNOTS ( 'NONE', 3,
 ( #44285, #174297, #189452, #24806, #43230, #110406 ),
 .UNSPECIFIED., .F., .F.,
 ( 4, 2, 4 ),
 ( 0.000000000000000000, 0.0007391056041462109151, 0.001478211208292421830 ),
 .UNSPECIFIED. ) ;
#162225=CARTESIAN_POINT ( 'NONE',  ( -6.577113915960836721, 8.766661883411348555, -1.443375672974066548 ) ) ;
#162228=CARTESIAN_POINT ( 'NONE',  ( -5.817856928050925802, 5.960123635580414359, -1.359047942450207100E-08 ) ) ;
#162242=CARTESIAN_POINT ( 'NONE',  ( 5.806634928402749196, 9.996434193103704402, -0.7998128361456481317 ) ) ;
#162260=CARTESIAN_POINT ( 'NONE',  ( -5.915100157312088491, 10.12297696016459092, -0.7998128361456362523 ) ) ;
#162264=CARTESIAN_POINT ( 'NONE',  ( 5.885121196783658526, 9.023669275293071834, 1.199719254218452047 ) ) ;
#162266=CARTESIAN_POINT ( 'NONE',  ( -5.998939594393441155, 7.096481464931535754, 1.069142741232721461 ) ) ;
#162272=CARTESIAN_POINT ( 'NONE',  ( 6.378184920586140727, 6.405913593630768510, 0.000000000000000000 ) ) ;
#162282=CARTESIAN_POINT ( 'NONE',  ( 6.427974226654860956, 7.632296364919712417, -1.082531754730548412 ) ) ;
#162293=CARTESIAN_POINT ( 'NONE',  ( -4.502716413514296079, 8.267269892493059658, -0.7216878364870338292 ) ) ;
#162324=VERTEX_POINT ( 'NONE', #75173 ) ;
#162328=CARTESIAN_POINT ( 'NONE',  ( 6.690022453700429139, 6.769724048930809701, 0.7998128361456331437 ) ) ;
#162330=CARTESIAN_POINT ( 'NONE',  ( 6.398522151006641678, 6.429640362454684954, 0.000000000000000000 ) ) ;
#162343=CARTESIAN_POINT ( 'NONE',  ( -3.135678666510573365, 6.880318554229450712, 0.000000000000000000 ) ) ;
#162346=CARTESIAN_POINT ( 'NONE',  ( 6.183927461164522299, 6.387205924212962849, 0.000000000000000000 ) ) ;
#162356=EDGE_CURVE ( 'NONE', #81693, #95637, #194271, .T. ) ;
#162357=CARTESIAN_POINT ( 'NONE',  ( 4.929342268689171469, 7.989555622611471897, -1.003472558803005565 ) ) ;
#162363=CARTESIAN_POINT ( 'NONE',  ( -5.966997003790228682, 8.054858819212300958, -1.443375672974066548 ) ) ;
#162365=CARTESIAN_POINT ( 'NONE',  ( -4.611181642423629157, 7.433443445252599702, 1.082531754730549967 ) ) ;
#162393=CARTESIAN_POINT ( 'NONE',  ( -3.481411583659053566, 7.283673624236017830, 0.000000000000000000 ) ) ;
#162403=CARTESIAN_POINT ( 'NONE',  ( -6.994027139803241866, 9.253060644560830994, -1.599625672291271394 ) ) ;
#162404=CARTESIAN_POINT ( 'NONE',  ( -4.631600894319110040, 8.440630447364583233, 0.4419995416731822280 ) ) ;
#162412=CARTESIAN_POINT ( 'NONE',  ( -4.522526758610270647, 7.433975764090723359, -1.199719254218453823 ) ) ;
#162415=CARTESIAN_POINT ( 'NONE',  ( -5.978219388983010418, 5.939287140093762574, -0.7998128361456362523 ) ) ;
#162425=CARTESIAN_POINT ( 'NONE',  ( 5.899733120602060232, 6.912052057904395141, -1.199719254218452047 ) ) ;
#162430=CARTESIAN_POINT ( 'NONE',  ( 0.01777464290183803503, 3.404255796403599987, -2.081138097628782990 ) ) ;
#162448=CARTESIAN_POINT ( 'NONE',  ( 5.123001941117305336, 7.070197912760590064, 1.599625672291268286 ) ) ;
#162449=CARTESIAN_POINT ( 'NONE',  ( 5.246079093845007257, 5.085123462432798114, 0.7998128361456352531 ) ) ;
#162451=CARTESIAN_POINT ( 'NONE',  ( 3.040771591214902259, 6.769593633051179005, -0.7998128361456362523 ) ) ;
#162454=DIRECTION ( 'NONE',  ( 0.6507913734559641616, -0.7592566023653004592, 0.000000000000000000 ) ) ;
#162463=CARTESIAN_POINT ( 'NONE',  ( 4.595652554671352696, 8.489339133230261680, -0.03962354257190832396 ) ) ;
#162464=VECTOR ( 'NONE', #47393, 1000.000000000000114 ) ;
#162465=CARTESIAN_POINT ( 'NONE',  ( -5.221298554594238084, 8.145246509451649075, 1.082531754730549967 ) ) ;
#162496=CARTESIAN_POINT ( 'NONE',  ( 3.705121118284530279, 7.544668081299086282, -1.734723475976807094E-15 ) ) ;
#162498=CARTESIAN_POINT ( 'NONE',  ( 3.410758162289653672, 6.136912401716668519, -1.199719254218453823 ) ) ;
#162514=CARTESIAN_POINT ( 'NONE',  ( -7.553827861469316396, 8.841829255582865699, -1.199719254218452047 ) ) ;
#162519=DIRECTION ( 'NONE',  ( 0.000000000000000000, 0.000000000000000000, 1.000000000000000000 ) ) ;
#162525=CARTESIAN_POINT ( 'NONE',  ( 5.397027666691686321, 8.454226823519094935, 1.199719254218451159 ) ) ;
#162530=CARTESIAN_POINT ( 'NONE',  ( 6.387826650694035990, 7.481494509678370264, -1.199719254218452047 ) ) ;
#162535=ORIENTED_EDGE ( 'NONE', *, *, #90176, .F. ) ;
#162543=CARTESIAN_POINT ( 'NONE',  ( 4.635702676548680401, 8.322458603728597026, -0.3981331281527732968 ) ) ;
#162551=CARTESIAN_POINT ( 'NONE',  ( 4.552304845665864796, 6.880248622055519903, 1.357528830636938189 ) ) ;
#162556=CARTESIAN_POINT ( 'NONE',  ( -6.243047111023654949, 6.927230885129543658, 0.8200755559147846485 ) ) ;
#162558=ORIENTED_EDGE ( 'NONE', *, *, #202320, .T. ) ;
#162563=CARTESIAN_POINT ( 'NONE',  ( -5.981082042284069367, 7.006959133200059142, 1.199719254218452935 ) ) ;
#162565=CARTESIAN_POINT ( 'NONE',  ( 6.225128807330042591, 7.291680359087043151, -1.199719254218452047 ) ) ;
#162568=CARTESIAN_POINT ( 'NONE',  ( -5.915100157312088491, 10.12297696016459092, -0.7998128361456362523 ) ) ;
#162576=CARTESIAN_POINT ( 'NONE',  ( -0.4603033281871871663, 3.129930857433576907, -1.947265364836649137 ) ) ;
#162591=CARTESIAN_POINT ( 'NONE',  ( 6.048345925472183637, 8.149765894507963182, 1.443375672974065660 ) ) ;
#162598=EDGE_CURVE ( 'NONE', #100096, #96449, #120023, .T. ) ;
#162606=CARTESIAN_POINT ( 'NONE',  ( -5.316205630334276400, 5.374863788244313767, -0.7216878364870338292 ) ) ;
#162609=CARTESIAN_POINT ( 'NONE',  ( 3.562760505341037831, 7.378580699531681830, -1.734723475976807094E-15 ) ) ;
#162615=LINE ( 'NONE', #66125, #108265 ) ;
#162634=DIRECTION ( 'NONE',  ( 0.7592566023652995710, 0.6507913734559650498, -0.000000000000000000 ) ) ;
#162643=EDGE_CURVE ( 'NONE', #82462, #109831, #153527, .T. ) ;
#162666=CARTESIAN_POINT ( 'NONE',  ( -3.648552735408985725, 7.270745601370182776, -0.7216878364870458196 ) ) ;
#162672=CARTESIAN_POINT ( 'NONE',  ( -5.261446130555064826, 8.296048364692991228, 1.199719254218452935 ) ) ;
#162680=CARTESIAN_POINT ( 'NONE',  ( 8.154303043976348420, 8.478051404252736845, 0.7998128361456281477 ) ) ;
#162681=CARTESIAN_POINT ( 'NONE',  ( -4.145761110728687804, 8.058748072483927771, -0.7998128361456481317 ) ) ;
#162683=CARTESIAN_POINT ( 'NONE',  ( 6.410638904775656677, 6.895589754593423493, 0.7569561588358000304 ) ) ;
#162686=DIRECTION ( 'NONE',  ( -0.7592566023652990159, -0.6507913734559659380, 0.000000000000000000 ) ) ;
#162688=CARTESIAN_POINT ( 'NONE',  ( 5.234329823327693809, 8.264412672927770487, 1.199719254218451159 ) ) ;
#162698=CARTESIAN_POINT ( 'NONE',  ( -4.630991987519598396, 7.560518531151607213, 1.199719254218452935 ) ) ;
#162702=CARTESIAN_POINT ( 'NONE',  ( -6.608673532018475960, 6.674816973635147477, -0.7998128361456362523 ) ) ;
#162706=CARTESIAN_POINT ( 'NONE',  ( 6.170369307550815030, 8.292126506933040986, 1.443375672974064550 ) ) ;
#162708=CARTESIAN_POINT ( 'NONE',  ( -4.923019175093582334, 8.757623114335565617, 0.7216878364870267237 ) ) ;
#162714=CARTESIAN_POINT ( 'NONE',  ( 6.527324610336440180, 6.579909898339485252, 0.7998128361456331437 ) ) ;
#162724=CARTESIAN_POINT ( 'NONE',  ( 0.3999999999999758193, 3.000000000029069636, -2.023857702507768419 ) ) ;
#162740=DIRECTION ( 'NONE',  ( -0.6507913734559640506, -0.7592566023653003482, 0.000000000000000000 ) ) ;
#162755=CARTESIAN_POINT ( 'NONE',  ( 7.452141709366786770, 8.723195411463290583, 1.199719254218452047 ) ) ;
#162760=CARTESIAN_POINT ( 'NONE',  ( -5.764421489320544545, 7.269302474779911982, -1.197982331091128616 ) ) ;
#162765=CARTESIAN_POINT ( 'NONE',  ( -3.648552735408985725, 7.270745601370182776, -0.7216878364870458196 ) ) ;
#162775=CARTESIAN_POINT ( 'NONE',  ( -3.494969737272722643, 7.299491470118629088, -0.7998128361456481317 ) ) ;
#162782=VERTEX_POINT ( 'NONE', #121108 ) ;
#162786=CARTESIAN_POINT ( 'NONE',  ( 3.881377115262159894, 7.750300077773022878, 0.7998128361456271485 ) ) ;
#162789=CARTESIAN_POINT ( 'NONE',  ( 4.950135482320912494, 6.868520377498098739, -1.443375672974068769 ) ) ;
#162797=CARTESIAN_POINT ( 'NONE',  ( 0.000000000000000000, 8.920000000000001705, 0.000000000000000000 ) ) ;
#162803=CARTESIAN_POINT ( 'NONE',  ( -6.608673532018475960, 6.674816973635147477, -0.7998128361456362523 ) ) ;
#162804=CARTESIAN_POINT ( 'NONE',  ( 4.960304097753311936, 6.880383762169266504, 1.599625672291268286 ) ) ;
#162816=CARTESIAN_POINT ( 'NONE',  ( -5.237192476628793614, 9.332084666034067055, 0.7998128361456291469 ) ) ;
#162817=CARTESIAN_POINT ( 'NONE',  ( 6.343235766347262938, 8.493804042195527870, -1.599625672291281386 ) ) ;
#162825=CARTESIAN_POINT ( 'NONE',  ( 3.203469434578891661, 6.959407783642502565, -0.7998128361456362523 ) ) ;
#162831=CARTESIAN_POINT ( 'NONE',  ( -6.169688749744446810, 7.059909438329341036, 1.079748085779270950 ) ) ;
#162840=CARTESIAN_POINT ( 'NONE',  ( -4.462041952228957165, 5.338708711422782471, -1.082531754730549967 ) ) ;
#162854=ORIENTED_EDGE ( 'NONE', *, *, #155093, .F. ) ;
#162886=CARTESIAN_POINT ( 'NONE',  ( 6.861835142292135536, 9.098836647464588978, 1.443375672974065660 ) ) ;
#162887=CARTESIAN_POINT ( 'NONE',  ( -3.851925040058337579, 6.547644075826416277, -1.082531754730546636 ) ) ;
#162918=CARTESIAN_POINT ( 'NONE',  ( -4.522526758610270647, 7.433975764090723359, -1.199719254218453823 ) ) ;
#162920=CARTESIAN_POINT ( 'NONE',  ( 5.465345319640213972, 8.429967735338637524, -1.082531754730548412 ) ) ;
#162925=CARTESIAN_POINT ( 'NONE',  ( -6.466312919074983512, 6.508729591867735031, -0.7998128361456362523 ) ) ;
#162930=CARTESIAN_POINT ( 'NONE',  ( -4.878955176071358757, 6.785476686873604280, -1.599625672291271394 ) ) ;
#162935=CARTESIAN_POINT ( 'NONE',  ( -5.367048706163331850, 7.354919138647580290, -1.599625672291271394 ) ) ;
#162947=CARTESIAN_POINT ( 'NONE',  ( -3.797165540279144214, 6.587721009371067638, 1.199719254218452935 ) ) ;
#162952=CARTESIAN_POINT ( 'NONE',  ( -6.509323148336870091, 7.727203440215372865, 1.082531754730549078 ) ) ;
#162953=CARTESIAN_POINT ( 'NONE',  ( -6.414416072596845986, 8.576847732820027659, -1.443375672974066548 ) ) ;
#162954=CARTESIAN_POINT ( 'NONE',  ( 7.095713291905693332, 9.371694488680407886, 1.599625672291268286 ) ) ;
#162955=CARTESIAN_POINT ( 'NONE',  ( -6.526270840131767059, 8.707344961610770540, -1.599625672291271394 ) ) ;
#162963=ORIENTED_EDGE ( 'NONE', *, *, #105361, .T. ) ;
#162968=ORIENTED_EDGE ( 'NONE', *, *, #46280, .T. ) ;
#162993=CARTESIAN_POINT ( 'NONE',  ( 4.597876849858236525, 8.486543085689454813, -0.1053875944492469602 ) ) ;
#163006=CARTESIAN_POINT ( 'NONE',  ( 5.840530312436913007, 10.03597880781023299, 0.000000000000000000 ) ) ;
#163009=CARTESIAN_POINT ( 'NONE',  ( -4.793689830883590020, 7.750332681742931662, 1.199719254218452935 ) ) ;
#163013=CARTESIAN_POINT ( 'NONE',  ( -6.075462232255183892, 10.10214001435745246, 0.000000000000000000 ) ) ;
#163023=CARTESIAN_POINT ( 'NONE',  ( 5.734172623936983904, 5.654565914206774124, 0.7998128361456352531 ) ) ;
#163025=CARTESIAN_POINT ( 'NONE',  ( 5.494797395288433250, 9.632623737803665875, 0.000000000000000000 ) ) ;
#163026=CARTESIAN_POINT ( 'NONE',  ( 0.4717386086568179926, 2.948512804476515647, -1.943622686712360714 ) ) ;
#163030=CARTESIAN_POINT ( 'NONE',  ( -4.848970937371709589, 4.819285127202144636, 0.1070505994550537271 ) ) ;
#163034=EDGE_LOOP ( 'NONE', ( #3858, #163064 ) ) ;
#163035=CARTESIAN_POINT ( 'NONE',  ( 3.573456005653643519, 6.326726552307992080, -1.199719254218453823 ) ) ;
#163042=CARTESIAN_POINT ( 'NONE',  ( 6.737475991348287785, 6.825086509519945999, -0.7998128361456481317 ) ) ;
#163043=ORIENTED_EDGE ( 'NONE', *, *, #6657, .T. ) ;
#163056=CARTESIAN_POINT ( 'NONE',  ( -5.234856708652269042, 7.200695141551334721, 1.443375672974058777 ) ) ;
#163057=CARTESIAN_POINT ( 'NONE',  ( 4.095971805104276164, 7.792734516014745871, 0.7216878364870257245 ) ) ;
#163064=ORIENTED_EDGE ( 'NONE', *, *, #186745, .F. ) ;
#163068=CARTESIAN_POINT ( 'NONE',  ( -4.496464221587651799, 5.274905009054215554, 1.199719254218452935 ) ) ;
#163069=CARTESIAN_POINT ( 'NONE',  ( -6.129694847154220305, 8.244672969803623630, -1.443375672974066548 ) ) ;
#163070=CARTESIAN_POINT ( 'NONE',  ( 5.826972158823246595, 10.02016096192762085, -0.7998128361456481317 ) ) ;
#163073=CARTESIAN_POINT ( 'NONE',  ( 4.380693030546913391, 7.164540064729805202, 1.082531754730549078 ) ) ;
#163090=CARTESIAN_POINT ( 'NONE',  ( 6.059568310664962709, 6.034194215389424798, 0.7998128361456352531 ) ) ;
#163092=CARTESIAN_POINT ( 'NONE',  ( -5.191846479390389568, 5.021852078902356631, 0.7998128361456281477 ) ) ;
#163105=CARTESIAN_POINT ( 'NONE',  ( 5.885648082108188461, 8.920320958217979879, 1.082531754730549967 ) ) ;
#163107=CARTESIAN_POINT ( 'NONE',  ( -4.932134020321308654, 8.976183133675331050, 0.7998128361456291469 ) ) ;
#163108=CARTESIAN_POINT ( 'NONE',  ( 5.234329823327693809, 8.264412672927770487, 1.199719254218451159 ) ) ;
#163116=CARTESIAN_POINT ( 'NONE',  ( -6.947627372360122955, 7.070263120700404968, 0.000000000000000000 ) ) ;
#163128=( BOUNDED_SURFACE ( )  B_SPLINE_SURFACE ( 3, 2, ( 
 ( #50147, #52279, #2422 ),
 ( #167104, #17612, #34940 ),
 ( #3491, #135671, #133565 ),
 ( #68499, #199571, #18691 ),
 ( #83698, #116271, #103160 ),
 ( #69561, #134627, #16550 ),
 ( #149786, #82632, #53339 ),
 ( #70625, #117339, #148717 ) ),
 .UNSPECIFIED., .F., .F., .T. ) 
 B_SPLINE_SURFACE_WITH_KNOTS ( ( 4, 2, 2, 4 ),
 ( 3, 3 ),
 ( 0.000000000000000000, 0.003135730046001663184, 0.004703595069002494342, 0.006271460092003326367 ),
 ( 0.000000000000000000, 1.000000000000000000 ),
 .UNSPECIFIED. ) 
 GEOMETRIC_REPRESENTATION_ITEM ( )  RATIONAL_B_SPLINE_SURFACE ( (
 ( 1.000000000000000000, 0.7762074382822432561, 1.000000000000000000),
 ( 1.000000000000000000, 0.7833603871961897225, 1.000000000000000000),
 ( 1.000000000000000000, 0.7921476697827543045, 1.000000000000000000),
 ( 1.000000000000000000, 0.8128220030704583765, 1.000000000000000000),
 ( 1.000000000000000000, 0.8210052159719404274, 1.000000000000000000),
 ( 1.000000000000000000, 0.8412342355964647078, 1.000000000000000000),
 ( 1.000000000000000000, 0.8534349975674863087, 1.000000000000000000),
 ( 1.000000000000000000, 0.8671614222306937014, 1.000000000000000000) ) ) 
 REPRESENTATION_ITEM ( '' )  SURFACE ( )  );
#163133=EDGE_LOOP ( 'NONE', ( #25218, #64218, #95956, #200765, #182331, #204832, #165084 ) ) ;
#163143=CARTESIAN_POINT ( 'NONE',  ( 5.560252395380222090, 5.659585014131299552, 0.7216878364870328300 ) ) ;
#163149=CARTESIAN_POINT ( 'NONE',  ( 5.411112705185558092, 6.445957923205511086, -1.082531754730548412 ) ) ;
#163161=CARTESIAN_POINT ( 'NONE',  ( -6.469175572376043348, 7.576401584974034265, 1.199719254218452047 ) ) ;
#163163=CARTESIAN_POINT ( 'NONE',  ( -7.370792787684826486, 8.628288336167626582, -1.199719254218452047 ) ) ;
#163171=CARTESIAN_POINT ( 'NONE',  ( 3.567203813726958828, 6.215469311773181182, 1.082531754730549078 ) ) ;
#163177=CARTESIAN_POINT ( 'NONE',  ( -7.110325215724114578, 7.260077271291732082, 0.000000000000000000 ) ) ;
#163183=CARTESIAN_POINT ( 'NONE',  ( -4.150204419558982671, 7.856005899545188242, 0.7216878364870338292 ) ) ;
#163187=CARTESIAN_POINT ( 'NONE',  ( -6.448838341955544173, 7.552674816150118708, 1.199719254218452047 ) ) ;
#163203=CARTESIAN_POINT ( 'NONE',  ( -6.615342224808818727, 6.750480251133849308, 0.3470571717737805373 ) ) ;
#163209=CARTESIAN_POINT ( 'NONE',  ( -7.957709816578236506, 8.248692638954882028, 0.7998128361456341429 ) ) ;
#163210=CARTESIAN_POINT ( 'NONE',  ( 4.706615602599436343, 5.520081620234675412, 1.199719254218452935 ) ) ;
#163211=CARTESIAN_POINT ( 'NONE',  ( -5.818384198920079520, 6.817144982608731141, 1.199719254218452935 ) ) ;
#163212=ORIENTED_EDGE ( 'NONE', *, *, #114761, .F. ) ;
#163220=DIRECTION ( 'NONE',  ( 0.7592566023653005702, 0.6507913734559639396, 0.000000000000000000 ) ) ;
#163225=CARTESIAN_POINT ( 'NONE',  ( -4.613268803136618246, 8.378775596900176481, 0.2107346534404584415 ) ) ;
#163235=CARTESIAN_POINT ( 'NONE',  ( -7.293360289508603600, 7.473618190706972086, 0.000000000000000000 ) ) ;
#163260=CARTESIAN_POINT ( 'NONE',  ( 6.210516883511641772, 9.403297576475722508, 1.199719254218452047 ) ) ;
#163261=CARTESIAN_POINT ( 'NONE',  ( 4.963960565410041603, 8.060099936542098220, -1.154953748940761971 ) ) ;
#163272=CARTESIAN_POINT ( 'NONE',  ( 6.162627863271451290, 6.966383021533493647, 0.9102919922300183320 ) ) ;
#163275=CARTESIAN_POINT ( 'NONE',  ( 2.891631901464575272, 6.595597328342462262, 0.000000000000000000 ) ) ;
#163279=CARTESIAN_POINT ( 'NONE',  ( -6.784929528996132220, 6.880448970109080520, 0.000000000000000000 ) ) ;
#163285=CARTESIAN_POINT ( 'NONE',  ( -7.743115126736118015, 8.206258200713163475, 0.7216878364870317197 ) ) ;
#163288=CARTESIAN_POINT ( 'NONE',  ( -5.153105136966797062, 6.602250206728904836, 1.217409160849269423 ) ) ;
#163294=CARTESIAN_POINT ( 'NONE',  ( -3.935609729716867289, 7.813571461303467913, 0.7998128361456352531 ) ) ;
#163304=CARTESIAN_POINT ( 'NONE',  ( 5.910428620914669473, 5.860197910680708944, 0.000000000000000000 ) ) ;
#163326=CARTESIAN_POINT ( 'NONE',  ( -5.901542003698421190, 10.10715911428198055, 0.000000000000000000 ) ) ;
#163331=CARTESIAN_POINT ( 'NONE',  ( -6.316227922719336974, 6.878322274790401814, 0.7073135764556655047 ) ) ;
#163338=CARTESIAN_POINT ( 'NONE',  ( 6.391743074199808916, 6.421731439513382433, -0.7998128361456481317 ) ) ;
#163341=CARTESIAN_POINT ( 'NONE',  ( -5.572146871515974986, 5.861678842484318253, -0.6761443037284958768 ) ) ;
#163346=CARTESIAN_POINT ( 'NONE',  ( 4.936577329151614180, 4.931964103531220722, -0.7216878364870458196 ) ) ;
#163350=CARTESIAN_POINT ( 'NONE',  ( 5.966997003790217136, 8.054858819212300958, -1.443375672974078761 ) ) ;
#163362=CARTESIAN_POINT ( 'NONE',  ( -5.777182853198894463, 9.754147405458438058, 0.7216878364870267237 ) ) ;
#163393=ORIENTED_EDGE ( 'NONE', *, *, #83796, .F. ) ;
#163397=CARTESIAN_POINT ( 'NONE',  ( 4.193214648376505593, 8.114110533073061404, 0.000000000000000000 ) ) ;
#163399=CARTESIAN_POINT ( 'NONE',  ( 6.710359684120930091, 6.793450817754725257, 0.7998128361456352531 ) ) ;
#163404=( LENGTH_UNIT ( ) NAMED_UNIT ( * ) SI_UNIT ( .MILLI., .METRE. ) );
#163411=CARTESIAN_POINT ( 'NONE',  ( -5.008811405605897882, 4.808311159487113073, 0.7998128361456281477 ) ) ;
#163414=CARTESIAN_POINT ( 'NONE',  ( 4.217995187182915551, 7.935095128439824563, 0.7216878364870257245 ) ) ;
#163428=CARTESIAN_POINT ( 'NONE',  ( -4.990809943606273613, 7.876343129965691858, -1.082531754730549967 ) ) ;
#163430=CARTESIAN_POINT ( 'NONE',  ( -5.153507786970275006, 7.105788066255672497, -1.443375672974066548 ) ) ;
#163437=CARTESIAN_POINT ( 'NONE',  ( -5.916355281146389089, 6.815393236815656230, -0.9995835186326230692 ) ) ;
#163456=CARTESIAN_POINT ( 'NONE',  ( -4.248501033035892327, 6.049946853332221153, -1.599625672291271394 ) ) ;
#163466=CARTESIAN_POINT ( 'NONE',  ( -6.424584688029276514, 8.588711117491191871, 1.599625672291269396 ) ) ;
#163467=CARTESIAN_POINT ( 'NONE',  ( -5.242543201390849283, 7.800132786123255002, 1.293859303942331840 ) ) ;
#163469=DIRECTION ( 'NONE',  ( -1.000000000000000000, 0.000000000000000000, 0.000000000000000000 ) ) ;
#163472=DIRECTION ( 'NONE',  ( -0.7592566023652995710, -0.6507913734559650498, 0.000000000000000000 ) ) ;
#163486=CARTESIAN_POINT ( 'NONE',  ( 6.282224075085741433, 8.422623735723785643, 1.599625672291268286 ) ) ;
#163510=CARTESIAN_POINT ( 'NONE',  ( 6.229045230835819069, 6.231917288922055320, -0.7998128361456481317 ) ) ;
#163511=CARTESIAN_POINT ( 'NONE',  ( 5.357406976055401948, 6.279338222599979424, 1.199719254218452935 ) ) ;
#163513=CARTESIAN_POINT ( 'NONE',  ( 5.551137550152489553, 5.441024994791534120, 0.7998128361456352531 ) ) ;
#163524=CARTESIAN_POINT ( 'NONE',  ( 5.084740326411086642, 7.951855545768795608, 1.193092838546747414 ) ) ;
#163526=CARTESIAN_POINT ( 'NONE',  ( -5.763624699140882157, 7.817591130454727200, -1.443375672974066548 ) ) ;
#163536=ADVANCED_FACE ( 'NONE', ( #187620 ), #75351, .T. ) ;
#163555=CARTESIAN_POINT ( 'NONE',  ( 6.364626766972446781, 6.390095747748157251, 0.7998128361456352531 ) ) ;
#163557=CARTESIAN_POINT ( 'NONE',  ( 3.223806664999388172, 6.983134552466421674, -0.7998128361456362523 ) ) ;
#163577=DIRECTION ( 'NONE',  ( -0.000000000000000000, -0.000000000000000000, 1.000000000000000000 ) ) ;
#163589=CARTESIAN_POINT ( 'NONE',  ( 5.855142236255289845, 7.924361590421551860, -1.599625672291281386 ) ) ;
#163593=CARTESIAN_POINT ( 'NONE',  ( 6.398522151006641678, 6.429640362454684954, 0.000000000000000000 ) ) ;
#163604=CARTESIAN_POINT ( 'NONE',  ( 4.675188888464441028, 8.274035074156913083, -0.5495550137140058355 ) ) ;
#163605=CARTESIAN_POINT ( 'NONE',  ( -1.806654366501805775, 2.518449987798942136, 2.500000000000000444 ) ) ;
#163618=EDGE_CURVE ( 'NONE', #2249, #104090, #81244, .T. ) ;
#163623=CARTESIAN_POINT ( 'NONE',  ( 3.607878275012313285, 6.262922849939428716, 1.082531754730549078 ) ) ;
#163628=CARTESIAN_POINT ( 'NONE',  ( -6.282224075085783177, 8.422623735723785643, 1.599625672291269396 ) ) ;
#163630=CARTESIAN_POINT ( 'NONE',  ( 5.363132282657546490, 8.414682208812571673, -1.199719254218452047 ) ) ;
#163633=CARTESIAN_POINT ( 'NONE',  ( -7.584860592202423035, 7.813701877183096833, -0.7998128361456362523 ) ) ;
#163640=CARTESIAN_POINT ( 'NONE',  ( 6.966220764712121927, 6.002124920821316323, 2.420000000000000373 ) ) ;
#163642=CARTESIAN_POINT ( 'NONE',  ( -0.1240337052346596886, 2.520685617421167368, -1.998971434602998087 ) ) ;
#163658=CARTESIAN_POINT ( 'NONE',  ( 6.875393295905841917, 7.193916064744513506, 0.000000000000000000 ) ) ;
#163661=CARTESIAN_POINT ( 'NONE',  ( -6.994027139803241866, 9.253060644560830994, -1.599625672291271394 ) ) ;
#163673=CARTESIAN_POINT ( 'NONE',  ( -4.502716413514310290, 6.346531463890372926, -1.443375672974066548 ) ) ;
#163675=CARTESIAN_POINT ( 'NONE',  ( 6.900173834712277632, 7.014900660111269559, -0.7998128361456341429 ) ) ;
#163689=ORIENTED_EDGE ( 'NONE', *, *, #138377, .T. ) ;
#163724=CARTESIAN_POINT ( 'NONE',  ( 4.848976215542928792, 5.686169002002086970, 1.199719254218452047 ) ) ;
#163728=CARTESIAN_POINT ( 'NONE',  ( -4.733205024502264102, 7.575804057677677505, 1.082531754730549967 ) ) ;
#163735=CARTESIAN_POINT ( 'NONE',  ( -5.798046968499580345, 6.793418213784815585, 1.199719254218452935 ) ) ;
#163743=CARTESIAN_POINT ( 'NONE',  ( 7.506374323821472849, 8.786466794993730289, -1.199719254218452047 ) ) ;
#163744=CARTESIAN_POINT ( 'NONE',  ( -5.550083779947821760, 7.568460058062819407, -1.599625672291271394 ) ) ;
#163747=CARTESIAN_POINT ( 'NONE',  ( 6.333059215844621725, 6.948315255594014417, 0.8781869475623119703 ) ) ;
#163752=CARTESIAN_POINT ( 'NONE',  ( 5.505492895601038938, 8.580769590579979678, -1.199719254218452047 ) ) ;
#163762=CARTESIAN_POINT ( 'NONE',  ( -3.955946960137363799, 7.837298230127379917, 0.7998128361456352531 ) ) ;
#163766=CARTESIAN_POINT ( 'NONE',  ( -6.424584688029276514, 8.588711117491191871, 1.599625672291269396 ) ) ;
#163770=CARTESIAN_POINT ( 'NONE',  ( 5.519577934094840543, 9.453608333170423705, 0.7216878364870317197 ) ) ;
#163772=CARTESIAN_POINT ( 'NONE',  ( -5.600926855776877211, 9.548515408466085930, -0.7216878364870338292 ) ) ;
#163778=CARTESIAN_POINT ( 'NONE',  ( 4.505052181490820651, 8.477920988373101707, -0.7998128361456381397 ) ) ;
#163787=CARTESIAN_POINT ( 'NONE',  ( -3.615586099537422271, 3.576626764850541651, -2.500000000000000444 ) ) ;
#163804=CARTESIAN_POINT ( 'NONE',  ( 5.051181283347249362, 7.973588670567067105, -1.225461877896296681 ) ) ;
#163816=CARTESIAN_POINT ( 'NONE',  ( 6.481679955784983349, 9.719654494127929922, -1.199719254218452047 ) ) ;
#163822=CARTESIAN_POINT ( 'NONE',  ( -5.902949979233523159, 7.165898849449257924, -1.132310321155009847 ) ) ;
#163840=CARTESIAN_POINT ( 'NONE',  ( -6.050681693448748177, 10.28115541899069463, 0.7998128361456291469 ) ) ;
#163852=CARTESIAN_POINT ( 'NONE',  ( 3.854260808034858155, 7.718664386007802136, -0.7998128361456362523 ) ) ;
#163855=CARTESIAN_POINT ( 'NONE',  ( 6.983858524370782916, 7.320458831286981827, 0.7216878364870328300 ) ) ;
#163863=CARTESIAN_POINT ( 'NONE',  ( 5.602074566136501232, 5.729665287594564838, 0.6253354971682704155 ) ) ;
#163868=EDGE_CURVE ( 'NONE', #52032, #47959, #174103, .T. ) ;
#163871=CARTESIAN_POINT ( 'NONE',  ( -4.261005416444848315, 8.193199762486115034, 0.7998128361456352531 ) ) ;
#163872=CARTESIAN_POINT ( 'NONE',  ( 3.555981428534177091, 7.370671776590375757, 0.7998128361456271485 ) ) ;
#163885=CARTESIAN_POINT ( 'NONE',  ( -6.668631453075260396, 8.873432343378178544, -1.599625672291271394 ) ) ;
#163886=CARTESIAN_POINT ( 'NONE',  ( 5.182959862174088883, 9.268813282503625572, 0.7998128361456331437 ) ) ;
#163888=CARTESIAN_POINT ( 'NONE',  ( 0.000000000000000000, 6.062865449010541141, 0.000000000000000000 ) ) ;
#163892=CARTESIAN_POINT ( 'NONE',  ( 5.388439706788500594, 5.251210844200210559, 0.7998128361456352531 ) ) ;
#163899=CARTESIAN_POINT ( 'NONE',  ( -6.329738897986983304, 6.948428204275519882, 0.9008771187248975076 ) ) ;
#163907=CARTESIAN_POINT ( 'NONE',  ( -3.594320120954326292, 6.247105003538398371, 1.082531754730549967 ) ) ;
#163908=CARTESIAN_POINT ( 'NONE',  ( -4.841670253411603397, 5.781608396135871075, 1.082531754730549078 ) ) ;
#163918=CARTESIAN_POINT ( 'NONE',  ( -5.398914348987532641, 6.259949555863199677, -2.420000000000000373 ) ) ;
#163949=ORIENTED_EDGE ( 'NONE', *, *, #36816, .F. ) ;
#163956=CARTESIAN_POINT ( 'NONE',  ( 6.021229618244865023, 10.03886863134542828, -0.7216878364870458196 ) ) ;
#163971=DIRECTION ( 'NONE',  ( 1.000000000000000000, 0.000000000000000000, 0.000000000000000000 ) ) ;
#163985=CARTESIAN_POINT ( 'NONE',  ( -4.118644803501354978, 8.027112380718707030, 0.7998128361456352531 ) ) ;
#163987=CARTESIAN_POINT ( 'NONE',  ( 5.492461626867537916, 9.421972641405202964, -0.7216878364870458196 ) ) ;
#163992=CARTESIAN_POINT ( 'NONE',  ( -7.130662446144611977, 7.283804040115648526, 0.000000000000000000 ) ) ;
#164000=CARTESIAN_POINT ( 'NONE',  ( -5.855142236255304944, 7.924361590421551860, -1.599625672291271394 ) ) ;
#164010=EDGE_CURVE ( 'NONE', #13120, #137516, #91396, .T. ) ;
#164013=CARTESIAN_POINT ( 'NONE',  ( -5.635349125135588721, 6.603604063193491136, 1.199719254218452935 ) ) ;
#164018=CARTESIAN_POINT ( 'NONE',  ( -5.628043163448566588, 9.580151100749725757, 0.000000000000000000 ) ) ;
#164020=CARTESIAN_POINT ( 'NONE',  ( -7.119440060507479018, 8.439006504414422238, 1.082531754730549078 ) ) ;
#164021=CARTESIAN_POINT ( 'NONE',  ( 5.338878628731272613, 9.450718510153643948, -0.7998128361456481317 ) ) ;
#164022=CARTESIAN_POINT ( 'NONE',  ( -7.228432174741334038, 8.462200954400218578, -1.199719254218452047 ) ) ;
#164038=FACE_OUTER_BOUND ( 'NONE', #208327, .T. ) ;
#164043=CARTESIAN_POINT ( 'NONE',  ( 6.472394699177205446, 6.854181287346997387, 0.6349317888264572884 ) ) ;
#164060=CARTESIAN_POINT ( 'NONE',  ( 6.492506472431533560, 6.747478052702773788, -0.04572756507489894595 ) ) ;
#164074=CARTESIAN_POINT ( 'NONE',  ( 7.713663051532233972, 7.963971413067895355, -0.7998128361456341429 ) ) ;
#164077=CARTESIAN_POINT ( 'NONE',  ( -5.991777542596674166, 5.955104985976372944, 0.000000000000000000 ) ) ;
#164090=CARTESIAN_POINT ( 'NONE',  ( 4.817943484809818600, 6.714296380401858499, 1.599625672291269396 ) ) ;
#164092=CARTESIAN_POINT ( 'NONE',  ( 6.210516883511641772, 9.403297576475722508, 1.199719254218452047 ) ) ;
#164097=CARTESIAN_POINT ( 'NONE',  ( -5.926322542504864899, 8.967774495347393682, -1.082531754730549967 ) ) ;
#164104=CARTESIAN_POINT ( 'NONE',  ( 5.854088466050551887, 10.05179665369283981, 0.7998128361456341429 ) ) ;
#164118=CARTESIAN_POINT ( 'NONE',  ( -7.268579750702168774, 7.652633595340216921, -0.7216878364870338292 ) ) ;
#164119=CARTESIAN_POINT ( 'NONE',  ( 4.855228407469603269, 7.718164671139588151, -1.082531754730548412 ) ) ;
#164130=CARTESIAN_POINT ( 'NONE',  ( -5.289089323106922258, 9.184704953684462936, 0.7216878364870267237 ) ) ;
#164135=CARTESIAN_POINT ( 'NONE',  ( 3.879041346841291649, 7.539648981374564407, 1.040834085586084257E-14 ) ) ;
#164150=CARTESIAN_POINT ( 'NONE',  ( -5.113360211009450040, 5.994616996712990975, -1.199719254218453823 ) ) ;
#164163=CARTESIAN_POINT ( 'NONE',  ( 4.065465959251388206, 5.836405933916976707, -1.599625672291269396 ) ) ;
#164165=CARTESIAN_POINT ( 'NONE',  ( -5.824109505522200081, 8.952488968821326054, -1.199719254218452047 ) ) ;
#164166=CARTESIAN_POINT ( 'NONE',  ( 5.017399365509065845, 8.011327138806002779, -1.199719254218450271 ) ) ;
#164175=CARTESIAN_POINT ( 'NONE',  ( -6.784929528996132220, 6.880448970109080520, 0.000000000000000000 ) ) ;
#164199=CARTESIAN_POINT ( 'NONE',  ( 5.072158865288243668, 6.050511776658669127, 1.082531754730549078 ) ) ;
#164201=ORIENTED_EDGE ( 'NONE', *, *, #195731, .T. ) ;
#164206=CARTESIAN_POINT ( 'NONE',  ( 6.183927461164522299, 6.387205924212962849, 0.000000000000000000 ) ) ;
#164218=CARTESIAN_POINT ( 'NONE',  ( -4.932134020321308654, 8.976183133675331050, 0.7998128361456291469 ) ) ;
#164220=CARTESIAN_POINT ( 'NONE',  ( -5.738844160334429567, 9.917344963690652548, 0.000000000000000000 ) ) ;
#164226=CARTESIAN_POINT ( 'NONE',  ( 6.230854113932139171, 9.427024345299638952, 1.199719254218452047 ) ) ;
#164231=CARTESIAN_POINT ( 'NONE',  ( -5.608470646763013434, 5.608483241851182299, 0.4208904006049640767 ) ) ;
#164232=CARTESIAN_POINT ( 'NONE',  ( -6.454563648557663846, 9.688018802362710957, -1.199719254218452047 ) ) ;
#164238=CARTESIAN_POINT ( 'NONE',  ( -4.990809943606273613, 7.876343129965691858, -1.082531754730549967 ) ) ;
#164241=CARTESIAN_POINT ( 'NONE',  ( -6.934069218746458318, 7.054445274817795486, -0.7998128361456362523 ) ) ;
#164262=VERTEX_POINT ( 'NONE', #135862 ) ;
#164263=CARTESIAN_POINT ( 'NONE',  ( -7.014364370223741929, 9.276787413384745662, -1.599625672291271394 ) ) ;
#164264=CARTESIAN_POINT ( 'NONE',  ( 4.492547798081839794, 6.334668079219206049, 1.599625672291262513 ) ) ;
#164265=CARTESIAN_POINT ( 'NONE',  ( -6.954406449166956605, 7.078172043641714595, -0.7998128361456362523 ) ) ;
#164278=LINE ( 'NONE', #15868, #110414 ) ;
#164290=CARTESIAN_POINT ( 'NONE',  ( -7.306918443122272677, 7.489436036589583345, 0.7998128361456341429 ) ) ;
#164315=CARTESIAN_POINT ( 'NONE',  ( 4.435452530326143616, 5.203724702582467998, -1.199719254218452047 ) ) ;
#164329=CARTESIAN_POINT ( 'NONE',  ( 4.746850994788568201, 8.189453717816405742, 0.7312505120831546135 ) ) ;
#164331=CARTESIAN_POINT ( 'NONE',  ( 7.349928672384119288, 8.707909884937221179, 1.082531754730549967 ) ) ;
#164338=CARTESIAN_POINT ( 'NONE',  ( -5.906512197408906317, 6.919960980845699439, -1.199719254218453823 ) ) ;
#164343=CARTESIAN_POINT ( 'NONE',  ( -7.905812970100109638, 8.396072351304486148, 0.7216878364870317197 ) ) ;
#164349=CARTESIAN_POINT ( 'NONE',  ( -4.344821003001812620, 7.342528190309904446, 0.9996755505292649335 ) ) ;
#164356=CARTESIAN_POINT ( 'NONE',  ( -4.098307573080856692, 8.003385611894792362, 0.7998128361456352531 ) ) ;
#164365=EDGE_CURVE ( 'NONE', #110637, #95923, #7250, .T. ) ;
#164367=CARTESIAN_POINT ( 'NONE',  ( 5.411639590510088027, 6.342609606130419131, -1.199719254218452047 ) ) ;
#164376=ORIENTED_EDGE ( 'NONE', *, *, #103129, .F. ) ;
#164387=CARTESIAN_POINT ( 'NONE',  ( -7.587723245503481095, 8.881373870289390737, 1.199719254218452047 ) ) ;
#164390=CARTESIAN_POINT ( 'NONE',  ( 5.969332771766739931, 10.18624834369502885, -0.7998128361456481317 ) ) ;
#164398=CARTESIAN_POINT ( 'NONE',  ( 4.366607992053101128, 7.252070536440704096, -1.199719254218448494 ) ) ;
#164399=FACE_OUTER_BOUND ( 'NONE', #28469, .T. ) ;
#164404=CARTESIAN_POINT ( 'NONE',  ( 3.933273961740296087, 6.642551151122080277, 1.082531754730549078 ) ) ;
#164407=CARTESIAN_POINT ( 'NONE',  ( 7.214347136247488912, 7.589362211809770997, -0.7216878364870317197 ) ) ;
#164418=CARTESIAN_POINT ( 'NONE',  ( -5.465345320084574965, 9.390336950158399532, 0.000000000000000000 ) ) ;
#164452=CARTESIAN_POINT ( 'NONE',  ( 4.694866332082116678, 8.699370830729650450, 0.7998128361456341429 ) ) ;
#164453=CARTESIAN_POINT ( 'NONE',  ( -4.285785955251283141, 8.014184357852876417, 0.000000000000000000 ) ) ;
#164454=CARTESIAN_POINT ( 'NONE',  ( 5.200434439293556643, 8.224868058221247225, -1.199719254218452047 ) ) ;
#164467=CARTESIAN_POINT ( 'NONE',  ( -2.810282979782591006, 6.500690253046801814, 0.000000000000000000 ) ) ;
#164470=CARTESIAN_POINT ( 'NONE',  ( 5.112833325684902341, 7.058334528089426740, -1.443375672974078761 ) ) ;
#164483=CARTESIAN_POINT ( 'NONE',  ( -5.966997003790221576, 9.015228033513643879, -1.082531754730549967 ) ) ;
#164485=CARTESIAN_POINT ( 'NONE',  ( -5.804299160426249493, 5.944306240018289778, -0.7216878364870338292 ) ) ;
#164497=EDGE_CURVE ( 'NONE', #35662, #38381, #26747, .T. ) ;
#164514=CARTESIAN_POINT ( 'NONE',  ( -4.197131071882288289, 7.054347462908075350, -1.199719254218455378 ) ) ;
#164521=CARTESIAN_POINT ( 'NONE',  ( -5.649528891068317016, 5.555814892526615090, 0.2055412888010339778 ) ) ;
#164523=CARTESIAN_POINT ( 'NONE',  ( -7.435720902452096936, 7.639705572474380091, 0.000000000000000000 ) ) ;
#164524=CARTESIAN_POINT ( 'NONE',  ( -5.747140441703231240, 7.374164810257596514, -1.320148062302946013 ) ) ;
#164543=CARTESIAN_POINT ( 'NONE',  ( 5.794130544993763898, 7.853181283949808744, 1.599625672291269396 ) ) ;
#164566=CARTESIAN_POINT ( 'NONE',  ( 7.340813827156391191, 7.528980651296110160, 0.7998128361456281477 ) ) ;
#164567=CARTESIAN_POINT ( 'NONE',  ( 5.712781623311797397, 7.758274208654143855, -1.599625672291283607 ) ) ;
#164569=CARTESIAN_POINT ( 'NONE',  ( 5.890091390494168522, 5.836471141856793388, 0.000000000000000000 ) ) ;
#164572=CARTESIAN_POINT ( 'NONE',  ( -2.713063801223519089, 3.002997225240221280, -2.500000000000000444 ) ) ;
#164581=CARTESIAN_POINT ( 'NONE',  ( 4.893454165248502186, 8.027304163657891678, -0.9628252682179049282 ) ) ;
#164582=CARTESIAN_POINT ( 'NONE',  ( -5.655159470231558849, 6.730679149092498648, 1.082531754730549078 ) ) ;
#164583=CARTESIAN_POINT ( 'NONE',  ( 3.418064124421011041, 7.001842221884225559, -0.7216878364870338292 ) ) ;
#164610=CARTESIAN_POINT ( 'NONE',  ( 5.448397627845284141, 7.449826213943242514, 1.599625672291268286 ) ) ;
#164612=CARTESIAN_POINT ( 'NONE',  ( 5.246079093845007257, 5.085123462432798114, 0.7998128361456352531 ) ) ;
#164641=CARTESIAN_POINT ( 'NONE',  ( 6.378184920586140727, 6.405913593630768510, 0.000000000000000000 ) ) ;
#164646=CARTESIAN_POINT ( 'NONE',  ( -6.497792602234238934, 6.760263899176822022, -0.1076752790035370722 ) ) ;
#164647=CARTESIAN_POINT ( 'NONE',  ( 7.049313524462606395, 7.188896964819984525, 0.000000000000000000 ) ) ;
#164658=CARTESIAN_POINT ( 'NONE',  ( 4.611577566919329740, 8.352668595566711929, -0.2595669225248058432 ) ) ;
#164679=CARTESIAN_POINT ( 'NONE',  ( -6.149505192250180663, 9.332117270003974951, -1.199719254218452047 ) ) ;
#164681=CARTESIAN_POINT ( 'NONE',  ( 7.035755370848908896, 7.173079118937375931, 0.7998128361456352531 ) ) ;
#164682=DIRECTION ( 'NONE',  ( -0.6507913734559640506, -0.7592566023653003482, 0.000000000000000000 ) ) ;
#164684=B_SPLINE_CURVE_WITH_KNOTS ( 'NONE', 3,
 ( #13072, #79151, #46674, #145268, #211275, #62898, #162556, #214410, #44547, #129068, #12013, #110662, #82341, #94368, #131172, #112794, #30421, #96506, #213395, #146319, #212334, #63972, #130128, #66065, #192890, #144211, #47753, #15201, #113868, #179863, #176663 ),
 .UNSPECIFIED., .F., .F.,
 ( 4, 2, 2, 2, 2, 2, 2, 2, 2, 2, 2, 2, 1, 2, 2, 4 ),
 ( 0.1193258592806614310, 0.1284789785326313494, 0.1376320977846012539, 0.1422086574105862200, 0.1467852170365712139, 0.1559383362885412294, 0.1582266161015338513, 0.1605148959145265009, 0.1650914555405115225, 0.1696680151664965996, 0.1708121550729926885, 0.1719562949794887774, 0.1742445747924811217, 0.1833976940444502213, 0.1879742536704346878, 0.1925508132964191543 ),
 .UNSPECIFIED. ) ;
#164692=CARTESIAN_POINT ( 'NONE',  ( -6.402982088906444602, 6.898597865962027065, -0.7910698893406533649 ) ) ;
#164708=CARTESIAN_POINT ( 'NONE',  ( 6.888951449519509218, 7.209733910627123876, -0.7216878364870317197 ) ) ;
#164721=CARTESIAN_POINT ( 'NONE',  ( -4.828112100242294424, 5.765790550771681566, -1.082531754730549967 ) ) ;
#164723=CARTESIAN_POINT ( 'NONE',  ( 6.119526231721748033, 8.232809585132461194, 1.599625672291269396 ) ) ;
#164728=CARTESIAN_POINT ( 'NONE',  ( -3.494969737272722643, 7.299491470118629088, -0.7998128361456481317 ) ) ;
#164739=CARTESIAN_POINT ( 'NONE',  ( -5.194182247366913252, 7.153241603385088965, 1.443375672974058777 ) ) ;
#164776=CARTESIAN_POINT ( 'NONE',  ( 5.239300017038202917, 5.077214539491492928, 0.000000000000000000 ) ) ;
#164781=CARTESIAN_POINT ( 'NONE',  ( -3.784134271545645412, 7.428924060196286483, 0.7216878364870338292 ) ) ;
#164786=EDGE_LOOP ( 'NONE', ( #203356, #212537, #29864, #87394 ) ) ;
#164787=CARTESIAN_POINT ( 'NONE',  ( -7.611976899429754084, 7.845337568948314022, 0.7998128361456341429 ) ) ;
#164792=CARTESIAN_POINT ( 'NONE',  ( 4.743677682280330821, 4.888648074256856546, -0.7989307584942272333 ) ) ;
#164793=CARTESIAN_POINT ( 'NONE',  ( 5.969332771766739931, 10.18624834369502885, -0.7998128361456481317 ) ) ;
#164795=CARTESIAN_POINT ( 'NONE',  ( -5.631432701629818460, 7.663367133358481631, 1.599625672291263179 ) ) ;
#164798=CARTESIAN_POINT ( 'NONE',  ( 5.820234798683411981, 7.319712794923219690, 1.284739950006764220 ) ) ;
#164803=CARTESIAN_POINT ( 'NONE',  ( 5.830888582329017744, 8.960397891762626799, -1.199719254218452047 ) ) ;
#164811=CARTESIAN_POINT ( 'NONE',  ( -3.644109427023046521, 7.473487774827342278, 0.000000000000000000 ) ) ;
#164815=CARTESIAN_POINT ( 'NONE',  ( -7.286581212701773502, 7.465709267765667789, 0.7998128361456341429 ) ) ;
#164820=CARTESIAN_POINT ( 'NONE',  ( 7.485510208076452621, 7.905719128943566432, 0.000000000000000000 ) ) ;
#164822=CARTESIAN_POINT ( 'NONE',  ( -6.414416072596845986, 8.576847732820027659, -1.443375672974066548 ) ) ;
#164829=CARTESIAN_POINT ( 'NONE',  ( 5.182959862174088883, 9.268813282503625572, 0.7998128361456331437 ) ) ;
#164830=ORIENTED_EDGE ( 'NONE', *, *, #31247, .T. ) ;
#164847=CARTESIAN_POINT ( 'NONE',  ( -5.606595252507366567, 5.572856915785063592, -0.3451608010808376870 ) ) ;
#164868=CARTESIAN_POINT ( 'NONE',  ( -6.146561906247310247, 6.992958819738270826, -0.9370148970899976337 ) ) ;
#164887=CARTESIAN_POINT ( 'NONE',  ( -3.492107083971660586, 6.231819477012331632, 1.199719254218452935 ) ) ;
#164900=CARTESIAN_POINT ( 'NONE',  ( 5.879395890181562834, 6.888325289080478697, -1.199719254218452047 ) ) ;
#164903=CARTESIAN_POINT ( 'NONE',  ( 7.173672674962134899, 7.541908673643526129, -0.7216878364870317197 ) ) ;
#164917=CARTESIAN_POINT ( 'NONE',  ( -6.310394152517827315, 6.326824364217716656, 0.7998128361456281477 ) ) ;
#164918=CARTESIAN_POINT ( 'NONE',  ( 4.095444919779759552, 6.935713618788495793, 1.199719254218451159 ) ) ;
#164928=CARTESIAN_POINT ( 'NONE',  ( -7.262327558775498737, 8.501745569106741840, 1.199719254218452047 ) ) ;
#164929=CARTESIAN_POINT ( 'NONE',  ( 5.855142236255289845, 7.924361590421551860, -1.599625672291281386 ) ) ;
#164936=CARTESIAN_POINT ( 'NONE',  ( 3.691562964670865199, 7.528850235416478576, -0.7998128361456362523 ) ) ;
#164943=CARTESIAN_POINT ( 'NONE',  ( -5.739830873228516595, 7.379802178037835780, 1.322642659050039970 ) ) ;
#164953=CARTESIAN_POINT ( 'NONE',  ( -7.095713291905736853, 9.371694488680407886, 1.599625672291269396 ) ) ;
#164973=CARTESIAN_POINT ( 'NONE',  ( -6.194862797504346652, 7.033616388598824543, -1.131386643195183339 ) ) ;
#164984=CARTESIAN_POINT ( 'NONE',  ( 4.603875680292229156, 7.528882839386387360, 1.199719254218452047 ) ) ;
#165002=CARTESIAN_POINT ( 'NONE',  ( 5.727393547130178675, 5.646656991265468939, 0.000000000000000000 ) ) ;
#165003=CARTESIAN_POINT ( 'NONE',  ( -3.526529353330355221, 6.168015774643768268, -1.082531754730546636 ) ) ;
#165031=EDGE_LOOP ( 'NONE', ( #149413, #65798, #178396, #108935 ) ) ;
#165032=CARTESIAN_POINT ( 'NONE',  ( -5.631432701629818460, 7.663367133358481631, 1.599625672291263179 ) ) ;
#165034=CARTESIAN_POINT ( 'NONE',  ( 5.004368096775565711, 8.852530189631227842, -0.7216878364870458196 ) ) ;
#165039=CARTESIAN_POINT ( 'NONE',  ( -7.442499979258930587, 7.647614495415686164, -0.7998128361456362523 ) ) ;
#165046=ORIENTED_EDGE ( 'NONE', *, *, #189556, .F. ) ;
#165049=CARTESIAN_POINT ( 'NONE',  ( -7.435720902452096936, 7.639705572474380091, 0.000000000000000000 ) ) ;
#165056=CARTESIAN_POINT ( 'NONE',  ( 6.447401996410142999, 6.870587565654037832, 0.7192207954679635806 ) ) ;
#165061=CARTESIAN_POINT ( 'NONE',  ( -5.448397627845328550, 7.449826213943242514, 1.599625672291263179 ) ) ;
#165065=CARTESIAN_POINT ( 'NONE',  ( -6.075462232699549325, 9.141770800574526845, 1.082531754730549967 ) ) ;
#165068=CARTESIAN_POINT ( 'NONE',  ( -6.495764994278840021, 8.671754808115688107, 1.443375672974064550 ) ) ;
#165069=CARTESIAN_POINT ( 'NONE',  ( 5.677832469072920496, 9.846164657218904992, 0.000000000000000000 ) ) ;
#165070=CARTESIAN_POINT ( 'NONE',  ( -5.935437387732586778, 10.14670372898850381, -0.7998128361456362523 ) ) ;
#165072=ORIENTED_EDGE ( 'NONE', *, *, #128175, .F. ) ;
#165084=ORIENTED_EDGE ( 'NONE', *, *, #129354, .F. ) ;
#165091=CARTESIAN_POINT ( 'NONE',  ( 6.257994703896152089, 7.000112715747270009, 0.9732540237740094913 ) ) ;
#165109=CARTESIAN_POINT ( 'NONE',  ( 5.528015674651411970, 7.440572265265038787, -1.248273786418591103 ) ) ;
#165123=CARTESIAN_POINT ( 'NONE',  ( 7.550965208168244125, 7.774157262476569130, -0.7998128361456341429 ) ) ;
#165126=CARTESIAN_POINT ( 'NONE',  ( -5.330290668828105538, 6.247702530834755130, 1.199719254218452935 ) ) ;
#165140=CARTESIAN_POINT ( 'NONE',  ( 5.574337433874081427, 6.532423756721743580, -1.199719254218452047 ) ) ;
#165142=CARTESIAN_POINT ( 'NONE',  ( 6.180537922983273091, 8.303989891604203422, -1.599625672291281386 ) ) ;
#165148=CARTESIAN_POINT ( 'NONE',  ( -6.089020385868862739, 8.197219431637373432, -1.443375672974066548 ) ) ;
#165154=CARTESIAN_POINT ( 'NONE',  ( 8.174640274396848483, 8.501778173076651512, 0.7998128361456291469 ) ) ;
#165165=CARTESIAN_POINT ( 'NONE',  ( -5.316205630334255972, 8.255971431148344308, -1.082531754730549967 ) ) ;
#165166=CARTESIAN_POINT ( 'NONE',  ( 4.421367491832268293, 7.211993602896056288, 1.082531754730549078 ) ) ;
#165177=CARTESIAN_POINT ( 'NONE',  ( -3.851398154733808088, 6.650992392901508232, -1.199719254218450271 ) ) ;
#165178=CARTESIAN_POINT ( 'NONE',  ( -7.160114521792834807, 8.486460042580672436, 1.082531754730549078 ) ) ;
#165179=CARTESIAN_POINT ( 'NONE',  ( 7.635176783151273128, 8.936736330878529699, 1.199719254218452935 ) ) ;
#165183=CARTESIAN_POINT ( 'NONE',  ( 5.695833931072550094, 5.817763472438987726, 0.000000000000000000 ) ) ;
#165185=ORIENTED_EDGE ( 'NONE', *, *, #136789, .T. ) ;
#165194=AXIS2_PLACEMENT_3D ( 'NONE', #157494, #58910, #9088 ) ;
#165201=DIRECTION ( 'NONE',  ( -0.000000000000000000, -0.000000000000000000, 1.000000000000000000 ) ) ;
#165203=CARTESIAN_POINT ( 'NONE',  ( -5.679940009482361774, 5.591294530676332641, 0.7998128361456281477 ) ) ;
#165215=CARTESIAN_POINT ( 'NONE',  ( 2.905190055078214595, 6.611415174225076186, 0.7998128361456271485 ) ) ;
#165218=CARTESIAN_POINT ( 'NONE',  ( 4.692003678781083487, 7.631698837623355658, -1.199719254218450271 ) ) ;
#165250=CARTESIAN_POINT ( 'NONE',  ( 5.495418255317095380, 6.026204583819558813, -0.7979391942483995415 ) ) ;
#165253=CARTESIAN_POINT ( 'NONE',  ( 3.757017964762656703, 7.397288368949487491, -1.734723475976807094E-15 ) ) ;
#165259=CARTESIAN_POINT ( 'NONE',  ( 5.533136087708556694, 5.627949321847663278, 0.000000000000000000 ) ) ;
#165266=EDGE_CURVE ( 'NONE', #109313, #150264, #60158, .T. ) ;
#165273=CARTESIAN_POINT ( 'NONE',  ( -6.089547271193396227, 7.133501900260939443, -1.199719254218453823 ) ) ;
#165282=CARTESIAN_POINT ( 'NONE',  ( 6.013923656113508542, 9.173938811177871244, -1.199719254218452047 ) ) ;
#165287=CARTESIAN_POINT ( 'NONE',  ( -5.608757509019071996, 5.629766575911039794, 0.4613631940431175416 ) ) ;
#165288=CARTESIAN_POINT ( 'NONE',  ( -7.774674742793745708, 8.035151719539642912, 0.7998128361456341429 ) ) ;
#165294=CARTESIAN_POINT ( 'NONE',  ( -5.316205630334255972, 8.255971431148344308, -1.082531754730549967 ) ) ;
#165297=CARTESIAN_POINT ( 'NONE',  ( -7.096767062110449942, 7.244259425409119046, -0.7998128361456362523 ) ) ;
#165317=CARTESIAN_POINT ( 'NONE',  ( -4.095971805104331231, 5.871996087412059140, 1.443375672974065660 ) ) ;
#165318=EDGE_CURVE ( 'NONE', #111999, #154266, #204842, .T. ) ;
#165320=CARTESIAN_POINT ( 'NONE',  ( -5.908321080505254841, 10.11506803722328129, 0.7998128361456291469 ) ) ;
#165321=CARTESIAN_POINT ( 'NONE',  ( 3.074666975249065626, 6.809138247757705820, 0.000000000000000000 ) ) ;
#165322=CARTESIAN_POINT ( 'NONE',  ( -5.981082042284069367, 7.006959133200059142, 1.199719254218452935 ) ) ;
#165340=CARTESIAN_POINT ( 'NONE',  ( -6.966220764712169000, 6.002124920821316323, -2.500000000000000444 ) ) ;
#165346=CARTESIAN_POINT ( 'NONE',  ( 5.085343294144600179, 4.914812813773358435, 0.1758235994440172922 ) ) ;
#165374=CARTESIAN_POINT ( 'NONE',  ( 5.096939404094710468, 4.911127157724081371, 0.000000000000000000 ) ) ;
#165386=CARTESIAN_POINT ( 'NONE',  ( 4.720979226589129496, 8.219560628541461966, -0.6735110442024627719 ) ) ;
#165388=CARTESIAN_POINT ( 'NONE',  ( 4.309512724297349884, 6.121127159803966933, 1.599625672291261402 ) ) ;
#165393=CARTESIAN_POINT ( 'NONE',  ( -4.936050443827081580, 7.916420063510339666, 1.199719254218452935 ) ) ;
#165399=B_SPLINE_CURVE_WITH_KNOTS ( 'NONE', 3,
 ( #82413, #184177, #183118, #100797, #4336, #201476, #118188, #2202, #197231, #180987 ),
 .UNSPECIFIED., .F., .F.,
 ( 4, 2, 2, 2, 4 ),
 ( 0.001497391484644590995, 0.001840867574616280060, 0.002184343664587968907, 0.002527819754559657971, 0.002871295844531347036 ),
 .UNSPECIFIED. ) ;
#165401=CARTESIAN_POINT ( 'NONE',  ( -7.566859129758459979, 8.000626204239226880, 0.000000000000000000 ) ) ;
#165405=CARTESIAN_POINT ( 'NONE',  ( -4.001001215408780176, 7.681935780300273464, 0.003373008766155432755 ) ) ;
#165409=CARTESIAN_POINT ( 'NONE',  ( 6.726253606155519371, 7.019919760035800316, -0.7216878364870458196 ) ) ;
#165412=CARTESIAN_POINT ( 'NONE',  ( -5.204350862799341115, 7.165104988056252289, -1.599625672291271394 ) ) ;
#165423=CARTESIAN_POINT ( 'NONE',  ( 4.115782150200256950, 6.959440387612411349, 1.199719254218452047 ) ) ;
#165440=CARTESIAN_POINT ( 'NONE',  ( 6.391719935120313778, 6.567462711928209629, -2.438448603877958476 ) ) ;
#165454=CARTESIAN_POINT ( 'NONE',  ( 4.993145711582793744, 9.047363440147082159, -0.7998128361456481317 ) ) ;
#165461=CARTESIAN_POINT ( 'NONE',  ( 5.560252395380222090, 5.659585014131299552, 0.7216878364870328300 ) ) ;
#165465=CARTESIAN_POINT ( 'NONE',  ( 7.363486825997814123, 7.763358516518489516, 0.000000000000000000 ) ) ;
#165477=CARTESIAN_POINT ( 'NONE',  ( -6.617788377246196951, 7.853746207276256719, -1.082531754730549967 ) ) ;
#165490=AXIS2_PLACEMENT_3D ( 'NONE', #115996, #181984, #99686 ) ;
#165496=B_SPLINE_CURVE_WITH_KNOTS ( 'NONE', 3,
 ( #214276, #213241, #166649, #47590, #197008, #200188, #97402, #15037, #81129, #131016 ),
 .UNSPECIFIED., .F., .F.,
 ( 4, 3, 3, 4 ),
 ( 3.001204002259073297E-18, 8.735586674212287715E-05, 0.0001834092658857657617, 0.0002312911391078497833 ),
 .UNSPECIFIED. ) ;
#165514=CARTESIAN_POINT ( 'NONE',  ( 6.866278450678116485, 6.975356045404744521, 0.000000000000000000 ) ) ;
#165516=CARTESIAN_POINT ( 'NONE',  ( 4.389807875774629942, 8.343469298370917997, 0.7998128361456271485 ) ) ;
#165530=CARTESIAN_POINT ( 'NONE',  ( -7.946487431385463651, 8.443525889470736345, 0.7216878364870317197 ) ) ;
#165533=CARTESIAN_POINT ( 'NONE',  ( 5.736508391913541338, 6.825586224388162648, -1.082531754730548412 ) ) ;
#165541=CARTESIAN_POINT ( 'NONE',  ( -3.298376509874564988, 7.070132704820777825, 0.000000000000000000 ) ) ;
#165547=CARTESIAN_POINT ( 'NONE',  ( -7.295696057929500711, 7.684269287105433222, 0.7216878364870317197 ) ) ;
#165549=CARTESIAN_POINT ( 'NONE',  ( -5.207740401424942434, 6.208690235484773723, 1.082531754730549078 ) ) ;
#165576=CARTESIAN_POINT ( 'NONE',  ( -4.411198876399886615, 6.239761003923544713, -1.599625672291271394 ) ) ;
#165586=CARTESIAN_POINT ( 'NONE',  ( -1.843739406749240750, 8.920000000000001705, -0.7749999999999996891 ) ) ;
#165587=CARTESIAN_POINT ( 'NONE',  ( 7.013428937081408243, 5.939655416065873439, -2.436399677959149024 ) ) ;
#165588=CARTESIAN_POINT ( 'NONE',  ( -4.584908210271880336, 8.498668195373706880, -0.01721603403951645073 ) ) ;
#165607=CARTESIAN_POINT ( 'NONE',  ( 6.723917837734620484, 6.809268663637336516, 0.000000000000000000 ) ) ;
#165632=CARTESIAN_POINT ( 'NONE',  ( 5.505492895601038938, 8.580769590579979678, -1.199719254218452047 ) ) ;
#165633=CARTESIAN_POINT ( 'NONE',  ( 4.050854035433010480, 7.948023151305657841, 0.000000000000000000 ) ) ;
#165635=CARTESIAN_POINT ( 'NONE',  ( 5.825163275726873202, 6.825053905550038991, 1.199719254218452047 ) ) ;
#165647=CARTESIAN_POINT ( 'NONE',  ( 5.631620320865258655, 7.357208097040313532, -1.234165276361798735 ) ) ;
#165648=CARTESIAN_POINT ( 'NONE',  ( -5.926322542504877333, 7.047036066744706950, -1.082531754730549967 ) ) ;
#165649=CARTESIAN_POINT ( 'NONE',  ( 4.800995793014950941, 5.734154859006458160, -1.082531754730548412 ) ) ;
#165674=CARTESIAN_POINT ( 'NONE',  ( 5.716698046817569434, 6.698511138489155137, -1.199719254218452047 ) ) ;
#165676=CARTESIAN_POINT ( 'NONE',  ( 4.573896719763862251, 6.429575154514868274, -1.599625672291273171 ) ) ;
#165692=DIRECTION ( 'NONE',  ( 0.000000000000000000, 0.000000000000000000, -1.000000000000000000 ) ) ;
#165705=CARTESIAN_POINT ( 'NONE',  ( 6.017840079619279692, 8.114175741012878973, -1.599625672291281386 ) ) ;
#165709=CARTESIAN_POINT ( 'NONE',  ( -5.911423380092099222, 7.159701334921778404, 1.127351979631958434 ) ) ;
#165710=CARTESIAN_POINT ( 'NONE',  ( 6.607619761813720238, 8.802252036906432764, 1.599625672291268286 ) ) ;
#165745=CARTESIAN_POINT ( 'NONE',  ( -5.582925393777276035, 9.735439736040634173, 0.7998128361456291469 ) ) ;
#165747=CARTESIAN_POINT ( 'NONE',  ( 7.201315867513990554, 8.430565262634994284, -1.199719254218452047 ) ) ;
#165751=CARTESIAN_POINT ( 'NONE',  ( -3.634994582239682526, 6.294558541704648569, 1.082531754730549967 ) ) ;
#165761=CARTESIAN_POINT ( 'NONE',  ( -6.529347706211431124, 6.814240946220119000, -0.5220719126654594922 ) ) ;
#165771=CARTESIAN_POINT ( 'NONE',  ( 6.343235766347262938, 8.493804042195527870, -1.599625672291281386 ) ) ;
#165780=CARTESIAN_POINT ( 'NONE',  ( 5.885648082108188461, 8.920320958217979879, 1.082531754730549967 ) ) ;
#165784=ORIENTED_EDGE ( 'NONE', *, *, #100023, .F. ) ;
#165793=CARTESIAN_POINT ( 'NONE',  ( -3.960390268967665328, 6.674186842887300131, 1.082531754730549967 ) ) ;
#165795=CARTESIAN_POINT ( 'NONE',  ( 4.850785098639300408, 8.881276058379668825, -0.7998128361456481317 ) ) ;
#165798=CARTESIAN_POINT ( 'NONE',  ( -5.772739544368596043, 9.956889578397179363, -0.7998128361456362523 ) ) ;
#165799=CARTESIAN_POINT ( 'NONE',  ( -3.006876207180748217, 6.730049018344652190, -0.7998128361456481317 ) ) ;
#165814=CARTESIAN_POINT ( 'NONE',  ( 0.000000000000000000, 8.999999999999998224, 0.000000000000000000 ) ) ;
#165825=EDGE_LOOP ( 'NONE', ( #152915, #213645, #88764, #105170 ) ) ;
#165842=CARTESIAN_POINT ( 'NONE',  ( 4.634908411025333130, 6.500755460986618495, 1.599625672291268286 ) ) ;
#165848=CARTESIAN_POINT ( 'NONE',  ( -4.773879485343255347, 8.583626809626847987, 0.000000000000000000 ) ) ;
#165855=CARTESIAN_POINT ( 'NONE',  ( -6.129167961829681488, 9.308390501180058507, -1.199719254218452047 ) ) ;
#165863=CARTESIAN_POINT ( 'NONE',  ( -7.130662446144611977, 7.283804040115648526, 0.000000000000000000 ) ) ;
#165866=CARTESIAN_POINT ( 'NONE',  ( 4.623177087595867540, 8.455029494522658950, -0.3425024339245314464 ) ) ;
#165871=CARTESIAN_POINT ( 'NONE',  ( 8.005163354226054295, 8.304055099544019214, 0.000000000000000000 ) ) ;
#165878=CARTESIAN_POINT ( 'NONE',  ( -5.492988512192097161, 6.437516681426083132, 1.199719254218452935 ) ) ;
#165883=CARTESIAN_POINT ( 'NONE',  ( -6.261886844665283114, 8.398896966899865646, 1.599625672291269396 ) ) ;
#165888=CARTESIAN_POINT ( 'NONE',  ( 7.973603738168424826, 8.475161580717541554, 0.000000000000000000 ) ) ;
#165890=CARTESIAN_POINT ( 'NONE',  ( -7.390603132780795725, 8.755363422066633206, -1.082531754730549967 ) ) ;
#165896=CARTESIAN_POINT ( 'NONE',  ( 4.694866332082116678, 8.699370830729650450, 0.7998128361456341429 ) ) ;
#165906=LINE ( 'NONE', #200510, #73856 ) ;
#165910=CARTESIAN_POINT ( 'NONE',  ( 5.796475149741596056, 7.337953333587568849, -1.293683646293428913 ) ) ;
#165924=CARTESIAN_POINT ( 'NONE',  ( -5.492461626867567226, 6.540864998501174199, 1.082531754730549078 ) ) ;
#165925=AXIS2_PLACEMENT_3D ( 'NONE', #101226, #34098, #166234 ) ;
#165937=CARTESIAN_POINT ( 'NONE',  ( -5.432786300537782331, 7.535064667520821047, -1.248352293942560642 ) ) ;
#165955=CARTESIAN_POINT ( 'NONE',  ( -5.438755897737433287, 6.374245297895642537, -1.199719254218453823 ) ) ;
#165968=CARTESIAN_POINT ( 'NONE',  ( 7.178115983792402233, 7.339166500704784823, 0.7998128361456281477 ) ) ;
#165971=CARTESIAN_POINT ( 'NONE',  ( 7.499068361690118145, 7.921536974826172361, -0.7216878364870317197 ) ) ;
#165986=CARTESIAN_POINT ( 'NONE',  ( -5.041653019435350380, 6.975290837464928728, -1.599625672291271394 ) ) ;
#165988=CARTESIAN_POINT ( 'NONE',  ( 5.903649544107831382, 5.852288987739402870, -0.7998128361456481317 ) ) ;
#165997=CARTESIAN_POINT ( 'NONE',  ( -2.830620210203090181, 6.524417021870718258, 0.000000000000000000 ) ) ;
#165998=CARTESIAN_POINT ( 'NONE',  ( 7.180978637093494044, 8.406838493811077839, -1.199719254218452047 ) ) ;
#166006=CARTESIAN_POINT ( 'NONE',  ( 3.542423274920540432, 7.354853930707762721, -1.734723475976807094E-15 ) ) ;
#166012=CARTESIAN_POINT ( 'NONE',  ( -6.365373075063135211, 6.924066019909299818, 0.8511317711424144505 ) ) ;
#166021=CIRCLE ( 'NONE', #214360, 0.07999999999999983513 ) ;
#166022=CARTESIAN_POINT ( 'NONE',  ( -3.594320120954326292, 6.247105003538398371, 1.082531754730549967 ) ) ;
#166032=FACE_OUTER_BOUND ( 'NONE', #75710, .T. ) ;
#166035=CARTESIAN_POINT ( 'NONE',  ( -4.492294583947431086, 8.028511867738693297, 2.499999999999999556 ) ) ;
#166053=CARTESIAN_POINT ( 'NONE',  ( 4.037295881819344956, 7.932205305423044805, -0.7998128361456361413 ) ) ;
#166072=CARTESIAN_POINT ( 'NONE',  ( 0.2923161531638042709, 3.292654673391459674, 2.051239600996176637 ) ) ;
#166073=CARTESIAN_POINT ( 'NONE',  ( 4.878955176071345434, 6.785476686873604280, -1.599625672291269396 ) ) ;
#166074=CARTESIAN_POINT ( 'NONE',  ( -4.095971805104331231, 5.871996087412059140, 1.443375672974065660 ) ) ;
#166098=CARTESIAN_POINT ( 'NONE',  ( -6.577640801285370209, 7.702944352034914566, -1.199719254218452047 ) ) ;
#166101=CARTESIAN_POINT ( 'NONE',  ( 6.278834536460164983, 9.379038488295265097, -1.082531754730548412 ) ) ;
#166109=CARTESIAN_POINT ( 'NONE',  ( -6.102578539482539810, 6.292298848917299736, 0.000000000000000000 ) ) ;
#166114=CARTESIAN_POINT ( 'NONE',  ( -6.749980374757255319, 8.968339418673846097, 1.599625672291269396 ) ) ;
#166121=FACE_OUTER_BOUND ( 'NONE', #97676, .T. ) ;
#166125=CARTESIAN_POINT ( 'NONE',  ( -5.152980901645737077, 8.169505597632108262, -1.199719254218453823 ) ) ;
#166128=CARTESIAN_POINT ( 'NONE',  ( -6.373741612200205076, 8.529394195690610303, 1.443375672974064550 ) ) ;
#166130=CARTESIAN_POINT ( 'NONE',  ( 8.025500584646550806, 8.327781868367935658, 0.000000000000000000 ) ) ;
#166131=CARTESIAN_POINT ( 'NONE',  ( -3.757017964318317471, 6.436919154129725484, 1.082531754730549967 ) ) ;
#166145=CARTESIAN_POINT ( 'NONE',  ( -0.4135631787092041711, 3.000773892238208784, 2.020199156340489743 ) ) ;
#166150=CARTESIAN_POINT ( 'NONE',  ( 6.505076094845553492, 6.832456077006010098, -0.5564590407885674495 ) ) ;
#166153=CARTESIAN_POINT ( 'NONE',  ( 6.142902043169038429, 7.013529245237516641, 0.9864344219776898237 ) ) ;
#166156=CARTESIAN_POINT ( 'NONE',  ( -3.707465945607718805, 7.355851012256872323, 0.5743249234583160945 ) ) ;
#166170=CARTESIAN_POINT ( 'NONE',  ( 5.788239156490550208, 7.236076679697275083, -1.185412701995581797 ) ) ;
#166184=CARTESIAN_POINT ( 'NONE',  ( 8.011942431032855083, 8.311964022485323511, 0.7998128361456291469 ) ) ;
#166187=CARTESIAN_POINT ( 'NONE',  ( -7.130662446144611977, 7.283804040115648526, 0.000000000000000000 ) ) ;
#166200=CARTESIAN_POINT ( 'NONE',  ( 5.585032934186686226, 5.480569609498057382, 0.000000000000000000 ) ) ;
#166202=CARTESIAN_POINT ( 'NONE',  ( 5.671053392266061977, 9.838255734277600695, 0.7998128361456331437 ) ) ;
#166207=DIRECTION ( 'NONE',  ( 0.000000000000000000, 0.000000000000000000, 1.000000000000000000 ) ) ;
#166209=CARTESIAN_POINT ( 'NONE',  ( -6.468648687051513413, 7.679749902049126220, 1.082531754730549078 ) ) ;
#166215=CARTESIAN_POINT ( 'NONE',  ( 5.826972158823246595, 10.02016096192762085, -0.7998128361456481317 ) ) ;
#166230=CARTESIAN_POINT ( 'NONE',  ( -6.183927461608886844, 7.347575139032721303, 1.082531754730548412 ) ) ;
#166232=CARTESIAN_POINT ( 'NONE',  ( 4.421367491832258523, 8.172362817197399210, 0.7216878364870257245 ) ) ;
#166234=DIRECTION ( 'NONE',  ( 2.168404344971003188E-14, 0.000000000000000000, -1.000000000000000000 ) ) ;
#166242=CARTESIAN_POINT ( 'NONE',  ( -3.311934663488232733, 7.085950550703385531, -0.7998128361456481317 ) ) ;
#166243=CARTESIAN_POINT ( 'NONE',  ( -5.153507786970262572, 9.026526494858359229, -0.7216878364870338292 ) ) ;
#166244=CARTESIAN_POINT ( 'NONE',  ( 7.862802741282558294, 8.137967717776607657, 0.000000000000000000 ) ) ;
#166247=CARTESIAN_POINT ( 'NONE',  ( 4.950135482320912494, 6.868520377498098739, -1.443375672974068769 ) ) ;
#166252=CARTESIAN_POINT ( 'NONE',  ( -5.658207315435856088, 5.763393968100056775, -0.1070472433331712409 ) ) ;
#166262=CARTESIAN_POINT ( 'NONE',  ( -3.719872605471121751, 6.605953636083950364, 2.420000000000000373 ) ) ;
#166263=CARTESIAN_POINT ( 'NONE',  ( 4.909461021924256485, 4.900328411765999981, 0.7216878364870338292 ) ) ;
#166266=CARTESIAN_POINT ( 'NONE',  ( -3.955946960137363799, 7.837298230127379917, 0.7998128361456352531 ) ) ;
#166280=CARTESIAN_POINT ( 'NONE',  ( 3.390420931869152721, 6.113185632892752075, -1.199719254218452047 ) ) ;
#166301=ADVANCED_FACE ( 'NONE', ( #9595 ), #138870, .T. ) ;
#166318=CARTESIAN_POINT ( 'NONE',  ( 4.909461021924231616, 8.741805268971372556, 0.7216878364870317197 ) ) ;
#166323=CARTESIAN_POINT ( 'NONE',  ( 4.516274566683592617, 8.283087737857252719, -0.7216878364870357165 ) ) ;
#166336=CARTESIAN_POINT ( 'NONE',  ( -6.583366107887490770, 9.838288338247510367, 1.199719254218452935 ) ) ;
#166338=CARTESIAN_POINT ( 'NONE',  ( -6.064239847062411926, 10.29697326487330500, 0.000000000000000000 ) ) ;
#166341=CARTESIAN_POINT ( 'NONE',  ( 4.666094584615946061, 4.902326079784082857, -0.7990728202500730903 ) ) ;
#166347=CARTESIAN_POINT ( 'NONE',  ( 5.691390622686558487, 9.861982503101517139, 0.7998128361456341429 ) ) ;
#166354=CARTESIAN_POINT ( 'NONE',  ( -5.725286006720766707, 9.901527117808042178, 0.7998128361456291469 ) ) ;
#166360=CARTESIAN_POINT ( 'NONE',  ( -4.651856103264620401, 8.441266197201775512, 0.000000000000000000 ) ) ;
#166363=CARTESIAN_POINT ( 'NONE',  ( -6.099189001301292379, 8.209082816308541197, 1.599625672291263179 ) ) ;
#166374=AXIS2_PLACEMENT_3D ( 'NONE', #201884, #71892, #105513 ) ;
#166383=CARTESIAN_POINT ( 'NONE',  ( -4.394251184604987870, 5.259619482528146150, 1.082531754730549078 ) ) ;
#166385=CARTESIAN_POINT ( 'NONE',  ( -2.997761361953021009, 6.511488999004883205, -0.7216878364870458196 ) ) ;
#166386=FACE_OUTER_BOUND ( 'NONE', #153767, .T. ) ;
#166387=CARTESIAN_POINT ( 'NONE',  ( -3.467853430045390706, 7.267855778353407459, 0.7998128361456352531 ) ) ;
#166388=CARTESIAN_POINT ( 'NONE',  ( -5.956828388357799042, 8.042995434541133193, 1.599625672291263179 ) ) ;
#166418=AXIS2_PLACEMENT_3D ( 'NONE', #108335, #6472, #25934 ) ;
#166442=EDGE_LOOP ( 'NONE', ( #36905, #114274, #147507 ) ) ;
#166445=CARTESIAN_POINT ( 'NONE',  ( 4.115782150200256950, 6.959440387612411349, 1.199719254218452047 ) ) ;
#166448=( BOUNDED_SURFACE ( )  B_SPLINE_SURFACE ( 1, 2, ( 
 ( #187603, #135677, #34946, #167109, #202770, #68504, #171359, #21875, #20819, #3497, #22953, #89067, #18696, #186539, #136743, #84778, #134632, #155125, #6707, #118413, #154056, #101018, #200636, #56556, #39230, #122716, #4558, #38168, #104241, #2427, #150865, #121634, #184398, #52284, #69567, #70632, #36018, #204902, #170287, #169227, #120561, #86915, #152983, #54420, #85847, #105322, #201702, #53345, #87982, #102097, #168167, #37087, #5623, #19765, #72784, #137816, #151924, #203835, #119479, #185467, #103166, #55481, #138884, #209173, #44586, #73866, #208115, #192930, #110699, #139961, #190797, #189737, #172442, #156199, #106419, #42457, #7775, #25101, #205984, #158330, #176699, #59744, #28312, #144252, #142102, #12054, #93342, #207051, #126972, #58683, #94408, #27234, #160447, #125903, #173528, #75997, #191861, #124830, #43522, #74934, #24029, #57620, #174593, #109645, #40312, #78122, #108565, #77051, #91203, #26167, #90132, #8855, #60811, #123777, #92285, #210245, #188678, #41389, #107500, #159378, #9923, #175648, #10977, #143181, #157264, #61881, #141044, #178848, #114952, #177774, #82381, #47793, #213432, #194001, #146359, #32575, #116018, #40, #31525, #112832, #180952, #30459, #211314, #161531, #64013, #128046, #79194, #13116, #132246, #145309, #17363, #16296, #182004, #96544, #130161, #212372, #163658, #164708, #81327, #129107, #45650, #62939, #111767, #195081, #14165, #162591, #80260, #196153, #29389, #46719, #113907, #1113, #179902, #97599, #147406, #15240, #65055, #66104, #33635, #95483, #131211, #197199, #48838, #98651, #148472, #198254, #49894, #99708, #165780, #83447, #149527, #151671, #5364, #67174, #135420, #3242, #68244, #150607, #153794, #105063, #19505, #184140, #119217, #87721, #21613, #167907, #187348, #69308, #2167, #170027, #154864, #200382, #71446, #35764, #201441, #121373, #137558, #171101, #202510, #38977, #133309, #54160, #101839, #186272, #53082, #199314, #22692, #34695, #70373, #50960, #134378, #120299, #203576, #185200, #86652, #36825, #102906, #88805, #100764, #37908, #166846 ),
 ( #117084, #183083, #103984, #18442, #55227, #84519, #52030, #118156, #85581, #168965, #20569, #152720, #4302, #136488, #10722, #76791, #106159, #8594, #7517, #204643, #188413, #138620, #74676, #40050, #57359, #172185, #190540, #142913, #25907, #208913, #176444, #174331, #44320, #125640, #24843, #159121, #90942, #60547, #59483, #126705, #92017, #205724, #108311, #158075, #157008, #9663, #107241, #56294, #23775, #206794, #75739, #72524, #192666, #140779, #109381, #123522, #58426, #122454, #41129, #26974, #89880, #124579, #28056, #6446, #189486, #43263, #110442, #42196, #173262, #155932, #94149, #73599, #139701, #141852, #207857, #191601, #175388, #93079, #77863, #113640, #193743, #82122, #147154, #146098, #128830, #148215, #214217, #143986, #97339, #47527, #209977, #45389, #65846, #131995, #29123, #64808, #11789, #111505, #181746, #98388, #33376, #129905, #163397, #14971, #127788, #61618, #32320, #95210, #177511, #194812, #195889, #161259, #115755, #81068, #79994, #31265, #212109, #63746, #179645, #211045, #16039, #46448, #112569, #213179, #12846, #78920, #145042, #62671, #178580, #30188, #96278, #162328, #13912, #130955, #196945, #48585, #160188, #114701, #180695, #164452, #198004, #49630, #186016, #87478, #165514, #135176, #168715, #17106, #167651, #4052, #20319, #103730, #52830, #187091, #19252, #85332, #183894, #37652, #99457, #151415, #35506, #100514, #182825, #169781, #137307, #51784, #1920, #2989, #120042, #53907, #200131, #5113, #101583, #34441, #202256, #83184, #18178, #21370, #67979, #69056, #153544, #71190, #203324, #86405, #54975, #149267, #152472, #134122, #70122, #201191, #846, #121127, #66911, #102658, #133051, #166589, #136233, #199053, #118967, #184945, #36572, #50699, #116823, #84265, #150350, #117901, #158875, #58172, #6192, #155678, #154613, #122198, #157823, #8345, #74430, #206542, #124330, #72261, #208666, #59227, #89626, #25657, #88552, #207608, #173006, #190290, #104806, #57106, #9419, #26729, #125385, #156756, #23520, #91767, #7260, #188160, #138369, #189237, #38725, #204386, #56042 ) ),
 .UNSPECIFIED., .F., .F., .T. ) 
 B_SPLINE_SURFACE_WITH_KNOTS ( ( 2, 2 ),
 ( 3, 2, 2, 2, 2, 2, 2, 2, 2, 2, 2, 2, 2, 2, 2, 2, 2, 2, 2, 2, 2, 2, 2, 2, 2, 2, 2, 2, 2, 2, 2, 2, 2, 2, 2, 2, 2, 2, 2, 2, 2, 2, 2, 2, 2, 2, 2, 2, 2, 2, 2, 2, 2, 2, 2, 2, 2, 2, 2, 2, 2, 2, 2, 2, 2, 2, 2, 2, 2, 2, 2, 2, 2, 2, 2, 2, 2, 2, 2, 2, 2, 2, 2, 2, 2, 2, 2, 2, 2, 2, 2, 2, 2, 2, 2, 2, 2, 2, 2, 2, 2, 2, 2, 2, 2, 2, 2, 2, 2, 2, 2, 2, 2, 2, 2, 2, 2, 2, 2, 2, 3 ),
 ( 0.000000000000000000, 1.000000000000000000 ),
 ( 0.000000000000000000, 0.008333333333333333218, 0.01666666666666666644, 0.02500000000000000139, 0.03333333333333333287, 0.04166666666666666435, 0.05000000000000000278, 0.05833333333333333426, 0.06666666666666666574, 0.07499999999999999722, 0.08333333333333332871, 0.09166666666666666019, 0.1000000000000000056, 0.1083333333333333370, 0.1166666666666666685, 0.1250000000000000000, 0.1333333333333333315, 0.1416666666666666630, 0.1499999999999999944, 0.1583333333333333259, 0.1666666666666666574, 0.1749999999999999889, 0.1833333333333333204, 0.1916666666666666796, 0.2000000000000000111, 0.2083333333333333426, 0.2166666666666666741, 0.2250000000000000056, 0.2333333333333333370, 0.2416666666666666685, 0.2500000000000000000, 0.2583333333333333592, 0.2666666666666666630, 0.2750000000000000222, 0.2833333333333333259, 0.2916666666666666852, 0.2999999999999999889, 0.3083333333333333481, 0.3166666666666666519, 0.3250000000000000111, 0.3333333333333333148, 0.3416666666666666741, 0.3499999999999999778, 0.3583333333333333370, 0.3666666666666666408, 0.3750000000000000000, 0.3833333333333333592, 0.3916666666666666630, 0.4000000000000000222, 0.4083333333333333259, 0.4166666666666666852, 0.4249999999999999889, 0.4333333333333333481, 0.4416666666666666519, 0.4500000000000000111, 0.4583333333333333148, 0.4666666666666666741, 0.4749999999999999778, 0.4833333333333333370, 0.4916666666666666408, 0.5000000000000000000, 0.5083333333333333037, 0.5166666666666667185, 0.5250000000000000222, 0.5333333333333333259, 0.5416666666666666297, 0.5500000000000000444, 0.5583333333333333481, 0.5666666666666666519, 0.5749999999999999556, 0.5833333333333333703, 0.5916666666666666741, 0.5999999999999999778, 0.6083333333333332815, 0.6166666666666666963, 0.6250000000000000000, 0.6333333333333333037, 0.6416666666666667185, 0.6500000000000000222, 0.6583333333333333259, 0.6666666666666666297, 0.6750000000000000444, 0.6833333333333333481, 0.6916666666666666519, 0.6999999999999999556, 0.7083333333333333703, 0.7166666666666666741, 0.7249999999999999778, 0.7333333333333332815, 0.7416666666666666963, 0.7500000000000000000, 0.7583333333333333037, 0.7666666666666667185, 0.7750000000000000222, 0.7833333333333333259, 0.7916666666666666297, 0.8000000000000000444, 0.8083333333333333481, 0.8166666666666666519, 0.8249999999999999556, 0.8333333333333333703, 0.8416666666666666741, 0.8499999999999999778, 0.8583333333333332815, 0.8666666666666666963, 0.8750000000000000000, 0.8833333333333333037, 0.8916666666666667185, 0.9000000000000000222, 0.9083333333333333259, 0.9166666666666666297, 0.9250000000000000444, 0.9333333333333333481, 0.9416666666666666519, 0.9499999999999999556, 0.9583333333333333703, 0.9666666666666666741, 0.9749999999999999778, 0.9833333333333332815, 0.9916666666666666963, 1.000000000000000000 ),
 .UNSPECIFIED. ) 
 GEOMETRIC_REPRESENTATION_ITEM ( )  RATIONAL_B_SPLINE_SURFACE ( (
 ( 1.000000000000000000, 0.8660254037844387076, 1.000000000000000000, 0.8660254037844387076, 1.000000000000000000, 0.8660254037844387076, 1.000000000000000000, 0.8660254037844387076, 1.000000000000000000, 0.8660254037844387076, 1.000000000000000000, 0.8660254037844387076, 1.000000000000000000, 0.8660254037844387076, 1.000000000000000000, 0.8660254037844387076, 1.000000000000000000, 0.8660254037844387076, 1.000000000000000000, 0.8660254037844387076, 1.000000000000000000, 0.8660254037844387076, 1.000000000000000000, 0.8660254037844387076, 1.000000000000000000, 0.8660254037844387076, 1.000000000000000000, 0.8660254037844387076, 1.000000000000000000, 0.8660254037844387076, 1.000000000000000000, 0.8660254037844387076, 1.000000000000000000, 0.8660254037844387076, 1.000000000000000000, 0.8660254037844387076, 1.000000000000000000, 0.8660254037844387076, 1.000000000000000000, 0.8660254037844387076, 1.000000000000000000, 0.8660254037844387076, 1.000000000000000000, 0.8660254037844387076, 1.000000000000000000, 0.8660254037844387076, 1.000000000000000000, 0.8660254037844387076, 1.000000000000000000, 0.8660254037844387076, 1.000000000000000000, 0.8660254037844387076, 1.000000000000000000, 0.8660254037844387076, 1.000000000000000000, 0.8660254037844387076, 1.000000000000000000, 0.8660254037844387076, 1.000000000000000000, 0.8660254037844387076, 1.000000000000000000, 0.8660254037844387076, 1.000000000000000000, 0.8660254037844387076, 1.000000000000000000, 0.8660254037844387076, 1.000000000000000000, 0.8660254037844387076, 1.000000000000000000, 0.8660254037844387076, 1.000000000000000000, 0.8660254037844387076, 1.000000000000000000, 0.8660254037844387076, 1.000000000000000000, 0.8660254037844387076, 1.000000000000000000, 0.8660254037844387076, 1.000000000000000000, 0.8660254037844387076, 1.000000000000000000, 0.8660254037844387076, 1.000000000000000000, 0.8660254037844387076, 1.000000000000000000, 0.8660254037844387076, 1.000000000000000000, 0.8660254037844387076, 1.000000000000000000, 0.8660254037844387076, 1.000000000000000000, 0.8660254037844387076, 1.000000000000000000, 0.8660254037844387076, 1.000000000000000000, 0.8660254037844387076, 1.000000000000000000, 0.8660254037844387076, 1.000000000000000000, 0.8660254037844387076, 1.000000000000000000, 0.8660254037844387076, 1.000000000000000000, 0.8660254037844387076, 1.000000000000000000, 0.8660254037844387076, 1.000000000000000000, 0.8660254037844387076, 1.000000000000000000, 0.8660254037844387076, 1.000000000000000000, 0.8660254037844387076, 1.000000000000000000, 0.8660254037844387076, 1.000000000000000000, 0.8660254037844387076, 1.000000000000000000, 0.8660254037844387076, 1.000000000000000000, 0.8660254037844387076, 1.000000000000000000, 0.8660254037844387076, 1.000000000000000000, 0.8660254037844387076, 1.000000000000000000, 0.8660254037844387076, 1.000000000000000000, 0.8660254037844387076, 1.000000000000000000, 0.8660254037844387076, 1.000000000000000000, 0.8660254037844387076, 1.000000000000000000, 0.8660254037844387076, 1.000000000000000000, 0.8660254037844387076, 1.000000000000000000, 0.8660254037844387076, 1.000000000000000000, 0.8660254037844387076, 1.000000000000000000, 0.8660254037844387076, 1.000000000000000000, 0.8660254037844387076, 1.000000000000000000, 0.8660254037844387076, 1.000000000000000000, 0.8660254037844387076, 1.000000000000000000, 0.8660254037844387076, 1.000000000000000000, 0.8660254037844387076, 1.000000000000000000, 0.8660254037844387076, 1.000000000000000000, 0.8660254037844387076, 1.000000000000000000, 0.8660254037844387076, 1.000000000000000000, 0.8660254037844387076, 1.000000000000000000, 0.8660254037844387076, 1.000000000000000000, 0.8660254037844387076, 1.000000000000000000, 0.8660254037844387076, 1.000000000000000000, 0.8660254037844387076, 1.000000000000000000, 0.8660254037844387076, 1.000000000000000000, 0.8660254037844387076, 1.000000000000000000, 0.8660254037844387076, 1.000000000000000000, 0.8660254037844387076, 1.000000000000000000, 0.8660254037844387076, 1.000000000000000000, 0.8660254037844387076, 1.000000000000000000, 0.8660254037844387076, 1.000000000000000000, 0.8660254037844387076, 1.000000000000000000, 0.8660254037844387076, 1.000000000000000000, 0.8660254037844387076, 1.000000000000000000, 0.8660254037844387076, 1.000000000000000000, 0.8660254037844387076, 1.000000000000000000, 0.8660254037844387076, 1.000000000000000000, 0.8660254037844387076, 1.000000000000000000, 0.8660254037844387076, 1.000000000000000000, 0.8660254037844387076, 1.000000000000000000, 0.8660254037844387076, 1.000000000000000000, 0.8660254037844387076, 1.000000000000000000, 0.8660254037844387076, 1.000000000000000000, 0.8660254037844387076, 1.000000000000000000, 0.8660254037844387076, 1.000000000000000000, 0.8660254037844387076, 1.000000000000000000, 0.8660254037844387076, 1.000000000000000000, 0.8660254037844387076, 1.000000000000000000, 0.8660254037844387076, 1.000000000000000000, 0.8660254037844387076, 1.000000000000000000, 0.8660254037844387076, 1.000000000000000000, 0.8660254037844387076, 1.000000000000000000, 0.8660254037844387076, 1.000000000000000000, 0.8660254037844387076, 1.000000000000000000, 0.8660254037844387076, 1.000000000000000000, 0.8660254037844387076, 1.000000000000000000, 0.8660254037844387076, 1.000000000000000000, 0.8660254037844387076, 1.000000000000000000, 0.8660254037844387076, 1.000000000000000000, 0.8660254037844387076, 1.000000000000000000),
 ( 1.000000000000000000, 0.8660254037844387076, 1.000000000000000000, 0.8660254037844387076, 1.000000000000000000, 0.8660254037844387076, 1.000000000000000000, 0.8660254037844387076, 1.000000000000000000, 0.8660254037844387076, 1.000000000000000000, 0.8660254037844387076, 1.000000000000000000, 0.8660254037844387076, 1.000000000000000000, 0.8660254037844387076, 1.000000000000000000, 0.8660254037844387076, 1.000000000000000000, 0.8660254037844387076, 1.000000000000000000, 0.8660254037844387076, 1.000000000000000000, 0.8660254037844387076, 1.000000000000000000, 0.8660254037844387076, 1.000000000000000000, 0.8660254037844387076, 1.000000000000000000, 0.8660254037844387076, 1.000000000000000000, 0.8660254037844387076, 1.000000000000000000, 0.8660254037844387076, 1.000000000000000000, 0.8660254037844387076, 1.000000000000000000, 0.8660254037844387076, 1.000000000000000000, 0.8660254037844387076, 1.000000000000000000, 0.8660254037844387076, 1.000000000000000000, 0.8660254037844387076, 1.000000000000000000, 0.8660254037844387076, 1.000000000000000000, 0.8660254037844387076, 1.000000000000000000, 0.8660254037844387076, 1.000000000000000000, 0.8660254037844387076, 1.000000000000000000, 0.8660254037844387076, 1.000000000000000000, 0.8660254037844387076, 1.000000000000000000, 0.8660254037844387076, 1.000000000000000000, 0.8660254037844387076, 1.000000000000000000, 0.8660254037844387076, 1.000000000000000000, 0.8660254037844387076, 1.000000000000000000, 0.8660254037844387076, 1.000000000000000000, 0.8660254037844387076, 1.000000000000000000, 0.8660254037844387076, 1.000000000000000000, 0.8660254037844387076, 1.000000000000000000, 0.8660254037844387076, 1.000000000000000000, 0.8660254037844387076, 1.000000000000000000, 0.8660254037844387076, 1.000000000000000000, 0.8660254037844387076, 1.000000000000000000, 0.8660254037844387076, 1.000000000000000000, 0.8660254037844387076, 1.000000000000000000, 0.8660254037844387076, 1.000000000000000000, 0.8660254037844387076, 1.000000000000000000, 0.8660254037844387076, 1.000000000000000000, 0.8660254037844387076, 1.000000000000000000, 0.8660254037844387076, 1.000000000000000000, 0.8660254037844387076, 1.000000000000000000, 0.8660254037844387076, 1.000000000000000000, 0.8660254037844387076, 1.000000000000000000, 0.8660254037844387076, 1.000000000000000000, 0.8660254037844387076, 1.000000000000000000, 0.8660254037844387076, 1.000000000000000000, 0.8660254037844387076, 1.000000000000000000, 0.8660254037844387076, 1.000000000000000000, 0.8660254037844387076, 1.000000000000000000, 0.8660254037844387076, 1.000000000000000000, 0.8660254037844387076, 1.000000000000000000, 0.8660254037844387076, 1.000000000000000000, 0.8660254037844387076, 1.000000000000000000, 0.8660254037844387076, 1.000000000000000000, 0.8660254037844387076, 1.000000000000000000, 0.8660254037844387076, 1.000000000000000000, 0.8660254037844387076, 1.000000000000000000, 0.8660254037844387076, 1.000000000000000000, 0.8660254037844387076, 1.000000000000000000, 0.8660254037844387076, 1.000000000000000000, 0.8660254037844387076, 1.000000000000000000, 0.8660254037844387076, 1.000000000000000000, 0.8660254037844387076, 1.000000000000000000, 0.8660254037844387076, 1.000000000000000000, 0.8660254037844387076, 1.000000000000000000, 0.8660254037844387076, 1.000000000000000000, 0.8660254037844387076, 1.000000000000000000, 0.8660254037844387076, 1.000000000000000000, 0.8660254037844387076, 1.000000000000000000, 0.8660254037844387076, 1.000000000000000000, 0.8660254037844387076, 1.000000000000000000, 0.8660254037844387076, 1.000000000000000000, 0.8660254037844387076, 1.000000000000000000, 0.8660254037844387076, 1.000000000000000000, 0.8660254037844387076, 1.000000000000000000, 0.8660254037844387076, 1.000000000000000000, 0.8660254037844387076, 1.000000000000000000, 0.8660254037844387076, 1.000000000000000000, 0.8660254037844387076, 1.000000000000000000, 0.8660254037844387076, 1.000000000000000000, 0.8660254037844387076, 1.000000000000000000, 0.8660254037844387076, 1.000000000000000000, 0.8660254037844387076, 1.000000000000000000, 0.8660254037844387076, 1.000000000000000000, 0.8660254037844387076, 1.000000000000000000, 0.8660254037844387076, 1.000000000000000000, 0.8660254037844387076, 1.000000000000000000, 0.8660254037844387076, 1.000000000000000000, 0.8660254037844387076, 1.000000000000000000, 0.8660254037844387076, 1.000000000000000000, 0.8660254037844387076, 1.000000000000000000, 0.8660254037844387076, 1.000000000000000000, 0.8660254037844387076, 1.000000000000000000, 0.8660254037844387076, 1.000000000000000000, 0.8660254037844387076, 1.000000000000000000, 0.8660254037844387076, 1.000000000000000000, 0.8660254037844387076, 1.000000000000000000, 0.8660254037844387076, 1.000000000000000000, 0.8660254037844387076, 1.000000000000000000, 0.8660254037844387076, 1.000000000000000000, 0.8660254037844387076, 1.000000000000000000, 0.8660254037844387076, 1.000000000000000000, 0.8660254037844387076, 1.000000000000000000, 0.8660254037844387076, 1.000000000000000000, 0.8660254037844387076, 1.000000000000000000, 0.8660254037844387076, 1.000000000000000000, 0.8660254037844387076, 1.000000000000000000, 0.8660254037844387076, 1.000000000000000000, 0.8660254037844387076, 1.000000000000000000, 0.8660254037844387076, 1.000000000000000000, 0.8660254037844387076, 1.000000000000000000, 0.8660254037844387076, 1.000000000000000000, 0.8660254037844387076, 1.000000000000000000) ) ) 
 REPRESENTATION_ITEM ( '' )  SURFACE ( )  );
#166461=CARTESIAN_POINT ( 'NONE',  ( 5.885648082108177803, 9.880690172519326353, 0.7216878364870317197 ) ) ;
#166465=CARTESIAN_POINT ( 'NONE',  ( -6.445975688654487001, 6.485002823043819475, -0.7998128361456362523 ) ) ;
#166471=CARTESIAN_POINT ( 'NONE',  ( -7.282137903871469753, 8.628820655005750240, 1.082531754730549078 ) ) ;
#166475=CARTESIAN_POINT ( 'NONE',  ( 5.411112705185558092, 6.445957923205511086, -1.082531754730548412 ) ) ;
#166479=CARTESIAN_POINT ( 'NONE',  ( 4.556949027968946631, 8.330541276023501140, -0.7216878364870357165 ) ) ;
#166483=CARTESIAN_POINT ( 'NONE',  ( -5.123001941117347080, 7.070197912760590064, 1.599625672291263179 ) ) ;
#166494=CARTESIAN_POINT ( 'NONE',  ( 5.727393547130178675, 5.646656991265468939, 0.000000000000000000 ) ) ;
#166495=CARTESIAN_POINT ( 'NONE',  ( 4.441177836928239309, 7.339068688795062911, 1.199719254218452047 ) ) ;
#166521=CARTESIAN_POINT ( 'NONE',  ( 6.912678218121202534, 9.158153569265168770, 1.599625672291268286 ) ) ;
#166528=CARTESIAN_POINT ( 'NONE',  ( 6.866278450678116485, 6.975356045404744521, 0.000000000000000000 ) ) ;
#166536=CARTESIAN_POINT ( 'NONE',  ( 3.580761967785000888, 7.191656372475549119, -0.7216878364870338292 ) ) ;
#166539=CARTESIAN_POINT ( 'NONE',  ( 6.861835142292147083, 7.178098218861903135, 0.7216878364870328300 ) ) ;
#166544=LINE ( 'NONE', #179602, #171609 ) ;
#166552=CARTESIAN_POINT ( 'NONE',  ( 6.053075614097062740, 7.042710966267798689, -1.019147762646470001 ) ) ;
#166553=CARTESIAN_POINT ( 'NONE',  ( -5.641601317062233001, 9.595968946632336127, -0.7216878364870338292 ) ) ;
#166589=CARTESIAN_POINT ( 'NONE',  ( 6.505933609711257226, 8.683618192786854095, -1.599625672291281386 ) ) ;
#166590=CARTESIAN_POINT ( 'NONE',  ( -5.275531169048909952, 7.248148678680751189, -1.443375672974066770 ) ) ;
#166591=CARTESIAN_POINT ( 'NONE',  ( 5.515134625708930649, 9.656350506627580543, 0.000000000000000000 ) ) ;
#166605=CARTESIAN_POINT ( 'NONE',  ( -3.786470039966538970, 7.639575156594750283, 0.000000000000000000 ) ) ;
#166607=CARTESIAN_POINT ( 'NONE',  ( 4.706088717274895750, 6.583799151611112954, 1.443375672974065660 ) ) ;
#166620=CARTESIAN_POINT ( 'NONE',  ( -5.777182853198894463, 9.754147405458438058, 0.7216878364870267237 ) ) ;
#166622=CARTESIAN_POINT ( 'NONE',  ( -5.099275172515603138, 8.002885897026576600, 1.082531754730549967 ) ) ;
#166639=B_SPLINE_CURVE_WITH_KNOTS ( 'NONE', 3,
 ( #49977, #135504, #16385, #36912, #2255, #169052, #185289, #200467, #102995, #118241 ),
 .UNSPECIFIED., .F., .F.,
 ( 4, 3, 3, 4 ),
 ( 4.670885906470136028E-18, 3.125212466446787460E-05, 6.250460353101360055E-05, 0.0001200463674512635038 ),
 .UNSPECIFIED. ) ;
#166648=CARTESIAN_POINT ( 'NONE',  ( -4.625266680917477835, 5.425174544939014964, -1.199719254218453823 ) ) ;
#166649=CARTESIAN_POINT ( 'NONE',  ( -5.605292224350291619, 5.702808290780939871, -0.2219334806705375862 ) ) ;
#166651=CARTESIAN_POINT ( 'NONE',  ( 5.014534001275664288, 7.922250005646839455, -1.103081721458569309 ) ) ;
#166660=CARTESIAN_POINT ( 'NONE',  ( 3.591464764177854541, 3.560402065510233083, -2.500000000000000444 ) ) ;
#166661=CARTESIAN_POINT ( 'NONE',  ( -4.585403371929053229, 8.498043419817562949, 0.04945426522169442396 ) ) ;
#166679=CARTESIAN_POINT ( 'NONE',  ( 6.333594036239346359, 7.418223126147930557, 1.199719254218453823 ) ) ;
#166701=CARTESIAN_POINT ( 'NONE',  ( 6.475954649182838807, 7.584310507915338562, 1.199719254218452047 ) ) ;
#166702=CARTESIAN_POINT ( 'NONE',  ( 5.387385936583818591, 7.378645907471495846, -1.599625672291283607 ) ) ;
#166704=CARTESIAN_POINT ( 'NONE',  ( 6.229045230835819069, 6.231917288922055320, -0.7998128361456481317 ) ) ;
#166718=CARTESIAN_POINT ( 'NONE',  ( 4.754190777897029818, 8.299541367957775861, -0.7767638722561143183 ) ) ;
#166719=CARTESIAN_POINT ( 'NONE',  ( -5.519577934094894722, 7.532869904567736974, 1.443375672974058777 ) ) ;
#166720=CARTESIAN_POINT ( 'NONE',  ( 4.828112100242277549, 6.726159765073026264, -1.443375672974068769 ) ) ;
#166741=CARTESIAN_POINT ( 'NONE',  ( -4.706088717274938382, 6.583799151611112954, 1.443375672974058777 ) ) ;
#166746=CARTESIAN_POINT ( 'NONE',  ( 5.855142236255289845, 7.924361590421551860, -1.599625672291281386 ) ) ;
#166775=CARTESIAN_POINT ( 'NONE',  ( 5.722423353419669567, 8.833855124701747386, 1.199719254218451159 ) ) ;
#166779=CARTESIAN_POINT ( 'NONE',  ( -6.401963353335964335, 6.822014978843597532, 0.5293317295896986518 ) ) ;
#166780=CARTESIAN_POINT ( 'NONE',  ( 6.688968683495743583, 8.897159112202094988, -1.599625672291283607 ) ) ;
#166788=CARTESIAN_POINT ( 'NONE',  ( -1.909527279894951413, 8.998253746724575564, 0.7750000000000013545 ) ) ;
#166789=VECTOR ( 'NONE', #204742, 1000.000000000000000 ) ;
#166813=CARTESIAN_POINT ( 'NONE',  ( -7.618755976236585958, 7.853246491889623648, 0.000000000000000000 ) ) ;
#166815=CARTESIAN_POINT ( 'NONE',  ( 5.691390622686558487, 9.861982503101517139, 0.7998128361456341429 ) ) ;
#166837=CARTESIAN_POINT ( 'NONE',  ( 5.508355548902068577, 9.648441583686274470, 0.7998128361456331437 ) ) ;
#166846=CARTESIAN_POINT ( 'NONE',  ( 8.014278199453778839, 8.522615118883788199, 0.000000000000000000 ) ) ;
#166859=CARTESIAN_POINT ( 'NONE',  ( -6.292392690518214593, 7.474117906093608710, -1.082531754730549967 ) ) ;
#166862=CARTESIAN_POINT ( 'NONE',  ( 6.038177310039780643, 8.137902509836795417, -1.599625672291283607 ) ) ;
#166867=CARTESIAN_POINT ( 'NONE',  ( -3.817502770699643388, 6.611447778194983194, 1.199719254218452935 ) ) ;
#166869=CARTESIAN_POINT ( 'NONE',  ( 3.933798568561588826, 7.324796930770500758, -0.8815854234727003025 ) ) ;
#166910=CARTESIAN_POINT ( 'NONE',  ( 4.177320726786311056, 5.966903162707725805, -1.443375672974068769 ) ) ;
#166915=CARTESIAN_POINT ( 'NONE',  ( 5.228604516725597229, 6.129068686715179126, -1.199719254218450271 ) ) ;
#166917=CARTESIAN_POINT ( 'NONE',  ( 4.858757509019037357, 5.629766575900002401, 2.420000000000000373 ) ) ;
#166918=CARTESIAN_POINT ( 'NONE',  ( -5.906512197408906317, 6.919960980845699439, -1.199719254218453823 ) ) ;
#166922=CARTESIAN_POINT ( 'NONE',  ( -5.844973620822877969, 7.912498205750389424, 1.443375672974058777 ) ) ;
#166928=CARTESIAN_POINT ( 'NONE',  ( -7.045397100956844127, 8.248660034984974132, -1.199719254218452047 ) ) ;
#166935=CARTESIAN_POINT ( 'NONE',  ( 4.773438866691874338, 4.884607349446686619, -0.7620046207243836855 ) ) ;
#166936=FACE_OUTER_BOUND ( 'NONE', #205039, .T. ) ;
#166937=( BOUNDED_SURFACE ( )  B_SPLINE_SURFACE ( 1, 2, ( 
 ( #65019, #144212, #183834, #19191, #151355, #2924, #135114, #12014, #187032, #170791, #168653, #185959, #202192, #22382, #123214, #55981, #136173, #118904, #119982, #70061, #204324, #20257, #87418, #172947, #52768, #40815, #122134, #24526, #74370, #188099, #106923, #39730, #171862, #201130, #184888, #137248, #36512, #154553, #54914, #139378, #121065, #105835, #156695, #38665, #102598, #23456, #86341, #90635, #8285, #53848, #6132, #104744, #169721, #89568, #88492, #152413, #3992, #37591, #103673, #21311, #153484, #155617, #72201, #5055, #7202, #71130, #138309, #73275, #205410, #203268, #57050, #189178, #159881, #207551, #126398, #94904, #10415, #208607, #41890, #141545, #157761, #60239, #111201, #27747, #9361, #206484, #75433, #91712, #110135, #108001, #191293, #160955, #58114, #28819, #176147, #12545, #210755, #93843, #78620, #11486, #77558, #140472, #174028, #76487, #25599, #143681, #209673, #44016, #175084, #144744, #124273, #59171, #61317, #177205, #127477, #190231, #125330, #192358, #193448, #42959, #45092, #109068, #26671, #92775, #158819, #142597, #122854, #205043, #136877, #206121, #54548, #5757, #56687, #105462, #75068, #25239, #171496, #172578, #188815, #40449, #106551, #157401, #186670, #90262, #156330, #88119, #23087, #38297, #7914, #89202, #71836, #155255, #74001, #24159, #140094, #57751, #39365, #8993, #141181, #6837, #72915, #70763, #139020, #170421, #104375, #123911, #189878, #41521, #107633, #202903, #173665, #120695, #137945, #91341, #207190, #119613, #185598, #37229, #103300, #169362, #20947, #87044, #153116, #22009, #4688, #154189, #203967, #55613, #121768, #187737, #130731, #97119, #196724, #115529, #147987, #181524, #165282, #64592, #34208, #100281, #48364, #32092, #96053, #98178, #195667, #211890, #16876, #114477, #82957, #180475, #197771, #166347, #164226, #17938, #213997, #46230, #182585, #144823, #13695, #15814, #81899, #113416, #65617, #131767, #210830, #112347, #116591, #178359, #29967, #47302, #49408, #33152, #62455, #99233, #179423, #149030, #606, #66673, #162106, #31043, #80847 ),
 ( #129683, #145881, #132821, #198825, #50470, #79767, #128618, #63529, #163171, #14756, #146938, #184710, #55797, #150114, #138133, #87233, #121952, #171678, #4873, #204142, #137062, #54731, #84024, #1687, #20078, #133891, #37411, #70952, #119798, #118725, #154373, #39549, #67741, #103487, #170609, #153297, #199897, #22196, #19015, #151180, #187918, #68820, #105650, #134942, #36334, #202007, #2750, #51544, #117668, #168480, #101342, #169548, #85095, #72020, #88309, #3809, #183661, #152237, #200948, #167423, #35265, #52597, #86167, #186856, #102412, #69882, #5950, #135993, #53667, #21129, #203087, #120882, #38487, #104564, #23275, #10244, #206310, #107824, #24342, #40638, #123044, #208434, #156518, #57934, #188995, #27567, #158646, #42784, #111023, #89386, #141370, #106740, #59003, #41714, #108893, #207382, #205227, #8109, #44915, #92603, #174916, #73096, #26496, #209497, #124098, #60068, #109963, #7020, #125159, #155435, #90452, #142425, #75256, #61137, #76320, #74197, #127299, #140291, #191118, #192185, #175973, #91532, #190062, #193269, #173849, #25425, #43849, #157590, #126224, #9185, #93665, #159707, #11306, #77384, #139197, #56868, #114232, #177028, #128370, #30791, #213752, #96870, #178103, #195417, #212704, #64345, #179167, #130491, #162920, #165034, #211636, #29719, #15562, #181277, #13446, #32903, #95801, #45979, #210582, #79523, #194337, #112100, #80592, #358, #161857, #31853, #16627, #145641, #47047, #63272, #28645, #160778, #14500, #129434, #113163, #146688, #115286, #196478, #48120, #12371, #78451, #180230, #82710, #98981, #94732, #163987, #97929, #81649, #147736, #65374, #62213, #131521, #197524, #49168, #148788, #66430, #132573, #198576, #50223, #144569, #85920, #133644, #185534, #37162, #103240, #169300, #51291, #101087, #166101, #20884, #54488, #183413, #186610, #5695, #2499, #71772, #18763, #71521, #57431, #5442, #154937, #206866, #205800, #125712, #74751, #6521, #59553, #88883, #123592, #174405, #25982, #156003, #122529, #191673, #40122, #72598, #92090, #138698, #9736, #7590, #75811 ) ),
 .UNSPECIFIED., .F., .F., .T. ) 
 B_SPLINE_SURFACE_WITH_KNOTS ( ( 2, 2 ),
 ( 3, 2, 2, 2, 2, 2, 2, 2, 2, 2, 2, 2, 2, 2, 2, 2, 2, 2, 2, 2, 2, 2, 2, 2, 2, 2, 2, 2, 2, 2, 2, 2, 2, 2, 2, 2, 2, 2, 2, 2, 2, 2, 2, 2, 2, 2, 2, 2, 2, 2, 2, 2, 2, 2, 2, 2, 2, 2, 2, 2, 2, 2, 2, 2, 2, 2, 2, 2, 2, 2, 2, 2, 2, 2, 2, 2, 2, 2, 2, 2, 2, 2, 2, 2, 2, 2, 2, 2, 2, 2, 2, 2, 2, 2, 2, 2, 2, 2, 2, 2, 2, 2, 2, 2, 2, 2, 2, 2, 2, 2, 2, 2, 2, 2, 2, 2, 2, 2, 2, 2, 3 ),
 ( 0.000000000000000000, 1.000000000000000000 ),
 ( 0.000000000000000000, 0.008333333333333333218, 0.01666666666666666644, 0.02500000000000000139, 0.03333333333333333287, 0.04166666666666666435, 0.05000000000000000278, 0.05833333333333333426, 0.06666666666666666574, 0.07499999999999999722, 0.08333333333333332871, 0.09166666666666666019, 0.1000000000000000056, 0.1083333333333333370, 0.1166666666666666685, 0.1250000000000000000, 0.1333333333333333315, 0.1416666666666666630, 0.1499999999999999944, 0.1583333333333333259, 0.1666666666666666574, 0.1749999999999999889, 0.1833333333333333204, 0.1916666666666666796, 0.2000000000000000111, 0.2083333333333333426, 0.2166666666666666741, 0.2250000000000000056, 0.2333333333333333370, 0.2416666666666666685, 0.2500000000000000000, 0.2583333333333333592, 0.2666666666666666630, 0.2750000000000000222, 0.2833333333333333259, 0.2916666666666666852, 0.2999999999999999889, 0.3083333333333333481, 0.3166666666666666519, 0.3250000000000000111, 0.3333333333333333148, 0.3416666666666666741, 0.3499999999999999778, 0.3583333333333333370, 0.3666666666666666408, 0.3750000000000000000, 0.3833333333333333592, 0.3916666666666666630, 0.4000000000000000222, 0.4083333333333333259, 0.4166666666666666852, 0.4249999999999999889, 0.4333333333333333481, 0.4416666666666666519, 0.4500000000000000111, 0.4583333333333333148, 0.4666666666666666741, 0.4749999999999999778, 0.4833333333333333370, 0.4916666666666666408, 0.5000000000000000000, 0.5083333333333333037, 0.5166666666666667185, 0.5250000000000000222, 0.5333333333333333259, 0.5416666666666666297, 0.5500000000000000444, 0.5583333333333333481, 0.5666666666666666519, 0.5749999999999999556, 0.5833333333333333703, 0.5916666666666666741, 0.5999999999999999778, 0.6083333333333332815, 0.6166666666666666963, 0.6250000000000000000, 0.6333333333333333037, 0.6416666666666667185, 0.6500000000000000222, 0.6583333333333333259, 0.6666666666666666297, 0.6750000000000000444, 0.6833333333333333481, 0.6916666666666666519, 0.6999999999999999556, 0.7083333333333333703, 0.7166666666666666741, 0.7249999999999999778, 0.7333333333333332815, 0.7416666666666666963, 0.7500000000000000000, 0.7583333333333333037, 0.7666666666666667185, 0.7750000000000000222, 0.7833333333333333259, 0.7916666666666666297, 0.8000000000000000444, 0.8083333333333333481, 0.8166666666666666519, 0.8249999999999999556, 0.8333333333333333703, 0.8416666666666666741, 0.8499999999999999778, 0.8583333333333332815, 0.8666666666666666963, 0.8750000000000000000, 0.8833333333333333037, 0.8916666666666667185, 0.9000000000000000222, 0.9083333333333333259, 0.9166666666666666297, 0.9250000000000000444, 0.9333333333333333481, 0.9416666666666666519, 0.9499999999999999556, 0.9583333333333333703, 0.9666666666666666741, 0.9749999999999999778, 0.9833333333333332815, 0.9916666666666666963, 1.000000000000000000 ),
 .UNSPECIFIED. ) 
 GEOMETRIC_REPRESENTATION_ITEM ( )  RATIONAL_B_SPLINE_SURFACE ( (
 ( 1.000000000000000000, 0.8660254037844387076, 1.000000000000000000, 0.8660254037844387076, 1.000000000000000000, 0.8660254037844387076, 1.000000000000000000, 0.8660254037844387076, 1.000000000000000000, 0.8660254037844387076, 1.000000000000000000, 0.8660254037844387076, 1.000000000000000000, 0.8660254037844387076, 1.000000000000000000, 0.8660254037844387076, 1.000000000000000000, 0.8660254037844387076, 1.000000000000000000, 0.8660254037844387076, 1.000000000000000000, 0.8660254037844387076, 1.000000000000000000, 0.8660254037844387076, 1.000000000000000000, 0.8660254037844387076, 1.000000000000000000, 0.8660254037844387076, 1.000000000000000000, 0.8660254037844387076, 1.000000000000000000, 0.8660254037844387076, 1.000000000000000000, 0.8660254037844387076, 1.000000000000000000, 0.8660254037844387076, 1.000000000000000000, 0.8660254037844387076, 1.000000000000000000, 0.8660254037844387076, 1.000000000000000000, 0.8660254037844387076, 1.000000000000000000, 0.8660254037844387076, 1.000000000000000000, 0.8660254037844387076, 1.000000000000000000, 0.8660254037844387076, 1.000000000000000000, 0.8660254037844387076, 1.000000000000000000, 0.8660254037844387076, 1.000000000000000000, 0.8660254037844387076, 1.000000000000000000, 0.8660254037844387076, 1.000000000000000000, 0.8660254037844387076, 1.000000000000000000, 0.8660254037844387076, 1.000000000000000000, 0.8660254037844387076, 1.000000000000000000, 0.8660254037844387076, 1.000000000000000000, 0.8660254037844387076, 1.000000000000000000, 0.8660254037844387076, 1.000000000000000000, 0.8660254037844387076, 1.000000000000000000, 0.8660254037844387076, 1.000000000000000000, 0.8660254037844387076, 1.000000000000000000, 0.8660254037844387076, 1.000000000000000000, 0.8660254037844387076, 1.000000000000000000, 0.8660254037844387076, 1.000000000000000000, 0.8660254037844387076, 1.000000000000000000, 0.8660254037844387076, 1.000000000000000000, 0.8660254037844387076, 1.000000000000000000, 0.8660254037844387076, 1.000000000000000000, 0.8660254037844387076, 1.000000000000000000, 0.8660254037844387076, 1.000000000000000000, 0.8660254037844387076, 1.000000000000000000, 0.8660254037844387076, 1.000000000000000000, 0.8660254037844387076, 1.000000000000000000, 0.8660254037844387076, 1.000000000000000000, 0.8660254037844387076, 1.000000000000000000, 0.8660254037844387076, 1.000000000000000000, 0.8660254037844387076, 1.000000000000000000, 0.8660254037844387076, 1.000000000000000000, 0.8660254037844387076, 1.000000000000000000, 0.8660254037844387076, 1.000000000000000000, 0.8660254037844387076, 1.000000000000000000, 0.8660254037844387076, 1.000000000000000000, 0.8660254037844387076, 1.000000000000000000, 0.8660254037844387076, 1.000000000000000000, 0.8660254037844387076, 1.000000000000000000, 0.8660254037844387076, 1.000000000000000000, 0.8660254037844387076, 1.000000000000000000, 0.8660254037844387076, 1.000000000000000000, 0.8660254037844387076, 1.000000000000000000, 0.8660254037844387076, 1.000000000000000000, 0.8660254037844387076, 1.000000000000000000, 0.8660254037844387076, 1.000000000000000000, 0.8660254037844387076, 1.000000000000000000, 0.8660254037844387076, 1.000000000000000000, 0.8660254037844387076, 1.000000000000000000, 0.8660254037844387076, 1.000000000000000000, 0.8660254037844387076, 1.000000000000000000, 0.8660254037844387076, 1.000000000000000000, 0.8660254037844387076, 1.000000000000000000, 0.8660254037844387076, 1.000000000000000000, 0.8660254037844387076, 1.000000000000000000, 0.8660254037844387076, 1.000000000000000000, 0.8660254037844387076, 1.000000000000000000, 0.8660254037844387076, 1.000000000000000000, 0.8660254037844387076, 1.000000000000000000, 0.8660254037844387076, 1.000000000000000000, 0.8660254037844387076, 1.000000000000000000, 0.8660254037844387076, 1.000000000000000000, 0.8660254037844387076, 1.000000000000000000, 0.8660254037844387076, 1.000000000000000000, 0.8660254037844387076, 1.000000000000000000, 0.8660254037844387076, 1.000000000000000000, 0.8660254037844387076, 1.000000000000000000, 0.8660254037844387076, 1.000000000000000000, 0.8660254037844387076, 1.000000000000000000, 0.8660254037844387076, 1.000000000000000000, 0.8660254037844387076, 1.000000000000000000, 0.8660254037844387076, 1.000000000000000000, 0.8660254037844387076, 1.000000000000000000, 0.8660254037844387076, 1.000000000000000000, 0.8660254037844387076, 1.000000000000000000, 0.8660254037844387076, 1.000000000000000000, 0.8660254037844387076, 1.000000000000000000, 0.8660254037844387076, 1.000000000000000000, 0.8660254037844387076, 1.000000000000000000, 0.8660254037844387076, 1.000000000000000000, 0.8660254037844387076, 1.000000000000000000, 0.8660254037844387076, 1.000000000000000000, 0.8660254037844387076, 1.000000000000000000, 0.8660254037844387076, 1.000000000000000000, 0.8660254037844387076, 1.000000000000000000, 0.8660254037844387076, 1.000000000000000000, 0.8660254037844387076, 1.000000000000000000, 0.8660254037844387076, 1.000000000000000000, 0.8660254037844387076, 1.000000000000000000, 0.8660254037844387076, 1.000000000000000000, 0.8660254037844387076, 1.000000000000000000, 0.8660254037844387076, 1.000000000000000000, 0.8660254037844387076, 1.000000000000000000, 0.8660254037844387076, 1.000000000000000000, 0.8660254037844387076, 1.000000000000000000, 0.8660254037844387076, 1.000000000000000000, 0.8660254037844387076, 1.000000000000000000, 0.8660254037844387076, 1.000000000000000000),
 ( 1.000000000000000000, 0.8660254037844387076, 1.000000000000000000, 0.8660254037844387076, 1.000000000000000000, 0.8660254037844387076, 1.000000000000000000, 0.8660254037844387076, 1.000000000000000000, 0.8660254037844387076, 1.000000000000000000, 0.8660254037844387076, 1.000000000000000000, 0.8660254037844387076, 1.000000000000000000, 0.8660254037844387076, 1.000000000000000000, 0.8660254037844387076, 1.000000000000000000, 0.8660254037844387076, 1.000000000000000000, 0.8660254037844387076, 1.000000000000000000, 0.8660254037844387076, 1.000000000000000000, 0.8660254037844387076, 1.000000000000000000, 0.8660254037844387076, 1.000000000000000000, 0.8660254037844387076, 1.000000000000000000, 0.8660254037844387076, 1.000000000000000000, 0.8660254037844387076, 1.000000000000000000, 0.8660254037844387076, 1.000000000000000000, 0.8660254037844387076, 1.000000000000000000, 0.8660254037844387076, 1.000000000000000000, 0.8660254037844387076, 1.000000000000000000, 0.8660254037844387076, 1.000000000000000000, 0.8660254037844387076, 1.000000000000000000, 0.8660254037844387076, 1.000000000000000000, 0.8660254037844387076, 1.000000000000000000, 0.8660254037844387076, 1.000000000000000000, 0.8660254037844387076, 1.000000000000000000, 0.8660254037844387076, 1.000000000000000000, 0.8660254037844387076, 1.000000000000000000, 0.8660254037844387076, 1.000000000000000000, 0.8660254037844387076, 1.000000000000000000, 0.8660254037844387076, 1.000000000000000000, 0.8660254037844387076, 1.000000000000000000, 0.8660254037844387076, 1.000000000000000000, 0.8660254037844387076, 1.000000000000000000, 0.8660254037844387076, 1.000000000000000000, 0.8660254037844387076, 1.000000000000000000, 0.8660254037844387076, 1.000000000000000000, 0.8660254037844387076, 1.000000000000000000, 0.8660254037844387076, 1.000000000000000000, 0.8660254037844387076, 1.000000000000000000, 0.8660254037844387076, 1.000000000000000000, 0.8660254037844387076, 1.000000000000000000, 0.8660254037844387076, 1.000000000000000000, 0.8660254037844387076, 1.000000000000000000, 0.8660254037844387076, 1.000000000000000000, 0.8660254037844387076, 1.000000000000000000, 0.8660254037844387076, 1.000000000000000000, 0.8660254037844387076, 1.000000000000000000, 0.8660254037844387076, 1.000000000000000000, 0.8660254037844387076, 1.000000000000000000, 0.8660254037844387076, 1.000000000000000000, 0.8660254037844387076, 1.000000000000000000, 0.8660254037844387076, 1.000000000000000000, 0.8660254037844387076, 1.000000000000000000, 0.8660254037844387076, 1.000000000000000000, 0.8660254037844387076, 1.000000000000000000, 0.8660254037844387076, 1.000000000000000000, 0.8660254037844387076, 1.000000000000000000, 0.8660254037844387076, 1.000000000000000000, 0.8660254037844387076, 1.000000000000000000, 0.8660254037844387076, 1.000000000000000000, 0.8660254037844387076, 1.000000000000000000, 0.8660254037844387076, 1.000000000000000000, 0.8660254037844387076, 1.000000000000000000, 0.8660254037844387076, 1.000000000000000000, 0.8660254037844387076, 1.000000000000000000, 0.8660254037844387076, 1.000000000000000000, 0.8660254037844387076, 1.000000000000000000, 0.8660254037844387076, 1.000000000000000000, 0.8660254037844387076, 1.000000000000000000, 0.8660254037844387076, 1.000000000000000000, 0.8660254037844387076, 1.000000000000000000, 0.8660254037844387076, 1.000000000000000000, 0.8660254037844387076, 1.000000000000000000, 0.8660254037844387076, 1.000000000000000000, 0.8660254037844387076, 1.000000000000000000, 0.8660254037844387076, 1.000000000000000000, 0.8660254037844387076, 1.000000000000000000, 0.8660254037844387076, 1.000000000000000000, 0.8660254037844387076, 1.000000000000000000, 0.8660254037844387076, 1.000000000000000000, 0.8660254037844387076, 1.000000000000000000, 0.8660254037844387076, 1.000000000000000000, 0.8660254037844387076, 1.000000000000000000, 0.8660254037844387076, 1.000000000000000000, 0.8660254037844387076, 1.000000000000000000, 0.8660254037844387076, 1.000000000000000000, 0.8660254037844387076, 1.000000000000000000, 0.8660254037844387076, 1.000000000000000000, 0.8660254037844387076, 1.000000000000000000, 0.8660254037844387076, 1.000000000000000000, 0.8660254037844387076, 1.000000000000000000, 0.8660254037844387076, 1.000000000000000000, 0.8660254037844387076, 1.000000000000000000, 0.8660254037844387076, 1.000000000000000000, 0.8660254037844387076, 1.000000000000000000, 0.8660254037844387076, 1.000000000000000000, 0.8660254037844387076, 1.000000000000000000, 0.8660254037844387076, 1.000000000000000000, 0.8660254037844387076, 1.000000000000000000, 0.8660254037844387076, 1.000000000000000000, 0.8660254037844387076, 1.000000000000000000, 0.8660254037844387076, 1.000000000000000000, 0.8660254037844387076, 1.000000000000000000, 0.8660254037844387076, 1.000000000000000000, 0.8660254037844387076, 1.000000000000000000, 0.8660254037844387076, 1.000000000000000000, 0.8660254037844387076, 1.000000000000000000, 0.8660254037844387076, 1.000000000000000000, 0.8660254037844387076, 1.000000000000000000, 0.8660254037844387076, 1.000000000000000000, 0.8660254037844387076, 1.000000000000000000, 0.8660254037844387076, 1.000000000000000000, 0.8660254037844387076, 1.000000000000000000, 0.8660254037844387076, 1.000000000000000000, 0.8660254037844387076, 1.000000000000000000, 0.8660254037844387076, 1.000000000000000000, 0.8660254037844387076, 1.000000000000000000, 0.8660254037844387076, 1.000000000000000000) ) ) 
 REPRESENTATION_ITEM ( '' )  SURFACE ( )  );
#166938=CARTESIAN_POINT ( 'NONE',  ( -6.577640801285370209, 7.702944352034914566, -1.199719254218452047 ) ) ;
#166939=CARTESIAN_POINT ( 'NONE',  ( 4.966250736084032447, 8.070317005903060448, 1.090833899539983554 ) ) ;
#166944=CARTESIAN_POINT ( 'NONE',  ( 5.993586425693011144, 9.150212042353954800, -1.199719254218452047 ) ) ;
#166953=CARTESIAN_POINT ( 'NONE',  ( -6.005335696210345020, 5.970922831858983315, 0.7998128361456281477 ) ) ;
#166958=CARTESIAN_POINT ( 'NONE',  ( -6.784929528996132220, 6.880448970109080520, 0.000000000000000000 ) ) ;
#166962=CARTESIAN_POINT ( 'NONE',  ( 7.309254211098760834, 8.660456346770972758, 1.082531754730549967 ) ) ;
#166964=CARTESIAN_POINT ( 'NONE',  ( -5.899206235277530297, 9.896508017883515862, 0.7216878364870267237 ) ) ;
#166970=CARTESIAN_POINT ( 'NONE',  ( 5.345657705538078730, 9.458627433094950021, 0.7998128361456331437 ) ) ;
#166979=CARTESIAN_POINT ( 'NONE',  ( -5.015689319493858100, 6.483061930202996592, 1.345460504475339159 ) ) ;
#166985=CARTESIAN_POINT ( 'NONE',  ( 5.413027408713817046, 7.651055653456078076, -1.328921179265474262 ) ) ;
#167007=CARTESIAN_POINT ( 'NONE',  ( 5.833751235630055376, 10.02806988486892514, 0.7998128361456331437 ) ) ;
#167012=CARTESIAN_POINT ( 'NONE',  ( -6.510788175286835511, 6.826513026331759271, 0.5708727117093035375 ) ) ;
#167014=CARTESIAN_POINT ( 'NONE',  ( 5.484430959185961463, 6.043327615839654499, 0.8208683321978844649 ) ) ;
#167028=CARTESIAN_POINT ( 'NONE',  ( -4.281342646865346602, 8.216926531310035031, 0.7998128361456352531 ) ) ;
#167044=CARTESIAN_POINT ( 'NONE',  ( 6.717138760927786834, 6.801359740696030443, -0.7998128361456481317 ) ) ;
#167047=CARTESIAN_POINT ( 'NONE',  ( 5.031484404002867450, 8.884165881396448583, 0.7216878364870317197 ) ) ;
#167055=EDGE_CURVE ( 'NONE', #23394, #212524, #212867, .T. ) ;
#167061=CARTESIAN_POINT ( 'NONE',  ( -6.473091995881817162, 6.516638514809040217, 0.7998128361456281477 ) ) ;
#167062=CARTESIAN_POINT ( 'NONE',  ( 4.030516805012513082, 7.924296382481737844, 0.000000000000000000 ) ) ;
#167071=CARTESIAN_POINT ( 'NONE',  ( -3.546339698426324460, 6.295090860542775779, -1.199719254218450271 ) ) ;
#167072=CARTESIAN_POINT ( 'NONE',  ( 5.096939404094710468, 4.911127157724081371, 0.000000000000000000 ) ) ;
#167074=CARTESIAN_POINT ( 'NONE',  ( 4.913904330310220558, 4.697586238308844919, 0.000000000000000000 ) ) ;
#167081=CARTESIAN_POINT ( 'NONE',  ( 5.337069745634900997, 6.255611453776062980, 1.199719254218452047 ) ) ;
#167083=CARTESIAN_POINT ( 'NONE',  ( 6.737475991348287785, 6.825086509519945999, -0.7998128361456481317 ) ) ;
#167088=CARTESIAN_POINT ( 'NONE',  ( -6.239605170154193026, 7.010755437975583426, 1.009914170685573875 ) ) ;
#167098=CARTESIAN_POINT ( 'NONE',  ( -6.474900878978163021, 9.711745571186627402, -1.199719254218452047 ) ) ;
#167104=CARTESIAN_POINT ( 'NONE',  ( -6.178787966739591297, 5.309377612922442147, 2.438151698559690939 ) ) ;
#167109=CARTESIAN_POINT ( 'NONE',  ( 3.851925040058331806, 5.587274861525073355, -1.443375672974066548 ) ) ;
#167112=CARTESIAN_POINT ( 'NONE',  ( -7.006746397889327405, 6.052176462752765218, 2.500000000000000000 ) ) ;
#167129=CARTESIAN_POINT ( 'NONE',  ( 6.222266154028957885, 6.224008365980749247, 0.7998128361456350310 ) ) ;
#167147=CARTESIAN_POINT ( 'NONE',  ( 0.4598555752060234925, 3.132870877575693935, 1.947419802861296123 ) ) ;
#167149=CARTESIAN_POINT ( 'NONE',  ( 5.391302360089590628, 6.318882837306503575, -1.199719254218452047 ) ) ;
#167150=CARTESIAN_POINT ( 'NONE',  ( -3.499413046103020175, 7.096749297179887783, 0.7216878364870338292 ) ) ;
#167174=CARTESIAN_POINT ( 'NONE',  ( -6.119526231721793330, 8.232809585132461194, 1.599625672291263179 ) ) ;
#167179=CARTESIAN_POINT ( 'NONE',  ( -2.986538976760251263, 6.706322249520737522, -0.7998128361456481317 ) ) ;
#167187=CARTESIAN_POINT ( 'NONE',  ( -6.099189001301292379, 8.209082816308541197, 1.599625672291263179 ) ) ;
#167199=CARTESIAN_POINT ( 'NONE',  ( -5.611095471209320174, 7.639640364534566075, 1.599625672291263179 ) ) ;
#167202=CARTESIAN_POINT ( 'NONE',  ( -7.268579750702160780, 8.613002809641560731, -1.082531754730549967 ) ) ;
#167206=CARTESIAN_POINT ( 'NONE',  ( 3.241808126998965811, 6.796210224891872542, 0.7216878364870257245 ) ) ;
#167207=EDGE_CURVE ( 'NONE', #191915, #60728, #168678, .T. ) ;
#167208=CARTESIAN_POINT ( 'NONE',  ( -7.014364370223741929, 9.276787413384745662, -1.599625672291271394 ) ) ;
#167210=ORIENTED_EDGE ( 'NONE', *, *, #181214, .T. ) ;
#167222=CARTESIAN_POINT ( 'NONE',  ( 0.2923534576129138141, 2.707453654964923739, 2.053134718767547273 ) ) ;
#167227=CARTESIAN_POINT ( 'NONE',  ( 6.604365638557201379, 6.767254738080503706, -0.09251035838216993545 ) ) ;
#167246=CARTESIAN_POINT ( 'NONE',  ( 6.450676980830294838, 6.774405823990504949, -0.3487213023658369826 ) ) ;
#167249=CIRCLE ( 'NONE', #98149, 1.250000000000000888 ) ;
#167257=EDGE_CURVE ( 'NONE', #150264, #153847, #49757, .T. ) ;
#167263=FACE_OUTER_BOUND ( 'NONE', #194000, .T. ) ;
#167268=CARTESIAN_POINT ( 'NONE',  ( -5.631432701629818460, 7.663367133358481631, 1.599625672291263179 ) ) ;
#167272=CARTESIAN_POINT ( 'NONE',  ( -7.553300976144787349, 8.945177572657957654, -1.082531754730549967 ) ) ;
#167281=CARTESIAN_POINT ( 'NONE',  ( 6.333594036239346359, 7.418223126147930557, 1.199719254218453823 ) ) ;
#167283=CARTESIAN_POINT ( 'NONE',  ( 6.343235766347262938, 8.493804042195527870, -1.599625672291281386 ) ) ;
#167288=CARTESIAN_POINT ( 'NONE',  ( -6.794044373779495771, 8.059378203231773341, 1.082531754730549078 ) ) ;
#167293=CARTESIAN_POINT ( 'NONE',  ( 6.013923656113508542, 9.173938811177871244, -1.199719254218452047 ) ) ;
#167299=DIRECTION ( 'NONE',  ( 0.000000000000000000, -1.000000000000000000, 0.000000000000000000 ) ) ;
#167306=CARTESIAN_POINT ( 'NONE',  ( -6.631346530859867805, 6.909194838857525944, 0.000000000000000000 ) ) ;
#167307=CARTESIAN_POINT ( 'NONE',  ( 5.722950238744200391, 7.770137593325314285, 1.443375672974065660 ) ) ;
#167317=CARTESIAN_POINT ( 'NONE',  ( -3.637330350216213759, 7.465578851886037093, -0.7998128361456481317 ) ) ;
#167318=CARTESIAN_POINT ( 'NONE',  ( -6.563555762791521531, 9.711213252348503744, 1.082531754730549967 ) ) ;
#167321=CARTESIAN_POINT ( 'NONE',  ( 5.844973620822844218, 6.952128991449046502, 1.082531754730549967 ) ) ;
#167334=CARTESIAN_POINT ( 'NONE',  ( -6.265474751258844677, 6.912123529488261475, 0.7890932636151950508 ) ) ;
#167339=CARTESIAN_POINT ( 'NONE',  ( 3.716343503921665459, 6.389465617000312569, -1.082531754730549967 ) ) ;
#167342=CARTESIAN_POINT ( 'NONE',  ( -6.629010762438975135, 6.698543742459062145, -0.7998128361456362523 ) ) ;
#167354=EDGE_CURVE ( 'NONE', #162324, #65240, #101547, .T. ) ;
#167355=CARTESIAN_POINT ( 'NONE',  ( 5.011674058906918638, 5.875983152593414971, 1.199719254218452047 ) ) ;
#167391=CARTESIAN_POINT ( 'NONE',  ( 4.719646871332936477, 8.520355426614829142, -0.7216878364870357165 ) ) ;
#167397=CARTESIAN_POINT ( 'NONE',  ( 4.706088717274885092, 8.504537580213796133, 0.7216878364870317197 ) ) ;
#167411=CARTESIAN_POINT ( 'NONE',  ( -7.618755976236585958, 7.853246491889623648, 0.000000000000000000 ) ) ;
#167423=CARTESIAN_POINT ( 'NONE',  ( 5.682275777458854371, 5.801945626556378244, 0.7216878364870328300 ) ) ;
#167428=CARTESIAN_POINT ( 'NONE',  ( -5.399890319992785237, 9.521898816625391504, 0.7998128361456291469 ) ) ;
#167433=CARTESIAN_POINT ( 'NONE',  ( -6.956742217587851052, 7.288823140040177506, 0.000000000000000000 ) ) ;
#167436=CARTESIAN_POINT ( 'NONE',  ( -4.911796789900812144, 8.952456364851418158, 0.7998128361456291469 ) ) ;
#167455=CARTESIAN_POINT ( 'NONE',  ( -3.011319516011047082, 6.527306845405913549, 0.7216878364870328300 ) ) ;
#167456=ORIENTED_EDGE ( 'NONE', *, *, #28350, .F. ) ;
#167457=CARTESIAN_POINT ( 'NONE',  ( -4.950135482320926705, 6.868520377498098739, -1.443375672974066548 ) ) ;
#167458=CARTESIAN_POINT ( 'NONE',  ( 6.059568310664962709, 6.034194215389424798, 0.7998128361456352531 ) ) ;
#167460=CARTESIAN_POINT ( 'NONE',  ( -4.492547798081878874, 6.334668079219206049, 1.599625672291263179 ) ) ;
#167461=CARTESIAN_POINT ( 'NONE',  ( -5.173318132066234476, 8.193232366456022930, -1.199719254218453823 ) ) ;
#167514=CARTESIAN_POINT ( 'NONE',  ( 5.246079093845007257, 5.085123462432798114, 0.7998128361456352531 ) ) ;
#167526=CARTESIAN_POINT ( 'NONE',  ( 4.596293493935747598, 8.372084169494645067, 0.08663659024946840370 ) ) ;
#167529=CARTESIAN_POINT ( 'NONE',  ( 3.715816618597135523, 6.492813934075403637, -1.199719254218453823 ) ) ;
#167535=CARTESIAN_POINT ( 'NONE',  ( -6.947627372360122955, 7.070263120700404968, 0.000000000000000000 ) ) ;
#167548=CARTESIAN_POINT ( 'NONE',  ( 4.421367491832258523, 8.172362817197399210, 0.7216878364870257245 ) ) ;
#167551=CARTESIAN_POINT ( 'NONE',  ( -3.959863383643135393, 6.777535159962392086, 1.199719254218452935 ) ) ;
#167559=ORIENTED_EDGE ( 'NONE', *, *, #158769, .T. ) ;
#167563=CARTESIAN_POINT ( 'NONE',  ( 4.848976215542928792, 5.686169002002086970, 1.199719254218452047 ) ) ;
#167564=CARTESIAN_POINT ( 'NONE',  ( 4.736594563127852098, 6.619389305106191834, -1.599625672291273171 ) ) ;
#167597=CARTESIAN_POINT ( 'NONE',  ( 7.205232291019763480, 7.370802192470005565, -0.7998128361456341429 ) ) ;
#167598=CARTESIAN_POINT ( 'NONE',  ( 2.889872605471108802, 6.605953636083950364, -2.500000000000002220 ) ) ;
#167603=CARTESIAN_POINT ( 'NONE',  ( 4.584065335196261692, 7.401807753487379848, 1.082531754730549078 ) ) ;
#167606=CARTESIAN_POINT ( 'NONE',  ( 5.885648082108177803, 9.880690172519326353, 0.7216878364870317197 ) ) ;
#167607=ORIENTED_EDGE ( 'NONE', *, *, #144373, .F. ) ;
#167618=CARTESIAN_POINT ( 'NONE',  ( 6.206332990038123221, 6.936436922908462144, -0.8583981852504622978 ) ) ;
#167619=CARTESIAN_POINT ( 'NONE',  ( -6.834718835064852449, 8.106831741398025315, 1.082531754730549078 ) ) ;
#167651=CARTESIAN_POINT ( 'NONE',  ( 5.342795052237045539, 8.390955439988655229, -1.199719254218450271 ) ) ;
#167653=CARTESIAN_POINT ( 'NONE',  ( 5.677832469072920496, 9.846164657218904992, 0.000000000000000000 ) ) ;
#167666=CARTESIAN_POINT ( 'NONE',  ( -4.634908411025374875, 6.500755460986618495, 1.599625672291263179 ) ) ;
#167668=CARTESIAN_POINT ( 'NONE',  ( 5.926322542504858681, 8.007405281046052536, -1.443375672974078761 ) ) ;
#167684=CARTESIAN_POINT ( 'NONE',  ( -7.946487431385463651, 8.443525889470736345, 0.7216878364870317197 ) ) ;
#167686=CARTESIAN_POINT ( 'NONE',  ( -5.261973015879593873, 8.192700047617899273, 1.082531754730549967 ) ) ;
#167710=CARTESIAN_POINT ( 'NONE',  ( -6.466312919074983512, 6.508729591867735031, -0.7998128361456362523 ) ) ;
#167723=CARTESIAN_POINT ( 'NONE',  ( -4.609429383499759503, 8.467968972964683871, -0.3232828671759068739 ) ) ;
#167741=CARTESIAN_POINT ( 'NONE',  ( 5.688527969385528849, 8.794310509995222347, -1.199719254218452047 ) ) ;
#167764=CARTESIAN_POINT ( 'NONE',  ( 7.205232291019763480, 7.370802192470005565, -0.7998128361456341429 ) ) ;
#167765=CARTESIAN_POINT ( 'NONE',  ( 5.468734858265785093, 7.473552982767158070, 1.599625672291269396 ) ) ;
#167767=CARTESIAN_POINT ( 'NONE',  ( 6.391743074199808916, 6.421731439513382433, -0.7998128361456481317 ) ) ;
#167781=CARTESIAN_POINT ( 'NONE',  ( 4.937886321289528979, 7.980522944944189234, -1.013380012275147291 ) ) ;
#167783=CARTESIAN_POINT ( 'NONE',  ( -4.448483798615272100, 8.203998508444197313, 0.000000000000000000 ) ) ;
#167784=CARTESIAN_POINT ( 'NONE',  ( 3.743459811148990291, 7.381470523066878009, -0.7216878364870338292 ) ) ;
#167803=CARTESIAN_POINT ( 'NONE',  ( -5.112833325684920993, 6.097965313788082931, -1.082531754730549967 ) ) ;
#167808=CARTESIAN_POINT ( 'NONE',  ( 5.345657705538078730, 9.458627433094950021, 0.7998128361456331437 ) ) ;
#167835=CARTESIAN_POINT ( 'NONE',  ( 6.047819040147648373, 9.213483425884394507, 1.199719254218452047 ) ) ;
#167839=CARTESIAN_POINT ( 'NONE',  ( -5.303700083894403505, 7.646886670761364968, 1.227282432737321294 ) ) ;
#167840=CARTESIAN_POINT ( 'NONE',  ( 7.713663051532233972, 7.963971413067895355, -0.7998128361456341429 ) ) ;
#167872=CARTESIAN_POINT ( 'NONE',  ( -6.740338644649361832, 7.892758502626242567, -1.199719254218452047 ) ) ;
#167874=CARTESIAN_POINT ( 'NONE',  ( 5.515134625708930649, 9.656350506627580543, 0.000000000000000000 ) ) ;
#167877=CARTESIAN_POINT ( 'NONE',  ( -2.875737979874388284, 6.369128386579808954, -0.7216878364870458196 ) ) ;
#167888=CARTESIAN_POINT ( 'NONE',  ( -5.926322542504887991, 6.086666852443358700, -0.7216878364870307205 ) ) ;
#167896=CARTESIAN_POINT ( 'NONE',  ( 8.018721507839716267, 8.319872945426633137, -0.7998128361456341429 ) ) ;
#167907=CARTESIAN_POINT ( 'NONE',  ( 7.539742822975472158, 7.968990512992423447, -0.7216878364870317197 ) ) ;
#167921=CARTESIAN_POINT ( 'NONE',  ( -6.780486220610195680, 7.083191143566240910, -0.7216878364870338292 ) ) ;
#167923=CARTESIAN_POINT ( 'NONE',  ( 7.201315867513990554, 8.430565262634994284, -1.199719254218452047 ) ) ;
#167926=CARTESIAN_POINT ( 'NONE',  ( -8.093291352714894415, 8.406871097780989288, -0.7998128361456362523 ) ) ;
#167928=CARTESIAN_POINT ( 'NONE',  ( -5.490125858891038213, 5.369844688319787451, -0.7998128361456362523 ) ) ;
#167930=DIRECTION ( 'NONE',  ( 0.000000000000000000, 1.000000000000000000, 0.000000000000000000 ) ) ;
#167967=CARTESIAN_POINT ( 'NONE',  ( 3.418064124421011041, 7.001842221884225559, -0.7216878364870338292 ) ) ;
#167972=CARTESIAN_POINT ( 'NONE',  ( 3.393283585170187688, 7.180857625999046867, 0.7998128361456271485 ) ) ;
#167975=CARTESIAN_POINT ( 'NONE',  ( -4.288121723672178476, 8.224835454251337552, -0.7998128361456362523 ) ) ;
#167979=CARTESIAN_POINT ( 'NONE',  ( -6.902509602688830626, 7.225551755991315162, -0.7216878364870338292 ) ) ;
#167986=CARTESIAN_POINT ( 'NONE',  ( -6.017840079619296567, 8.114175741012878973, -1.599625672291271394 ) ) ;
#167992=DIRECTION ( 'NONE',  ( 0.000000000000000000, -1.000000000000000000, -1.496258514059622730E-16 ) ) ;
#167994=CARTESIAN_POINT ( 'NONE',  ( -4.769436176957319695, 8.786368983084006601, 0.7998128361456281477 ) ) ;
#167996=CARTESIAN_POINT ( 'NONE',  ( 4.626831674679969808, 8.450518883791096059, -0.3637425496919588497 ) ) ;
#168001=CARTESIAN_POINT ( 'NONE',  ( 7.666209513884374438, 7.908608952478760834, 0.7998128361456281477 ) ) ;
#168008=CARTESIAN_POINT ( 'NONE',  ( -6.818824913030298696, 6.919993584815607335, 0.7998128361456341429 ) ) ;
#168011=AXIS2_PLACEMENT_3D ( 'NONE', #33742, #86764, #99820 ) ;
#168013=CARTESIAN_POINT ( 'NONE',  ( -7.435720902452096936, 7.639705572474380091, 0.000000000000000000 ) ) ;
#168019=CARTESIAN_POINT ( 'NONE',  ( -7.146556367734805626, 9.431011410480991231, 1.443375672974064550 ) ) ;
#168025=CARTESIAN_POINT ( 'NONE',  ( 7.503511670520385479, 7.718794801887437274, 0.7998128361456281477 ) ) ;
#168036=CARTESIAN_POINT ( 'NONE',  ( -6.468692700515624949, 6.719432036793461904, 1.751973777778555601E-06 ) ) ;
#168041=CARTESIAN_POINT ( 'NONE',  ( 5.178155719255617129, 7.862379301422712352, -1.251444257556088457 ) ) ;
#168071=CARTESIAN_POINT ( 'NONE',  ( -6.477282242306868554, 6.848760321534919093, 0.6499626829332164624 ) ) ;
#168089=B_SPLINE_CURVE_WITH_KNOTS ( 'NONE', 3,
 ( #89700, #109202, #155750, #27874 ),
 .UNSPECIFIED., .F., .F.,
 ( 4, 4 ),
 ( 0.000000000000000000, 0.0003289350697890357504 ),
 .UNSPECIFIED. ) ;
#168091=CARTESIAN_POINT ( 'NONE',  ( -5.468734858265826837, 7.473552982767158070, 1.599625672291263179 ) ) ;
#168107=CARTESIAN_POINT ( 'NONE',  ( 4.857564175446106525, 8.889184981320973122, 0.7998128361456331437 ) ) ;
#168108=CARTESIAN_POINT ( 'NONE',  ( 4.947799714344386146, 4.737130853015369958, -0.7998128361456481317 ) ) ;
#168110=CARTESIAN_POINT ( 'NONE',  ( 5.519577934094851202, 8.493239118869080784, 1.082531754730547524 ) ) ;
#168122=CARTESIAN_POINT ( 'NONE',  ( -6.394605727500880299, 7.489403432619674561, -1.199719254218452047 ) ) ;
#168123=CARTESIAN_POINT ( 'NONE',  ( 5.716698046817569434, 6.698511138489155137, -1.199719254218452047 ) ) ;
#168131=CARTESIAN_POINT ( 'NONE',  ( -4.625266680917477835, 5.425174544939014964, -1.199719254218453823 ) ) ;
#168132=CARTESIAN_POINT ( 'NONE',  ( 5.259637247458703868, 5.100941308315409373, 0.000000000000000000 ) ) ;
#168139=CARTESIAN_POINT ( 'NONE',  ( 4.712340909201580885, 7.655425606447271214, -1.199719254218452047 ) ) ;
#168146=CARTESIAN_POINT ( 'NONE',  ( -5.012442140716328431, 8.020463026761962766, 1.150573971286508845 ) ) ;
#168152=EDGE_CURVE ( 'NONE', #207114, #85668, #603, .T. ) ;
#168157=CARTESIAN_POINT ( 'NONE',  ( -3.146901051703345331, 6.685485303713597283, 0.000000000000000000 ) ) ;
#168167=CARTESIAN_POINT ( 'NONE',  ( 4.963693636378940788, 5.923969009597785274, -1.082531754730548412 ) ) ;
#168169=CARTESIAN_POINT ( 'NONE',  ( -5.717509255324703332, 7.006698007003612894, 2.500000000000000444 ) ) ;
#168170=CARTESIAN_POINT ( 'NONE',  ( -6.635789839245807897, 6.706452665400368218, 0.7998128361456341429 ) ) ;
#168187=CARTESIAN_POINT ( 'NONE',  ( 5.910428620914669473, 5.860197910680708944, 0.000000000000000000 ) ) ;
#168206=CARTESIAN_POINT ( 'NONE',  ( -0.4152101148468765324, 3.244511181007482481, 1.956683416369788819 ) ) ;
#168208=CARTESIAN_POINT ( 'NONE',  ( 4.583538449871731757, 7.505156070562471804, 1.199719254218451159 ) ) ;
#168209=CARTESIAN_POINT ( 'NONE',  ( -5.980555157403903976, 6.149938236492225485, 0.000000000000000000 ) ) ;
#168235=CARTESIAN_POINT ( 'NONE',  ( -7.442499979258930587, 7.647614495415686164, -0.7998128361456362523 ) ) ;
#168248=CARTESIAN_POINT ( 'NONE',  ( -5.562588163356775972, 9.711712967216715953, 0.7998128361456291469 ) ) ;
#168255=CARTESIAN_POINT ( 'NONE',  ( 6.204464077730128757, 7.037555732820855781, 1.030856974308017149 ) ) ;
#168260=CARTESIAN_POINT ( 'NONE',  ( -4.749098946536820520, 8.762642214260091933, 0.7998128361456281477 ) ) ;
#168263=CARTESIAN_POINT ( 'NONE',  ( -7.919371124158132602, 8.411890197705517380, -0.7216878364870338292 ) ) ;
#168267=CARTESIAN_POINT ( 'NONE',  ( -7.146556367734805626, 9.431011410480991231, 1.443375672974064550 ) ) ;
#168268=CARTESIAN_POINT ( 'NONE',  ( 4.326460416092276162, 7.101268681199365496, -1.082531754730548412 ) ) ;
#168269=CARTESIAN_POINT ( 'NONE',  ( -4.082413651046300274, 6.816547455312373494, 1.082531754730549967 ) ) ;
#168284=CARTESIAN_POINT ( 'NONE',  ( 0.4149352601330746348, 2.754396095944236400, 1.956746367768555706 ) ) ;
#168290=CARTESIAN_POINT ( 'NONE',  ( 6.400241882075590638, 6.902609158730609096, 0.7749192096189911894 ) ) ;
#168294=CARTESIAN_POINT ( 'NONE',  ( 6.204464077730128757, 7.037555732820855781, 1.030856974308017149 ) ) ;
#168309=CARTESIAN_POINT ( 'NONE',  ( 5.960708871395055120, 7.108654626955757116, 1.090683939682752124 ) ) ;
#168329=CARTESIAN_POINT ( 'NONE',  ( -4.782994330570982555, 8.802186828966616972, 0.000000000000000000 ) ) ;
#168341=CARTESIAN_POINT ( 'NONE',  ( 6.710359684120930091, 6.793450817754725257, 0.7998128361456352531 ) ) ;
#168347=DIRECTION ( 'NONE',  ( -1.000000000000000000, 0.000000000000000000, 0.000000000000000000 ) ) ;
#168350=CARTESIAN_POINT ( 'NONE',  ( -5.600926855776882540, 8.588146194164741232, -1.082531754730549967 ) ) ;
#168354=CARTESIAN_POINT ( 'NONE',  ( 5.691390622686558487, 9.861982503101517139, 0.7998128361456341429 ) ) ;
#168368=CARTESIAN_POINT ( 'NONE',  ( -5.316205630334251531, 9.216340645449683677, -0.7216878364870338292 ) ) ;
#168369=CARTESIAN_POINT ( 'NONE',  ( 6.265276383290871109, 7.442482214328385304, -1.082531754730548412 ) ) ;
#168373=EDGE_LOOP ( 'NONE', ( #116807, #89546, #192227, #187235 ) ) ;
#168374=CARTESIAN_POINT ( 'NONE',  ( 4.814553946184248368, 7.670711132973337065, -1.082531754730548412 ) ) ;
#168378=CARTESIAN_POINT ( 'NONE',  ( -4.878955176071358757, 6.785476686873604280, -1.599625672291271394 ) ) ;
#168379=CARTESIAN_POINT ( 'NONE',  ( -3.851398154733808088, 6.650992392901508232, -1.199719254218450271 ) ) ;
#168382=CARTESIAN_POINT ( 'NONE',  ( 6.495764994278809823, 7.711385593814346073, 1.082531754730549967 ) ) ;
#168394=CARTESIAN_POINT ( 'NONE',  ( -4.721755537811513470, 8.238515690766082145, -0.6557258408305451924 ) ) ;
#168398=CARTESIAN_POINT ( 'NONE',  ( -5.798199202927275309, 6.683866596142988392, 0.9905280086691092833 ) ) ;
#168399=CARTESIAN_POINT ( 'NONE',  ( 4.014622883422321209, 5.777089012116397804, -1.443375672974068769 ) ) ;
#168403=CARTESIAN_POINT ( 'NONE',  ( -5.468734858265826837, 7.473552982767158070, 1.599625672291263179 ) ) ;
#168414=CARTESIAN_POINT ( 'NONE',  ( 7.024532985656128936, 9.288650798055913427, 1.443375672974065660 ) ) ;
#168449=CARTESIAN_POINT ( 'NONE',  ( 5.180624094197585627, 8.097792972322238825, -1.082531754730548412 ) ) ;
#168454=CARTESIAN_POINT ( 'NONE',  ( 4.841670253411575864, 8.662716039039905169, -0.7216878364870458196 ) ) ;
#168468=CARTESIAN_POINT ( 'NONE',  ( -5.921879234118920365, 10.13088588310589699, 0.000000000000000000 ) ) ;
#168470=CARTESIAN_POINT ( 'NONE',  ( -6.050681693448748177, 10.28115541899069463, 0.7998128361456291469 ) ) ;
#168480=CARTESIAN_POINT ( 'NONE',  ( 5.546694241322223107, 5.643767167730274537, -0.7216878364870458196 ) ) ;
#168486=CARTESIAN_POINT ( 'NONE',  ( -7.208094944320834863, 8.438474185576302133, -1.199719254218452047 ) ) ;
#168491=CARTESIAN_POINT ( 'NONE',  ( -5.139949633356594383, 9.010708648975750634, 0.000000000000000000 ) ) ;
#168495=CARTESIAN_POINT ( 'NONE',  ( -6.505933609711270549, 8.683618192786854095, -1.599625672291271394 ) ) ;
#168513=CARTESIAN_POINT ( 'NONE',  ( 3.179715765502657554, 5.975770656120749535, -2.420000000000002149 ) ) ;
#168514=CARTESIAN_POINT ( 'NONE',  ( -4.665414256878304577, 5.575976400180357118, -1.082531754730549967 ) ) ;
#168517=CARTESIAN_POINT ( 'NONE',  ( -5.438229012412911345, 5.517224400669388018, -0.7216878364870338292 ) ) ;
#168519=CARTESIAN_POINT ( 'NONE',  ( 5.574337433874081427, 6.532423756721743580, -1.199719254218452047 ) ) ;
#168520=CARTESIAN_POINT ( 'NONE',  ( -4.118644803501354978, 8.027112380718707030, 0.7998128361456352531 ) ) ;
#168521=CARTESIAN_POINT ( 'NONE',  ( -6.770317605177755382, 8.992066187497757213, 1.599625672291269396 ) ) ;
#168522=ORIENTED_EDGE ( 'NONE', *, *, #132650, .F. ) ;
#168573=CARTESIAN_POINT ( 'NONE',  ( 5.086243903782109221, 5.962981304947771122, -1.199719254218452047 ) ) ;
#168575=DIRECTION ( 'NONE',  ( 1.000000000000000000, 0.000000000000000000, 0.000000000000000000 ) ) ;
#168578=AXIS2_PLACEMENT_3D ( 'NONE', #44394, #81145, #77940 ) ;
#168586=CARTESIAN_POINT ( 'NONE',  ( 4.700249516990034238, 8.244041944096728969, -0.6212051699984559860 ) ) ;
#168589=CARTESIAN_POINT ( 'NONE',  ( 5.065906673361608270, 5.939254536123854677, -1.199719254218450271 ) ) ;
#168596=CARTESIAN_POINT ( 'NONE',  ( -7.435720902452096936, 7.639705572474380091, 0.000000000000000000 ) ) ;
#168609=CARTESIAN_POINT ( 'NONE',  ( 4.855228407469603269, 7.718164671139588151, -1.082531754730548412 ) ) ;
#168612=CARTESIAN_POINT ( 'NONE',  ( -4.762657100150483380, 8.778460060142702304, 0.000000000000000000 ) ) ;
#168623=CARTESIAN_POINT ( 'NONE',  ( 5.065906673361608270, 5.939254536123854677, -1.199719254218450271 ) ) ;
#168624=CARTESIAN_POINT ( 'NONE',  ( 6.574778147984297938, 6.635272358928617997, -0.7998128361456481317 ) ) ;
#168645=CARTESIAN_POINT ( 'NONE',  ( 6.142241479726070708, 7.081583759122534794, -1.089790755372788800 ) ) ;
#168653=CARTESIAN_POINT ( 'NONE',  ( 4.543917759235442944, 5.330267469643351852, 1.199719254218452935 ) ) ;
#168658=CARTESIAN_POINT ( 'NONE',  ( 6.261886844665240481, 8.398896966899865646, 1.599625672291268286 ) ) ;
#168664=CARTESIAN_POINT ( 'NONE',  ( 4.746763178560250651, 7.591621904078704297, 1.082531754730549078 ) ) ;
#168667=CARTESIAN_POINT ( 'NONE',  ( 8.014278199453778839, 8.522615118883788199, 0.000000000000000000 ) ) ;
#168678=B_SPLINE_CURVE_WITH_KNOTS ( 'NONE', 3,
 ( #211326, #129120, #97615, #209185, #195097, #112846, #14181, #212387, #15255, #196167, #126986, #160460, #108213, #25809, #172082, #8496, #27954, #206697, #205623, #10619, #209878, #126604, #192567, #76694, #109282, #91919 ),
 .UNSPECIFIED., .F., .F.,
 ( 4, 2, 1, 1, 1, 1, 2, 2, 2, 2, 2, 2, 2, 2, 4 ),
 ( 0.02490545872912452649, 0.02512859161056170063, 0.02535172449199887129, 0.02579799025487321956, 0.02669052178062191263, 0.02847558483211929531, 0.03204571093511406066, 0.03918596314110360523, 0.05346646755308270826, 0.06774697196506181129, 0.08202747637704091432, 0.09630798078902001735, 0.1105884852009991343, 0.1248689896129782373, 0.1391494940249573542 ),
 .UNSPECIFIED. ) ;
#168680=CARTESIAN_POINT ( 'NONE',  ( 6.479309170914094196, 6.755949689298615723, 0.1985876171829506487 ) ) ;
#168681=CARTESIAN_POINT ( 'NONE',  ( -5.953438850176548947, 9.959779401932374654, 0.000000000000000000 ) ) ;
#168685=CARTESIAN_POINT ( 'NONE',  ( 3.188928480291308265, 8.980740528189235405, 2.451733079074510879 ) ) ;
#168689=FACE_OUTER_BOUND ( 'NONE', #57825, .T. ) ;
#168715=CARTESIAN_POINT ( 'NONE',  ( 6.367489420273535039, 7.457767740854454708, -1.199719254218452047 ) ) ;
#168718=CARTESIAN_POINT ( 'NONE',  ( 6.984385409695311964, 8.177479728513226576, 1.199719254218452935 ) ) ;
#168732=CARTESIAN_POINT ( 'NONE',  ( -6.120580001926503755, 6.105374521861167914, -0.7998128361456362523 ) ) ;
#168735=CARTESIAN_POINT ( 'NONE',  ( 5.465345319640213972, 8.429967735338637524, -1.082531754730548412 ) ) ;
#168743=CARTESIAN_POINT ( 'NONE',  ( -4.767627293860968507, 5.591261926706423857, -1.199719254218453823 ) ) ;
#168750=CARTESIAN_POINT ( 'NONE',  ( -5.465345320084574965, 9.390336950158399532, 0.000000000000000000 ) ) ;
#168752=CARTESIAN_POINT ( 'NONE',  ( -5.966997003790228682, 8.054858819212300958, -1.443375672974066548 ) ) ;
#168760=CARTESIAN_POINT ( 'NONE',  ( 0.1472015564608893656, 3.384172088701932424, 2.075648132225481390 ) ) ;
#168764=VECTOR ( 'NONE', #7520, 1000.000000000000114 ) ;
#168775=CARTESIAN_POINT ( 'NONE',  ( -5.387385936583832802, 7.378645907471495846, -1.599625672291271394 ) ) ;
#168777=CARTESIAN_POINT ( 'NONE',  ( -3.383641855062333281, 6.105276709951447778, -1.199719254218452047 ) ) ;
#168782=CARTESIAN_POINT ( 'NONE',  ( -6.427974226210522168, 6.671927150099951298, 0.000000000000000000 ) ) ;
#168785=CARTESIAN_POINT ( 'NONE',  ( -5.188065202531182862, 7.850521293832936287, -1.269213148129512136 ) ) ;
#168800=CARTESIAN_POINT ( 'NONE',  ( 2.696596522755183578, 2.993039318081675226, 2.500000000000000444 ) ) ;
#168807=CARTESIAN_POINT ( 'NONE',  ( 4.647606103345025552, 8.407977806742819027, 0.6343139517084724899 ) ) ;
#168818=CARTESIAN_POINT ( 'NONE',  ( 3.562760505341037831, 7.378580699531681830, -1.734723475976807094E-15 ) ) ;
#168825=CARTESIAN_POINT ( 'NONE',  ( 6.170896192875352959, 7.228408975556602556, 1.199719254218453823 ) ) ;
#168827=CARTESIAN_POINT ( 'NONE',  ( 5.879395890181562834, 6.888325289080478697, -1.199719254218452047 ) ) ;
#168842=CARTESIAN_POINT ( 'NONE',  ( 5.010605496441194795, 7.906410611435644498, -1.080668833775387139 ) ) ;
#168844=CARTESIAN_POINT ( 'NONE',  ( -4.773879485343255347, 8.583626809626847987, 0.000000000000000000 ) ) ;
#168845=CARTESIAN_POINT ( 'NONE',  ( 5.397554552016226914, 6.430140077841320689, 1.082531754730549078 ) ) ;
#168863=CARTESIAN_POINT ( 'NONE',  ( -4.272227801637618505, 7.998366511970260717, 0.7216878364870338292 ) ) ;
#168867=CARTESIAN_POINT ( 'NONE',  ( 4.993145711582793744, 9.047363440147082159, -0.7998128361456481317 ) ) ;
#168874=SPHERICAL_SURFACE ( 'NONE', #141786, 0.08000000000000000167 ) ;
#168896=CARTESIAN_POINT ( 'NONE',  ( 6.831329296439236032, 9.063246493969506545, -1.599625672291267398 ) ) ;
#168899=CIRCLE ( 'NONE', #41058, 0.07999999999999984901 ) ;
#168907=DIRECTION ( 'NONE',  ( -0.000000000000000000, -1.000000000000000000, -0.000000000000000000 ) ) ;
#168927=CARTESIAN_POINT ( 'NONE',  ( 3.418064124421011041, 7.001842221884225559, -0.7216878364870338292 ) ) ;
#168935=CARTESIAN_POINT ( 'NONE',  ( 5.352436782344940802, 9.466536356036257871, 0.000000000000000000 ) ) ;
#168937=DIRECTION ( 'NONE',  ( 0.000000000000000000, 0.000000000000000000, -1.000000000000000000 ) ) ;
#168949=CARTESIAN_POINT ( 'NONE',  ( -4.950135482320926705, 6.868520377498098739, -1.443375672974066770 ) ) ;
#168956=CARTESIAN_POINT ( 'NONE',  ( 7.075376061485196821, 9.347967719856493218, 1.599625672291268286 ) ) ;
#168965=CARTESIAN_POINT ( 'NONE',  ( 3.984117037569365305, 5.741498858621315371, 1.599625672291261402 ) ) ;
#168968=DIRECTION ( 'NONE',  ( 0.000000000000000000, 1.000000000000000000, 0.000000000000000000 ) ) ;
#168981=CARTESIAN_POINT ( 'NONE',  ( -4.828112100242279325, 8.646898193675708555, -0.7216878364870338292 ) ) ;
#168983=CARTESIAN_POINT ( 'NONE',  ( 7.212011367826596242, 7.378711115411311638, 0.000000000000000000 ) ) ;
#168986=CARTESIAN_POINT ( 'NONE',  ( -6.420668264523499147, 9.648474187656182366, 1.199719254218452935 ) ) ;
#168989=CARTESIAN_POINT ( 'NONE',  ( -4.492547798081878874, 6.334668079219206049, 1.599625672291263179 ) ) ;
#169017=VERTEX_POINT ( 'NONE', #28812 ) ;
#169028=CARTESIAN_POINT ( 'NONE',  ( 5.085717018901939390, 5.105960408239938353, 0.000000000000000000 ) ) ;
#169032=CARTESIAN_POINT ( 'NONE',  ( -6.414942957921379474, 7.513130201443591005, -1.199719254218452047 ) ) ;
#169036=CARTESIAN_POINT ( 'NONE',  ( -4.111865726694519552, 8.019203457777400956, 0.000000000000000000 ) ) ;
#169037=CARTESIAN_POINT ( 'NONE',  ( -5.143339171537844479, 7.093924681584510061, 1.599625672291263401 ) ) ;
#169040=CARTESIAN_POINT ( 'NONE',  ( -6.251718229232867685, 6.466295153626015590, -0.7216878364870338292 ) ) ;
#169046=CARTESIAN_POINT ( 'NONE',  ( -6.611536185319534908, 7.742488966741438716, 1.199719254218452047 ) ) ;
#169052=CARTESIAN_POINT ( 'NONE',  ( 3.594580577241007102, 7.345424419493749468, 0.3531702171868136841 ) ) ;
#169054=CARTESIAN_POINT ( 'NONE',  ( -7.957709816578236506, 8.248692638954882028, 0.7998128361456341429 ) ) ;
#169056=CARTESIAN_POINT ( 'NONE',  ( 4.609415035364720303, 8.472105597856021575, 0.2450749143364742144 ) ) ;
#169061=CARTESIAN_POINT ( 'NONE',  ( 5.155843554946782703, 9.237177590738404831, -0.7998128361456481317 ) ) ;
#169084=CARTESIAN_POINT ( 'NONE',  ( 7.367930134383754215, 7.560616343061329125, -0.7998128361456341429 ) ) ;
#169088=CARTESIAN_POINT ( 'NONE',  ( -4.952079582221279530, 4.885585162322970021, 0.5000114801232704576 ) ) ;
#169093=CARTESIAN_POINT ( 'NONE',  ( -4.845788168165207743, 6.628691488484695249, 1.364795842686959526 ) ) ;
#169099=CARTESIAN_POINT ( 'NONE',  ( 5.612152705277200226, 7.484198595525810127, -1.333638438132278559 ) ) ;
#169100=CIRCLE ( 'NONE', #58397, 1.250000000000000888 ) ;
#169129=CARTESIAN_POINT ( 'NONE',  ( -6.253183873137761140, 7.001293123865100831, 0.9949814792902436089 ) ) ;
#169148=CARTESIAN_POINT ( 'NONE',  ( -5.306037014901836990, 7.283738832175834510, 1.599625672291263179 ) ) ;
#169159=VERTEX_POINT ( 'NONE', #62370 ) ;
#169165=CARTESIAN_POINT ( 'NONE',  ( 5.083381250481017410, 4.895309311841474553, 0.7998128361456352531 ) ) ;
#169167=CARTESIAN_POINT ( 'NONE',  ( 7.634649897826745857, 8.079715433652276957, 0.7216878364870267237 ) ) ;
#169176=CARTESIAN_POINT ( 'NONE',  ( -7.013428937081434000, 5.939655416065874327, -2.436399677959149468 ) ) ;
#169177=CARTESIAN_POINT ( 'NONE',  ( 6.346625304528514810, 6.577020074804287297, 0.000000000000000000 ) ) ;
#169181=CARTESIAN_POINT ( 'NONE',  ( -6.611536185319534908, 7.742488966741438716, 1.199719254218452047 ) ) ;
#169183=CARTESIAN_POINT ( 'NONE',  ( 6.391743074199808916, 6.421731439513382433, -0.7998128361456481317 ) ) ;
#169187=EDGE_CURVE ( 'NONE', #105939, #36876, #34772, .T. ) ;
#169193=CARTESIAN_POINT ( 'NONE',  ( -6.291865805193673111, 9.498204651771386509, -1.199719254218452047 ) ) ;
#169194=CARTESIAN_POINT ( 'NONE',  ( 3.410758162289653672, 6.136912401716668519, -1.199719254218453823 ) ) ;
#169201=CARTESIAN_POINT ( 'NONE',  ( 5.338878628731272613, 9.450718510153643948, -0.7998128361456481317 ) ) ;
#169208=CARTESIAN_POINT ( 'NONE',  ( -5.274058703912462676, 7.771439464937274444, 1.305864451146660388 ) ) ;
#169218=CARTESIAN_POINT ( 'NONE',  ( -5.438229012412903352, 6.477593614970734492, -1.082531754730549967 ) ) ;
#169227=CARTESIAN_POINT ( 'NONE',  ( 4.340018570150304456, 6.156717313299049366, -1.443375672974068769 ) ) ;
#169232=CARTESIAN_POINT ( 'NONE',  ( -6.557303570864871034, 7.679217583210999010, -1.199719254218452047 ) ) ;
#169246=CARTESIAN_POINT ( 'NONE',  ( 2.925527285498711549, 6.635141943048991742, 0.7998128361456281477 ) ) ;
#169251=MECHANICAL_DESIGN_GEOMETRIC_PRESENTATION_REPRESENTATION('',(#68881),#124357);
#169252=CARTESIAN_POINT ( 'NONE',  ( 3.716313722480235615, 7.557726119527409914, -0.5394532061484574870 ) ) ;
#169273=CARTESIAN_POINT ( 'NONE',  ( 5.740951700743842423, 5.662474837148078421, -0.7998128361456481317 ) ) ;
#169274=CARTESIAN_POINT ( 'NONE',  ( -4.177320726786315497, 7.887641591310407208, -0.7216878364870458196 ) ) ;
#169298=CARTESIAN_POINT ( 'NONE',  ( -6.149505192250180663, 9.332117270003974951, -1.199719254218452047 ) ) ;
#169300=CARTESIAN_POINT ( 'NONE',  ( 7.661766205054107992, 8.111351125417501251, -0.7216878364870317197 ) ) ;
#169313=CARTESIAN_POINT ( 'NONE',  ( -7.761116589180078407, 8.019333873657032541, 0.000000000000000000 ) ) ;
#169315=CARTESIAN_POINT ( 'NONE',  ( 5.120401779693986910, 7.917229619699595489, -1.217862772375446712 ) ) ;
#169320=CARTESIAN_POINT ( 'NONE',  ( 6.349632722739280588, 6.936441728539081808, -0.8798346732450362806 ) ) ;
#169326=CARTESIAN_POINT ( 'NONE',  ( -5.427006627220116286, 9.553534508390610469, -0.7998128361456362523 ) ) ;
#169330=CARTESIAN_POINT ( 'NONE',  ( -4.995253251992230581, 4.792493313604505367, 0.000000000000000000 ) ) ;
#169334=CARTESIAN_POINT ( 'NONE',  ( 5.519577934094864524, 5.612131475965050242, 0.7216878364870328300 ) ) ;
#169335=CARTESIAN_POINT ( 'NONE',  ( -4.787437638956935082, 6.678706226906775179, -1.443375672974066548 ) ) ;
#169342=FACE_OUTER_BOUND ( 'NONE', #114191, .T. ) ;
#169353=CARTESIAN_POINT ( 'NONE',  ( 5.966021608595377224, 7.209656400309186530, 1.216315744458285719 ) ) ;
#169356=CARTESIAN_POINT ( 'NONE',  ( 0.3633518834214408688, 2.686172036145575426, 1.968336656323642853 ) ) ;
#169358=FACE_OUTER_BOUND ( 'NONE', #18527, .T. ) ;
#169362=CARTESIAN_POINT ( 'NONE',  ( 7.361151057576892143, 7.552707420120024828, 0.7998128361456291469 ) ) ;
#169369=ADVANCED_FACE ( 'NONE', ( #17853 ), #133579, .T. ) ;
#169373=CARTESIAN_POINT ( 'NONE',  ( 5.685886686578042415, 7.314606927785019863, 1.221034997698521307 ) ) ;
#169391=CARTESIAN_POINT ( 'NONE',  ( -6.200875153403786477, 8.327716660428123419, -1.599625672291271394 ) ) ;
#169403=CARTESIAN_POINT ( 'NONE',  ( 6.170896192875352959, 7.228408975556602556, 1.199719254218453823 ) ) ;
#169414=FACE_OUTER_BOUND ( 'NONE', #163133, .T. ) ;
#169417=CARTESIAN_POINT ( 'NONE',  ( 3.702785349863636277, 7.334016984900627811, -0.7216878364870338292 ) ) ;
#169420=AXIS2_PLACEMENT_3D ( 'NONE', #1015, #48749, #84428 ) ;
#169430=CARTESIAN_POINT ( 'NONE',  ( -7.444835747679825033, 7.858265591814152629, 0.000000000000000000 ) ) ;
#169431=CARTESIAN_POINT ( 'NONE',  ( 6.373741612200171325, 7.569024981389272710, 1.082531754730549967 ) ) ;
#169437=ORIENTED_EDGE ( 'NONE', *, *, #74578, .T. ) ;
#169442=CARTESIAN_POINT ( 'NONE',  ( -3.461074353238556167, 7.259946855412102273, 0.000000000000000000 ) ) ;
#169443=CARTESIAN_POINT ( 'NONE',  ( -5.144392941742557568, 4.966489618313220333, -0.7998128361456362523 ) ) ;
#169445=CARTESIAN_POINT ( 'NONE',  ( 6.224601922005513543, 7.395028676162137771, -1.082531754730548412 ) ) ;
#169456=CARTESIAN_POINT ( 'NONE',  ( -4.607477032339801326, 8.379641378740778634, 0.1280868206084313787 ) ) ;
#169460=CARTESIAN_POINT ( 'NONE',  ( 3.445180431648323882, 6.073108699348104267, 1.082531754730549078 ) ) ;
#169465=CARTESIAN_POINT ( 'NONE',  ( -6.791708605802965870, 6.888357893050385705, -0.7998128361456362523 ) ) ;
#169478=CARTESIAN_POINT ( 'NONE',  ( 5.448397627845284141, 7.449826213943242514, 1.599625672291268286 ) ) ;
#169486=EDGE_CURVE ( 'NONE', #138513, #182199, #38030, .T. ) ;
#169514=EDGE_CURVE ( 'NONE', #60728, #2366, #191670, .T. ) ;
#169515=CARTESIAN_POINT ( 'NONE',  ( 4.895902868310594513, 8.725987423088758632, 0.000000000000000000 ) ) ;
#169521=CARTESIAN_POINT ( 'NONE',  ( 7.173672674962134899, 7.541908673643526129, -0.7216878364870317197 ) ) ;
#169535=CARTESIAN_POINT ( 'NONE',  ( -6.688968683495758683, 8.897159112202094988, -1.599625672291271394 ) ) ;
#169548=CARTESIAN_POINT ( 'NONE',  ( 4.624739795592929248, 6.488892076315451618, -1.443375672974068769 ) ) ;
#169554=CARTESIAN_POINT ( 'NONE',  ( -4.329849954717889915, 6.144853928627882489, 1.599625672291270506 ) ) ;
#169559=CARTESIAN_POINT ( 'NONE',  ( -5.302647476720585118, 9.200522799567075083, 0.000000000000000000 ) ) ;
#169562=CARTESIAN_POINT ( 'NONE',  ( -6.074935347375019390, 9.245119117649618801, 1.199719254218452047 ) ) ;
#169567=CARTESIAN_POINT ( 'NONE',  ( -3.122120512896910505, 6.864500708346841229, 0.7998128361456352531 ) ) ;
#169581=CARTESIAN_POINT ( 'NONE',  ( -5.153507786970276783, 6.145418851954329575, -1.082531754730549967 ) ) ;
#169583=CARTESIAN_POINT ( 'NONE',  ( -5.953438849732214599, 6.118302544208584770, 0.7216878364870257245 ) ) ;
#169585=CARTESIAN_POINT ( 'NONE',  ( 3.711900195091365262, 7.552577004240394132, -0.7998128361456362523 ) ) ;
#169586=CARTESIAN_POINT ( 'NONE',  ( -5.601453741101424022, 6.564059448486966986, -1.199719254218453823 ) ) ;
#169587=CARTESIAN_POINT ( 'NONE',  ( -7.306918443122272677, 7.489436036589583345, 0.7998128361456341429 ) ) ;
#169632=DIRECTION ( 'NONE',  ( 0.7592566023653005702, -0.6507913734559639396, 0.000000000000000000 ) ) ;
#169635=DIRECTION ( 'NONE',  ( 0.7771862570881703514, 0.6292706268317952434, 0.000000000000000000 ) ) ;
#169643=CARTESIAN_POINT ( 'NONE',  ( 6.249382461256315580, 6.255644057745969988, -0.7998128361456481317 ) ) ;
#169658=CARTESIAN_POINT ( 'NONE',  ( 4.193214648376505593, 8.114110533073061404, 0.000000000000000000 ) ) ;
#169663=ORIENTED_EDGE ( 'NONE', *, *, #140883, .F. ) ;
#169664=CARTESIAN_POINT ( 'NONE',  ( -6.774234028683526532, 7.932303117332766718, 1.199719254218452047 ) ) ;
#169668=CARTESIAN_POINT ( 'NONE',  ( 5.734172623936983904, 5.654565914206774124, 0.7998128361456352531 ) ) ;
#169673=CARTESIAN_POINT ( 'NONE',  ( -4.507082409677585666, 8.222350002982272699, 0.3272366024553932107 ) ) ;
#169678=CARTESIAN_POINT ( 'NONE',  ( 6.861835142292147083, 7.178098218861903135, 0.7216878364870328300 ) ) ;
#169680=CARTESIAN_POINT ( 'NONE',  ( -2.862179826260718762, 6.353310540697199471, 0.000000000000000000 ) ) ;
#169681=CARTESIAN_POINT ( 'NONE',  ( -4.274563570058511175, 8.209017608368725405, 0.000000000000000000 ) ) ;
#169693=CARTESIAN_POINT ( 'NONE',  ( 5.228604516725597229, 6.129068686715179126, -1.199719254218450271 ) ) ;
#169694=CARTESIAN_POINT ( 'NONE',  ( 6.886615681098613884, 6.999082814228660077, 0.000000000000000000 ) ) ;
#169712=CARTESIAN_POINT ( 'NONE',  ( 5.943507298343291723, 7.226397084328657350, -1.228854570503196575 ) ) ;
#169716=CARTESIAN_POINT ( 'NONE',  ( 6.142902043169038429, 7.013529245237516641, 0.9864344219776898237 ) ) ;
#169719=CARTESIAN_POINT ( 'NONE',  ( 4.245111494854632461, 7.966730820723463502, 0.000000000000000000 ) ) ;
#169721=CARTESIAN_POINT ( 'NONE',  ( 4.061549535745618833, 6.896169004081968090, -1.199719254218452047 ) ) ;
#169726=CARTESIAN_POINT ( 'NONE',  ( 5.020262018810099924, 9.078999131912302900, 0.7998128361456331437 ) ) ;
#169731=CARTESIAN_POINT ( 'NONE',  ( 5.560252395380206103, 8.540692657035327429, 1.082531754730547524 ) ) ;
#169734=CARTESIAN_POINT ( 'NONE',  ( 5.063044020060520900, 4.871582543017558109, 0.7998128361456352531 ) ) ;
#169746=CARTESIAN_POINT ( 'NONE',  ( 6.492781079782697695, 6.747302000852300807, 0.03582484399037785816 ) ) ;
#169748=CARTESIAN_POINT ( 'NONE',  ( -3.122120512896910505, 6.864500708346841229, 0.7998128361456352531 ) ) ;
#169765=ORIENTED_EDGE ( 'NONE', *, *, #381, .T. ) ;
#169772=CARTESIAN_POINT ( 'NONE',  ( 5.356880090730872013, 6.382686539675070492, 1.082531754730549078 ) ) ;
#169774=EDGE_CURVE ( 'NONE', #95128, #19248, #104447, .T. ) ;
#169781=CARTESIAN_POINT ( 'NONE',  ( 5.020262018810099924, 9.078999131912302900, 0.7998128361456331437 ) ) ;
#169783=CARTESIAN_POINT ( 'NONE',  ( 7.364013710877980401, 8.620379413226322285, -1.199719254218452047 ) ) ;
#169790=( LENGTH_UNIT ( ) NAMED_UNIT ( * ) SI_UNIT ( .MILLI., .METRE. ) );
#169797=CARTESIAN_POINT ( 'NONE',  ( -4.797606254389363833, 6.690569611577942943, 1.599625672291263179 ) ) ;
#169799=CARTESIAN_POINT ( 'NONE',  ( 5.356880090730857802, 8.303424968277756335, 1.082531754730548412 ) ) ;
#169808=CARTESIAN_POINT ( 'NONE',  ( -4.664887371553763096, 7.600063145858131364, -1.199719254218453823 ) ) ;
#169813=CARTESIAN_POINT ( 'NONE',  ( -5.167065940583949413, 5.200867483535597913, 0.000000000000000000 ) ) ;
#169817=CARTESIAN_POINT ( 'NONE',  ( -5.334207092333882017, 5.187939460669764635, 0.7998128361456281477 ) ) ;
#169819=CARTESIAN_POINT ( 'NONE',  ( -6.455090533882213322, 6.703562842383589349, -0.7216878364870338292 ) ) ;
#169841=CARTESIAN_POINT ( 'NONE',  ( -4.620296487206990932, 8.612372678375294299, 0.000000000000000000 ) ) ;
#169843=CARTESIAN_POINT ( 'NONE',  ( -5.002032328799064231, 4.800402236545811441, -0.7998128361456362523 ) ) ;
#169851=CARTESIAN_POINT ( 'NONE',  ( -6.434009798946909164, 6.877700593631734804, -0.7366733183416813713 ) ) ;
#169858=CARTESIAN_POINT ( 'NONE',  ( -4.450808633097256717, 7.987047222781189504, 2.500000000000000888 ) ) ;
#169879=CARTESIAN_POINT ( 'NONE',  ( 4.492547798081839794, 6.334668079219206049, 1.599625672291262513 ) ) ;
#169888=CARTESIAN_POINT ( 'NONE',  ( 5.365994935958575240, 9.482354201918870018, 0.7998128361456341429 ) ) ;
#169890=CARTESIAN_POINT ( 'NONE',  ( 6.852720297064418986, 6.959538199522133262, 0.7998128361456331437 ) ) ;
#169904=CARTESIAN_POINT ( 'NONE',  ( 6.119462805442048570, 6.996221746119736018, -0.9567421715909133484 ) ) ;
#169907=CARTESIAN_POINT ( 'NONE',  ( -5.221298554594238084, 8.145246509451649075, 1.082531754730549967 ) ) ;
#169908=CARTESIAN_POINT ( 'NONE',  ( 5.885648082108190238, 7.959951743916638733, 1.443375672974065660 ) ) ;
#169916=CARTESIAN_POINT ( 'NONE',  ( -3.902768115887413014, 5.646591783325653147, -1.599625672291283607 ) ) ;
#169926=CARTESIAN_POINT ( 'NONE',  ( -5.939880696118548187, 6.102484698325975288, 0.000000000000000000 ) ) ;
#169930=CARTESIAN_POINT ( 'NONE',  ( 5.559725510055676168, 8.644040974110419384, 1.199719254218451159 ) ) ;
#169960=VECTOR ( 'NONE', #47211, 1000.000000000000000 ) ;
#169969=CARTESIAN_POINT ( 'NONE',  ( -2.998506705650354487, 6.400614325406102978, -0.7302056868632772479 ) ) ;
#169986=CARTESIAN_POINT ( 'NONE',  ( 5.573810548993915148, 5.675402860013913475, 0.000000000000000000 ) ) ;
#169993=CARTESIAN_POINT ( 'NONE',  ( 5.826972158823246595, 10.02016096192762085, -0.7998128361456481317 ) ) ;
#169997=CARTESIAN_POINT ( 'NONE',  ( -3.499413046103020175, 7.096749297179887783, 0.7216878364870338292 ) ) ;
#170027=CARTESIAN_POINT ( 'NONE',  ( 5.695833931516881776, 9.659240330162777610, -0.7216878364870458196 ) ) ;
#170040=CARTESIAN_POINT ( 'NONE',  ( -4.502716413514296079, 8.267269892493059658, -0.7216878364870338292 ) ) ;
#170042=CARTESIAN_POINT ( 'NONE',  ( 5.528692779322568640, 9.672168352510192690, 0.7998128361456341429 ) ) ;
#170048=CARTESIAN_POINT ( 'NONE',  ( -4.956387674247580755, 7.940146832334256111, 1.199719254218452935 ) ) ;
#170058=CARTESIAN_POINT ( 'NONE',  ( 4.858757509019057785, 5.629766575900002401, 7.500000000000000000 ) ) ;
#170089=CARTESIAN_POINT ( 'NONE',  ( 4.584065335196271462, 5.481069324884694005, 1.082531754730549078 ) ) ;
#170093=CARTESIAN_POINT ( 'NONE',  ( -5.444481204339554736, 8.509589284108232121, 1.199719254218454489 ) ) ;
#170097=CARTESIAN_POINT ( 'NONE',  ( -5.581116510680924847, 6.540332679663050541, -1.199719254218453823 ) ) ;
#170098=CARTESIAN_POINT ( 'NONE',  ( -3.955946960137363799, 7.837298230127379917, 0.7998128361456350310 ) ) ;
#170102=CARTESIAN_POINT ( 'NONE',  ( -7.065207446052822249, 7.415365906582643163, -0.7216878364870338292 ) ) ;
#170108=CARTESIAN_POINT ( 'NONE',  ( -8.072954122294394352, 8.383144328957069291, -0.7998128361456362523 ) ) ;
#170116=CARTESIAN_POINT ( 'NONE',  ( -5.596483547390937119, 9.751257581923240991, 0.000000000000000000 ) ) ;
#170118=CARTESIAN_POINT ( 'NONE',  ( 4.797842130449009090, 8.250315290282747682, 0.8618622828703215166 ) ) ;
#170124=CARTESIAN_POINT ( 'NONE',  ( 3.250922972226694352, 7.014770244231638863, 0.7998128361456281477 ) ) ;
#170137=CARTESIAN_POINT ( 'NONE',  ( -7.075376061485238566, 9.347967719856493218, 1.599625672291269396 ) ) ;
#170147=EDGE_CURVE ( 'NONE', #203624, #85209, #125015, .T. ) ;
#170150=CARTESIAN_POINT ( 'NONE',  ( 6.505933609711257226, 8.683618192786854095, -1.599625672291281386 ) ) ;
#170161=CARTESIAN_POINT ( 'NONE',  ( 0.3029082221123034491, 2.721802924646587130, 2.050239952424178558 ) ) ;
#170162=CARTESIAN_POINT ( 'NONE',  ( 6.225987253121650689, 7.022442755726078900, -1.008712875586889712 ) ) ;
#170185=CARTESIAN_POINT ( 'NONE',  ( -5.534896847468681713, 7.440644035717915550, -1.251640694545209209 ) ) ;
#170190=CARTESIAN_POINT ( 'NONE',  ( -6.019435214058361794, 7.168094078216475040, 1.196694171119830008 ) ) ;
#170195=EDGE_LOOP ( 'NONE', ( #27972, #90581, #208703, #200502 ) ) ;
#170211=CARTESIAN_POINT ( 'NONE',  ( -4.630991987519598396, 7.560518531151607213, 1.199719254218452935 ) ) ;
#170214=FACE_OUTER_BOUND ( 'NONE', #151593, .T. ) ;
#170230=CARTESIAN_POINT ( 'NONE',  ( 5.259637247458703868, 5.100941308315409373, 0.000000000000000000 ) ) ;
#170233=CARTESIAN_POINT ( 'NONE',  ( 5.085343294144599291, 4.914812813773358435, 0.1758235994440172922 ) ) ;
#170245=CARTESIAN_POINT ( 'NONE',  ( 5.773793314573267388, 7.829454515125894964, 1.599625672291268286 ) ) ;
#170255=CARTESIAN_POINT ( 'NONE',  ( -4.655245641445871385, 6.524482229810530498, 1.599625672291263179 ) ) ;
#170256=CARTESIAN_POINT ( 'NONE',  ( 6.318982112420993502, 9.529840343536603697, -1.199719254218452047 ) ) ;
#170260=CARTESIAN_POINT ( 'NONE',  ( -5.960744811863571968, 6.983232364376142698, 1.199719254218452935 ) ) ;
#170263=CARTESIAN_POINT ( 'NONE',  ( 7.212011367826596242, 7.378711115411311638, 0.000000000000000000 ) ) ;
#170269=CARTESIAN_POINT ( 'NONE',  ( -4.586029276033976920, 8.497253585842676316, 0.07182003436798957419 ) ) ;
#170278=CARTESIAN_POINT ( 'NONE',  ( -3.797692425159308716, 7.444741906078900406, 0.000000000000000000 ) ) ;
#170287=CARTESIAN_POINT ( 'NONE',  ( 4.800995793014950941, 5.734154859006458160, -1.082531754730548412 ) ) ;
#170291=CARTESIAN_POINT ( 'NONE',  ( -4.925354943514475003, 8.968274210734028529, 0.000000000000000000 ) ) ;
#170303=CARTESIAN_POINT ( 'NONE',  ( 4.098537063712264228, 7.253343185014818673, 1.055677455976588686 ) ) ;
#170332=CARTESIAN_POINT ( 'NONE',  ( -5.641601317062248988, 6.714861303728305586, -1.082531754730549967 ) ) ;
#170357=CARTESIAN_POINT ( 'NONE',  ( -7.781453819600577582, 8.043060642480948985, 0.000000000000000000 ) ) ;
#170364=CARTESIAN_POINT ( 'NONE',  ( -5.632486471834530661, 5.535932070087196344, -0.7998128361456362523 ) ) ;
#170372=CARTESIAN_POINT ( 'NONE',  ( -3.923105346307911745, 5.670318552149568703, -1.599625672291283607 ) ) ;
#170378=CARTESIAN_POINT ( 'NONE',  ( 4.634908411025333130, 6.500755460986618495, 1.599625672291268286 ) ) ;
#170382=CARTESIAN_POINT ( 'NONE',  ( -6.611536185319534908, 7.742488966741438716, 1.199719254218452047 ) ) ;
#170385=CARTESIAN_POINT ( 'NONE',  ( -3.526002468005825286, 6.271364091718859335, -1.199719254218450271 ) ) ;
#170388=CARTESIAN_POINT ( 'NONE',  ( 6.075462232699536891, 6.260663157670513179, -0.7216878364870596974 ) ) ;
#170389=CARTESIAN_POINT ( 'NONE',  ( 3.729901657090938460, 7.365652676665848553, 0.7216878364870257245 ) ) ;
#170390=CARTESIAN_POINT ( 'NONE',  ( -4.299344108864953995, 7.069632989434141201, -1.082531754730551743 ) ) ;
#170396=CARTESIAN_POINT ( 'NONE',  ( -5.041653019435350380, 6.975290837464928728, -1.599625672291271394 ) ) ;
#170405=CARTESIAN_POINT ( 'NONE',  ( 4.030516805012513082, 7.924296382481737844, 0.000000000000000000 ) ) ;
#170409=CARTESIAN_POINT ( 'NONE',  ( -1.834547262740437557, 2.517098059729869330, -2.498887020409608084 ) ) ;
#170410=CARTESIAN_POINT ( 'NONE',  ( 5.853046489161108035, 7.294594176516559614, 1.271900669079442325 ) ) ;
#170417=ORIENTED_EDGE ( 'NONE', *, *, #106933, .T. ) ;
#170419=AXIS2_PLACEMENT_3D ( 'NONE', #35232, #11793, #208917 ) ;
#170421=CARTESIAN_POINT ( 'NONE',  ( 5.040599249230596435, 9.102725900736217568, 0.7998128361456341429 ) ) ;
#170432=CARTESIAN_POINT ( 'NONE',  ( 5.916355900263067014, 7.140870225795406867, 1.119544393390920600 ) ) ;
#170451=CARTESIAN_POINT ( 'NONE',  ( -5.281783360975562225, 8.319775133516907673, 1.199719254218452935 ) ) ;
#170456=CARTESIAN_POINT ( 'NONE',  ( -3.725947703184500970, 7.355943492750648183, 0.6041107585062406304 ) ) ;
#170464=CARTESIAN_POINT ( 'NONE',  ( 5.417364897112183719, 8.477953592343014932, 1.199719254218451159 ) ) ;
#170475=CARTESIAN_POINT ( 'NONE',  ( 3.214691819771663628, 6.764574533126651801, -0.7216878364870338292 ) ) ;
#170483=CARTESIAN_POINT ( 'NONE',  ( 0.4799999999999758349, 2.999999999999999112, 2.420000000000000373 ) ) ;
#170484=DIRECTION ( 'NONE',  ( -0.000000000000000000, -0.000000000000000000, -1.000000000000000000 ) ) ;
#170491=CARTESIAN_POINT ( 'NONE',  ( -5.641601317062233001, 9.595968946632336127, -0.7216878364870338292 ) ) ;
#170492=CARTESIAN_POINT ( 'NONE',  ( 5.397554552016204710, 9.311247720745345902, 0.7216878364870317197 ) ) ;
#170495=CIRCLE ( 'NONE', #39095, 1.250000000000000888 ) ;
#170503=CARTESIAN_POINT ( 'NONE',  ( -6.120580001926503755, 6.105374521861167914, -0.7998128361456362523 ) ) ;
#170504=CARTESIAN_POINT ( 'NONE',  ( -5.483346782084204563, 5.361935765378481378, 0.000000000000000000 ) ) ;
#170507=CARTESIAN_POINT ( 'NONE',  ( 5.031484404002867450, 8.884165881396448583, 0.7216878364870317197 ) ) ;
#170510=AXIS2_PLACEMENT_3D ( 'NONE', #174068, #109111, #108044 ) ;
#170515=CARTESIAN_POINT ( 'NONE',  ( -5.070811854594947654, 7.957075094197910481, 1.225549284076495438 ) ) ;
#170519=CARTESIAN_POINT ( 'NONE',  ( -4.844715248835366417, 8.098060037232425401, 0.8884674472836263659 ) ) ;
#170523=CARTESIAN_POINT ( 'NONE',  ( 4.800995793014950941, 5.734154859006458160, -1.082531754730548412 ) ) ;
#170527=CARTESIAN_POINT ( 'NONE',  ( -4.471156797456668386, 8.438376373666578445, -0.7998128361456362523 ) ) ;
#170538=CARTESIAN_POINT ( 'NONE',  ( 6.229045230835819069, 6.231917288922055320, -0.7998128361456481317 ) ) ;
#170577=CARTESIAN_POINT ( 'NONE',  ( 6.061904079085887354, 6.244845311787889486, 0.000000000000000000 ) ) ;
#170582=CARTESIAN_POINT ( 'NONE',  ( 6.089020385868848528, 8.197219431637373432, -1.443375672974078761 ) ) ;
#170596=CARTESIAN_POINT ( 'NONE',  ( -8.093291352714894415, 8.406871097780989288, -0.7998128361456362523 ) ) ;
#170607=CARTESIAN_POINT ( 'NONE',  ( -5.002032328799064231, 4.800402236545811441, -0.7998128361456362523 ) ) ;
#170609=CARTESIAN_POINT ( 'NONE',  ( 4.868786560638896255, 5.813244087901094481, 1.082531754730549078 ) ) ;
#170615=CARTESIAN_POINT ( 'NONE',  ( -3.332271893908731464, 7.109677319527304640, -0.7998128361456481317 ) ) ;
#170620=CARTESIAN_POINT ( 'NONE',  ( -5.316205630334251531, 9.216340645449683677, -0.7216878364870338292 ) ) ;
#170624=CARTESIAN_POINT ( 'NONE',  ( -6.912678218121246942, 9.158153569265168770, 1.599625672291269396 ) ) ;
#170629=CARTESIAN_POINT ( 'NONE',  ( -3.851398154733808088, 6.650992392901508232, -1.199719254218450271 ) ) ;
#170644=CARTESIAN_POINT ( 'NONE',  ( -4.909461021924285795, 6.821066840368686712, 1.443375672974058777 ) ) ;
#170646=CARTESIAN_POINT ( 'NONE',  ( -3.973948422136970748, 6.690004688251493192, -1.082531754730546636 ) ) ;
#170648=CARTESIAN_POINT ( 'NONE',  ( 6.398522151006641678, 6.429640362454684954, 0.000000000000000000 ) ) ;
#170649=CARTESIAN_POINT ( 'NONE',  ( -6.791708605802965870, 6.888357893050385705, -0.7998128361456362523 ) ) ;
#170650=CARTESIAN_POINT ( 'NONE',  ( -7.293360289508603600, 7.473618190706972086, 0.000000000000000000 ) ) ;
#170696=CARTESIAN_POINT ( 'NONE',  ( -1.896098101912877310, 8.993996023093842496, -0.7749999999999996891 ) ) ;
#170698=CARTESIAN_POINT ( 'NONE',  ( 5.763039058787653879, 7.049721345481424706, -2.500000000000000000 ) ) ;
#170707=CARTESIAN_POINT ( 'NONE',  ( 4.929271367020211514, 7.908511140569038922, 1.199719254218452047 ) ) ;
#170725=CARTESIAN_POINT ( 'NONE',  ( 5.228604516725597229, 6.129068686715179126, -1.199719254218450271 ) ) ;
#170732=CARTESIAN_POINT ( 'NONE',  ( -7.262327558775498737, 8.501745569106741840, 1.199719254218452047 ) ) ;
#170737=CARTESIAN_POINT ( 'NONE',  ( 5.248941747146098180, 6.152795455539095570, -1.199719254218452047 ) ) ;
#170750=CARTESIAN_POINT ( 'NONE',  ( 7.688882512725796481, 8.142986817701137525, 0.000000000000000000 ) ) ;
#170751=CARTESIAN_POINT ( 'NONE',  ( -3.472296738875691346, 6.104744391113324120, 1.082531754730549967 ) ) ;
#170752=CARTESIAN_POINT ( 'NONE',  ( -4.450819567036169211, 8.414649604842665553, -0.7998128361456362523 ) ) ;
#170763=CARTESIAN_POINT ( 'NONE',  ( 6.852720297064418986, 6.959538199522133262, 0.7998128361456331437 ) ) ;
#170764=CARTESIAN_POINT ( 'NONE',  ( 6.062430963966053632, 7.101866208495718702, -1.199719254218452047 ) ) ;
#170770=ORIENTED_EDGE ( 'NONE', *, *, #42883, .F. ) ;
#170781=CARTESIAN_POINT ( 'NONE',  ( 5.038060948978250408, 7.997685013099862239, -1.157798351953726490 ) ) ;
#170784=ORIENTED_EDGE ( 'NONE', *, *, #40036, .F. ) ;
#170791=CARTESIAN_POINT ( 'NONE',  ( 4.004454267989866700, 5.765225627445230927, 1.599625672291262513 ) ) ;
#170796=CARTESIAN_POINT ( 'NONE',  ( 2.911969131885072670, 6.619324097166378706, 0.000000000000000000 ) ) ;
#170802=CARTESIAN_POINT ( 'NONE',  ( 4.719646871332936477, 8.520355426614829142, -0.7216878364870357165 ) ) ;
#170804=CARTESIAN_POINT ( 'NONE',  ( -6.642568916052639771, 6.714361588341672515, 0.000000000000000000 ) ) ;
#170806=CARTESIAN_POINT ( 'NONE',  ( 4.228163802615382494, 6.026220084508304708, -1.599625672291269396 ) ) ;
#170814=CARTESIAN_POINT ( 'NONE',  ( 4.787437623848783907, 6.678706240755900581, -1.249999999999999334 ) ) ;
#170817=CARTESIAN_POINT ( 'NONE',  ( 6.438112759045284683, 6.782534085545247393, 0.3978009605737874432 ) ) ;
#170818=CARTESIAN_POINT ( 'NONE',  ( -7.770231434407805615, 8.237893892996801526, 0.000000000000000000 ) ) ;
#170847=VERTEX_POINT ( 'NONE', #213879 ) ;
#170853=CARTESIAN_POINT ( 'NONE',  ( 5.525830126021535449, 8.604496359403894346, -1.199719254218452047 ) ) ;
#170868=CARTESIAN_POINT ( 'NONE',  ( -5.041653019435350380, 6.975290837464928728, -1.599625672291271394 ) ) ;
#170870=CARTESIAN_POINT ( 'NONE',  ( 4.678972410047582464, 8.472901888448573615, -0.7216878364870357165 ) ) ;
#170878=CARTESIAN_POINT ( 'NONE',  ( -5.309953438407606363, 6.223975762010839574, 1.199719254218452935 ) ) ;
#170881=CARTESIAN_POINT ( 'NONE',  ( -3.363831509966360489, 6.938570838353784076, -0.7216878364870458196 ) ) ;
#170884=CARTESIAN_POINT ( 'NONE',  ( -4.496464221587651799, 5.274905009054215554, 1.199719254218452935 ) ) ;
#170889=B_SPLINE_CURVE_WITH_KNOTS ( 'NONE', 3,
 ( #124613, #28085, #159152, #94181 ),
 .UNSPECIFIED., .F., .F.,
 ( 4, 4 ),
 ( 0.003642155973307022437, 0.004387807266393894436 ),
 .UNSPECIFIED. ) ;
#170907=CARTESIAN_POINT ( 'NONE',  ( -5.550083779947821760, 7.568460058062819407, -1.599625672291271394 ) ) ;
#170917=CARTESIAN_POINT ( 'NONE',  ( -6.258858270227934284, 6.997355405945988593, -0.9884160956115575214 ) ) ;
#170937=CARTESIAN_POINT ( 'NONE',  ( 6.739811759324814133, 8.956476034002680109, -1.443375672974078761 ) ) ;
#170951=CARTESIAN_POINT ( 'NONE',  ( 3.549202351727371862, 7.362762853649070571, -0.7998128361456362523 ) ) ;
#170953=CARTESIAN_POINT ( 'NONE',  ( 4.037319642967612587, 7.289149851185872997, 0.9744337199438335428 ) ) ;
#170959=CARTESIAN_POINT ( 'NONE',  ( 5.203297092594585393, 9.292540051327542017, 0.7998128361456341429 ) ) ;
#170961=CARTESIAN_POINT ( 'NONE',  ( 4.355912491740495440, 8.303924683664389406, 0.000000000000000000 ) ) ;
#170975=CARTESIAN_POINT ( 'NONE',  ( 6.381672224870991172, 6.819330018336470012, -0.5576268912585117254 ) ) ;
#170977=CARTESIAN_POINT ( 'NONE',  ( 5.804299160426222848, 7.865044668620976509, -1.443375672974078761 ) ) ;
#170984=CARTESIAN_POINT ( 'NONE',  ( -2.972980823146582186, 6.690504403638126263, 0.000000000000000000 ) ) ;
#170992=ORIENTED_EDGE ( 'NONE', *, *, #108550, .T. ) ;
#170996=CARTESIAN_POINT ( 'NONE',  ( -4.448483798615272100, 8.203998508444197313, 0.000000000000000000 ) ) ;
#171001=CARTESIAN_POINT ( 'NONE',  ( 6.692885107001518286, 7.837396042037102717, -1.199719254218452047 ) ) ;
#171053=CARTESIAN_POINT ( 'NONE',  ( 4.855228407469603269, 7.718164671139588151, -1.082531754730548412 ) ) ;
#171056=CARTESIAN_POINT ( 'NONE',  ( 3.594320121398666856, 7.207474218358159490, -1.734723475976807094E-15 ) ) ;
#171067=CARTESIAN_POINT ( 'NONE',  ( -4.421367491832313590, 6.251624388594711590, 1.443375672974065660 ) ) ;
#171079=CARTESIAN_POINT ( 'NONE',  ( -4.326460414921602826, 8.061637894134911164, 8.322892513849239118E-08 ) ) ;
#171088=CARTESIAN_POINT ( 'NONE',  ( -4.791166081694341550, 4.882818525799564213, 0.4357780244859492669 ) ) ;
#171101=CARTESIAN_POINT ( 'NONE',  ( 7.702440666339465558, 8.158804663583751449, -0.7216878364870317197 ) ) ;
#171105=CARTESIAN_POINT ( 'NONE',  ( 5.346851039111033543, 6.199209027673978412, -2.420000000000000373 ) ) ;
#171114=CARTESIAN_POINT ( 'NONE',  ( -6.129694847154222970, 7.284303755502281597, -1.082531754730549967 ) ) ;
#171116=CARTESIAN_POINT ( 'NONE',  ( 6.200875153403774043, 8.327716660428123419, -1.599625672291283607 ) ) ;
#171121=CARTESIAN_POINT ( 'NONE',  ( -4.685224601974262271, 7.623789914682047808, -1.199719254218453823 ) ) ;
#171151=EDGE_CURVE ( 'NONE', #183115, #199688, #69542, .T. ) ;
#171162=CARTESIAN_POINT ( 'NONE',  ( 4.204437034013637664, 6.958908068774287692, -1.082531754730548412 ) ) ;
#171166=CARTESIAN_POINT ( 'NONE',  ( -6.818824913030298696, 6.919993584815607335, 0.7998128361456341429 ) ) ;
#171170=CARTESIAN_POINT ( 'NONE',  ( -6.784929528996132220, 6.880448970109080520, 0.000000000000000000 ) ) ;
#171175=CARTESIAN_POINT ( 'NONE',  ( -7.390603132780803719, 7.794994207765291172, -0.7216878364870338292 ) ) ;
#171182=CARTESIAN_POINT ( 'NONE',  ( -2.993318053567081360, 6.714231172462041819, 0.000000000000000000 ) ) ;
#171186=ORIENTED_EDGE ( 'NONE', *, *, #64855, .T. ) ;
#171189=CARTESIAN_POINT ( 'NONE',  ( -5.769876891067536206, 8.889217585290882795, 1.199719254218454489 ) ) ;
#171191=CARTESIAN_POINT ( 'NONE',  ( 5.535985025370705692, 7.434063834270491000, -1.247683609459742549 ) ) ;
#171196=CARTESIAN_POINT ( 'NONE',  ( 4.061549535745618833, 6.896169004081968090, -1.199719254218452047 ) ) ;
#171205=CARTESIAN_POINT ( 'NONE',  ( -7.533490631048818109, 8.818102486758951031, -1.199719254218452047 ) ) ;
#171208=CARTESIAN_POINT ( 'NONE',  ( -4.009193028827814587, 7.297902834095492786, -0.7581239365674132813 ) ) ;
#171217=CARTESIAN_POINT ( 'NONE',  ( 6.210516883511641772, 9.403297576475722508, 1.199719254218452047 ) ) ;
#171227=CARTESIAN_POINT ( 'NONE',  ( 4.580108180932601414, 8.499999999999996447, -0.1719113009628105149 ) ) ;
#171230=CARTESIAN_POINT ( 'NONE',  ( -0.3639057010162629613, 2.808035090322519522, 2.035120794639562636 ) ) ;
#171231=CARTESIAN_POINT ( 'NONE',  ( 6.270956187569860063, 6.991113019333711875, 0.9580997929081371822 ) ) ;
#171255=ORIENTED_EDGE ( 'NONE', *, *, #88039, .T. ) ;
#171260=CARTESIAN_POINT ( 'NONE',  ( -6.601093878019091754, 6.767222581227101408, 0.2246719935465150975 ) ) ;
#171280=CARTESIAN_POINT ( 'NONE',  ( -4.606738333593328072, 8.596554832492683929, 0.7998128361456281477 ) ) ;
#171288=( BOUNDED_CURVE ( )  B_SPLINE_CURVE ( 2, ( #186648, #171473, #38274, #73976, #119590, #106527, #140071, #206095, #88093, #155231, #187712, #123886, #8970, #157375, #104351, #20924, #136853, #87020, #6812, #170396, #189852, #91318, #172553, #72890, #153092, #4667, #173641, #202877, #75044, #120670, #185573, #37203, #71811, #54525, #103277, #203942, #39341, #208224, #177891, #175760, #181842, #12168, #198100, #11091, #110809, #210363, #95597, #77168, #176814, #128159, #28429, #160560, #78240, #26278, #190908, #59856, #132091 ),
 .UNSPECIFIED., .F., .T. ) 
 B_SPLINE_CURVE_WITH_KNOTS ( ( 3, 2, 2, 2, 2, 2, 2, 2, 2, 2, 2, 2, 2, 2, 2, 2, 2, 2, 2, 2, 2, 2, 2, 2, 2, 2, 2, 2, 3 ),
 ( 0.2844739210328576795, 0.2916666666666666852, 0.2999999999999999889, 0.3083333333333333481, 0.3166666666666666519, 0.3250000000000000111, 0.3333333333333333148, 0.3416666666666666741, 0.3499999999999999778, 0.3583333333333333370, 0.3666666666666666408, 0.3750000000000000000, 0.3833333333333333592, 0.3916666666666666630, 0.4000000000000000222, 0.4083333333333333259, 0.4166666666666666852, 0.4249999999999999889, 0.4333333333333333481, 0.4416666666666666519, 0.4500000000000000111, 0.4583333333333333148, 0.4666666666666666741, 0.4749999999999999778, 0.4833333333333333370, 0.4916666666666666408, 0.5000000000000000000, 0.5083333333333333037, 0.5119843065236711066 ),
 .UNSPECIFIED. ) 
 CURVE ( )  GEOMETRIC_REPRESENTATION_ITEM ( )  RATIONAL_B_SPLINE_CURVE ( ( 0.9683452906431710971, 0.8843625769635039546, 1.000000000000000000, 0.8660254037844387076, 1.000000000000000000, 0.8660254037844387076, 1.000000000000000000, 0.8660254037844387076, 1.000000000000000000, 0.8660254037844387076, 1.000000000000000000, 0.8660254037844387076, 1.000000000000000000, 0.8660254037844387076, 1.000000000000000000, 0.8660254037844387076, 1.000000000000000000, 0.8660254037844387076, 1.000000000000000000, 0.8660254037844387076, 1.000000000000000000, 0.8660254037844387076, 1.000000000000000000, 0.8660254037844387076, 1.000000000000000000, 0.8660254037844387076, 1.000000000000000000, 0.8660254037844387076, 1.000000000000000000, 0.8660254037844387076, 1.000000000000000000, 0.8660254037844387076, 1.000000000000000000, 0.8660254037844387076, 1.000000000000000000, 0.8660254037844387076, 1.000000000000000000, 0.8660254037844387076, 1.000000000000000000, 0.8660254037844387076, 1.000000000000000000, 0.8660254037844387076, 1.000000000000000000, 0.8660254037844387076, 1.000000000000000000, 0.8660254037844387076, 1.000000000000000000, 0.8660254037844387076, 1.000000000000000000, 0.8660254037844387076, 1.000000000000000000, 0.8660254037844387076, 1.000000000000000000, 0.8660254037844387076, 1.000000000000000000, 0.9413034809236788814, 0.9340388220506692374 ) ) 
 REPRESENTATION_ITEM ( '' )  );
#171298=CARTESIAN_POINT ( 'NONE',  ( 4.329849954717849947, 6.144853928627882489, 1.599625672291262513 ) ) ;
#171300=CARTESIAN_POINT ( 'NONE',  ( 7.661766205054107992, 8.111351125417501251, -0.7216878364870317197 ) ) ;
#171301=CARTESIAN_POINT ( 'NONE',  ( 5.094532678321557206, 4.917790403868676385, -0.1305349544365452807 ) ) ;
#171307=CARTESIAN_POINT ( 'NONE',  ( -6.329176825324663191, 6.889957431341297678, 0.7450545735031323114 ) ) ;
#171313=CARTESIAN_POINT ( 'NONE',  ( 5.825163275726873202, 6.825053905550038991, 1.199719254218452047 ) ) ;
#171323=CARTESIAN_POINT ( 'NONE',  ( -3.305155586681401303, 7.078041627762083898, 0.7998128361456352531 ) ) ;
#171325=CARTESIAN_POINT ( 'NONE',  ( 3.237364818613055473, 6.998952398349030268, -1.734723475976807094E-15 ) ) ;
#171329=CARTESIAN_POINT ( 'NONE',  ( -5.586841817283045408, 8.675676665875643678, 1.199719254218454489 ) ) ;
#171332=CARTESIAN_POINT ( 'NONE',  ( 5.176180785367283654, 9.260904359562321275, -0.7998128361456481317 ) ) ;
#171333=CARTESIAN_POINT ( 'NONE',  ( 3.913815762669449416, 7.330443837381343641, -0.8582294057540799104 ) ) ;
#171338=CARTESIAN_POINT ( 'NONE',  ( -4.688377817131518910, 8.372325690950924937, 0.6434091164432588217 ) ) ;
#171349=CARTESIAN_POINT ( 'NONE',  ( -3.621436428181653788, 7.239109909604962922, 0.7216878364870338292 ) ) ;
#171359=CARTESIAN_POINT ( 'NONE',  ( 2.943528747942701695, 6.448217615992859919, 0.000000000000000000 ) ) ;
#171363=CARTESIAN_POINT ( 'NONE',  ( -6.261886844665283114, 8.398896966899865646, 1.599625672291269396 ) ) ;
#171378=CARTESIAN_POINT ( 'NONE',  ( 4.435452530326143616, 5.203724702582467998, -1.199719254218452047 ) ) ;
#171382=CARTESIAN_POINT ( 'NONE',  ( -4.880762754383670021, 4.880089465954365657, -0.6148759978819359207 ) ) ;
#171406=CARTESIAN_POINT ( 'NONE',  ( -4.014622883422329203, 6.737458226417744278, -1.082531754730546636 ) ) ;
#171422=ORIENTED_EDGE ( 'NONE', *, *, #162356, .T. ) ;
#171432=ORIENTED_EDGE ( 'NONE', *, *, #194419, .T. ) ;
#171433=CARTESIAN_POINT ( 'NONE',  ( -7.957709816578236506, 8.248692638954882028, 0.7998128361456341429 ) ) ;
#171439=CARTESIAN_POINT ( 'NONE',  ( -5.957882158562513908, 5.915560371269843465, -0.7998128361456362523 ) ) ;
#171448=CARTESIAN_POINT ( 'NONE',  ( -3.492107083971660586, 6.231819477012331632, 1.199719254218452935 ) ) ;
#171450=CARTESIAN_POINT ( 'NONE',  ( 6.480989489388473856, 6.848452138476523565, -0.6157061703677743081 ) ) ;
#171454=CARTESIAN_POINT ( 'NONE',  ( 5.228604516725597229, 6.129068686715179126, -1.199719254218450271 ) ) ;
#171459=CARTESIAN_POINT ( 'NONE',  ( -6.394605727500880299, 7.489403432619674561, -1.199719254218452047 ) ) ;
#171463=CARTESIAN_POINT ( 'NONE',  ( -4.981695098378565945, 4.776675467721892332, -0.7998128361456362523 ) ) ;
#171468=CARTESIAN_POINT ( 'NONE',  ( 4.706088717274895750, 6.583799151611112954, 1.443375672974065660 ) ) ;
#171469=CARTESIAN_POINT ( 'NONE',  ( -4.733205024502264102, 7.575804057677677505, 1.082531754730549967 ) ) ;
#171473=CARTESIAN_POINT ( 'NONE',  ( -4.718311597035095062, 6.762783142908123324, 1.537733183400904702 ) ) ;
#171476=CARTESIAN_POINT ( 'NONE',  ( 4.577813143269636065, 5.369812084349879555, -1.199719254218450271 ) ) ;
#171487=CARTESIAN_POINT ( 'NONE',  ( 5.917965873332177829, 7.245500866451762612, 1.242176317587460943 ) ) ;
#171492=DIRECTION ( 'NONE',  ( 0.000000000000000000, -1.496258514059622730E-16, 1.000000000000000000 ) ) ;
#171496=CARTESIAN_POINT ( 'NONE',  ( 5.200434439293556643, 8.224868058221247225, -1.199719254218452047 ) ) ;
#171505=CARTESIAN_POINT ( 'NONE',  ( 5.840936731490688594, 7.196517624969346549, 1.161314407385056313 ) ) ;
#171521=CARTESIAN_POINT ( 'NONE',  ( -7.228432174741334038, 8.462200954400218578, -1.199719254218452047 ) ) ;
#171534=CARTESIAN_POINT ( 'NONE',  ( 4.929271367020211514, 7.908511140569038922, 1.199719254218452047 ) ) ;
#171542=CARTESIAN_POINT ( 'NONE',  ( 3.054329744828568227, 6.785411478933790264, 0.000000000000000000 ) ) ;
#171544=CARTESIAN_POINT ( 'NONE',  ( 3.716343503477301802, 7.349834830783237294, -1.734723475976807094E-15 ) ) ;
#171559=CARTESIAN_POINT ( 'NONE',  ( -5.614485009834902840, 9.564333254867113610, 0.7216878364870267237 ) ) ;
#171560=CARTESIAN_POINT ( 'NONE',  ( 6.549997609177859559, 6.814287763561861944, 0.000000000000000000 ) ) ;
#171570=CARTESIAN_POINT ( 'NONE',  ( -4.450819567036169211, 8.414649604842665553, -0.7998128361456362523 ) ) ;
#171571=CARTESIAN_POINT ( 'NONE',  ( -5.496904935697871863, 5.377753611261092637, 0.7998128361456281477 ) ) ;
#171574=CARTESIAN_POINT ( 'NONE',  ( 5.682275777458841048, 8.683053269460405232, 1.082531754730547524 ) ) ;
#171588=CARTESIAN_POINT ( 'NONE',  ( -4.606532530031762995, 8.380852375923623754, -0.1178885281021696541 ) ) ;
#171591=CARTESIAN_POINT ( 'NONE',  ( 5.248414862265931902, 5.295774558831261913, 0.000000000000000000 ) ) ;
#171594=CARTESIAN_POINT ( 'NONE',  ( 3.231779075379134003, 6.036511184309971689, 7.500000000000000000 ) ) ;
#171595=CARTESIAN_POINT ( 'NONE',  ( -6.200875153403786477, 8.327716660428123419, -1.599625672291271394 ) ) ;
#171606=CARTESIAN_POINT ( 'NONE',  ( -0.4000000000000001332, 2.999999999999999112, -2.420000000000000373 ) ) ;
#171609=VECTOR ( 'NONE', #32281, 1000.000000000000000 ) ;
#171610=CARTESIAN_POINT ( 'NONE',  ( 4.030516805012513082, 7.924296382481737844, 0.000000000000000000 ) ) ;
#171618=DIRECTION ( 'NONE',  ( 0.6507913734559658270, 0.7592566023652989049, 0.000000000000000000 ) ) ;
#171627=EDGE_CURVE ( 'NONE', #211313, #160372, #173503, .T. ) ;
#171645=CARTESIAN_POINT ( 'NONE',  ( 6.319508997745523438, 9.426492026461511742, -1.082531754730548412 ) ) ;
#171650=CARTESIAN_POINT ( 'NONE',  ( 5.519577934094840543, 9.453608333170423705, 0.7216878364870317197 ) ) ;
#171676=CARTESIAN_POINT ( 'NONE',  ( -4.736594563127865420, 6.619389305106191834, -1.599625672291271394 ) ) ;
#171678=CARTESIAN_POINT ( 'NONE',  ( 3.214691819771663628, 6.764574533126651801, -0.7216878364870338292 ) ) ;
#171684=CARTESIAN_POINT ( 'NONE',  ( -5.178288325776719603, 5.006034233019745372, 0.000000000000000000 ) ) ;
#171689=CARTESIAN_POINT ( 'NONE',  ( -7.770231434407805615, 8.237893892996801526, 0.000000000000000000 ) ) ;
#171691=CARTESIAN_POINT ( 'NONE',  ( -1.822139829856989079, 2.508700120398218214, 2.498486944294419754 ) ) ;
#171692=CARTESIAN_POINT ( 'NONE',  ( -6.291865805193673111, 9.498204651771386509, -1.199719254218452047 ) ) ;
#171697=CARTESIAN_POINT ( 'NONE',  ( -5.957882158562513908, 5.915560371269843465, -0.7998128361456362523 ) ) ;
#171713=CARTESIAN_POINT ( 'NONE',  ( -4.990809943606286048, 5.955604701363006015, -1.082531754730549967 ) ) ;
#171714=CARTESIAN_POINT ( 'NONE',  ( -5.275531169048922386, 5.327410250078064458, -0.7216878364870338292 ) ) ;
#171716=CARTESIAN_POINT ( 'NONE',  ( 4.213551878797002992, 8.137837301896977849, 0.000000000000000000 ) ) ;
#171717=CARTESIAN_POINT ( 'NONE',  ( -6.656127069666307072, 6.730179434224282886, 0.7998128361456341429 ) ) ;
#171718=CARTESIAN_POINT ( 'NONE',  ( -6.607619761813764647, 8.802252036906432764, 1.599625672291269396 ) ) ;
#171733=CARTESIAN_POINT ( 'NONE',  ( 3.667627899390076607, 3.521066046765033430, 2.447586748966623649 ) ) ;
#171738=CARTESIAN_POINT ( 'NONE',  ( 6.444921918449731280, 8.612437886315108315, 1.599625672291268286 ) ) ;
#171762=CARTESIAN_POINT ( 'NONE',  ( 5.318541398310776103, 9.426991741329731056, -0.7998128361456481317 ) ) ;
#171776=EDGE_LOOP ( 'NONE', ( #174668, #17800, #202134, #187152, #148926 ) ) ;
#171778=DIRECTION ( 'NONE',  ( 0.000000000000000000, -1.000000000000000000, 0.000000000000000000 ) ) ;
#171779=CARTESIAN_POINT ( 'NONE',  ( 5.037736595929563244, 8.035053907629919223, -1.199719254218452047 ) ) ;
#171793=CARTESIAN_POINT ( 'NONE',  ( 6.966220764712121927, 6.002124920821316323, 2.500000000000000444 ) ) ;
#171797=CARTESIAN_POINT ( 'NONE',  ( 4.529305835417093640, 7.441884687032027657, -1.199719254218450271 ) ) ;
#171802=ORIENTED_EDGE ( 'NONE', *, *, #101474, .F. ) ;
#171804=CARTESIAN_POINT ( 'NONE',  ( -7.208094944320834863, 8.438474185576302133, -1.199719254218452047 ) ) ;
#171809=CARTESIAN_POINT ( 'NONE',  ( 5.845500506147374153, 6.848780674373954547, 1.199719254218453823 ) ) ;
#171820=CARTESIAN_POINT ( 'NONE',  ( 7.675324359112103423, 8.127168971818530707, 0.7216878364870267237 ) ) ;
#171821=CARTESIAN_POINT ( 'NONE',  ( -3.933273961740340496, 5.682181936820735579, 1.443375672974065660 ) ) ;
#171822=CARTESIAN_POINT ( 'NONE',  ( -5.529746549527323474, 7.544733289238903851, -1.599625672291271394 ) ) ;
#171835=CARTESIAN_POINT ( 'NONE',  ( 5.554000203453580475, 6.508696987897830688, -1.199719254218452047 ) ) ;
#171836=CARTESIAN_POINT ( 'NONE',  ( 5.224688093219824303, 7.188831756880171397, -1.599625672291283607 ) ) ;
#171839=CARTESIAN_POINT ( 'NONE',  ( 6.658989722967328717, 7.797851427330578566, 1.199719254218452935 ) ) ;
#171853=CARTESIAN_POINT ( 'NONE',  ( 4.913571454530422322, 8.125067815752732514, -1.031885869761673069 ) ) ;
#171855=CARTESIAN_POINT ( 'NONE',  ( 0.3999999999999834799, 2.982849289862649744, 2.023857702508388812 ) ) ;
#171856=CARTESIAN_POINT ( 'NONE',  ( 3.549202351727371862, 7.362762853649070571, -0.7998128361456362523 ) ) ;
#171862=CARTESIAN_POINT ( 'NONE',  ( 3.790386463472274148, 6.579812086429759788, 1.199719254218452047 ) ) ;
#171867=CARTESIAN_POINT ( 'NONE',  ( 5.657495238652423097, 9.822437888394988548, 0.000000000000000000 ) ) ;
#171872=CARTESIAN_POINT ( 'NONE',  ( 7.051649292883499953, 7.399548061218447437, -0.7216878364870317197 ) ) ;
#171874=ADVANCED_FACE ( 'NONE', ( #155314 ), #131610, .T. ) ;
#171875=CARTESIAN_POINT ( 'NONE',  ( -4.606738333593328072, 8.596554832492683929, 0.7998128361456281477 ) ) ;
#171877=CARTESIAN_POINT ( 'NONE',  ( 4.848976215542928792, 5.686169002002086970, 1.199719254218452047 ) ) ;
#171884=CARTESIAN_POINT ( 'NONE',  ( -4.326776511726841967, 7.444344370598463989, -0.9316558831735276547 ) ) ;
#171888=CARTESIAN_POINT ( 'NONE',  ( -6.455090533882193782, 9.584670485287619002, -1.082531754730549967 ) ) ;
#171920=ORIENTED_EDGE ( 'NONE', *, *, #10408, .T. ) ;
#171926=CARTESIAN_POINT ( 'NONE',  ( 5.370438244344566847, 5.438135171256338829, 0.000000000000000000 ) ) ;
#171934=ADVANCED_FACE ( 'NONE', ( #204459 ), #122270, .F. ) ;
#171941=CARTESIAN_POINT ( 'NONE',  ( -6.069210040772897052, 7.109775131437022999, -1.199719254218453823 ) ) ;
#171943=CARTESIAN_POINT ( 'NONE',  ( 6.509323147892504657, 6.766834225395614411, 0.000000000000000000 ) ) ;
#171954=CARTESIAN_POINT ( 'NONE',  ( -6.283277845290492714, 6.295188672452495915, -0.7998128361456362523 ) ) ;
#171959=CARTESIAN_POINT ( 'NONE',  ( -4.665414256878304577, 5.575976400180357118, -1.082531754730549967 ) ) ;
#171962=CARTESIAN_POINT ( 'NONE',  ( -4.442231607132987925, 5.211633625523774960, -1.199719254218453823 ) ) ;
#171972=CARTESIAN_POINT ( 'NONE',  ( 3.231779075379113131, 6.036511184309971689, 2.420000000000000373 ) ) ;
#171987=CARTESIAN_POINT ( 'NONE',  ( -5.468734858265826837, 7.473552982767158070, 1.599625672291263179 ) ) ;
#171989=CARTESIAN_POINT ( 'NONE',  ( -4.625266680917477835, 5.425174544939014964, -1.199719254218453823 ) ) ;
#172001=VECTOR ( 'NONE', #205709, 1000.000000000000000 ) ;
#172013=CARTESIAN_POINT ( 'NONE',  ( -4.457598643843001973, 8.422558527783969851, 0.000000000000000000 ) ) ;
#172021=CARTESIAN_POINT ( 'NONE',  ( 7.634649897826745857, 8.079715433652276957, 0.7216878364870267237 ) ) ;
#172034=CARTESIAN_POINT ( 'NONE',  ( 5.422335090822693715, 5.290755458906732933, 0.000000000000000000 ) ) ;
#172042=CARTESIAN_POINT ( 'NONE',  ( 6.821687566331318564, 7.987665577921906568, 1.199719254218452935 ) ) ;
#172044=CARTESIAN_POINT ( 'NONE',  ( 6.099189001301251523, 8.209082816308541197, 1.599625672291268286 ) ) ;
#172057=CARTESIAN_POINT ( 'NONE',  ( 6.357275476766607980, 6.835366726881293431, -0.6123070361637416026 ) ) ;
#172059=CARTESIAN_POINT ( 'NONE',  ( 5.153507786970260796, 7.105788066255672497, -1.443375672974078761 ) ) ;
#172067=CARTESIAN_POINT ( 'NONE',  ( -3.526002468005825286, 6.271364091718859335, -1.199719254218450271 ) ) ;
#172078=CARTESIAN_POINT ( 'NONE',  ( -5.112833325684916552, 7.058334528089422300, -1.443375672974066548 ) ) ;
#172081=CARTESIAN_POINT ( 'NONE',  ( 8.005163354226054295, 8.304055099544019214, 0.000000000000000000 ) ) ;
#172082=CARTESIAN_POINT ( 'NONE',  ( -4.334696837225959776, 7.118203947705221246, -1.092094898011612747 ) ) ;
#172098=CARTESIAN_POINT ( 'NONE',  ( 3.615147460157889903, 7.348606074266929689, 0.4009180521483968196 ) ) ;
#172100=CARTESIAN_POINT ( 'NONE',  ( 5.668190738965027897, 8.770583741171307679, -1.199719254218452047 ) ) ;
#172118=EDGE_LOOP ( 'NONE', ( #181888, #24648, #211679, #189821, #99122, #83662, #50773, #60501 ) ) ;
#172137=ADVANCED_FACE ( 'NONE', ( #192489 ), #160010, .F. ) ;
#172141=CARTESIAN_POINT ( 'NONE',  ( 4.421367491832268293, 7.211993602896056288, 1.082531754730549078 ) ) ;
#172142=ORIENTED_EDGE ( 'NONE', *, *, #15512, .T. ) ;
#172146=CARTESIAN_POINT ( 'NONE',  ( -7.445362632559989535, 8.715286488521982733, 1.199719254218452047 ) ) ;
#172152=CARTESIAN_POINT ( 'NONE',  ( -5.316205630334276400, 5.374863788244313767, -0.7216878364870338292 ) ) ;
#172162=CARTESIAN_POINT ( 'NONE',  ( 0.4917504562595223505, 10.46609003534429405, -2.420000000000000373 ) ) ;
#172169=CARTESIAN_POINT ( 'NONE',  ( -3.837393226078555042, 7.491049807724315279, 0.05206913311947320572 ) ) ;
#172185=CARTESIAN_POINT ( 'NONE',  ( 5.252858170651868441, 5.093032385374103299, -0.7998128361456481317 ) ) ;
#172187=EDGE_CURVE ( 'NONE', #78339, #206450, #83466, .T. ) ;
#172198=CARTESIAN_POINT ( 'NONE',  ( -6.292392690518209264, 8.434487120394948079, -1.443375672974066548 ) ) ;
#172201=CARTESIAN_POINT ( 'NONE',  ( 7.225569521440261767, 7.394528961293920233, -0.7998128361456341429 ) ) ;
#172217=DIRECTION ( 'NONE',  ( 0.9446243521954068578, 0.000000000000000000, -0.3281536732072456997 ) ) ;
#172218=CARTESIAN_POINT ( 'NONE',  ( 4.963960565410041603, 8.060099936542098220, -1.154953748940761971 ) ) ;
#172224=AXIS2_PLACEMENT_3D ( 'NONE', #68172, #115945, #147336 ) ;
#172230=EDGE_CURVE ( 'NONE', #19248, #138713, #136092, .T. ) ;
#172249=CARTESIAN_POINT ( 'NONE',  ( 4.326460416092276162, 7.101268681199365496, -1.082531754730548412 ) ) ;
#172252=CARTESIAN_POINT ( 'NONE',  ( -5.749539660647037032, 8.865490816466966351, 1.199719254218454489 ) ) ;
#172253=CARTESIAN_POINT ( 'NONE',  ( -5.607095878192051686, 5.679663321520620478, 0.4065408311600144375 ) ) ;
#172257=CARTESIAN_POINT ( 'NONE',  ( -7.227905289416814760, 7.605180057173966723, -0.7216878364870338292 ) ) ;
#172264=CARTESIAN_POINT ( 'NONE',  ( -7.262327558775498737, 8.501745569106741840, 1.199719254218452047 ) ) ;
#172268=EDGE_LOOP ( 'NONE', ( #68441, #8145, #42949, #99671 ) ) ;
#172271=CARTESIAN_POINT ( 'NONE',  ( -7.605197822622922210, 7.837428646007010613, -0.7998128361456362523 ) ) ;
#172273=CARTESIAN_POINT ( 'NONE',  ( 4.722521264130603136, 8.336029038342307018, -0.7037175076533495055 ) ) ;
#172276=CARTESIAN_POINT ( 'NONE',  ( 4.415294977175556745, 5.022068982770194090, -0.9668805111738097979 ) ) ;
#172278=CARTESIAN_POINT ( 'NONE',  ( 3.410758162289653672, 6.136912401716668519, -1.199719254218453823 ) ) ;
#172287=CARTESIAN_POINT ( 'NONE',  ( -6.129167961829681488, 9.308390501180058507, -1.199719254218452047 ) ) ;
#172299=CARTESIAN_POINT ( 'NONE',  ( 7.614839552730775729, 8.913009562054615031, 1.199719254218452047 ) ) ;
#172313=CARTESIAN_POINT ( 'NONE',  ( 6.590809034589254267, 6.776089313701147532, -0.2235409772415736240 ) ) ;
#172314=CARTESIAN_POINT ( 'NONE',  ( -5.465345319640241506, 5.548860092434608760, 0.7216878364870257245 ) ) ;
#172317=CIRCLE ( 'NONE', #78898, 0.7500000000000006661 ) ;
#172335=DIRECTION ( 'NONE',  ( 0.000000000000000000, 0.000000000000000000, 1.000000000000000000 ) ) ;
#172339=AXIS2_PLACEMENT_3D ( 'NONE', #71927, #105550, #23178 ) ;
#172343=CARTESIAN_POINT ( 'NONE',  ( 3.393283585170187688, 7.180857625999046867, 0.7998128361456271485 ) ) ;
#172361=CARTESIAN_POINT ( 'NONE',  ( -6.629010762438975135, 6.698543742459062145, -0.7998128361456362523 ) ) ;
#172379=CARTESIAN_POINT ( 'NONE',  ( 3.576318658954677598, 7.394398545414291313, 0.7998128361456281477 ) ) ;
#172389=CARTESIAN_POINT ( 'NONE',  ( 4.694814482132247946, 8.250513237351190909, 0.6064353157786159798 ) ) ;
#172391=CARTESIAN_POINT ( 'NONE',  ( 5.701630405109389343, 7.302376724489803905, 1.216486997566777584 ) ) ;
#172408=CARTESIAN_POINT ( 'NONE',  ( -4.573896719763875574, 6.429575154514868274, -1.599625672291271394 ) ) ;
#172410=CARTESIAN_POINT ( 'NONE',  ( 6.086684617892325733, 6.065829907154645539, -0.7998128361456481317 ) ) ;
#172412=DIRECTION ( 'NONE',  ( 0.000000000000000000, 0.000000000000000000, -1.000000000000000000 ) ) ;
#172413=CARTESIAN_POINT ( 'NONE',  ( -7.286581212701773502, 7.465709267765667789, 0.7998128361456341429 ) ) ;
#172417=CARTESIAN_POINT ( 'NONE',  ( 6.496291879603339758, 7.608037276739255006, 1.199719254218452935 ) ) ;
#172422=CARTESIAN_POINT ( 'NONE',  ( -4.648357846327917819, 8.420182996469929293, -0.5132882116619559287 ) ) ;
#172432=CARTESIAN_POINT ( 'NONE',  ( -5.600926855776894975, 6.667407765562058053, -1.082531754730549967 ) ) ;
#172442=CARTESIAN_POINT ( 'NONE',  ( 5.736508392357904107, 5.865217010605237924, 0.000000000000000000 ) ) ;
#172446=CARTESIAN_POINT ( 'NONE',  ( -6.831329296439251131, 9.063246493969506545, -1.599625672291271394 ) ) ;
#172448=VERTEX_POINT ( 'NONE', #114526 ) ;
#172460=CARTESIAN_POINT ( 'NONE',  ( 3.573456005653643519, 6.326726552307992080, -1.199719254218453823 ) ) ;
#172465=CARTESIAN_POINT ( 'NONE',  ( 4.376249722160992839, 8.327651452488305850, 0.000000000000000000 ) ) ;
#172489=CARTESIAN_POINT ( 'NONE',  ( -5.966997003790232235, 7.094489604910957148, -1.082531754730549967 ) ) ;
#172503=ORIENTED_EDGE ( 'NONE', *, *, #76698, .F. ) ;
#172514=CARTESIAN_POINT ( 'NONE',  ( -5.745623237141265882, 9.925253886631958622, 0.7998128361456291469 ) ) ;
#172520=CARTESIAN_POINT ( 'NONE',  ( -3.298376509874564988, 7.070132704820777825, 0.000000000000000000 ) ) ;
#172524=CARTESIAN_POINT ( 'NONE',  ( 6.373741612200174878, 6.608655767087928012, 0.7216878364870328300 ) ) ;
#172529=CARTESIAN_POINT ( 'NONE',  ( -5.340986169140711226, 5.195848383611072485, 0.000000000000000000 ) ) ;
#172531=CARTESIAN_POINT ( 'NONE',  ( 5.713240515264599750, 7.403118591225121392, -1.316831503761767719 ) ) ;
#172535=CARTESIAN_POINT ( 'NONE',  ( 6.215487077222150880, 6.216099443039444949, 0.000000000000000000 ) ) ;
#172540=CARTESIAN_POINT ( 'NONE',  ( -5.586841817283045408, 8.675676665875643678, 1.199719254218454489 ) ) ;
#172543=CARTESIAN_POINT ( 'NONE',  ( -5.659602779061863487, 5.567567761852417085, 0.7998128361456281477 ) ) ;
#172548=CARTESIAN_POINT ( 'NONE',  ( 5.438229012412886476, 7.437962829272074750, -1.443375672974078761 ) ) ;
#172549=CARTESIAN_POINT ( 'NONE',  ( -6.102578539482539810, 6.292298848917299736, 0.000000000000000000 ) ) ;
#172553=CARTESIAN_POINT ( 'NONE',  ( -6.134138155540168391, 6.121192367743780949, 0.000000000000000000 ) ) ;
#172556=CARTESIAN_POINT ( 'NONE',  ( 4.740510986633625024, 5.559626234941203116, -1.199719254218450271 ) ) ;
#172567=CARTESIAN_POINT ( 'NONE',  ( 4.783863686166085039, 8.265937597628173705, 0.8363946479656783062 ) ) ;
#172573=DIRECTION ( 'NONE',  ( 0.000000000000000000, -1.000000000000000000, -1.496258514059622730E-16 ) ) ;
#172578=CARTESIAN_POINT ( 'NONE',  ( 4.688087255275310561, 8.691461907788344377, -0.7998128361456381397 ) ) ;
#172590=CARTESIAN_POINT ( 'NONE',  ( 6.361499291607088935, 6.832587723092125032, 0.6030276918116053153 ) ) ;
#172609=CARTESIAN_POINT ( 'NONE',  ( -5.596483547390937119, 9.751257581923240991, 0.000000000000000000 ) ) ;
#172622=CARTESIAN_POINT ( 'NONE',  ( 5.338878628731272613, 9.450718510153643948, -0.7998128361456481317 ) ) ;
#172630=ORIENTED_EDGE ( 'NONE', *, *, #121643, .F. ) ;
#172631=CARTESIAN_POINT ( 'NONE',  ( 5.388439706788500594, 5.251210844200210559, 0.7998128361456352531 ) ) ;
#172635=CARTESIAN_POINT ( 'NONE',  ( 4.543390873910913896, 5.433615786718446472, 1.082531754730549078 ) ) ;
#172636=CARTESIAN_POINT ( 'NONE',  ( 5.608194732729899101, 5.660561533053829031, 0.1769238548265182898 ) ) ;
#172641=AXIS2_PLACEMENT_3D ( 'NONE', #73001, #188897, #158547 ) ;
#172650=CARTESIAN_POINT ( 'NONE',  ( -5.628043163448566588, 9.580151100749725757, 0.000000000000000000 ) ) ;
#172651=CARTESIAN_POINT ( 'NONE',  ( 2.905190055078214595, 6.611415174225076186, 0.7998128361456271485 ) ) ;
#172662=CARTESIAN_POINT ( 'NONE',  ( -4.827585214917754719, 7.789877296449459365, -1.199719254218453823 ) ) ;
#172663=CARTESIAN_POINT ( 'NONE',  ( -5.808742468812186033, 5.741564066561132940, 0.000000000000000000 ) ) ;
#172664=CARTESIAN_POINT ( 'NONE',  ( 5.844973620822830895, 8.872867420051733234, 1.082531754730549967 ) ) ;
#172675=CARTESIAN_POINT ( 'NONE',  ( -4.879429750001362365, 8.060225557361109239, -0.9362273787268098335 ) ) ;
#172679=CARTESIAN_POINT ( 'NONE',  ( 4.041739190649647817, 6.769093918182960579, -1.082531754730548412 ) ) ;
#172684=CARTESIAN_POINT ( 'NONE',  ( -5.271087860662956537, 9.371629280740593870, 0.000000000000000000 ) ) ;
#172696=CARTESIAN_POINT ( 'NONE',  ( 5.391302360089590628, 6.318882837306503575, -1.199719254218452047 ) ) ;
#172735=CARTESIAN_POINT ( 'NONE',  ( 7.214347136247488912, 7.589362211809770997, -0.7216878364870317197 ) ) ;
#172740=CARTESIAN_POINT ( 'NONE',  ( 6.156811153937166381, 10.19704708965311468, 0.000000000000000000 ) ) ;
#172767=CARTESIAN_POINT ( 'NONE',  ( -3.654804927335652209, 6.421633627603656080, 1.199719254218452935 ) ) ;
#172774=CARTESIAN_POINT ( 'NONE',  ( -3.481411583659053566, 7.283673624236017830, 0.000000000000000000 ) ) ;
#172779=CARTESIAN_POINT ( 'NONE',  ( -6.129694847154211423, 9.205042184104968328, -1.082531754730549967 ) ) ;
#172783=CARTESIAN_POINT ( 'NONE',  ( -7.075376061485238566, 9.347967719856493218, 1.599625672291269396 ) ) ;
#172788=CARTESIAN_POINT ( 'NONE',  ( -3.447516199624892419, 7.244129009529488350, 0.7998128361456352531 ) ) ;
#172801=CARTESIAN_POINT ( 'NONE',  ( -6.129694847154231852, 6.323934541200937787, -0.7216878364870338292 ) ) ;
#172803=CARTESIAN_POINT ( 'NONE',  ( -5.112833325684908559, 8.018703742390766109, -1.082531754730549967 ) ) ;
#172804=CARTESIAN_POINT ( 'NONE',  ( 6.875920180786008196, 8.050936961452347163, -1.199719254218452047 ) ) ;
#172805=CARTESIAN_POINT ( 'NONE',  ( -5.981082042284069367, 7.006959133200059142, 1.199719254218452935 ) ) ;
#172820=CARTESIAN_POINT ( 'NONE',  ( 2.795860172527830922, 2.967839529530313936, 2.452799336324935631 ) ) ;
#172859=CARTESIAN_POINT ( 'NONE',  ( 5.558836782162523527, 7.518240855878357110, -1.384758111419038817 ) ) ;
#172866=CARTESIAN_POINT ( 'NONE',  ( 4.389807875774629942, 8.343469298370917997, 0.7998128361456271485 ) ) ;
#172869=DIRECTION ( 'NONE',  ( 1.000000000000000000, 0.000000000000000000, 0.000000000000000000 ) ) ;
#172882=CARTESIAN_POINT ( 'NONE',  ( 3.867818961648523235, 7.734482231890414283, 1.040834085586084257E-14 ) ) ;
#172889=CARTESIAN_POINT ( 'NONE',  ( -6.454563648557663846, 9.688018802362710957, -1.199719254218452047 ) ) ;
#172894=CARTESIAN_POINT ( 'NONE',  ( 4.389807875774629942, 8.343469298370917997, 0.7998128361456271485 ) ) ;
#172895=VERTEX_POINT ( 'NONE', #2467 ) ;
#172905=CARTESIAN_POINT ( 'NONE',  ( 5.397554552016204710, 9.311247720745345902, 0.7216878364870317197 ) ) ;
#172907=CARTESIAN_POINT ( 'NONE',  ( -3.350273356352693188, 6.922752992471175482, 0.000000000000000000 ) ) ;
#172908=CARTESIAN_POINT ( 'NONE',  ( -6.123442655227560927, 7.173046514967467147, 1.199719254218452047 ) ) ;
#172919=CARTESIAN_POINT ( 'NONE',  ( 7.205232291019763480, 7.370802192470005565, -0.7998128361456341429 ) ) ;
#172920=CARTESIAN_POINT ( 'NONE',  ( 4.746236293235721604, 7.694970221153795364, 1.199719254218451159 ) ) ;
#172921=CARTESIAN_POINT ( 'NONE',  ( 4.929271367020211514, 7.908511140569038922, 1.199719254218452047 ) ) ;
#172924=CARTESIAN_POINT ( 'NONE',  ( 7.876360894896227371, 8.153785563659219804, -0.7998128361456341429 ) ) ;
#172933=ADVANCED_FACE ( 'NONE', ( #132547 ), #30178, .T. ) ;
#172941=ORIENTED_EDGE ( 'NONE', *, *, #185371, .F. ) ;
#172943=CARTESIAN_POINT ( 'NONE',  ( 4.573896719763862251, 6.429575154514868274, -1.599625672291273171 ) ) ;
#172947=CARTESIAN_POINT ( 'NONE',  ( 5.246079093845007257, 5.085123462432798114, 0.7998128361456352531 ) ) ;
#172953=CARTESIAN_POINT ( 'NONE',  ( 5.833751235630055376, 10.02806988486892514, 0.7998128361456331437 ) ) ;
#172957=CARTESIAN_POINT ( 'NONE',  ( 5.560252395380206991, 7.580323442733986283, 1.443375672974065660 ) ) ;
#172959=CARTESIAN_POINT ( 'NONE',  ( -6.140917232347002042, 6.129101290685087911, -0.7998128361456362523 ) ) ;
#172961=CARTESIAN_POINT ( 'NONE',  ( 3.854260808034858155, 7.718664386007802136, -0.7998128361456362523 ) ) ;
#172968=CARTESIAN_POINT ( 'NONE',  ( -4.647415939163805909, 7.189517123537264354, -1.183184842545903948 ) ) ;
#172971=CARTESIAN_POINT ( 'NONE',  ( -3.984117037569407938, 5.741498858621315371, 1.599625672291270506 ) ) ;
#172982=CARTESIAN_POINT ( 'NONE',  ( -0.1216878429548682999, 3.463015919485879834, -1.996294584693599994 ) ) ;
#173001=CARTESIAN_POINT ( 'NONE',  ( 4.475600106286968582, 5.354526557823810151, -1.082531754730548412 ) ) ;
#173006=CARTESIAN_POINT ( 'NONE',  ( 6.373214726875630731, 9.593111727067046957, 1.199719254218452047 ) ) ;
#173008=CARTESIAN_POINT ( 'NONE',  ( 4.882344714252594642, 4.868692719482363707, 0.000000000000000000 ) ) ;
#173020=CARTESIAN_POINT ( 'NONE',  ( -4.437261413422502798, 8.398831758960053406, 0.000000000000000000 ) ) ;
#173022=CARTESIAN_POINT ( 'NONE',  ( 7.661766205054107992, 8.111351125417501251, -0.7216878364870317197 ) ) ;
#173031=CARTESIAN_POINT ( 'NONE',  ( -4.553559489343377287, 6.405848385690952718, -1.599625672291271394 ) ) ;
#173036=CARTESIAN_POINT ( 'NONE',  ( -4.855228407469635243, 4.837057028235559386, 0.7216878364870257245 ) ) ;
#173040=CARTESIAN_POINT ( 'NONE',  ( -4.604929450496978660, 5.401447776115099408, -1.199719254218453823 ) ) ;
#173064=CARTESIAN_POINT ( 'NONE',  ( -6.607619761813764647, 8.802252036906432764, 1.599625672291269396 ) ) ;
#173065=CARTESIAN_POINT ( 'NONE',  ( -4.318600669050631780, 4.999583595936801572, -2.420000000000000373 ) ) ;
#173076=CARTESIAN_POINT ( 'NONE',  ( -6.218052724642120666, 7.025831364812846758, -1.032658732443512584 ) ) ;
#173091=CARTESIAN_POINT ( 'NONE',  ( -6.954406449166956605, 7.078172043641714595, -0.7998128361456362523 ) ) ;
#173092=CARTESIAN_POINT ( 'NONE',  ( 2.728371075039198512, 2.952267909019295367, 2.500000000000000000 ) ) ;
#173093=VERTEX_POINT ( 'NONE', #108608 ) ;
#173099=CARTESIAN_POINT ( 'NONE',  ( 7.526184668917440312, 8.913541880892736913, -1.082531754730548412 ) ) ;
#173108=CARTESIAN_POINT ( 'NONE',  ( -4.515041659042474897, 7.522260248201400934, 0.9990323037335177014 ) ) ;
#173112=CARTESIAN_POINT ( 'NONE',  ( 4.411198876399872404, 6.239761003923544713, -1.599625672291273171 ) ) ;
#173120=CARTESIAN_POINT ( 'NONE',  ( 7.537407054554579489, 7.758339416593960536, 0.000000000000000000 ) ) ;
#173122=CARTESIAN_POINT ( 'NONE',  ( 5.692444392891300886, 7.734547439830227411, -1.599625672291281386 ) ) ;
#173126=CARTESIAN_POINT ( 'NONE',  ( -2.296876792725286887, 2.697690400687393630, -2.500000000000000000 ) ) ;
#173135=CARTESIAN_POINT ( 'NONE',  ( 6.080034374691865473, 7.023743017405461586, -0.9950221519831742301 ) ) ;
#173137=CARTESIAN_POINT ( 'NONE',  ( 5.316205630334249754, 7.295602216847000498, -1.443375672974078761 ) ) ;
#173145=CARTESIAN_POINT ( 'NONE',  ( -3.284818356260900796, 7.054314858938165678, 0.7998128361456352531 ) ) ;
#173157=CARTESIAN_POINT ( 'NONE',  ( -4.570507181138272479, 7.385989907086349504, 1.082531754730549967 ) ) ;
#173161=CARTESIAN_POINT ( 'NONE',  ( 6.668631453075247073, 8.873432343378178544, -1.599625672291281386 ) ) ;
#173162=CARTESIAN_POINT ( 'NONE',  ( 4.879147978569815969, 4.879180288469956217, -0.1512534140984626019 ) ) ;
#173164=B_SPLINE_CURVE_WITH_KNOTS ( 'NONE', 1,
 ( #114133, #115184 ),
 .UNSPECIFIED., .F., .F.,
 ( 2, 2 ),
 ( 0.07258517961950859687, 1.000000000000000000 ),
 .UNSPECIFIED. ) ;
#173168=EDGE_CURVE ( 'NONE', #207594, #149695, #208158, .T. ) ;
#173178=CARTESIAN_POINT ( 'NONE',  ( 5.332099551924443404, 9.442809587212341427, 0.000000000000000000 ) ) ;
#173198=CARTESIAN_POINT ( 'NONE',  ( -7.286581212701773502, 7.465709267765667789, 0.7998128361456341429 ) ) ;
#173202=CARTESIAN_POINT ( 'NONE',  ( -6.497544600628390121, 6.760421010857692536, 0.1165534177344582784 ) ) ;
#173219=CARTESIAN_POINT ( 'NONE',  ( 6.549997609177859559, 6.814287763561861944, 0.000000000000000000 ) ) ;
#173229=CARTESIAN_POINT ( 'NONE',  ( -5.478903473698268023, 5.564677938835638216, -0.7216878364870338292 ) ) ;
#173238=( BOUNDED_CURVE ( )  B_SPLINE_CURVE ( 2, ( #10056, #126031, #77191 ),
 .UNSPECIFIED., .F., .T. ) 
 B_SPLINE_CURVE_WITH_KNOTS ( ( 3, 3 ),
 ( 0.000000000000000000, 0.004781798612014134114 ),
 .UNSPECIFIED. ) 
 CURVE ( )  GEOMETRIC_REPRESENTATION_ITEM ( )  RATIONAL_B_SPLINE_CURVE ( ( 1.000000000000000000, 0.9231232554125530232, 0.9344726973605665954 ) ) 
 REPRESENTATION_ITEM ( '' )  );
#173262=CARTESIAN_POINT ( 'NONE',  ( 4.258142763143749399, 7.125527769379820242, 1.199719254218451159 ) ) ;
#173273=CARTESIAN_POINT ( 'NONE',  ( -7.105881907338169157, 8.423188659050232729, -1.082531754730549967 ) ) ;
#173275=CARTESIAN_POINT ( 'NONE',  ( 8.174640274396848483, 8.501778173076651512, 0.7998128361456291469 ) ) ;
#173289=CARTESIAN_POINT ( 'NONE',  ( 5.090160327287878594, 4.903218234782778850, -0.7998128361456481317 ) ) ;
#173291=CARTESIAN_POINT ( 'NONE',  ( -5.329763783947941036, 5.390681634126922361, 0.000000000000000000 ) ) ;
#173293=CARTESIAN_POINT ( 'NONE',  ( 6.170369307550812366, 6.371388078330368465, 0.7216878364870467077 ) ) ;
#173321=EDGE_CURVE ( 'NONE', #26714, #198442, #28528, .T. ) ;
#173325=CARTESIAN_POINT ( 'NONE',  ( -7.957709816578236506, 8.248692638954882028, 0.7998128361456341429 ) ) ;
#173328=CARTESIAN_POINT ( 'NONE',  ( -4.911796789900812144, 8.952456364851418158, 0.7998128361456291469 ) ) ;
#173329=CARTESIAN_POINT ( 'NONE',  ( -5.306037014901836990, 7.283738832175834510, 1.599625672291263401 ) ) ;
#173331=EDGE_LOOP ( 'NONE', ( #102369, #59673, #212378 ) ) ;
#173333=CARTESIAN_POINT ( 'NONE',  ( -6.197485614778184271, 9.284131412999601096, 1.082531754730549967 ) ) ;
#173336=CARTESIAN_POINT ( 'NONE',  ( -3.318713740295064163, 7.093859473644694269, 0.000000000000000000 ) ) ;
#173339=CARTESIAN_POINT ( 'NONE',  ( -4.462568837553487100, 5.235360394347691404, -1.199719254218453823 ) ) ;
#173347=CARTESIAN_POINT ( 'NONE',  ( -6.420668264523499147, 9.648474187656182366, 1.199719254218452935 ) ) ;
#173349=CARTESIAN_POINT ( 'NONE',  ( 5.551963943121584144, 7.421064284658021037, -1.246246109899084020 ) ) ;
#173350=B_SPLINE_CURVE_WITH_KNOTS ( 'NONE', 3,
 ( #133694, #103290, #201821, #136866, #104364, #154179 ),
 .UNSPECIFIED., .F., .F.,
 ( 4, 2, 4 ),
 ( 0.001369432773569654585, 0.001631688116371318026, 0.001893943459172981250 ),
 .UNSPECIFIED. ) ;
#173354=CARTESIAN_POINT ( 'NONE',  ( 7.614839552730775729, 8.913009562054615031, 1.199719254218452047 ) ) ;
#173376=CARTESIAN_POINT ( 'NONE',  ( 2.898410978271408922, 6.603506251283770112, -0.7998128361456362523 ) ) ;
#173392=CARTESIAN_POINT ( 'NONE',  ( 6.606300428615679898, 6.765996464729716386, -0.04887194053871009303 ) ) ;
#173393=CARTESIAN_POINT ( 'NONE',  ( -4.950135482320929370, 5.908151163196758482, -1.082531754730549967 ) ) ;
#173423=CARTESIAN_POINT ( 'NONE',  ( 4.309512724297349884, 6.121127159803966933, 1.599625672291261402 ) ) ;
#173426=EDGE_CURVE ( 'NONE', #38781, #96770, #11106, .T. ) ;
#173439=EDGE_CURVE ( 'NONE', #75117, #211313, #11021, .T. ) ;
#173444=CARTESIAN_POINT ( 'NONE',  ( -7.130662446144611977, 7.283804040115648526, 0.000000000000000000 ) ) ;
#173460=CARTESIAN_POINT ( 'NONE',  ( 5.435893244436359240, 5.306573304789342416, -0.7998128361456481317 ) ) ;
#173471=CARTESIAN_POINT ( 'NONE',  ( -6.486624235763164492, 6.835203243035253173, 0.7121179707554707861 ) ) ;
#173475=CARTESIAN_POINT ( 'NONE',  ( 5.779562687394081522, 7.242644825714458001, 1.188994900607452054 ) ) ;
#173476=CARTESIAN_POINT ( 'NONE',  ( 5.375100870188143531, 7.683496445330359137, 1.324677879948222392 ) ) ;
#173490=ORIENTED_EDGE ( 'NONE', *, *, #48405, .T. ) ;
#173495=CARTESIAN_POINT ( 'NONE',  ( -4.522526758610270647, 7.433975764090723359, -1.199719254218453823 ) ) ;
#173497=CARTESIAN_POINT ( 'NONE',  ( 3.386504508363381571, 7.172948703057747011, -0.7998128361456362523 ) ) ;
#173500=CARTESIAN_POINT ( 'NONE',  ( -5.906512197408906317, 6.919960980845699439, -1.199719254218453823 ) ) ;
#173503=CIRCLE ( 'NONE', #204518, 0.8300000000000008482 ) ;
#173504=CARTESIAN_POINT ( 'NONE',  ( 5.363132282657546490, 8.414682208812571673, -1.199719254218452047 ) ) ;
#173509=CARTESIAN_POINT ( 'NONE',  ( -5.281148723220589147, 7.765029056575591504, -1.308346332658766986 ) ) ;
#173518=CARTESIAN_POINT ( 'NONE',  ( -4.136646265500964148, 6.879818838842817641, -1.082531754730551743 ) ) ;
#173521=CARTESIAN_POINT ( 'NONE',  ( 2.969872605471105764, 6.605953636083951253, 0.1972538285620730192 ) ) ;
#173528=CARTESIAN_POINT ( 'NONE',  ( 5.560252395380215873, 6.619954228432645138, 1.082531754730549078 ) ) ;
#173531=CARTESIAN_POINT ( 'NONE',  ( 5.045036709957831711, 4.903268083610561767, 0.3063280728123271568 ) ) ;
#173532=CARTESIAN_POINT ( 'NONE',  ( -7.435720902452096936, 7.639705572474380091, 0.000000000000000000 ) ) ;
#173546=CARTESIAN_POINT ( 'NONE',  ( 3.074666975249065626, 6.809138247757705820, 0.000000000000000000 ) ) ;
#173578=CARTESIAN_POINT ( 'NONE',  ( -5.316205630334255972, 8.255971431148344308, -1.082531754730549967 ) ) ;
#173603=CARTESIAN_POINT ( 'NONE',  ( -7.944151662964566540, 8.232874793072271657, 0.000000000000000000 ) ) ;
#173609=CARTESIAN_POINT ( 'NONE',  ( -4.390861645979385663, 6.216034235099629157, -1.599625672291271394 ) ) ;
#173617=CARTESIAN_POINT ( 'NONE',  ( -6.912678218121246942, 9.158153569265168770, 1.599625672291269396 ) ) ;
#173619=CARTESIAN_POINT ( 'NONE',  ( 5.911136963822321455, 7.250628055112136039, -1.245581879728396846 ) ) ;
#173623=CARTESIAN_POINT ( 'NONE',  ( 4.041212305325117882, 6.872442235258051646, -1.199719254218448494 ) ) ;
#173628=CARTESIAN_POINT ( 'NONE',  ( -5.589704470584107909, 9.743348658981940247, -0.7998128361456362523 ) ) ;
#173630=VERTEX_POINT ( 'NONE', #180822 ) ;
#173632=CARTESIAN_POINT ( 'NONE',  ( -2.986538976760251263, 6.706322249520737522, -0.7998128361456481317 ) ) ;
#173637=CARTESIAN_POINT ( 'NONE',  ( 6.333067150914820864, 6.561202228921677815, 0.7216878364870328300 ) ) ;
#173638=CARTESIAN_POINT ( 'NONE',  ( -4.462041952228942954, 8.219816354326809460, -0.7216878364870338292 ) ) ;
#173641=CARTESIAN_POINT ( 'NONE',  ( -4.610654757099099221, 7.536791762327691657, 1.199719254218452935 ) ) ;
#173644=CARTESIAN_POINT ( 'NONE',  ( 3.715816618597135523, 6.492813934075403637, -1.199719254218453823 ) ) ;
#173655=CARTESIAN_POINT ( 'NONE',  ( 4.749341595749815070, 8.305088035112140332, 0.7662636247844747395 ) ) ;
#173665=CARTESIAN_POINT ( 'NONE',  ( 6.713222337422018349, 7.861122810861019161, -1.199719254218452047 ) ) ;
#173675=CARTESIAN_POINT ( 'NONE',  ( 4.651083699394226834, 8.303454393088664176, 0.4639335724816190942 ) ) ;
#173682=CARTESIAN_POINT ( 'NONE',  ( 7.679767667498067496, 7.924426798361372093, 0.000000000000000000 ) ) ;
#173686=CARTESIAN_POINT ( 'NONE',  ( -4.634775730458505549, 8.344889633747440527, 0.3497604727749434872 ) ) ;
#173693=CARTESIAN_POINT ( 'NONE',  ( -7.632314129850253259, 7.869064337772231355, 0.7998128361456341429 ) ) ;
#173697=CARTESIAN_POINT ( 'NONE',  ( -3.741063380996889620, 7.355675534244899616, 0.6276085112526242904 ) ) ;
#173707=CARTESIAN_POINT ( 'NONE',  ( 7.876360894896227371, 8.153785563659219804, -0.7998128361456341429 ) ) ;
#173714=CARTESIAN_POINT ( 'NONE',  ( -6.075462232255183892, 10.10214001435745246, 0.000000000000000000 ) ) ;
#173716=CARTESIAN_POINT ( 'NONE',  ( 2.891631901464575272, 6.595597328342462262, 0.000000000000000000 ) ) ;
#173718=CARTESIAN_POINT ( 'NONE',  ( 4.462041952228939401, 6.299077925724123617, -1.443375672974068769 ) ) ;
#173720=ORIENTED_EDGE ( 'NONE', *, *, #101206, .F. ) ;
#173726=ADVANCED_FACE ( 'NONE', ( #978 ), #133181, .T. ) ;
#173731=CARTESIAN_POINT ( 'NONE',  ( -6.943184063974175757, 9.193743722760251202, -1.443375672974066548 ) ) ;
#173732=CARTESIAN_POINT ( 'NONE',  ( 4.927462483923885195, 4.713404084191450849, -0.7998128361456481317 ) ) ;
#173745=CARTESIAN_POINT ( 'NONE',  ( -6.283277845290492714, 6.295188672452495915, -0.7998128361456362523 ) ) ;
#173746=CARTESIAN_POINT ( 'NONE',  ( -5.795184315198522285, 5.725746220678519904, -0.7998128361456362523 ) ) ;
#173748=CARTESIAN_POINT ( 'NONE',  ( 6.278834536460164983, 9.379038488295265097, -1.082531754730548412 ) ) ;
#173750=ORIENTED_EDGE ( 'NONE', *, *, #183912, .T. ) ;
#173752=TOROIDAL_SURFACE ( 'NONE', #187481, 0.8300000000000010703, 0.08000000000000000167 ) ;
#173759=CARTESIAN_POINT ( 'NONE',  ( -6.202194133424988820, 6.954874670134298498, -0.8734430727420500196 ) ) ;
#173764=CARTESIAN_POINT ( 'NONE',  ( 5.424670859243587273, 5.501406555305196733, -0.7216878364870458196 ) ) ;
#173769=CARTESIAN_POINT ( 'NONE',  ( -5.824109505522200081, 8.952488968821326054, -1.199719254218452047 ) ) ;
#173784=CARTESIAN_POINT ( 'NONE',  ( 5.825163275726873202, 6.825053905550038991, 1.199719254218452047 ) ) ;
#173819=CARTESIAN_POINT ( 'NONE',  ( 6.617788377246179188, 8.814115421577600529, -1.443375672974078761 ) ) ;
#173824=CARTESIAN_POINT ( 'NONE',  ( 5.506019780481205217, 9.437790487287811558, 0.000000000000000000 ) ) ;
#173844=SHAPE_DEFINITION_REPRESENTATION ( #57414, #11178 ) ;
#173847=CARTESIAN_POINT ( 'NONE',  ( -3.318713740295064163, 7.093859473644694269, 0.000000000000000000 ) ) ;
#173849=CARTESIAN_POINT ( 'NONE',  ( 5.139949632912227173, 8.050339434155988627, -1.082531754730548412 ) ) ;
#173855=CARTESIAN_POINT ( 'NONE',  ( -5.503684012504701961, 5.385662534202396934, 0.000000000000000000 ) ) ;
#173860=CARTESIAN_POINT ( 'NONE',  ( -6.780486220610184134, 9.003929572168926754, -1.443375672974066548 ) ) ;
#173862=CIRCLE ( 'NONE', #135806, 2.080000000000000071 ) ;
#173863=CARTESIAN_POINT ( 'NONE',  ( -7.015401035077363900, 6.062865449010541141, 2.437084766375292144 ) ) ;
#173869=CARTESIAN_POINT ( 'NONE',  ( -5.795184315198522285, 5.725746220678519904, -0.7998128361456362523 ) ) ;
#173879=CARTESIAN_POINT ( 'NONE',  ( -3.984117037569407938, 5.741498858621315371, 1.599625672291270506 ) ) ;
#173882=CARTESIAN_POINT ( 'NONE',  ( -5.045042558060949034, 6.018876084893449274, 1.082531754730549078 ) ) ;
#173884=CARTESIAN_POINT ( 'NONE',  ( -4.773879485343255347, 8.583626809626847987, 0.000000000000000000 ) ) ;
#173886=CARTESIAN_POINT ( 'NONE',  ( 7.062871678076271920, 7.204714810702593120, -0.7998128361456341429 ) ) ;
#173887=CARTESIAN_POINT ( 'NONE',  ( -5.794130544993808307, 7.853181283949808744, 1.599625672291263179 ) ) ;
#173895=ORIENTED_EDGE ( 'NONE', *, *, #160720, .T. ) ;
#173900=ORIENTED_EDGE ( 'NONE', *, *, #188786, .T. ) ;
#173908=B_SPLINE_CURVE_WITH_KNOTS ( 'NONE', 3,
 ( #131387, #33819, #18627, #150793 ),
 .UNSPECIFIED., .F., .F.,
 ( 4, 4 ),
 ( 0.003007768841253834029, 0.003753604288505242494 ),
 .UNSPECIFIED. ) ;
#173909=CARTESIAN_POINT ( 'NONE',  ( 6.339319342841494453, 9.553567112360518365, -1.199719254218452047 ) ) ;
#173946=CARTESIAN_POINT ( 'NONE',  ( 4.064412189046650248, 7.963840997188264659, 0.7998128361456271485 ) ) ;
#173947=DIRECTION ( 'NONE',  ( 0.000000000000000000, 0.000000000000000000, -1.000000000000000000 ) ) ;
#173951=CARTESIAN_POINT ( 'NONE',  ( -6.577113915960841162, 7.806292669110006521, -1.082531754730549967 ) ) ;
#173963=CARTESIAN_POINT ( 'NONE',  ( 4.706615602599436343, 5.520081620234675412, 1.199719254218452935 ) ) ;
#173964=CARTESIAN_POINT ( 'NONE',  ( 7.191674137406095291, 7.354984346587396082, 0.000000000000000000 ) ) ;
#173967=DIRECTION ( 'NONE',  ( 0.000000000000000000, 0.000000000000000000, -1.000000000000000000 ) ) ;
#173975=CARTESIAN_POINT ( 'NONE',  ( 4.115782150200256950, 6.959440387612411349, 1.199719254218452047 ) ) ;
#173987=CARTESIAN_POINT ( 'NONE',  ( 5.858531774880875176, 9.849054480754103835, -0.7216878364870458196 ) ) ;
#173989=CARTESIAN_POINT ( 'NONE',  ( -3.634994582239682526, 6.294558541704648569, 1.082531754730549967 ) ) ;
#173990=CARTESIAN_POINT ( 'NONE',  ( -5.427006627220116286, 9.553534508390610469, -0.7998128361456362523 ) ) ;
#174000=CARTESIAN_POINT ( 'NONE',  ( 7.126746022638799971, 8.343567110280638133, 1.199719254218452047 ) ) ;
#174002=CARTESIAN_POINT ( 'NONE',  ( 4.532168488718122390, 8.509556680138327778, 0.7998128361456271485 ) ) ;
#174003=CARTESIAN_POINT ( 'NONE',  ( 7.198453214212898743, 7.362893269528701268, 0.7998128361456291469 ) ) ;
#174006=CARTESIAN_POINT ( 'NONE',  ( 4.706088717274906408, 5.623429937309770921, 1.082531754730549078 ) ) ;
#174024=CARTESIAN_POINT ( 'NONE',  ( 3.413620815590684199, 7.204584394822967752, 0.7998128361456281477 ) ) ;
#174028=CARTESIAN_POINT ( 'NONE',  ( 4.213551878797002992, 8.137837301896977849, 0.000000000000000000 ) ) ;
#174033=CARTESIAN_POINT ( 'NONE',  ( 5.643937085038755797, 9.806620042512378177, -0.7998128361456481317 ) ) ;
#174037=CARTESIAN_POINT ( 'NONE',  ( 4.909461021924231616, 8.741805268971372556, 0.7216878364870317197 ) ) ;
#174039=CARTESIAN_POINT ( 'NONE',  ( -5.387385936583832802, 7.378645907471495846, -1.599625672291271394 ) ) ;
#174040=CARTESIAN_POINT ( 'NONE',  ( 6.039231080244466199, 6.010467446565510130, 0.7998128361456352531 ) ) ;
#174050=CARTESIAN_POINT ( 'NONE',  ( -5.659602779061863487, 5.567567761852417085, 0.7998128361456281477 ) ) ;
#174068=CARTESIAN_POINT ( 'NONE',  ( 3.719872605471106208, 6.605953636083950364, 7.500000000000000000 ) ) ;
#174080=CARTESIAN_POINT ( 'NONE',  ( 2.929970594329034395, 6.432399770110250437, -0.7216878364870338292 ) ) ;
#174086=CARTESIAN_POINT ( 'NONE',  ( 3.675669042636310557, 6.342012078834061484, -1.082531754730549967 ) ) ;
#174099=CARTESIAN_POINT ( 'NONE',  ( -4.749098946536820520, 8.762642214260091933, 0.7998128361456281477 ) ) ;
#174101=CARTESIAN_POINT ( 'NONE',  ( 7.973603738168424826, 8.475161580717541554, 0.000000000000000000 ) ) ;
#174103=B_SPLINE_CURVE_WITH_KNOTS ( 'NONE', 3,
 ( #37283, #185651, #70819, #172636, #90313, #206174 ),
 .UNSPECIFIED., .F., .F.,
 ( 4, 2, 4 ),
 ( 0.000000000000000000, 0.0006788971861661711581, 0.001357794372332342316 ),
 .UNSPECIFIED. ) ;
#174112=CARTESIAN_POINT ( 'NONE',  ( -5.822300622425855110, 5.757381912443740646, 0.7998128361456281477 ) ) ;
#174118=FACE_OUTER_BOUND ( 'NONE', #172268, .T. ) ;
#174120=ORIENTED_EDGE ( 'NONE', *, *, #7244, .F. ) ;
#174122=CARTESIAN_POINT ( 'NONE',  ( -4.767627293860968507, 5.591261926706423857, -1.199719254218453823 ) ) ;
#174143=CARTESIAN_POINT ( 'NONE',  ( -5.121948170912633991, 9.197632976031879792, -0.7998128361456362523 ) ) ;
#174146=CARTESIAN_POINT ( 'NONE',  ( -3.806807270387036368, 7.663301925418665839, 0.000000000000000000 ) ) ;
#174155=CARTESIAN_POINT ( 'NONE',  ( -6.402982088906444602, 6.898597865962027065, -0.7910698893406533649 ) ) ;
#174171=CARTESIAN_POINT ( 'NONE',  ( -6.317173229324657413, 6.334733287159020954, 0.000000000000000000 ) ) ;
#174197=CARTESIAN_POINT ( 'NONE',  ( 5.664274315459256748, 9.830346811336296398, -0.7998128361456481317 ) ) ;
#174199=CARTESIAN_POINT ( 'NONE',  ( 5.180097208873055692, 8.201141289397330780, -1.199719254218450271 ) ) ;
#174208=CARTESIAN_POINT ( 'NONE',  ( 6.313255789627134185, 6.931427761816202349, -0.8697005975955690582 ) ) ;
#174213=CARTESIAN_POINT ( 'NONE',  ( 6.469672735924913987, 6.762149564967588233, 0.2594904213018677797 ) ) ;
#174215=CARTESIAN_POINT ( 'NONE',  ( 7.214347136247488912, 7.589362211809770997, -0.7216878364870317197 ) ) ;
#174222=CARTESIAN_POINT ( 'NONE',  ( -5.469788628470539926, 5.346117919495872783, -0.7998128361456362523 ) ) ;
#174231=CARTESIAN_POINT ( 'NONE',  ( -5.682275777458886346, 7.722684055159061423, 1.443375672974058777 ) ) ;
#174235=CARTESIAN_POINT ( 'NONE',  ( 5.996449078994045223, 10.21788403546024782, 0.7998128361456331437 ) ) ;
#174241=CARTESIAN_POINT ( 'NONE',  ( -3.311934663488232733, 7.085950550703385531, -0.7998128361456481317 ) ) ;
#174251=CARTESIAN_POINT ( 'NONE',  ( 7.452141709366786770, 8.723195411463290583, 1.199719254218452047 ) ) ;
#174268=CARTESIAN_POINT ( 'NONE',  ( -5.803772275101700906, 8.928762199997411386, -1.199719254218452047 ) ) ;
#174272=CARTESIAN_POINT ( 'NONE',  ( -6.457230086593013674, 6.786253674495239530, 0.3580049749655131452 ) ) ;
#174289=CARTESIAN_POINT ( 'NONE',  ( 5.560252395380215873, 6.619954228432645138, 1.082531754730549078 ) ) ;
#174290=ORIENTED_EDGE ( 'NONE', *, *, #72253, .F. ) ;
#174297=CARTESIAN_POINT ( 'NONE',  ( -4.827315259302275230, 8.191461316972679541, -0.9557250891021950023 ) ) ;
#174300=CARTESIAN_POINT ( 'NONE',  ( -5.153507786970276783, 6.145418851954329575, -1.082531754730549967 ) ) ;
#174331=CARTESIAN_POINT ( 'NONE',  ( 3.230585741806197841, 6.991043475407723307, 0.7998128361456271485 ) ) ;
#174343=CARTESIAN_POINT ( 'NONE',  ( -5.153507786970262572, 9.026526494858359229, -0.7216878364870338292 ) ) ;
#174345=CARTESIAN_POINT ( 'NONE',  ( 6.003228155800906407, 10.22579295840155744, 0.000000000000000000 ) ) ;
#174363=CARTESIAN_POINT ( 'NONE',  ( -3.689227196694346400, 6.357829925235092716, -1.082531754730546636 ) ) ;
#174395=CARTESIAN_POINT ( 'NONE',  ( -8.106849506328558164, 8.422688943663599659, 0.000000000000000000 ) ) ;
#174398=CARTESIAN_POINT ( 'NONE',  ( -5.586841817283045408, 8.675676665875643678, 1.199719254218454489 ) ) ;
#174403=CARTESIAN_POINT ( 'NONE',  ( -6.251718229232846369, 9.347402796530044355, -1.082531754730549967 ) ) ;
#174405=CARTESIAN_POINT ( 'NONE',  ( 7.987161891782087686, 8.490979426600148372, -0.7216878364870317197 ) ) ;
#174407=CARTESIAN_POINT ( 'NONE',  ( -4.516801452008150086, 5.298631777878131111, 1.199719254218452935 ) ) ;
#174411=CARTESIAN_POINT ( 'NONE',  ( -5.178288325776719603, 5.006034233019745372, 0.000000000000000000 ) ) ;
#174421=CARTESIAN_POINT ( 'NONE',  ( 5.170590401584001405, 7.751911629329717002, -1.182414590771277085 ) ) ;
#174425=CARTESIAN_POINT ( 'NONE',  ( 3.790386463472274148, 6.579812086429759788, 1.199719254218452047 ) ) ;
#174428=EDGE_LOOP ( 'NONE', ( #173720, #94610, #8745, #74426, #66392, #89559, #78206 ) ) ;
#174448=CARTESIAN_POINT ( 'NONE',  ( 8.005163354226054295, 8.304055099544019214, 0.000000000000000000 ) ) ;
#174462=CARTESIAN_POINT ( 'NONE',  ( 0.000000000000000000, 0.08000000000000020983, 0.000000000000000000 ) ) ;
#174463=CARTESIAN_POINT ( 'NONE',  ( 6.044612043767858545, 7.151903759757407109, 1.166429756139725660 ) ) ;
#174464=CARTESIAN_POINT ( 'NONE',  ( -4.299344108864953995, 7.069632989434141201, -1.082531754730551743 ) ) ;
#174489=ORIENTED_EDGE ( 'NONE', *, *, #142352, .T. ) ;
#174494=CARTESIAN_POINT ( 'NONE',  ( 5.401997860402196316, 5.267028690082820930, 0.000000000000000000 ) ) ;
#174514=CARTESIAN_POINT ( 'NONE',  ( -7.306918443122272677, 7.489436036589583345, 0.7998128361456341429 ) ) ;
#174528=CARTESIAN_POINT ( 'NONE',  ( 4.386945222473598527, 7.275797305264619652, -1.199719254218452047 ) ) ;
#174539=CARTESIAN_POINT ( 'NONE',  ( 4.833798585616123411, 8.091670711168742258, 0.8834425186924599327 ) ) ;
#174541=CARTESIAN_POINT ( 'NONE',  ( 5.028717893731355026, 7.888467461587344687, 1.094519599958807765 ) ) ;
#174549=CARTESIAN_POINT ( 'NONE',  ( -3.855349344377450027, 7.344262544186459074, -0.7342876487609185654 ) ) ;
#174557=ORIENTED_EDGE ( 'NONE', *, *, #193710, .T. ) ;
#174561=ORIENTED_EDGE ( 'NONE', *, *, #32706, .F. ) ;
#174563=CARTESIAN_POINT ( 'NONE',  ( -6.303615075710993665, 6.318915441276411471, -0.7998128361456362523 ) ) ;
#174565=CARTESIAN_POINT ( 'NONE',  ( 4.492547798081839794, 6.334668079219206049, 1.599625672291262513 ) ) ;
#174568=CARTESIAN_POINT ( 'NONE',  ( -4.990283058281743678, 7.979691447040783814, -1.199719254218453823 ) ) ;
#174571=CARTESIAN_POINT ( 'NONE',  ( 7.862802741282558294, 8.137967717776607657, 0.000000000000000000 ) ) ;
#174576=CARTESIAN_POINT ( 'NONE',  ( -4.780157383859068077, 8.266535928781179265, -0.8537241328121815132 ) ) ;
#174593=CARTESIAN_POINT ( 'NONE',  ( 4.245111494854632461, 7.966730820723463502, 0.000000000000000000 ) ) ;
#174596=CARTESIAN_POINT ( 'NONE',  ( -7.774674742793745708, 8.035151719539642912, 0.7998128361456341429 ) ) ;
#174598=ORIENTED_EDGE ( 'NONE', *, *, #72494, .T. ) ;
#174612=CARTESIAN_POINT ( 'NONE',  ( 3.549202351727371862, 7.362762853649070571, -0.7998128361456362523 ) ) ;
#174616=CARTESIAN_POINT ( 'NONE',  ( -4.913752204202785023, 4.881785571126718182, -0.5639616748225815268 ) ) ;
#174662=CARTESIAN_POINT ( 'NONE',  ( -6.084577077482911101, 10.32070003369722144, 0.000000000000000000 ) ) ;
#174667=FACE_OUTER_BOUND ( 'NONE', #159459, .T. ) ;
#174668=ORIENTED_EDGE ( 'NONE', *, *, #173439, .T. ) ;
#174669=CARTESIAN_POINT ( 'NONE',  ( -4.984557751679625781, 5.844347460828191565, 1.199719254218452935 ) ) ;
#174678=CARTESIAN_POINT ( 'NONE',  ( -5.002032328799064231, 4.800402236545811441, -0.7998128361456362523 ) ) ;
#174680=CARTESIAN_POINT ( 'NONE',  ( 5.544801429207002030, 7.539493339695484408, -1.337888636821100041 ) ) ;
#174684=CARTESIAN_POINT ( 'NONE',  ( 5.727393547130178675, 5.646656991265468939, 0.000000000000000000 ) ) ;
#174688=CARTESIAN_POINT ( 'NONE',  ( -6.563028877466991595, 9.814561569423593923, 1.199719254218452935 ) ) ;
#174690=ADVANCED_FACE ( 'NONE', ( #120970 ), #71037, .F. ) ;
#174692=ORIENTED_EDGE ( 'NONE', *, *, #170147, .F. ) ;
#174693=VECTOR ( 'NONE', #144206, 1000.000000000000114 ) ;
#174695=CARTESIAN_POINT ( 'NONE',  ( -4.176793841461789114, 7.030620694084159794, -1.199719254218455378 ) ) ;
#174699=CARTESIAN_POINT ( 'NONE',  ( 5.356880090730872013, 6.382686539675070492, 1.082531754730549078 ) ) ;
#174700=CARTESIAN_POINT ( 'NONE',  ( -4.773879485343255347, 8.583626809626847987, 0.000000000000000000 ) ) ;
#174707=CARTESIAN_POINT ( 'NONE',  ( 3.932747076415766596, 6.745899468197171345, 1.199719254218451159 ) ) ;
#174712=CARTESIAN_POINT ( 'NONE',  ( -4.497580221328687067, 8.250285843153577048, -0.1439893610950530312 ) ) ;
#174716=CARTESIAN_POINT ( 'NONE',  ( 5.987861119090863049, 7.014868056141362551, 1.199719254218452047 ) ) ;
#174739=CARTESIAN_POINT ( 'NONE',  ( 4.594558193676899549, 8.374302254291812631, 0.02480325318809234458 ) ) ;
#174746=CARTESIAN_POINT ( 'NONE',  ( 7.289443866002793371, 8.533381260871966134, 1.199719254218452047 ) ) ;
#174751=CARTESIAN_POINT ( 'NONE',  ( -4.820236115778962827, 8.125194398966316456, -0.8510355349711593576 ) ) ;
#174760=CARTESIAN_POINT ( 'NONE',  ( -6.770317605177755382, 8.992066187497757213, 1.599625672291269396 ) ) ;
#174766=LINE ( 'NONE', #72949, #187923 ) ;
#174771=CARTESIAN_POINT ( 'NONE',  ( 5.189738938980948291, 9.276722205444929870, 0.000000000000000000 ) ) ;
#174778=CARTESIAN_POINT ( 'NONE',  ( 5.011674058906918638, 5.875983152593414971, 1.199719254218452047 ) ) ;
#174781=CARTESIAN_POINT ( 'NONE',  ( 5.438229012412886476, 7.437962829272074750, -1.443375672974078761 ) ) ;
#174784=ADVANCED_FACE ( 'NONE', ( #11422 ), #29808, .T. ) ;
#174797=CARTESIAN_POINT ( 'NONE',  ( -4.065465959251405081, 5.836405933916976707, -1.599625672291271394 ) ) ;
#174798=CARTESIAN_POINT ( 'NONE',  ( 5.722950238744187956, 9.690876021928001904, 0.7216878364870317197 ) ) ;
#174811=CARTESIAN_POINT ( 'NONE',  ( -5.204350862799341115, 7.165104988056252289, -1.599625672291271394 ) ) ;
#174812=CARTESIAN_POINT ( 'NONE',  ( -5.041653019435350380, 6.975290837464928728, -1.599625672291271394 ) ) ;
#174814=CARTESIAN_POINT ( 'NONE',  ( 6.495764994278795612, 9.632124022417032805, 1.082531754730549078 ) ) ;
#174821=DIRECTION ( 'NONE',  ( 0.000000000000000000, 1.000000000000000000, 1.496258514059622730E-16 ) ) ;
#174826=CARTESIAN_POINT ( 'NONE',  ( -6.259328228163411723, 6.916251825828671151, -0.7980491773402348388 ) ) ;
#174829=CARTESIAN_POINT ( 'NONE',  ( 4.367134877377630175, 7.148722219365612141, -1.082531754730548412 ) ) ;
#174833=CARTESIAN_POINT ( 'NONE',  ( -6.414942957921379474, 7.513130201443591005, -1.199719254218452047 ) ) ;
#174849=CARTESIAN_POINT ( 'NONE',  ( 5.722423353419669567, 8.833855124701747386, 1.199719254218451159 ) ) ;
#174883=CARTESIAN_POINT ( 'NONE',  ( 6.129694847154206983, 8.244672969803623630, -1.443375672974078761 ) ) ;
#174890=CARTESIAN_POINT ( 'NONE',  ( 6.902509602688803980, 9.146290184594002781, -1.443375672974064550 ) ) ;
#174914=CARTESIAN_POINT ( 'NONE',  ( -4.817943484809863008, 6.714296380401858499, 1.599625672291263179 ) ) ;
#174916=CARTESIAN_POINT ( 'NONE',  ( 4.814553946184248368, 7.670711132973337065, -1.082531754730548412 ) ) ;
#174921=CARTESIAN_POINT ( 'NONE',  ( -5.330290668828105538, 6.247702530834755130, 1.199719254218452935 ) ) ;
#174926=CARTESIAN_POINT ( 'NONE',  ( -5.334207092333882017, 5.187939460669764635, 0.7998128361456281477 ) ) ;
#174933=CARTESIAN_POINT ( 'NONE',  ( -5.581116510680924847, 6.540332679663050541, -1.199719254218453823 ) ) ;
#174941=CARTESIAN_POINT ( 'NONE',  ( -4.821859908315634158, 5.654533310236863564, 1.199719254218452935 ) ) ;
#174945=CARTESIAN_POINT ( 'NONE',  ( -6.455090533882206216, 7.663932056684933158, -1.082531754730549967 ) ) ;
#174946=CARTESIAN_POINT ( 'NONE',  ( -5.356880090730904875, 7.343055753976412525, 1.443375672974058777 ) ) ;
#174947=CARTESIAN_POINT ( 'NONE',  ( 6.200875153403774043, 8.327716660428123419, -1.599625672291283607 ) ) ;
#174948=CARTESIAN_POINT ( 'NONE',  ( -6.805266759416629618, 6.904175738932996964, 0.000000000000000000 ) ) ;
#174956=EDGE_LOOP ( 'NONE', ( #67779, #42543, #27441, #145528 ) ) ;
#174966=CARTESIAN_POINT ( 'NONE',  ( 8.025500584646550806, 8.327781868367935658, 0.000000000000000000 ) ) ;
#174972=CARTESIAN_POINT ( 'NONE',  ( -5.346851039111045978, 6.199209027673974859, 1.173132900504408438 ) ) ;
#174985=CARTESIAN_POINT ( 'NONE',  ( 5.303225773876714122, 7.631601692149430072, -1.229104931163179426 ) ) ;
#175000=CARTESIAN_POINT ( 'NONE',  ( 5.352436782344940802, 9.466536356036257871, 0.000000000000000000 ) ) ;
#175003=CARTESIAN_POINT ( 'NONE',  ( -4.085803189671902480, 5.860132702740892263, -1.599625672291271394 ) ) ;
#175006=CARTESIAN_POINT ( 'NONE',  ( -7.065207446052813367, 8.375735120883982532, -1.082531754730549967 ) ) ;
#175016=CARTESIAN_POINT ( 'NONE',  ( 7.343676480457483002, 8.596652644402405841, -1.199719254218452047 ) ) ;
#175017=CARTESIAN_POINT ( 'NONE',  ( 6.527324610336440180, 6.579909898339485252, 0.7998128361456331437 ) ) ;
#175026=CARTESIAN_POINT ( 'NONE',  ( 4.947799714344386146, 4.737130853015369958, -0.7998128361456481317 ) ) ;
#175032=CARTESIAN_POINT ( 'NONE',  ( 6.038177310039780643, 8.137902509836795417, -1.599625672291283607 ) ) ;
#175044=CARTESIAN_POINT ( 'NONE',  ( 6.211043768836170820, 9.299949259400630552, 1.082531754730549967 ) ) ;
#175045=CARTESIAN_POINT ( 'NONE',  ( -4.163762573172648196, 7.871823745427799501, 0.000000000000000000 ) ) ;
#175046=CARTESIAN_POINT ( 'NONE',  ( -6.831329296439251131, 9.063246493969506545, -1.599625672291271394 ) ) ;
#175048=CARTESIAN_POINT ( 'NONE',  ( -4.803422538100232231, 4.881709431271958444, 0.4436329477108340025 ) ) ;
#175058=CARTESIAN_POINT ( 'NONE',  ( 4.179656494762836516, 8.098292687190454586, -0.7998128361456362523 ) ) ;
#175059=CARTESIAN_POINT ( 'NONE',  ( 5.580062740476173566, 8.667767742934335828, 1.199719254218451159 ) ) ;
#175062=CARTESIAN_POINT ( 'NONE',  ( 6.003228155800906407, 10.22579295840155744, 0.000000000000000000 ) ) ;
#175080=CARTESIAN_POINT ( 'NONE',  ( 4.441177836928239309, 7.339068688795062911, 1.199719254218452047 ) ) ;
#175084=CARTESIAN_POINT ( 'NONE',  ( 6.398522151006641678, 6.429640362454684954, 0.000000000000000000 ) ) ;
#175095=CARTESIAN_POINT ( 'NONE',  ( 5.858531774880875176, 9.849054480754103835, -0.7216878364870458196 ) ) ;
#175097=CARTESIAN_POINT ( 'NONE',  ( -6.252245114557387851, 7.323316050852266557, -1.199719254218453823 ) ) ;
#175098=CARTESIAN_POINT ( 'NONE',  ( 4.716257332707354699, 6.595662536282280719, -1.599625672291269396 ) ) ;
#175109=CARTESIAN_POINT ( 'NONE',  ( -4.664887371553763096, 7.600063145858131364, -1.199719254218453823 ) ) ;
#175137=FACE_OUTER_BOUND ( 'NONE', #24839, .T. ) ;
#175144=CARTESIAN_POINT ( 'NONE',  ( 5.058600711230250013, 5.074324715956299414, -0.7216878364870458196 ) ) ;
#175155=CARTESIAN_POINT ( 'NONE',  ( -5.061990249855848667, 6.999017606288844284, -1.599625672291271394 ) ) ;
#175157=CARTESIAN_POINT ( 'NONE',  ( -5.261446130555064826, 8.296048364692991228, 1.199719254218452935 ) ) ;
#175159=CARTESIAN_POINT ( 'NONE',  ( 6.333067150914805765, 9.442309871825708356, 1.082531754730549967 ) ) ;
#175168=CARTESIAN_POINT ( 'NONE',  ( -6.069210040772897052, 7.109775131437022999, -1.199719254218453823 ) ) ;
#175174=CARTESIAN_POINT ( 'NONE',  ( -5.153507786970275006, 7.105788066255672497, -1.443375672974066548 ) ) ;
#175178=( BOUNDED_SURFACE ( )  B_SPLINE_SURFACE ( 1, 2, ( 
 ( #80320, #66161, #132307, #47855, #49954, #99772, #17423, #83506, #149588, #97661, #51023, #29451, #79259, #211374, #195148, #63000, #64077, #30521, #46782, #112896, #178907, #113966, #170089, #72584, #169028, #204702, #37970, #166910, #138685, #117144, #203636, #200442, #54221, #183148, #120360, #86714, #100825, #84583, #88869, #150670, #2231, #167967, #87785, #36888, #68308, #104044, #19573, #202570, #153859, #185264, #134439, #151733, #53149, #71508, #69373, #137618, #55287, #121437, #187406, #52088, #135481, #118215, #39037, #105122, #171162, #201503, #22751, #13582, #115420, #149995, #146821, #494, #50355, #161992, #147871, #29856, #30928, #82845, #15702, #1566, #165166, #97004, #67628, #179307, #81788, #132704, #116477, #16761, #95936, #79655, #198710, #163057, #182467, #14637, #66562, #114365, #34096, #196611, #113300, #148921, #180359, #213887, #181412, #178240, #129562, #31985, #100167, #98063, #80731, #48250, #65509, #131655, #164119, #197658, #49304, #166232, #212841, #64478, #17822, #83905, #130619, #133773, #33039, #47187, #211773, #99117, #195549, #199781, #51427, #145772, #63411, #186742, #171560, #102295, #135877, #118611, #117547, #101224, #185667, #184599, #36216, #167307, #139085, #201897, #134827, #136950, #168369, #105526, #55678, #37296, #35148, #88188, #19964, #84978, #169431, #86048, #119680, #5835, #152124, #68705, #121834, #3694, #69771, #18894, #151070, #53549, #23158, #187805, #183541, #104443, #103369, #21015, #52482, #200831, #2632, #87113, #153183, #154261, #39433, #89272, #38364, #202975, #205112, #4757, #70833, #54616, #120764, #170492, #22076, #71906, #138015, #204030, #155321, #6905, #72982, #206188, #157471, #208318, #42664, #12255, #176909, #108773, #109842, #59948, #192064, #126104, #94615, #123978, #27445, #93543, #25309, #174798, #189946, #159587, #26374, #9066, #92487, #11186, #43727, #77265, #143379, #190998, #160659, #78332, #158526, #10123, #7983, #76198, #107706, #41595, #209377, #125043, #61021, #142308, #175856, #144454, #127180, #56755, #193148, #106622, #122920 ),
 ( #44798, #173732, #74072, #110903, #91411, #75141, #40519, #172651, #141250, #28524, #188878, #24226, #90328, #207259, #58888, #57816, #140165, #156397, #79404, #130372, #32791, #248, #66320, #131410, #15449, #83657, #210457, #114120, #95685, #31736, #14381, #81537, #180112, #177986, #129321, #17573, #65264, #147619, #45862, #213638, #182222, #179052, #98866, #82594, #194217, #97809, #62095, #63156, #115171, #48002, #33845, #197410, #195298, #99926, #211520, #163872, #164918, #148680, #49051, #128254, #111983, #16511, #46928, #132464, #113046, #198466, #146572, #50111, #80473, #145521, #181166, #212591, #116231, #165988, #29599, #161739, #64229, #13330, #196362, #30671, #96754, #162804, #202726, #154012, #200591, #5578, #2385, #18654, #183295, #52239, #167062, #84734, #53304, #187560, #134591, #4514, #203790, #118367, #168123, #150822, #149747, #133525, #3457, #68463, #184355, #199532, #171313, #19724, #35977, #169183, #102058, #137772, #87938, #69527, #67385, #120516, #85803, #117298, #201655, #151883, #135634, #38125, #119436, #100973, #71658, #185423, #37041, #51175, #34901, #103125, #55436, #121588, #1324, #136702, #20775, #86871, #152937, #70587, #54378, #186494, #104198, #170245, #39187, #105276, #21830, #22908, #179579, #89024, #209916, #191539, #127719, #110378, #111442, #61554, #59421, #10656, #113577, #161194, #177446, #141789, #29061, #63685, #60480, #128770, #178512, #75679, #193679, #155077, #159060, #210981, #143919, #129841, #78855, #76729, #195822, #93017, #45322, #46384, #30124, #144976, #9602, #207793, #112502, #142845, #96213, #208850, #194746, #27989, #162264, #176383, #26910, #62608, #94085, #95144, #12782, #125577, #43204, #160123, #13851, #11724, #126639, #77800, #79927, #192604, #44257, #47462, #146034, #109317, #212043, #175327, #149201, #18111, #34375, #116758, #48519, #117839, #180633, #131928, #182757, #17042, #201127, #151351, #83121, #84197, #100448, #166521, #150287, #68993, #98325, #1854, #67914, #214152, #776, #164390, #134060, #66842, #197938, #132986, #200068, #51719, #183831 ) ),
 .UNSPECIFIED., .F., .F., .T. ) 
 B_SPLINE_SURFACE_WITH_KNOTS ( ( 2, 2 ),
 ( 3, 2, 2, 2, 2, 2, 2, 2, 2, 2, 2, 2, 2, 2, 2, 2, 2, 2, 2, 2, 2, 2, 2, 2, 2, 2, 2, 2, 2, 2, 2, 2, 2, 2, 2, 2, 2, 2, 2, 2, 2, 2, 2, 2, 2, 2, 2, 2, 2, 2, 2, 2, 2, 2, 2, 2, 2, 2, 2, 2, 2, 2, 2, 2, 2, 2, 2, 2, 2, 2, 2, 2, 2, 2, 2, 2, 2, 2, 2, 2, 2, 2, 2, 2, 2, 2, 2, 2, 2, 2, 2, 2, 2, 2, 2, 2, 2, 2, 2, 2, 2, 2, 2, 2, 2, 2, 2, 2, 2, 2, 2, 2, 2, 2, 2, 2, 2, 2, 2, 2, 3 ),
 ( 0.000000000000000000, 1.000000000000000000 ),
 ( 0.000000000000000000, 0.008333333333333333218, 0.01666666666666666644, 0.02500000000000000139, 0.03333333333333333287, 0.04166666666666666435, 0.05000000000000000278, 0.05833333333333333426, 0.06666666666666666574, 0.07499999999999999722, 0.08333333333333332871, 0.09166666666666666019, 0.1000000000000000056, 0.1083333333333333370, 0.1166666666666666685, 0.1250000000000000000, 0.1333333333333333315, 0.1416666666666666630, 0.1499999999999999944, 0.1583333333333333259, 0.1666666666666666574, 0.1749999999999999889, 0.1833333333333333204, 0.1916666666666666796, 0.2000000000000000111, 0.2083333333333333426, 0.2166666666666666741, 0.2250000000000000056, 0.2333333333333333370, 0.2416666666666666685, 0.2500000000000000000, 0.2583333333333333592, 0.2666666666666666630, 0.2750000000000000222, 0.2833333333333333259, 0.2916666666666666852, 0.2999999999999999889, 0.3083333333333333481, 0.3166666666666666519, 0.3250000000000000111, 0.3333333333333333148, 0.3416666666666666741, 0.3499999999999999778, 0.3583333333333333370, 0.3666666666666666408, 0.3750000000000000000, 0.3833333333333333592, 0.3916666666666666630, 0.4000000000000000222, 0.4083333333333333259, 0.4166666666666666852, 0.4249999999999999889, 0.4333333333333333481, 0.4416666666666666519, 0.4500000000000000111, 0.4583333333333333148, 0.4666666666666666741, 0.4749999999999999778, 0.4833333333333333370, 0.4916666666666666408, 0.5000000000000000000, 0.5083333333333333037, 0.5166666666666667185, 0.5250000000000000222, 0.5333333333333333259, 0.5416666666666666297, 0.5500000000000000444, 0.5583333333333333481, 0.5666666666666666519, 0.5749999999999999556, 0.5833333333333333703, 0.5916666666666666741, 0.5999999999999999778, 0.6083333333333332815, 0.6166666666666666963, 0.6250000000000000000, 0.6333333333333333037, 0.6416666666666667185, 0.6500000000000000222, 0.6583333333333333259, 0.6666666666666666297, 0.6750000000000000444, 0.6833333333333333481, 0.6916666666666666519, 0.6999999999999999556, 0.7083333333333333703, 0.7166666666666666741, 0.7249999999999999778, 0.7333333333333332815, 0.7416666666666666963, 0.7500000000000000000, 0.7583333333333333037, 0.7666666666666667185, 0.7750000000000000222, 0.7833333333333333259, 0.7916666666666666297, 0.8000000000000000444, 0.8083333333333333481, 0.8166666666666666519, 0.8249999999999999556, 0.8333333333333333703, 0.8416666666666666741, 0.8499999999999999778, 0.8583333333333332815, 0.8666666666666666963, 0.8750000000000000000, 0.8833333333333333037, 0.8916666666666667185, 0.9000000000000000222, 0.9083333333333333259, 0.9166666666666666297, 0.9250000000000000444, 0.9333333333333333481, 0.9416666666666666519, 0.9499999999999999556, 0.9583333333333333703, 0.9666666666666666741, 0.9749999999999999778, 0.9833333333333332815, 0.9916666666666666963, 1.000000000000000000 ),
 .UNSPECIFIED. ) 
 GEOMETRIC_REPRESENTATION_ITEM ( )  RATIONAL_B_SPLINE_SURFACE ( (
 ( 1.000000000000000000, 0.8660254037844387076, 1.000000000000000000, 0.8660254037844387076, 1.000000000000000000, 0.8660254037844387076, 1.000000000000000000, 0.8660254037844387076, 1.000000000000000000, 0.8660254037844387076, 1.000000000000000000, 0.8660254037844387076, 1.000000000000000000, 0.8660254037844387076, 1.000000000000000000, 0.8660254037844387076, 1.000000000000000000, 0.8660254037844387076, 1.000000000000000000, 0.8660254037844387076, 1.000000000000000000, 0.8660254037844387076, 1.000000000000000000, 0.8660254037844387076, 1.000000000000000000, 0.8660254037844387076, 1.000000000000000000, 0.8660254037844387076, 1.000000000000000000, 0.8660254037844387076, 1.000000000000000000, 0.8660254037844387076, 1.000000000000000000, 0.8660254037844387076, 1.000000000000000000, 0.8660254037844387076, 1.000000000000000000, 0.8660254037844387076, 1.000000000000000000, 0.8660254037844387076, 1.000000000000000000, 0.8660254037844387076, 1.000000000000000000, 0.8660254037844387076, 1.000000000000000000, 0.8660254037844387076, 1.000000000000000000, 0.8660254037844387076, 1.000000000000000000, 0.8660254037844387076, 1.000000000000000000, 0.8660254037844387076, 1.000000000000000000, 0.8660254037844387076, 1.000000000000000000, 0.8660254037844387076, 1.000000000000000000, 0.8660254037844387076, 1.000000000000000000, 0.8660254037844387076, 1.000000000000000000, 0.8660254037844387076, 1.000000000000000000, 0.8660254037844387076, 1.000000000000000000, 0.8660254037844387076, 1.000000000000000000, 0.8660254037844387076, 1.000000000000000000, 0.8660254037844387076, 1.000000000000000000, 0.8660254037844387076, 1.000000000000000000, 0.8660254037844387076, 1.000000000000000000, 0.8660254037844387076, 1.000000000000000000, 0.8660254037844387076, 1.000000000000000000, 0.8660254037844387076, 1.000000000000000000, 0.8660254037844387076, 1.000000000000000000, 0.8660254037844387076, 1.000000000000000000, 0.8660254037844387076, 1.000000000000000000, 0.8660254037844387076, 1.000000000000000000, 0.8660254037844387076, 1.000000000000000000, 0.8660254037844387076, 1.000000000000000000, 0.8660254037844387076, 1.000000000000000000, 0.8660254037844387076, 1.000000000000000000, 0.8660254037844387076, 1.000000000000000000, 0.8660254037844387076, 1.000000000000000000, 0.8660254037844387076, 1.000000000000000000, 0.8660254037844387076, 1.000000000000000000, 0.8660254037844387076, 1.000000000000000000, 0.8660254037844387076, 1.000000000000000000, 0.8660254037844387076, 1.000000000000000000, 0.8660254037844387076, 1.000000000000000000, 0.8660254037844387076, 1.000000000000000000, 0.8660254037844387076, 1.000000000000000000, 0.8660254037844387076, 1.000000000000000000, 0.8660254037844387076, 1.000000000000000000, 0.8660254037844387076, 1.000000000000000000, 0.8660254037844387076, 1.000000000000000000, 0.8660254037844387076, 1.000000000000000000, 0.8660254037844387076, 1.000000000000000000, 0.8660254037844387076, 1.000000000000000000, 0.8660254037844387076, 1.000000000000000000, 0.8660254037844387076, 1.000000000000000000, 0.8660254037844387076, 1.000000000000000000, 0.8660254037844387076, 1.000000000000000000, 0.8660254037844387076, 1.000000000000000000, 0.8660254037844387076, 1.000000000000000000, 0.8660254037844387076, 1.000000000000000000, 0.8660254037844387076, 1.000000000000000000, 0.8660254037844387076, 1.000000000000000000, 0.8660254037844387076, 1.000000000000000000, 0.8660254037844387076, 1.000000000000000000, 0.8660254037844387076, 1.000000000000000000, 0.8660254037844387076, 1.000000000000000000, 0.8660254037844387076, 1.000000000000000000, 0.8660254037844387076, 1.000000000000000000, 0.8660254037844387076, 1.000000000000000000, 0.8660254037844387076, 1.000000000000000000, 0.8660254037844387076, 1.000000000000000000, 0.8660254037844387076, 1.000000000000000000, 0.8660254037844387076, 1.000000000000000000, 0.8660254037844387076, 1.000000000000000000, 0.8660254037844387076, 1.000000000000000000, 0.8660254037844387076, 1.000000000000000000, 0.8660254037844387076, 1.000000000000000000, 0.8660254037844387076, 1.000000000000000000, 0.8660254037844387076, 1.000000000000000000, 0.8660254037844387076, 1.000000000000000000, 0.8660254037844387076, 1.000000000000000000, 0.8660254037844387076, 1.000000000000000000, 0.8660254037844387076, 1.000000000000000000, 0.8660254037844387076, 1.000000000000000000, 0.8660254037844387076, 1.000000000000000000, 0.8660254037844387076, 1.000000000000000000, 0.8660254037844387076, 1.000000000000000000, 0.8660254037844387076, 1.000000000000000000, 0.8660254037844387076, 1.000000000000000000, 0.8660254037844387076, 1.000000000000000000, 0.8660254037844387076, 1.000000000000000000, 0.8660254037844387076, 1.000000000000000000, 0.8660254037844387076, 1.000000000000000000, 0.8660254037844387076, 1.000000000000000000, 0.8660254037844387076, 1.000000000000000000, 0.8660254037844387076, 1.000000000000000000, 0.8660254037844387076, 1.000000000000000000, 0.8660254037844387076, 1.000000000000000000, 0.8660254037844387076, 1.000000000000000000, 0.8660254037844387076, 1.000000000000000000, 0.8660254037844387076, 1.000000000000000000, 0.8660254037844387076, 1.000000000000000000, 0.8660254037844387076, 1.000000000000000000, 0.8660254037844387076, 1.000000000000000000, 0.8660254037844387076, 1.000000000000000000, 0.8660254037844387076, 1.000000000000000000, 0.8660254037844387076, 1.000000000000000000, 0.8660254037844387076, 1.000000000000000000),
 ( 1.000000000000000000, 0.8660254037844387076, 1.000000000000000000, 0.8660254037844387076, 1.000000000000000000, 0.8660254037844387076, 1.000000000000000000, 0.8660254037844387076, 1.000000000000000000, 0.8660254037844387076, 1.000000000000000000, 0.8660254037844387076, 1.000000000000000000, 0.8660254037844387076, 1.000000000000000000, 0.8660254037844387076, 1.000000000000000000, 0.8660254037844387076, 1.000000000000000000, 0.8660254037844387076, 1.000000000000000000, 0.8660254037844387076, 1.000000000000000000, 0.8660254037844387076, 1.000000000000000000, 0.8660254037844387076, 1.000000000000000000, 0.8660254037844387076, 1.000000000000000000, 0.8660254037844387076, 1.000000000000000000, 0.8660254037844387076, 1.000000000000000000, 0.8660254037844387076, 1.000000000000000000, 0.8660254037844387076, 1.000000000000000000, 0.8660254037844387076, 1.000000000000000000, 0.8660254037844387076, 1.000000000000000000, 0.8660254037844387076, 1.000000000000000000, 0.8660254037844387076, 1.000000000000000000, 0.8660254037844387076, 1.000000000000000000, 0.8660254037844387076, 1.000000000000000000, 0.8660254037844387076, 1.000000000000000000, 0.8660254037844387076, 1.000000000000000000, 0.8660254037844387076, 1.000000000000000000, 0.8660254037844387076, 1.000000000000000000, 0.8660254037844387076, 1.000000000000000000, 0.8660254037844387076, 1.000000000000000000, 0.8660254037844387076, 1.000000000000000000, 0.8660254037844387076, 1.000000000000000000, 0.8660254037844387076, 1.000000000000000000, 0.8660254037844387076, 1.000000000000000000, 0.8660254037844387076, 1.000000000000000000, 0.8660254037844387076, 1.000000000000000000, 0.8660254037844387076, 1.000000000000000000, 0.8660254037844387076, 1.000000000000000000, 0.8660254037844387076, 1.000000000000000000, 0.8660254037844387076, 1.000000000000000000, 0.8660254037844387076, 1.000000000000000000, 0.8660254037844387076, 1.000000000000000000, 0.8660254037844387076, 1.000000000000000000, 0.8660254037844387076, 1.000000000000000000, 0.8660254037844387076, 1.000000000000000000, 0.8660254037844387076, 1.000000000000000000, 0.8660254037844387076, 1.000000000000000000, 0.8660254037844387076, 1.000000000000000000, 0.8660254037844387076, 1.000000000000000000, 0.8660254037844387076, 1.000000000000000000, 0.8660254037844387076, 1.000000000000000000, 0.8660254037844387076, 1.000000000000000000, 0.8660254037844387076, 1.000000000000000000, 0.8660254037844387076, 1.000000000000000000, 0.8660254037844387076, 1.000000000000000000, 0.8660254037844387076, 1.000000000000000000, 0.8660254037844387076, 1.000000000000000000, 0.8660254037844387076, 1.000000000000000000, 0.8660254037844387076, 1.000000000000000000, 0.8660254037844387076, 1.000000000000000000, 0.8660254037844387076, 1.000000000000000000, 0.8660254037844387076, 1.000000000000000000, 0.8660254037844387076, 1.000000000000000000, 0.8660254037844387076, 1.000000000000000000, 0.8660254037844387076, 1.000000000000000000, 0.8660254037844387076, 1.000000000000000000, 0.8660254037844387076, 1.000000000000000000, 0.8660254037844387076, 1.000000000000000000, 0.8660254037844387076, 1.000000000000000000, 0.8660254037844387076, 1.000000000000000000, 0.8660254037844387076, 1.000000000000000000, 0.8660254037844387076, 1.000000000000000000, 0.8660254037844387076, 1.000000000000000000, 0.8660254037844387076, 1.000000000000000000, 0.8660254037844387076, 1.000000000000000000, 0.8660254037844387076, 1.000000000000000000, 0.8660254037844387076, 1.000000000000000000, 0.8660254037844387076, 1.000000000000000000, 0.8660254037844387076, 1.000000000000000000, 0.8660254037844387076, 1.000000000000000000, 0.8660254037844387076, 1.000000000000000000, 0.8660254037844387076, 1.000000000000000000, 0.8660254037844387076, 1.000000000000000000, 0.8660254037844387076, 1.000000000000000000, 0.8660254037844387076, 1.000000000000000000, 0.8660254037844387076, 1.000000000000000000, 0.8660254037844387076, 1.000000000000000000, 0.8660254037844387076, 1.000000000000000000, 0.8660254037844387076, 1.000000000000000000, 0.8660254037844387076, 1.000000000000000000, 0.8660254037844387076, 1.000000000000000000, 0.8660254037844387076, 1.000000000000000000, 0.8660254037844387076, 1.000000000000000000, 0.8660254037844387076, 1.000000000000000000, 0.8660254037844387076, 1.000000000000000000, 0.8660254037844387076, 1.000000000000000000, 0.8660254037844387076, 1.000000000000000000, 0.8660254037844387076, 1.000000000000000000, 0.8660254037844387076, 1.000000000000000000, 0.8660254037844387076, 1.000000000000000000, 0.8660254037844387076, 1.000000000000000000, 0.8660254037844387076, 1.000000000000000000, 0.8660254037844387076, 1.000000000000000000, 0.8660254037844387076, 1.000000000000000000, 0.8660254037844387076, 1.000000000000000000, 0.8660254037844387076, 1.000000000000000000, 0.8660254037844387076, 1.000000000000000000, 0.8660254037844387076, 1.000000000000000000, 0.8660254037844387076, 1.000000000000000000, 0.8660254037844387076, 1.000000000000000000, 0.8660254037844387076, 1.000000000000000000, 0.8660254037844387076, 1.000000000000000000, 0.8660254037844387076, 1.000000000000000000, 0.8660254037844387076, 1.000000000000000000, 0.8660254037844387076, 1.000000000000000000, 0.8660254037844387076, 1.000000000000000000, 0.8660254037844387076, 1.000000000000000000, 0.8660254037844387076, 1.000000000000000000, 0.8660254037844387076, 1.000000000000000000, 0.8660254037844387076, 1.000000000000000000) ) ) 
 REPRESENTATION_ITEM ( '' )  SURFACE ( )  );
#175180=CARTESIAN_POINT ( 'NONE',  ( -4.423703259808839938, 8.383013913077441259, 0.7998128361456352531 ) ) ;
#175202=AXIS2_PLACEMENT_3D ( 'NONE', #170058, #204675, #5397 ) ;
#175203=CARTESIAN_POINT ( 'NONE',  ( -6.957269102468015554, 8.145844036748005834, 1.199719254218452047 ) ) ;
#175205=CARTESIAN_POINT ( 'NONE',  ( -4.817943484809863008, 6.714296380401858499, 1.599625672291263179 ) ) ;
#175214=DIRECTION ( 'NONE',  ( 0.6507913734559641616, -0.7592566023653004592, 0.000000000000000000 ) ) ;
#175230=CARTESIAN_POINT ( 'NONE',  ( -6.303615075710993665, 6.318915441276411471, -0.7998128361456362523 ) ) ;
#175239=CARTESIAN_POINT ( 'NONE',  ( 4.572363442555127833, 8.499999999999996447, 0.3169179603640607246 ) ) ;
#175254=CARTESIAN_POINT ( 'NONE',  ( 6.230854113932139171, 9.427024345299638952, 1.199719254218452047 ) ) ;
#175256=CARTESIAN_POINT ( 'NONE',  ( 7.828907357248368726, 8.098423103070084395, 0.7998128361456281477 ) ) ;
#175269=CARTESIAN_POINT ( 'NONE',  ( 4.990887655837901171, 7.926359819171765686, 1.063311220390166234 ) ) ;
#175271=CARTESIAN_POINT ( 'NONE',  ( 7.038091139269835317, 7.383730215335837954, 0.000000000000000000 ) ) ;
#175277=CARTESIAN_POINT ( 'NONE',  ( -4.984557751679625781, 5.844347460828191565, 1.199719254218452935 ) ) ;
#175286=CARTESIAN_POINT ( 'NONE',  ( -6.414416072596849538, 7.616478518518682073, -1.082531754730549967 ) ) ;
#175290=CARTESIAN_POINT ( 'NONE',  ( 6.424584688029230328, 8.588711117491191871, 1.599625672291268286 ) ) ;
#175304=CARTESIAN_POINT ( 'NONE',  ( 4.004454267989866700, 5.765225627445230927, 1.599625672291262513 ) ) ;
#175310=DIRECTION ( 'NONE',  ( -1.000000000000000000, 0.000000000000000000, 0.000000000000000000 ) ) ;
#175325=CARTESIAN_POINT ( 'NONE',  ( -5.855142236255304944, 7.924361590421551860, -1.599625672291271394 ) ) ;
#175327=CARTESIAN_POINT ( 'NONE',  ( 5.643937085038755797, 9.806620042512378177, -0.7998128361456481317 ) ) ;
#175349=CARTESIAN_POINT ( 'NONE',  ( 5.939880696562888751, 7.062853913145737295, -1.082531754730548412 ) ) ;
#175356=CARTESIAN_POINT ( 'NONE',  ( 8.188198428010544205, 8.517596018959260107, 0.000000000000000000 ) ) ;
#175360=CARTESIAN_POINT ( 'NONE',  ( -6.468648687495877958, 6.719380688266201496, 0.000000000000000000 ) ) ;
#175364=CARTESIAN_POINT ( 'NONE',  ( 2.974019135304241335, 6.526997603303817286, -0.5344409224624764310 ) ) ;
#175388=CARTESIAN_POINT ( 'NONE',  ( 4.366607992053101128, 7.252070536440704096, -1.199719254218448494 ) ) ;
#175399=CARTESIAN_POINT ( 'NONE',  ( -5.628043163448566588, 9.580151100749725757, 0.000000000000000000 ) ) ;
#175402=CARTESIAN_POINT ( 'NONE',  ( 4.462041952228939401, 6.299077925724123617, -1.443375672974068769 ) ) ;
#175410=DIRECTION ( 'NONE',  ( 0.7592566023653005702, -0.6507913734559639396, 0.000000000000000000 ) ) ;
#175421=CARTESIAN_POINT ( 'NONE',  ( 3.947104627881218963, 8.980740528189222971, -0.7749999999999996891 ) ) ;
#175425=CARTESIAN_POINT ( 'NONE',  ( -4.533519451513712717, 7.918419216724965182, -0.7681833670988020835 ) ) ;
#175435=ORIENTED_EDGE ( 'NONE', *, *, #186987, .F. ) ;
#175446=CARTESIAN_POINT ( 'NONE',  ( 5.583108480610128765, 5.824348371890765819, -0.7571734975398980438 ) ) ;
#175454=CARTESIAN_POINT ( 'NONE',  ( -5.315678745009726924, 8.359319748223434487, -1.199719254218453823 ) ) ;
#175455=CARTESIAN_POINT ( 'NONE',  ( -4.725015201957559086, 8.329469486225510977, 0.7380969479929339050 ) ) ;
#175456=CARTESIAN_POINT ( 'NONE',  ( -5.468734858265826837, 7.473552982767156294, 1.599625672291263401 ) ) ;
#175457=CARTESIAN_POINT ( 'NONE',  ( -4.489157070319179432, 8.251450656689856444, 5.811111664500048210E-05 ) ) ;
#175463=CARTESIAN_POINT ( 'NONE',  ( -2.979759899953417612, 6.698413326579433225, 0.7998128361456352531 ) ) ;
#175467=CARTESIAN_POINT ( 'NONE',  ( -5.517242166118370150, 5.401480380085008193, 0.7998128361456281477 ) ) ;
#175481=CARTESIAN_POINT ( 'NONE',  ( 4.064412189046650248, 7.963840997188264659, 0.7998128361456271485 ) ) ;
#175485=AXIS2_PLACEMENT_3D ( 'NONE', #19332, #151495, #137384 ) ;
#175503=CARTESIAN_POINT ( 'NONE',  ( 5.071631979963703962, 8.074598522336444262, 1.199719254218451159 ) ) ;
#175504=CARTESIAN_POINT ( 'NONE',  ( 3.223806664999388172, 6.983134552466421674, -0.7998128361456362523 ) ) ;
#175519=CARTESIAN_POINT ( 'NONE',  ( 5.355371708033295874, 7.701368364266228284, 1.317571137710125351 ) ) ;
#175520=CARTESIAN_POINT ( 'NONE',  ( -3.296040741453672318, 6.859481608422314025, 0.7216878364870338292 ) ) ;
#175521=CARTESIAN_POINT ( 'NONE',  ( 3.553645660557675612, 6.199651466408984568, -1.082531754730549967 ) ) ;
#175549=CARTESIAN_POINT ( 'NONE',  ( 5.578253857379852576, 5.472660686556754861, -0.7998128361456481317 ) ) ;
#175568=CARTESIAN_POINT ( 'NONE',  ( -5.661411662158206681, 8.762674818229999829, -1.199719254218452047 ) ) ;
#175571=DIRECTION ( 'NONE',  ( 0.000000000000000000, 0.000000000000000000, -1.000000000000000000 ) ) ;
#175583=CARTESIAN_POINT ( 'NONE',  ( 5.408776937209000657, 5.274937613024121674, 0.7998128361456352531 ) ) ;
#175595=CARTESIAN_POINT ( 'NONE',  ( 5.590372323399994237, 7.390087136190794936, 1.241407824010079652 ) ) ;
#175607=ADVANCED_FACE ( 'NONE', ( #119253 ), #191064, .T. ) ;
#175617=CARTESIAN_POINT ( 'NONE',  ( -5.306037014901836990, 7.283738832175834510, 1.599625672291263179 ) ) ;
#175619=CARTESIAN_POINT ( 'NONE',  ( 5.143339171537801846, 7.093924681584509173, 1.599625672291269396 ) ) ;
#175623=CARTESIAN_POINT ( 'NONE',  ( -7.611976899429754084, 7.845337568948314022, 0.7998128361456341429 ) ) ;
#175626=CARTESIAN_POINT ( 'NONE',  ( 6.851666526859736983, 9.086973262793417661, -1.599625672291269396 ) ) ;
#175631=B_SPLINE_CURVE_WITH_KNOTS ( 'NONE', 3,
 ( #35367, #137165, #132912, #198917, #19112, #85191, #67841, #54835 ),
 .UNSPECIFIED., .F., .F.,
 ( 4, 2, 2, 4 ),
 ( 0.000000000000000000, 0.001552951981419670689, 0.003105903962839341378, 0.006211807925678680155 ),
 .UNSPECIFIED. ) ;
#175632=CARTESIAN_POINT ( 'NONE',  ( -5.847422642759834588, 7.296647196851402839, -1.286413008881746256 ) ) ;
#175648=CARTESIAN_POINT ( 'NONE',  ( 6.400857919427532572, 6.640291458853147866, -0.7216878364870458196 ) ) ;
#175651=CARTESIAN_POINT ( 'NONE',  ( -5.887983850084758330, 10.09134126839936840, 0.7998128361456291469 ) ) ;
#175660=CARTESIAN_POINT ( 'NONE',  ( -4.340018570150322219, 5.196348098997705556, -1.082531754730551743 ) ) ;
#175665=CARTESIAN_POINT ( 'NONE',  ( 4.061549535745618833, 6.896169004081968090, -1.199719254218452047 ) ) ;
#175688=CARTESIAN_POINT ( 'NONE',  ( -4.260029445439560192, 7.236136616047151193, 2.499999999999999556 ) ) ;
#175692=( BOUNDED_SURFACE ( )  B_SPLINE_SURFACE ( 1, 2, ( 
 ( #56622, #122787, #188746, #156268, #73937, #140031, #57691, #41461, #91278, #157337, #11846, #68040, #149329, #83244, #114760, #99518, #166648, #50757, #180757, #133115, #64870, #116886, #199112, #182885, #97401, #80055, #200187, #163456, #30253, #15036, #134179, #13970, #96337, #63807, #51840, #34502, #117959, #214275, #181809, #165576, #129967, #17170, #115821, #908, #146157, #213240, #65908, #212173, #162393, #81128, #31324, #100575, #195954, #47589, #48642, #18239, #66976, #84323, #150409, #1977, #113703, #16099, #164514, #179707, #147214, #131015, #82183, #32384, #197007, #98450, #132054, #148276, #198064, #49693, #33441, #89687, #119026, #72322, #85391, #202317, #139502, #183953, #152528, #6253, #73399, #53966, #120102, #22502, #153605, #138428, #151475, #35563, #136294, #7321, #88613, #154667, #186081, #38782, #105965, #204447, #37715, #56101, #4113, #122258, #188216, #39856, #36633, #19313, #205530, #102717, #101644, #168775, #57166, #167710, #3046, #69115, #135237, #171987, #201251, #5176, #121184, #104863, #52891, #170907, #55035, #23579, #185008, #70183, #71251, #20379, #86464, #103790, #169841, #155736, #21428, #87537, #137365, #187153, #203382, #92890, #93958, #156813, #74485, #110251, #58231, #140591, #206602, #190346, #43077, #11600, #45203, #142718, #207671, #158935, #124388, #109191, #143794, #193560, #8400, #208727, #127594, #111317, #40933, #42008, #108116, #159999, #177321, #125449, #59290, #174143, #176260, #107038, #12660, #78733, #28935, #95019, #25717, #26785, #60353, #77674, #91826, #126516, #157885, #9477, #75550, #141660, #24644, #191410, #175203, #210865, #10531, #76604, #144858, #192478, #44130, #209791, #161069, #189292, #27861, #61427, #123329, #173064, #90753, #198861, #100319, #132856, #179456, #115565, #646, #62491, #130766, #17977, #15852, #196761, #81938, #98212, #212989, #47338, #84064, #129719, #195703, #13731, #180511, #163209, #182624, #146972, #145916, #165320, #150153, #113452, #66711, #164263, #181561, #50508, #211928, #48403, #63562, #148022, #214032, #64627, #128655 ),
 ( #16914, #166385, #194621, #80882, #116630, #33189, #34248, #49446, #46264, #112381, #114515, #32131, #178393, #30005, #96088, #65657, #131804, #162143, #99272, #197813, #82994, #149069, #79804, #31080, #97154, #14791, #104600, #117707, #20116, #171714, #1723, #184746, #38522, #105687, #86201, #152274, #54769, #185815, #170646, #183698, #67780, #168517, #39584, #120917, #186890, #3846, #70987, #138169, #22232, #69920, #88344, #36373, #154408, #5987, #72058, #68858, #51582, #23313, #134978, #89422, #102450, #2787, #204178, #55834, #133930, #37447, #151218, #103524, #121990, #119836, #187956, #199935, #35305, #118761, #101382, #167457, #19051, #136030, #85131, #169583, #202043, #21166, #87270, #53704, #200987, #52633, #153337, #4910, #137100, #203127, #41747, #61171, #25460, #24374, #43880, #28677, #74229, #159739, #42819, #60100, #143533, #90487, #141404, #156551, #108924, #174946, #91567, #177061, #157620, #27598, #26528, #106775, #11337, #139231, #209529, #126258, #158677, #56903, #9217, #92636, #75289, #59031, #172803, #10275, #77418, #76350, #8146, #7056, #127332, #207412, #176006, #125189, #173884, #191151, #123077, #93698, #155471, #107858, #142457, #193301, #190093, #208465, #205262, #109994, #192217, #44946, #73129, #111054, #189034, #40672, #140323, #206341, #57968, #124132, #66462, #48151, #146720, #79553, #96902, #113195, #132603, #12402, #64373, #46011, #16660, #194368, #160811, #62242, #114265, #49199, #47077, #13477, #78483, #65406, #80628, #145671, #31885, #211668, #63304, #195448, #129465, #210615, #95833, #162953, #182363, #179200, #30825, #82745, #198609, #165068, #14531, #147767, #32937, #94764, #212737, #50255, #180261, #130519, #97962, #196509, #164020, #15594, #116375, #161890, #81681, #112131, #213783, #131553, #390, #197555, #178134, #115320, #144600, #181310, #99011, #148818, #128401, #29749, #117449, #19867, #183443, #135779, #53444, #184498, #55584, #36117, #120663, #201802, #199678, #38267, #17716, #88087, #153084, #37196, #149897, #102200, #119582, #168267, #152027, #51321, #185566 ) ),
 .UNSPECIFIED., .F., .F., .T. ) 
 B_SPLINE_SURFACE_WITH_KNOTS ( ( 2, 2 ),
 ( 3, 2, 2, 2, 2, 2, 2, 2, 2, 2, 2, 2, 2, 2, 2, 2, 2, 2, 2, 2, 2, 2, 2, 2, 2, 2, 2, 2, 2, 2, 2, 2, 2, 2, 2, 2, 2, 2, 2, 2, 2, 2, 2, 2, 2, 2, 2, 2, 2, 2, 2, 2, 2, 2, 2, 2, 2, 2, 2, 2, 2, 2, 2, 2, 2, 2, 2, 2, 2, 2, 2, 2, 2, 2, 2, 2, 2, 2, 2, 2, 2, 2, 2, 2, 2, 2, 2, 2, 2, 2, 2, 2, 2, 2, 2, 2, 2, 2, 2, 2, 2, 2, 2, 2, 2, 2, 2, 2, 2, 2, 2, 2, 2, 2, 2, 2, 2, 2, 2, 2, 3 ),
 ( 0.000000000000000000, 1.000000000000000000 ),
 ( 0.000000000000000000, 0.008333333333333333218, 0.01666666666666666644, 0.02500000000000000139, 0.03333333333333333287, 0.04166666666666666435, 0.05000000000000000278, 0.05833333333333333426, 0.06666666666666666574, 0.07499999999999999722, 0.08333333333333332871, 0.09166666666666666019, 0.1000000000000000056, 0.1083333333333333370, 0.1166666666666666685, 0.1250000000000000000, 0.1333333333333333315, 0.1416666666666666630, 0.1499999999999999944, 0.1583333333333333259, 0.1666666666666666574, 0.1749999999999999889, 0.1833333333333333204, 0.1916666666666666796, 0.2000000000000000111, 0.2083333333333333426, 0.2166666666666666741, 0.2250000000000000056, 0.2333333333333333370, 0.2416666666666666685, 0.2500000000000000000, 0.2583333333333333592, 0.2666666666666666630, 0.2750000000000000222, 0.2833333333333333259, 0.2916666666666666852, 0.2999999999999999889, 0.3083333333333333481, 0.3166666666666666519, 0.3250000000000000111, 0.3333333333333333148, 0.3416666666666666741, 0.3499999999999999778, 0.3583333333333333370, 0.3666666666666666408, 0.3750000000000000000, 0.3833333333333333592, 0.3916666666666666630, 0.4000000000000000222, 0.4083333333333333259, 0.4166666666666666852, 0.4249999999999999889, 0.4333333333333333481, 0.4416666666666666519, 0.4500000000000000111, 0.4583333333333333148, 0.4666666666666666741, 0.4749999999999999778, 0.4833333333333333370, 0.4916666666666666408, 0.5000000000000000000, 0.5083333333333333037, 0.5166666666666667185, 0.5250000000000000222, 0.5333333333333333259, 0.5416666666666666297, 0.5500000000000000444, 0.5583333333333333481, 0.5666666666666666519, 0.5749999999999999556, 0.5833333333333333703, 0.5916666666666666741, 0.5999999999999999778, 0.6083333333333332815, 0.6166666666666666963, 0.6250000000000000000, 0.6333333333333333037, 0.6416666666666667185, 0.6500000000000000222, 0.6583333333333333259, 0.6666666666666666297, 0.6750000000000000444, 0.6833333333333333481, 0.6916666666666666519, 0.6999999999999999556, 0.7083333333333333703, 0.7166666666666666741, 0.7249999999999999778, 0.7333333333333332815, 0.7416666666666666963, 0.7500000000000000000, 0.7583333333333333037, 0.7666666666666667185, 0.7750000000000000222, 0.7833333333333333259, 0.7916666666666666297, 0.8000000000000000444, 0.8083333333333333481, 0.8166666666666666519, 0.8249999999999999556, 0.8333333333333333703, 0.8416666666666666741, 0.8499999999999999778, 0.8583333333333332815, 0.8666666666666666963, 0.8750000000000000000, 0.8833333333333333037, 0.8916666666666667185, 0.9000000000000000222, 0.9083333333333333259, 0.9166666666666666297, 0.9250000000000000444, 0.9333333333333333481, 0.9416666666666666519, 0.9499999999999999556, 0.9583333333333333703, 0.9666666666666666741, 0.9749999999999999778, 0.9833333333333332815, 0.9916666666666666963, 1.000000000000000000 ),
 .UNSPECIFIED. ) 
 GEOMETRIC_REPRESENTATION_ITEM ( )  RATIONAL_B_SPLINE_SURFACE ( (
 ( 1.000000000000000000, 0.8660254037844387076, 1.000000000000000000, 0.8660254037844387076, 1.000000000000000000, 0.8660254037844387076, 1.000000000000000000, 0.8660254037844387076, 1.000000000000000000, 0.8660254037844387076, 1.000000000000000000, 0.8660254037844387076, 1.000000000000000000, 0.8660254037844387076, 1.000000000000000000, 0.8660254037844387076, 1.000000000000000000, 0.8660254037844387076, 1.000000000000000000, 0.8660254037844387076, 1.000000000000000000, 0.8660254037844387076, 1.000000000000000000, 0.8660254037844387076, 1.000000000000000000, 0.8660254037844387076, 1.000000000000000000, 0.8660254037844387076, 1.000000000000000000, 0.8660254037844387076, 1.000000000000000000, 0.8660254037844387076, 1.000000000000000000, 0.8660254037844387076, 1.000000000000000000, 0.8660254037844387076, 1.000000000000000000, 0.8660254037844387076, 1.000000000000000000, 0.8660254037844387076, 1.000000000000000000, 0.8660254037844387076, 1.000000000000000000, 0.8660254037844387076, 1.000000000000000000, 0.8660254037844387076, 1.000000000000000000, 0.8660254037844387076, 1.000000000000000000, 0.8660254037844387076, 1.000000000000000000, 0.8660254037844387076, 1.000000000000000000, 0.8660254037844387076, 1.000000000000000000, 0.8660254037844387076, 1.000000000000000000, 0.8660254037844387076, 1.000000000000000000, 0.8660254037844387076, 1.000000000000000000, 0.8660254037844387076, 1.000000000000000000, 0.8660254037844387076, 1.000000000000000000, 0.8660254037844387076, 1.000000000000000000, 0.8660254037844387076, 1.000000000000000000, 0.8660254037844387076, 1.000000000000000000, 0.8660254037844387076, 1.000000000000000000, 0.8660254037844387076, 1.000000000000000000, 0.8660254037844387076, 1.000000000000000000, 0.8660254037844387076, 1.000000000000000000, 0.8660254037844387076, 1.000000000000000000, 0.8660254037844387076, 1.000000000000000000, 0.8660254037844387076, 1.000000000000000000, 0.8660254037844387076, 1.000000000000000000, 0.8660254037844387076, 1.000000000000000000, 0.8660254037844387076, 1.000000000000000000, 0.8660254037844387076, 1.000000000000000000, 0.8660254037844387076, 1.000000000000000000, 0.8660254037844387076, 1.000000000000000000, 0.8660254037844387076, 1.000000000000000000, 0.8660254037844387076, 1.000000000000000000, 0.8660254037844387076, 1.000000000000000000, 0.8660254037844387076, 1.000000000000000000, 0.8660254037844387076, 1.000000000000000000, 0.8660254037844387076, 1.000000000000000000, 0.8660254037844387076, 1.000000000000000000, 0.8660254037844387076, 1.000000000000000000, 0.8660254037844387076, 1.000000000000000000, 0.8660254037844387076, 1.000000000000000000, 0.8660254037844387076, 1.000000000000000000, 0.8660254037844387076, 1.000000000000000000, 0.8660254037844387076, 1.000000000000000000, 0.8660254037844387076, 1.000000000000000000, 0.8660254037844387076, 1.000000000000000000, 0.8660254037844387076, 1.000000000000000000, 0.8660254037844387076, 1.000000000000000000, 0.8660254037844387076, 1.000000000000000000, 0.8660254037844387076, 1.000000000000000000, 0.8660254037844387076, 1.000000000000000000, 0.8660254037844387076, 1.000000000000000000, 0.8660254037844387076, 1.000000000000000000, 0.8660254037844387076, 1.000000000000000000, 0.8660254037844387076, 1.000000000000000000, 0.8660254037844387076, 1.000000000000000000, 0.8660254037844387076, 1.000000000000000000, 0.8660254037844387076, 1.000000000000000000, 0.8660254037844387076, 1.000000000000000000, 0.8660254037844387076, 1.000000000000000000, 0.8660254037844387076, 1.000000000000000000, 0.8660254037844387076, 1.000000000000000000, 0.8660254037844387076, 1.000000000000000000, 0.8660254037844387076, 1.000000000000000000, 0.8660254037844387076, 1.000000000000000000, 0.8660254037844387076, 1.000000000000000000, 0.8660254037844387076, 1.000000000000000000, 0.8660254037844387076, 1.000000000000000000, 0.8660254037844387076, 1.000000000000000000, 0.8660254037844387076, 1.000000000000000000, 0.8660254037844387076, 1.000000000000000000, 0.8660254037844387076, 1.000000000000000000, 0.8660254037844387076, 1.000000000000000000, 0.8660254037844387076, 1.000000000000000000, 0.8660254037844387076, 1.000000000000000000, 0.8660254037844387076, 1.000000000000000000, 0.8660254037844387076, 1.000000000000000000, 0.8660254037844387076, 1.000000000000000000, 0.8660254037844387076, 1.000000000000000000, 0.8660254037844387076, 1.000000000000000000, 0.8660254037844387076, 1.000000000000000000, 0.8660254037844387076, 1.000000000000000000, 0.8660254037844387076, 1.000000000000000000, 0.8660254037844387076, 1.000000000000000000, 0.8660254037844387076, 1.000000000000000000, 0.8660254037844387076, 1.000000000000000000, 0.8660254037844387076, 1.000000000000000000, 0.8660254037844387076, 1.000000000000000000, 0.8660254037844387076, 1.000000000000000000, 0.8660254037844387076, 1.000000000000000000, 0.8660254037844387076, 1.000000000000000000, 0.8660254037844387076, 1.000000000000000000, 0.8660254037844387076, 1.000000000000000000, 0.8660254037844387076, 1.000000000000000000, 0.8660254037844387076, 1.000000000000000000, 0.8660254037844387076, 1.000000000000000000, 0.8660254037844387076, 1.000000000000000000, 0.8660254037844387076, 1.000000000000000000, 0.8660254037844387076, 1.000000000000000000, 0.8660254037844387076, 1.000000000000000000, 0.8660254037844387076, 1.000000000000000000, 0.8660254037844387076, 1.000000000000000000, 0.8660254037844387076, 1.000000000000000000),
 ( 1.000000000000000000, 0.8660254037844387076, 1.000000000000000000, 0.8660254037844387076, 1.000000000000000000, 0.8660254037844387076, 1.000000000000000000, 0.8660254037844387076, 1.000000000000000000, 0.8660254037844387076, 1.000000000000000000, 0.8660254037844387076, 1.000000000000000000, 0.8660254037844387076, 1.000000000000000000, 0.8660254037844387076, 1.000000000000000000, 0.8660254037844387076, 1.000000000000000000, 0.8660254037844387076, 1.000000000000000000, 0.8660254037844387076, 1.000000000000000000, 0.8660254037844387076, 1.000000000000000000, 0.8660254037844387076, 1.000000000000000000, 0.8660254037844387076, 1.000000000000000000, 0.8660254037844387076, 1.000000000000000000, 0.8660254037844387076, 1.000000000000000000, 0.8660254037844387076, 1.000000000000000000, 0.8660254037844387076, 1.000000000000000000, 0.8660254037844387076, 1.000000000000000000, 0.8660254037844387076, 1.000000000000000000, 0.8660254037844387076, 1.000000000000000000, 0.8660254037844387076, 1.000000000000000000, 0.8660254037844387076, 1.000000000000000000, 0.8660254037844387076, 1.000000000000000000, 0.8660254037844387076, 1.000000000000000000, 0.8660254037844387076, 1.000000000000000000, 0.8660254037844387076, 1.000000000000000000, 0.8660254037844387076, 1.000000000000000000, 0.8660254037844387076, 1.000000000000000000, 0.8660254037844387076, 1.000000000000000000, 0.8660254037844387076, 1.000000000000000000, 0.8660254037844387076, 1.000000000000000000, 0.8660254037844387076, 1.000000000000000000, 0.8660254037844387076, 1.000000000000000000, 0.8660254037844387076, 1.000000000000000000, 0.8660254037844387076, 1.000000000000000000, 0.8660254037844387076, 1.000000000000000000, 0.8660254037844387076, 1.000000000000000000, 0.8660254037844387076, 1.000000000000000000, 0.8660254037844387076, 1.000000000000000000, 0.8660254037844387076, 1.000000000000000000, 0.8660254037844387076, 1.000000000000000000, 0.8660254037844387076, 1.000000000000000000, 0.8660254037844387076, 1.000000000000000000, 0.8660254037844387076, 1.000000000000000000, 0.8660254037844387076, 1.000000000000000000, 0.8660254037844387076, 1.000000000000000000, 0.8660254037844387076, 1.000000000000000000, 0.8660254037844387076, 1.000000000000000000, 0.8660254037844387076, 1.000000000000000000, 0.8660254037844387076, 1.000000000000000000, 0.8660254037844387076, 1.000000000000000000, 0.8660254037844387076, 1.000000000000000000, 0.8660254037844387076, 1.000000000000000000, 0.8660254037844387076, 1.000000000000000000, 0.8660254037844387076, 1.000000000000000000, 0.8660254037844387076, 1.000000000000000000, 0.8660254037844387076, 1.000000000000000000, 0.8660254037844387076, 1.000000000000000000, 0.8660254037844387076, 1.000000000000000000, 0.8660254037844387076, 1.000000000000000000, 0.8660254037844387076, 1.000000000000000000, 0.8660254037844387076, 1.000000000000000000, 0.8660254037844387076, 1.000000000000000000, 0.8660254037844387076, 1.000000000000000000, 0.8660254037844387076, 1.000000000000000000, 0.8660254037844387076, 1.000000000000000000, 0.8660254037844387076, 1.000000000000000000, 0.8660254037844387076, 1.000000000000000000, 0.8660254037844387076, 1.000000000000000000, 0.8660254037844387076, 1.000000000000000000, 0.8660254037844387076, 1.000000000000000000, 0.8660254037844387076, 1.000000000000000000, 0.8660254037844387076, 1.000000000000000000, 0.8660254037844387076, 1.000000000000000000, 0.8660254037844387076, 1.000000000000000000, 0.8660254037844387076, 1.000000000000000000, 0.8660254037844387076, 1.000000000000000000, 0.8660254037844387076, 1.000000000000000000, 0.8660254037844387076, 1.000000000000000000, 0.8660254037844387076, 1.000000000000000000, 0.8660254037844387076, 1.000000000000000000, 0.8660254037844387076, 1.000000000000000000, 0.8660254037844387076, 1.000000000000000000, 0.8660254037844387076, 1.000000000000000000, 0.8660254037844387076, 1.000000000000000000, 0.8660254037844387076, 1.000000000000000000, 0.8660254037844387076, 1.000000000000000000, 0.8660254037844387076, 1.000000000000000000, 0.8660254037844387076, 1.000000000000000000, 0.8660254037844387076, 1.000000000000000000, 0.8660254037844387076, 1.000000000000000000, 0.8660254037844387076, 1.000000000000000000, 0.8660254037844387076, 1.000000000000000000, 0.8660254037844387076, 1.000000000000000000, 0.8660254037844387076, 1.000000000000000000, 0.8660254037844387076, 1.000000000000000000, 0.8660254037844387076, 1.000000000000000000, 0.8660254037844387076, 1.000000000000000000, 0.8660254037844387076, 1.000000000000000000, 0.8660254037844387076, 1.000000000000000000, 0.8660254037844387076, 1.000000000000000000, 0.8660254037844387076, 1.000000000000000000, 0.8660254037844387076, 1.000000000000000000, 0.8660254037844387076, 1.000000000000000000, 0.8660254037844387076, 1.000000000000000000, 0.8660254037844387076, 1.000000000000000000, 0.8660254037844387076, 1.000000000000000000, 0.8660254037844387076, 1.000000000000000000, 0.8660254037844387076, 1.000000000000000000, 0.8660254037844387076, 1.000000000000000000, 0.8660254037844387076, 1.000000000000000000, 0.8660254037844387076, 1.000000000000000000, 0.8660254037844387076, 1.000000000000000000, 0.8660254037844387076, 1.000000000000000000, 0.8660254037844387076, 1.000000000000000000, 0.8660254037844387076, 1.000000000000000000, 0.8660254037844387076, 1.000000000000000000, 0.8660254037844387076, 1.000000000000000000, 0.8660254037844387076, 1.000000000000000000) ) ) 
 REPRESENTATION_ITEM ( '' )  SURFACE ( )  );
#175713=CARTESIAN_POINT ( 'NONE',  ( -7.282664789195997912, 8.525472337930658284, 1.199719254218452047 ) ) ;
#175719=EDGE_LOOP ( 'NONE', ( #117527, #91670, #145129, #13730 ) ) ;
#175720=CARTESIAN_POINT ( 'NONE',  ( -5.743814354044916470, 6.730146830254374990, -1.199719254218453823 ) ) ;
#175729=CARTESIAN_POINT ( 'NONE',  ( -6.154475385960665790, 6.144919136567696505, 0.000000000000000000 ) ) ;
#175732=CARTESIAN_POINT ( 'NONE',  ( 6.212391540903618115, 7.031971956796816414, -1.022972206104319826 ) ) ;
#175737=CARTESIAN_POINT ( 'NONE',  ( 7.042534447655770080, 7.180988041878682004, -0.7998128361456341429 ) ) ;
#175741=EDGE_CURVE ( 'NONE', #105328, #104090, #51943, .T. ) ;
#175744=CARTESIAN_POINT ( 'NONE',  ( -6.064239847062411926, 10.29697326487330500, 0.000000000000000000 ) ) ;
#175751=CARTESIAN_POINT ( 'NONE',  ( -4.111865726694519552, 8.019203457777400956, 0.000000000000000000 ) ) ;
#175755=CARTESIAN_POINT ( 'NONE',  ( 5.600926855776875435, 7.627776979863398310, -1.443375672974078761 ) ) ;
#175756=CARTESIAN_POINT ( 'NONE',  ( -5.926322542504872892, 8.007405281046052536, -1.443375672974066548 ) ) ;
#175760=CARTESIAN_POINT ( 'NONE',  ( -4.261005416444848315, 8.193199762486115034, 0.7998128361456350310 ) ) ;
#175764=CARTESIAN_POINT ( 'NONE',  ( 4.041212305325117882, 6.872442235258051646, -1.199719254218448494 ) ) ;
#175793=CARTESIAN_POINT ( 'NONE',  ( 4.702859892337409420, 8.240897811179339172, 0.6291740908887258898 ) ) ;
#175801=CARTESIAN_POINT ( 'NONE',  ( 5.722423353419669567, 8.833855124701747386, 1.199719254218451159 ) ) ;
#175806=CARTESIAN_POINT ( 'NONE',  ( -4.607477032339801326, 8.379641378740778634, 0.1280868206084313787 ) ) ;
#175813=CARTESIAN_POINT ( 'NONE',  ( -6.688968683495758683, 8.897159112202094988, -1.599625672291271394 ) ) ;
#175826=CARTESIAN_POINT ( 'NONE',  ( 6.013923656113508542, 9.173938811177871244, -1.199719254218452047 ) ) ;
#175830=EDGE_CURVE ( 'NONE', #105777, #118869, #110201, .T. ) ;
#175835=ORIENTED_EDGE ( 'NONE', *, *, #104398, .T. ) ;
#175837=CARTESIAN_POINT ( 'NONE',  ( 3.203469434578891661, 6.959407783642502565, -0.7998128361456362523 ) ) ;
#175839=CARTESIAN_POINT ( 'NONE',  ( 4.706088717274885092, 8.504537580213796133, 0.7216878364870317197 ) ) ;
#175846=CARTESIAN_POINT ( 'NONE',  ( 0.000000000000000000, 2.999999999999999112, -2.500000000000000444 ) ) ;
#175847=CARTESIAN_POINT ( 'NONE',  ( -6.435690514315323796, 6.800136771869164320, 0.4354173353855045336 ) ) ;
#175855=CARTESIAN_POINT ( 'NONE',  ( -5.496904935697871863, 5.377753611261092637, 0.7998128361456281477 ) ) ;
#175856=CARTESIAN_POINT ( 'NONE',  ( 6.034787771858531435, 10.05468647722803865, 0.000000000000000000 ) ) ;
#175863=VERTEX_POINT ( 'NONE', #59515 ) ;
#175869=CARTESIAN_POINT ( 'NONE',  ( -5.936491157937300756, 8.019268665717216749, 1.599625672291263179 ) ) ;
#175870=CARTESIAN_POINT ( 'NONE',  ( -4.447956913735107598, 7.346977611736363656, 1.199719254218452935 ) ) ;
#175872=CARTESIAN_POINT ( 'NONE',  ( 6.902509602688803980, 9.146290184594002781, -1.443375672974064550 ) ) ;
#175883=CARTESIAN_POINT ( 'NONE',  ( -5.670379370357061077, 7.341873695786736320, -1.227147999111227294 ) ) ;
#175887=CARTESIAN_POINT ( 'NONE',  ( 6.211043768836185031, 6.418841616496599123, 0.7216878364870328300 ) ) ;
#175892=CARTESIAN_POINT ( 'NONE',  ( -7.144220599758281054, 7.299621885998258897, 0.7998128361456341429 ) ) ;
#175908=CARTESIAN_POINT ( 'NONE',  ( 6.703580607314123085, 6.785541894813420072, 0.000000000000000000 ) ) ;
#175940=CARTESIAN_POINT ( 'NONE',  ( 7.241463443474815520, 8.581367117876336437, -1.082531754730548412 ) ) ;
#175964=( BOUNDED_SURFACE ( )  B_SPLINE_SURFACE ( 1, 2, ( 
 ( #102881, #167877, #98625, #85552, #148444, #14, #66078, #132219, #34669, #151642, #185172, #198229, #3211, #20541, #86625, #69279, #152692, #131187, #100739, #49865, #115991, #99682, #165751, #83419, #103954, #40018, #206761, #89849, #58393, #25875, #23744, #108279, #189455, #88775, #8564, #154833, #124549, #123491, #190507, #155899, #55196, #172152, #7486, #6417, #73568, #171067, #120268, #169997, #56264, #139670, #136461, #140750, #72489, #173229, #187318, #138590, #202480, #105029, #90910, #186243, #204613, #91985, #70344, #205692, #174300, #122423, #37878, #54133, #188380, #21584, #121343, #87689, #106129, #42164, #57327, #158044, #153764, #41096, #5332, #107206, #24809, #74645, #156975, #71415, #137527, #203542, #38946, #22664, #111473, #29093, #28019, #161226, #110410, #59453, #43233, #209946, #177478, #75707, #79959, #11756, #112532, #126672, #160158, #141822, #44288, #30154, #125610, #94117, #179608, #9630, #192635, #46415, #113604, #77830, #176413, #109350, #97303, #31229, #191569, #146062, #143951, #162293, #128796, #78886, #61585, #195855, #175360, #212075, #211015, #127754, #193711, #63714, #129872, #207824, #12813, #95177, #26941, #93048, #47495, #159089, #10687, #194778, #76757, #142879, #208881, #13880, #60511, #45354, #145009, #62638, #178544, #96242, #35472, #32287, #213146, #131956, #133018, #130917, #118934, #100477, #83151, #34405, #149230, #66873, #199017, #214181, #19218, #197966, #49597, #150317, #36538, #64776, #165477, #50664, #196910, #135140, #200096, #147120, #117868, #14938, #48550, #81033, #114668, #805, #183859, #85296, #180662, #182787, #167619, #151382, #116790, #98353, #164418, #99423, #101550, #51745, #115721, #16002, #82087, #52795, #2952, #69023, #181712, #17073, #33341, #166553, #201156, #18141, #148180, #65809, #84229, #1883, #67943, #134088, #184914, #163362, #5080, #4018, #103697, #104769, #190255, #153511, #170818, #56007, #22409, #88518, #189202, #90657, #168681, #138333, #171888, #20285, #154580, #7225, #23485, #106948, #122159, #102625, #6157, #72226, #187058 ),
 ( #139403, #86370, #57073, #152439, #70087, #136202, #53874, #204349, #123237, #172971, #202220, #188126, #24550, #156719, #39757, #89592, #140496, #105862, #120007, #185983, #155641, #37617, #71155, #169748, #73301, #8310, #205437, #74395, #58137, #40839, #206506, #124296, #121091, #21336, #38691, #87442, #137272, #203292, #54939, #26696, #143705, #61341, #60264, #193471, #142622, #91735, #75455, #27770, #209697, #108024, #112289, #44039, #144767, #158842, #192385, #174050, #76511, #62400, #157788, #126421, #211833, #41913, #10439, #78641, #145828, #110158, #208631, #141568, #129625, #63470, #25623, #176170, #160978, #29914, #128563, #159904, #92797, #28841, #93866, #125352, #207576, #11511, #194528, #210777, #77582, #9384, #59196, #191315, #46175, #95996, #127500, #45115, #111225, #177228, #178305, #94929, #42983, #109093, #175109, #12569, #162050, #13640, #79712, #81845, #98124, #97063, #196668, #197715, #71707, #32037, #49357, #151927, #115476, #184402, #70636, #186543, #47247, #19769, #53349, #113361, #36022, #103170, #119483, #202774, #3501, #195610, #102100, #168170, #65565, #136747, #179366, #85851, #131712, #48308, #64535, #54425, #21879, #147928, #164175, #69571, #4561, #152987, #213944, #104245, #135681, #130679, #86919, #30988, #114419, #120566, #163116, #146882, #212902, #14698, #87985, #185470, #170291, #80792, #37092, #15760, #169232, #201705, #180419, #154060, #20822, #38173, #5626, #138888, #124834, #92289, #139965, #157269, #73871, #41393, #109648, #105326, #108569, #171363, #43525, #8859, #22957, #40317, #39234, #6711, #42460, #107504, #173532, #91207, #74938, #89072, #93345, #158333, #188682, #190800, #187607, #9927, #57624, #141049, #205988, #76001, #26173, #90136, #155129, #72787, #27238, #142106, #125907, #106423, #123782, #156203, #25105, #174596, #207055, #204907, #55485, #56560, #203839, #122719, #24033, #172446, #7779, #189741, #58686, #208119, #59747, #10980, #191864, #175651, #159381, #137820, #121639, #163661, #65058, #143184, #112835, #146362, #209175, #145314, #196156, #212376, #81330 ) ),
 .UNSPECIFIED., .F., .F., .T. ) 
 B_SPLINE_SURFACE_WITH_KNOTS ( ( 2, 2 ),
 ( 3, 2, 2, 2, 2, 2, 2, 2, 2, 2, 2, 2, 2, 2, 2, 2, 2, 2, 2, 2, 2, 2, 2, 2, 2, 2, 2, 2, 2, 2, 2, 2, 2, 2, 2, 2, 2, 2, 2, 2, 2, 2, 2, 2, 2, 2, 2, 2, 2, 2, 2, 2, 2, 2, 2, 2, 2, 2, 2, 2, 2, 2, 2, 2, 2, 2, 2, 2, 2, 2, 2, 2, 2, 2, 2, 2, 2, 2, 2, 2, 2, 2, 2, 2, 2, 2, 2, 2, 2, 2, 2, 2, 2, 2, 2, 2, 2, 2, 2, 2, 2, 2, 2, 2, 2, 2, 2, 2, 2, 2, 2, 2, 2, 2, 2, 2, 2, 2, 2, 2, 3 ),
 ( 0.000000000000000000, 1.000000000000000000 ),
 ( 0.000000000000000000, 0.008333333333333333218, 0.01666666666666666644, 0.02500000000000000139, 0.03333333333333333287, 0.04166666666666666435, 0.05000000000000000278, 0.05833333333333333426, 0.06666666666666666574, 0.07499999999999999722, 0.08333333333333332871, 0.09166666666666666019, 0.1000000000000000056, 0.1083333333333333370, 0.1166666666666666685, 0.1250000000000000000, 0.1333333333333333315, 0.1416666666666666630, 0.1499999999999999944, 0.1583333333333333259, 0.1666666666666666574, 0.1749999999999999889, 0.1833333333333333204, 0.1916666666666666796, 0.2000000000000000111, 0.2083333333333333426, 0.2166666666666666741, 0.2250000000000000056, 0.2333333333333333370, 0.2416666666666666685, 0.2500000000000000000, 0.2583333333333333592, 0.2666666666666666630, 0.2750000000000000222, 0.2833333333333333259, 0.2916666666666666852, 0.2999999999999999889, 0.3083333333333333481, 0.3166666666666666519, 0.3250000000000000111, 0.3333333333333333148, 0.3416666666666666741, 0.3499999999999999778, 0.3583333333333333370, 0.3666666666666666408, 0.3750000000000000000, 0.3833333333333333592, 0.3916666666666666630, 0.4000000000000000222, 0.4083333333333333259, 0.4166666666666666852, 0.4249999999999999889, 0.4333333333333333481, 0.4416666666666666519, 0.4500000000000000111, 0.4583333333333333148, 0.4666666666666666741, 0.4749999999999999778, 0.4833333333333333370, 0.4916666666666666408, 0.5000000000000000000, 0.5083333333333333037, 0.5166666666666667185, 0.5250000000000000222, 0.5333333333333333259, 0.5416666666666666297, 0.5500000000000000444, 0.5583333333333333481, 0.5666666666666666519, 0.5749999999999999556, 0.5833333333333333703, 0.5916666666666666741, 0.5999999999999999778, 0.6083333333333332815, 0.6166666666666666963, 0.6250000000000000000, 0.6333333333333333037, 0.6416666666666667185, 0.6500000000000000222, 0.6583333333333333259, 0.6666666666666666297, 0.6750000000000000444, 0.6833333333333333481, 0.6916666666666666519, 0.6999999999999999556, 0.7083333333333333703, 0.7166666666666666741, 0.7249999999999999778, 0.7333333333333332815, 0.7416666666666666963, 0.7500000000000000000, 0.7583333333333333037, 0.7666666666666667185, 0.7750000000000000222, 0.7833333333333333259, 0.7916666666666666297, 0.8000000000000000444, 0.8083333333333333481, 0.8166666666666666519, 0.8249999999999999556, 0.8333333333333333703, 0.8416666666666666741, 0.8499999999999999778, 0.8583333333333332815, 0.8666666666666666963, 0.8750000000000000000, 0.8833333333333333037, 0.8916666666666667185, 0.9000000000000000222, 0.9083333333333333259, 0.9166666666666666297, 0.9250000000000000444, 0.9333333333333333481, 0.9416666666666666519, 0.9499999999999999556, 0.9583333333333333703, 0.9666666666666666741, 0.9749999999999999778, 0.9833333333333332815, 0.9916666666666666963, 1.000000000000000000 ),
 .UNSPECIFIED. ) 
 GEOMETRIC_REPRESENTATION_ITEM ( )  RATIONAL_B_SPLINE_SURFACE ( (
 ( 1.000000000000000000, 0.8660254037844387076, 1.000000000000000000, 0.8660254037844387076, 1.000000000000000000, 0.8660254037844387076, 1.000000000000000000, 0.8660254037844387076, 1.000000000000000000, 0.8660254037844387076, 1.000000000000000000, 0.8660254037844387076, 1.000000000000000000, 0.8660254037844387076, 1.000000000000000000, 0.8660254037844387076, 1.000000000000000000, 0.8660254037844387076, 1.000000000000000000, 0.8660254037844387076, 1.000000000000000000, 0.8660254037844387076, 1.000000000000000000, 0.8660254037844387076, 1.000000000000000000, 0.8660254037844387076, 1.000000000000000000, 0.8660254037844387076, 1.000000000000000000, 0.8660254037844387076, 1.000000000000000000, 0.8660254037844387076, 1.000000000000000000, 0.8660254037844387076, 1.000000000000000000, 0.8660254037844387076, 1.000000000000000000, 0.8660254037844387076, 1.000000000000000000, 0.8660254037844387076, 1.000000000000000000, 0.8660254037844387076, 1.000000000000000000, 0.8660254037844387076, 1.000000000000000000, 0.8660254037844387076, 1.000000000000000000, 0.8660254037844387076, 1.000000000000000000, 0.8660254037844387076, 1.000000000000000000, 0.8660254037844387076, 1.000000000000000000, 0.8660254037844387076, 1.000000000000000000, 0.8660254037844387076, 1.000000000000000000, 0.8660254037844387076, 1.000000000000000000, 0.8660254037844387076, 1.000000000000000000, 0.8660254037844387076, 1.000000000000000000, 0.8660254037844387076, 1.000000000000000000, 0.8660254037844387076, 1.000000000000000000, 0.8660254037844387076, 1.000000000000000000, 0.8660254037844387076, 1.000000000000000000, 0.8660254037844387076, 1.000000000000000000, 0.8660254037844387076, 1.000000000000000000, 0.8660254037844387076, 1.000000000000000000, 0.8660254037844387076, 1.000000000000000000, 0.8660254037844387076, 1.000000000000000000, 0.8660254037844387076, 1.000000000000000000, 0.8660254037844387076, 1.000000000000000000, 0.8660254037844387076, 1.000000000000000000, 0.8660254037844387076, 1.000000000000000000, 0.8660254037844387076, 1.000000000000000000, 0.8660254037844387076, 1.000000000000000000, 0.8660254037844387076, 1.000000000000000000, 0.8660254037844387076, 1.000000000000000000, 0.8660254037844387076, 1.000000000000000000, 0.8660254037844387076, 1.000000000000000000, 0.8660254037844387076, 1.000000000000000000, 0.8660254037844387076, 1.000000000000000000, 0.8660254037844387076, 1.000000000000000000, 0.8660254037844387076, 1.000000000000000000, 0.8660254037844387076, 1.000000000000000000, 0.8660254037844387076, 1.000000000000000000, 0.8660254037844387076, 1.000000000000000000, 0.8660254037844387076, 1.000000000000000000, 0.8660254037844387076, 1.000000000000000000, 0.8660254037844387076, 1.000000000000000000, 0.8660254037844387076, 1.000000000000000000, 0.8660254037844387076, 1.000000000000000000, 0.8660254037844387076, 1.000000000000000000, 0.8660254037844387076, 1.000000000000000000, 0.8660254037844387076, 1.000000000000000000, 0.8660254037844387076, 1.000000000000000000, 0.8660254037844387076, 1.000000000000000000, 0.8660254037844387076, 1.000000000000000000, 0.8660254037844387076, 1.000000000000000000, 0.8660254037844387076, 1.000000000000000000, 0.8660254037844387076, 1.000000000000000000, 0.8660254037844387076, 1.000000000000000000, 0.8660254037844387076, 1.000000000000000000, 0.8660254037844387076, 1.000000000000000000, 0.8660254037844387076, 1.000000000000000000, 0.8660254037844387076, 1.000000000000000000, 0.8660254037844387076, 1.000000000000000000, 0.8660254037844387076, 1.000000000000000000, 0.8660254037844387076, 1.000000000000000000, 0.8660254037844387076, 1.000000000000000000, 0.8660254037844387076, 1.000000000000000000, 0.8660254037844387076, 1.000000000000000000, 0.8660254037844387076, 1.000000000000000000, 0.8660254037844387076, 1.000000000000000000, 0.8660254037844387076, 1.000000000000000000, 0.8660254037844387076, 1.000000000000000000, 0.8660254037844387076, 1.000000000000000000, 0.8660254037844387076, 1.000000000000000000, 0.8660254037844387076, 1.000000000000000000, 0.8660254037844387076, 1.000000000000000000, 0.8660254037844387076, 1.000000000000000000, 0.8660254037844387076, 1.000000000000000000, 0.8660254037844387076, 1.000000000000000000, 0.8660254037844387076, 1.000000000000000000, 0.8660254037844387076, 1.000000000000000000, 0.8660254037844387076, 1.000000000000000000, 0.8660254037844387076, 1.000000000000000000, 0.8660254037844387076, 1.000000000000000000, 0.8660254037844387076, 1.000000000000000000, 0.8660254037844387076, 1.000000000000000000, 0.8660254037844387076, 1.000000000000000000, 0.8660254037844387076, 1.000000000000000000, 0.8660254037844387076, 1.000000000000000000, 0.8660254037844387076, 1.000000000000000000, 0.8660254037844387076, 1.000000000000000000, 0.8660254037844387076, 1.000000000000000000, 0.8660254037844387076, 1.000000000000000000, 0.8660254037844387076, 1.000000000000000000, 0.8660254037844387076, 1.000000000000000000, 0.8660254037844387076, 1.000000000000000000, 0.8660254037844387076, 1.000000000000000000, 0.8660254037844387076, 1.000000000000000000, 0.8660254037844387076, 1.000000000000000000, 0.8660254037844387076, 1.000000000000000000, 0.8660254037844387076, 1.000000000000000000, 0.8660254037844387076, 1.000000000000000000, 0.8660254037844387076, 1.000000000000000000, 0.8660254037844387076, 1.000000000000000000, 0.8660254037844387076, 1.000000000000000000, 0.8660254037844387076, 1.000000000000000000),
 ( 1.000000000000000000, 0.8660254037844387076, 1.000000000000000000, 0.8660254037844387076, 1.000000000000000000, 0.8660254037844387076, 1.000000000000000000, 0.8660254037844387076, 1.000000000000000000, 0.8660254037844387076, 1.000000000000000000, 0.8660254037844387076, 1.000000000000000000, 0.8660254037844387076, 1.000000000000000000, 0.8660254037844387076, 1.000000000000000000, 0.8660254037844387076, 1.000000000000000000, 0.8660254037844387076, 1.000000000000000000, 0.8660254037844387076, 1.000000000000000000, 0.8660254037844387076, 1.000000000000000000, 0.8660254037844387076, 1.000000000000000000, 0.8660254037844387076, 1.000000000000000000, 0.8660254037844387076, 1.000000000000000000, 0.8660254037844387076, 1.000000000000000000, 0.8660254037844387076, 1.000000000000000000, 0.8660254037844387076, 1.000000000000000000, 0.8660254037844387076, 1.000000000000000000, 0.8660254037844387076, 1.000000000000000000, 0.8660254037844387076, 1.000000000000000000, 0.8660254037844387076, 1.000000000000000000, 0.8660254037844387076, 1.000000000000000000, 0.8660254037844387076, 1.000000000000000000, 0.8660254037844387076, 1.000000000000000000, 0.8660254037844387076, 1.000000000000000000, 0.8660254037844387076, 1.000000000000000000, 0.8660254037844387076, 1.000000000000000000, 0.8660254037844387076, 1.000000000000000000, 0.8660254037844387076, 1.000000000000000000, 0.8660254037844387076, 1.000000000000000000, 0.8660254037844387076, 1.000000000000000000, 0.8660254037844387076, 1.000000000000000000, 0.8660254037844387076, 1.000000000000000000, 0.8660254037844387076, 1.000000000000000000, 0.8660254037844387076, 1.000000000000000000, 0.8660254037844387076, 1.000000000000000000, 0.8660254037844387076, 1.000000000000000000, 0.8660254037844387076, 1.000000000000000000, 0.8660254037844387076, 1.000000000000000000, 0.8660254037844387076, 1.000000000000000000, 0.8660254037844387076, 1.000000000000000000, 0.8660254037844387076, 1.000000000000000000, 0.8660254037844387076, 1.000000000000000000, 0.8660254037844387076, 1.000000000000000000, 0.8660254037844387076, 1.000000000000000000, 0.8660254037844387076, 1.000000000000000000, 0.8660254037844387076, 1.000000000000000000, 0.8660254037844387076, 1.000000000000000000, 0.8660254037844387076, 1.000000000000000000, 0.8660254037844387076, 1.000000000000000000, 0.8660254037844387076, 1.000000000000000000, 0.8660254037844387076, 1.000000000000000000, 0.8660254037844387076, 1.000000000000000000, 0.8660254037844387076, 1.000000000000000000, 0.8660254037844387076, 1.000000000000000000, 0.8660254037844387076, 1.000000000000000000, 0.8660254037844387076, 1.000000000000000000, 0.8660254037844387076, 1.000000000000000000, 0.8660254037844387076, 1.000000000000000000, 0.8660254037844387076, 1.000000000000000000, 0.8660254037844387076, 1.000000000000000000, 0.8660254037844387076, 1.000000000000000000, 0.8660254037844387076, 1.000000000000000000, 0.8660254037844387076, 1.000000000000000000, 0.8660254037844387076, 1.000000000000000000, 0.8660254037844387076, 1.000000000000000000, 0.8660254037844387076, 1.000000000000000000, 0.8660254037844387076, 1.000000000000000000, 0.8660254037844387076, 1.000000000000000000, 0.8660254037844387076, 1.000000000000000000, 0.8660254037844387076, 1.000000000000000000, 0.8660254037844387076, 1.000000000000000000, 0.8660254037844387076, 1.000000000000000000, 0.8660254037844387076, 1.000000000000000000, 0.8660254037844387076, 1.000000000000000000, 0.8660254037844387076, 1.000000000000000000, 0.8660254037844387076, 1.000000000000000000, 0.8660254037844387076, 1.000000000000000000, 0.8660254037844387076, 1.000000000000000000, 0.8660254037844387076, 1.000000000000000000, 0.8660254037844387076, 1.000000000000000000, 0.8660254037844387076, 1.000000000000000000, 0.8660254037844387076, 1.000000000000000000, 0.8660254037844387076, 1.000000000000000000, 0.8660254037844387076, 1.000000000000000000, 0.8660254037844387076, 1.000000000000000000, 0.8660254037844387076, 1.000000000000000000, 0.8660254037844387076, 1.000000000000000000, 0.8660254037844387076, 1.000000000000000000, 0.8660254037844387076, 1.000000000000000000, 0.8660254037844387076, 1.000000000000000000, 0.8660254037844387076, 1.000000000000000000, 0.8660254037844387076, 1.000000000000000000, 0.8660254037844387076, 1.000000000000000000, 0.8660254037844387076, 1.000000000000000000, 0.8660254037844387076, 1.000000000000000000, 0.8660254037844387076, 1.000000000000000000, 0.8660254037844387076, 1.000000000000000000, 0.8660254037844387076, 1.000000000000000000, 0.8660254037844387076, 1.000000000000000000, 0.8660254037844387076, 1.000000000000000000, 0.8660254037844387076, 1.000000000000000000, 0.8660254037844387076, 1.000000000000000000, 0.8660254037844387076, 1.000000000000000000, 0.8660254037844387076, 1.000000000000000000, 0.8660254037844387076, 1.000000000000000000, 0.8660254037844387076, 1.000000000000000000, 0.8660254037844387076, 1.000000000000000000, 0.8660254037844387076, 1.000000000000000000, 0.8660254037844387076, 1.000000000000000000, 0.8660254037844387076, 1.000000000000000000, 0.8660254037844387076, 1.000000000000000000, 0.8660254037844387076, 1.000000000000000000, 0.8660254037844387076, 1.000000000000000000, 0.8660254037844387076, 1.000000000000000000, 0.8660254037844387076, 1.000000000000000000, 0.8660254037844387076, 1.000000000000000000, 0.8660254037844387076, 1.000000000000000000, 0.8660254037844387076, 1.000000000000000000) ) ) 
 REPRESENTATION_ITEM ( '' )  SURFACE ( )  );
#175971=CARTESIAN_POINT ( 'NONE',  ( -3.630551273409382329, 7.457669928944732796, 0.7998128361456352531 ) ) ;
#175973=CARTESIAN_POINT ( 'NONE',  ( 6.509323147892504657, 6.766834225395614411, 0.000000000000000000 ) ) ;
#175979=CARTESIAN_POINT ( 'NONE',  ( -3.793249116773374396, 7.647484079536056356, 0.7998128361456352531 ) ) ;
#175984=CARTESIAN_POINT ( 'NONE',  ( -3.634467696915153034, 6.397906858779740524, 1.199719254218452935 ) ) ;
#175991=CARTESIAN_POINT ( 'NONE',  ( -4.925354943514475003, 8.968274210734028529, 0.000000000000000000 ) ) ;
#176002=CARTESIAN_POINT ( 'NONE',  ( -4.797606254389363833, 6.690569611577942943, 1.599625672291263179 ) ) ;
#176005=CARTESIAN_POINT ( 'NONE',  ( -5.397554552016258889, 7.390509292142662723, 1.443375672974058777 ) ) ;
#176006=CARTESIAN_POINT ( 'NONE',  ( -5.221298554594238084, 8.145246509451649075, 1.082531754730549967 ) ) ;
#176007=CARTESIAN_POINT ( 'NONE',  ( 6.387826650694035990, 7.481494509678370264, -1.199719254218452047 ) ) ;
#176008=CARTESIAN_POINT ( 'NONE',  ( -5.921879234118920365, 10.13088588310589699, 0.000000000000000000 ) ) ;
#176027=CARTESIAN_POINT ( 'NONE',  ( 5.826972158823246595, 10.02016096192762085, -0.7998128361456481317 ) ) ;
#176046=CARTESIAN_POINT ( 'NONE',  ( 4.595841027163160675, 8.489102040997540399, 0.04885061651019838302 ) ) ;
#176059=EDGE_CURVE ( 'NONE', #26620, #7055, #11411, .T. ) ;
#176060=CARTESIAN_POINT ( 'NONE',  ( 5.365994935958575240, 9.482354201918870018, 0.7998128361456341429 ) ) ;
#176063=CARTESIAN_POINT ( 'NONE',  ( -3.383641855062333281, 6.105276709951447778, -1.199719254218452047 ) ) ;
#176066=CARTESIAN_POINT ( 'NONE',  ( -5.573810548549546162, 9.516879716700865188, 0.7216878364870267237 ) ) ;
#176077=CARTESIAN_POINT ( 'NONE',  ( 8.154303043976348420, 8.478051404252736845, 0.7998128361456281477 ) ) ;
#176078=CARTESIAN_POINT ( 'NONE',  ( 4.667750024854814050, 8.667735138964429709, -0.7998128361456381397 ) ) ;
#176092=CARTESIAN_POINT ( 'NONE',  ( 4.864343252252968597, 8.897093904262280972, 0.000000000000000000 ) ) ;
#176102=CARTESIAN_POINT ( 'NONE',  ( 0.000000000000000000, 8.999999999999998224, 0.000000000000000000 ) ) ;
#176104=EDGE_CURVE ( 'NONE', #85209, #69840, #198181, .T. ) ;
#176106=CARTESIAN_POINT ( 'NONE',  ( -5.817857314039913241, 5.960124085900898372, 0.000000000000000000 ) ) ;
#176107=CARTESIAN_POINT ( 'NONE',  ( -5.725286006720766707, 9.901527117808042178, 0.7998128361456291469 ) ) ;
#176109=CARTESIAN_POINT ( 'NONE',  ( -4.858589159720606787, 4.879621185664173133, 0.4920435892086290064 ) ) ;
#176120=CARTESIAN_POINT ( 'NONE',  ( 6.200875153403774043, 8.327716660428123419, -1.599625672291283607 ) ) ;
#176123=CARTESIAN_POINT ( 'NONE',  ( 5.519577934094864524, 5.612131475965050242, 0.7216878364870328300 ) ) ;
#176131=CYLINDRICAL_SURFACE ( 'NONE', #78810, 0.08000000000000041800 ) ;
#176142=CARTESIAN_POINT ( 'NONE',  ( 3.562760505341037831, 7.378580699531681830, -1.734723475976807094E-15 ) ) ;
#176144=CARTESIAN_POINT ( 'NONE',  ( -2.993318053567081360, 6.714231172462041819, 0.000000000000000000 ) ) ;
#176147=CARTESIAN_POINT ( 'NONE',  ( 5.682802662783380754, 6.658966523782627434, 1.199719254218452935 ) ) ;
#176157=CARTESIAN_POINT ( 'NONE',  ( 5.234856708652215751, 9.121433570154021453, 0.7216878364870317197 ) ) ;
#176159=CARTESIAN_POINT ( 'NONE',  ( -5.769876891067536206, 8.889217585290882795, 1.199719254218454489 ) ) ;
#176160=CARTESIAN_POINT ( 'NONE',  ( 4.420840606507738357, 7.315341919971147355, 1.199719254218451159 ) ) ;
#176170=CARTESIAN_POINT ( 'NONE',  ( -3.772911886352873445, 7.623757310712140800, 0.7998128361456352531 ) ) ;
#176197=CARTESIAN_POINT ( 'NONE',  ( 4.773879485787624333, 4.742149952939897162, -0.7216878364870357165 ) ) ;
#176203=CARTESIAN_POINT ( 'NONE',  ( 4.543390873910913896, 5.433615786718446472, 1.082531754730549078 ) ) ;
#176214=CARTESIAN_POINT ( 'NONE',  ( -4.468294144155606773, 7.370704380560280100, 1.199719254218452935 ) ) ;
#176216=CARTESIAN_POINT ( 'NONE',  ( -4.762657100150483380, 8.778460060142702304, 0.000000000000000000 ) ) ;
#176218=CARTESIAN_POINT ( 'NONE',  ( 6.821160681006781523, 9.051383109298340557, 1.443375672974063439 ) ) ;
#176227=CARTESIAN_POINT ( 'NONE',  ( -4.925354943514475003, 8.968274210734028529, 0.000000000000000000 ) ) ;
#176235=CARTESIAN_POINT ( 'NONE',  ( -5.668717624289589807, 5.786127781192186958, 0.7216878364870257245 ) ) ;
#176239=CARTESIAN_POINT ( 'NONE',  ( -5.984998465789844069, 5.947196063035064206, 0.7998128361456281477 ) ) ;
#176260=CARTESIAN_POINT ( 'NONE',  ( -5.661411662158206681, 8.762674818229999829, -1.199719254218452047 ) ) ;
#176262=CARTESIAN_POINT ( 'NONE',  ( -3.318713740295064163, 7.093859473644694269, 0.000000000000000000 ) ) ;
#176271=CARTESIAN_POINT ( 'NONE',  ( 4.041739190205284160, 7.729463131965888856, 0.000000000000000000 ) ) ;
#176287=CARTESIAN_POINT ( 'NONE',  ( -5.271087860662956537, 9.371629280740593870, 0.000000000000000000 ) ) ;
#176312=CARTESIAN_POINT ( 'NONE',  ( 8.011942431032855083, 8.311964022485323511, 0.7998128361456291469 ) ) ;
#176314=CARTESIAN_POINT ( 'NONE',  ( 5.806634928402749196, 9.996434193103704402, -0.7998128361456481317 ) ) ;
#176322=CARTESIAN_POINT ( 'NONE',  ( 6.206481105300311718, 7.020237702803970414, -1.025761867992080356 ) ) ;
#176326=CARTESIAN_POINT ( 'NONE',  ( 5.590372323399994237, 7.390087136190794936, 1.241407824010079652 ) ) ;
#176328=CARTESIAN_POINT ( 'NONE',  ( 6.861835142292143530, 8.138467433163244280, 1.082531754730549967 ) ) ;
#176334=CARTESIAN_POINT ( 'NONE',  ( -5.984998465789844069, 5.947196063035064206, 0.7998128361456281477 ) ) ;
#176341=CARTESIAN_POINT ( 'NONE',  ( -5.438229012412888252, 9.358701257874761481, -0.7216878364870338292 ) ) ;
#176345=CARTESIAN_POINT ( 'NONE',  ( 7.075376061485196821, 9.347967719856493218, 1.599625672291268286 ) ) ;
#176351=CARTESIAN_POINT ( 'NONE',  ( -5.144392941742557568, 4.966489618313220333, -0.7998128361456362523 ) ) ;
#176361=CARTESIAN_POINT ( 'NONE',  ( 3.074666975249065626, 6.809138247757705820, 0.000000000000000000 ) ) ;
#176383=CARTESIAN_POINT ( 'NONE',  ( 6.424584688029230328, 8.588711117491191871, 1.599625672291268286 ) ) ;
#176385=CARTESIAN_POINT ( 'NONE',  ( -5.984664909832329904, 7.106694798503815136, 1.079546468792412783 ) ) ;
#176392=CARTESIAN_POINT ( 'NONE',  ( 6.364626766972446781, 6.390095747748157251, 0.7998128361456352531 ) ) ;
#176400=CARTESIAN_POINT ( 'NONE',  ( 4.312902262922978736, 5.164712407232485702, -1.082531754730548412 ) ) ;
#176402=CARTESIAN_POINT ( 'NONE',  ( 5.072158865288233009, 7.010880990960010273, 1.443375672974065660 ) ) ;
#176403=ORIENTED_EDGE ( 'NONE', *, *, #150546, .F. ) ;
#176413=CARTESIAN_POINT ( 'NONE',  ( -6.305950844131887223, 6.529566537674873494, 0.000000000000000000 ) ) ;
#176444=CARTESIAN_POINT ( 'NONE',  ( 3.217027588192558074, 6.975225629525113824, -1.734723475976807094E-15 ) ) ;
#176455=CARTESIAN_POINT ( 'NONE',  ( -5.750066545971566079, 8.762142499391876171, 1.082531754730550855 ) ) ;
#176457=CARTESIAN_POINT ( 'NONE',  ( 5.370438244344566847, 5.438135171256338829, 0.000000000000000000 ) ) ;
#176474=CARTESIAN_POINT ( 'NONE',  ( -3.797692425603673705, 6.484372692295976570, 1.082531754730549967 ) ) ;
#176509=CARTESIAN_POINT ( 'NONE',  ( -7.584860592202423035, 7.813701877183096833, -0.7998128361456362523 ) ) ;
#176510=CARTESIAN_POINT ( 'NONE',  ( -5.370252646843524325, 7.685795487962019834, 1.333085116894404232 ) ) ;
#176511=CARTESIAN_POINT ( 'NONE',  ( -5.387385936583831914, 7.378645907471495846, -1.599625672291271394 ) ) ;
#176518=CARTESIAN_POINT ( 'NONE',  ( -3.383641855062333281, 6.105276709951447778, -1.199719254218452047 ) ) ;
#176522=CARTESIAN_POINT ( 'NONE',  ( -4.197131071882288289, 7.054347462908075350, -1.199719254218455378 ) ) ;
#176536=CARTESIAN_POINT ( 'NONE',  ( 4.817943484809818600, 6.714296380401858499, 1.599625672291269396 ) ) ;
#176559=CARTESIAN_POINT ( 'NONE',  ( 4.016958651398847557, 7.908478536599129249, -0.7998128361456362523 ) ) ;
#176560=CARTESIAN_POINT ( 'NONE',  ( 5.259637247458703868, 5.100941308315409373, 0.000000000000000000 ) ) ;
#176563=CARTESIAN_POINT ( 'NONE',  ( 4.146814880933355596, 5.931313009212638931, 1.599625672291261402 ) ) ;
#176575=CARTESIAN_POINT ( 'NONE',  ( 4.725438941449205288, 8.332574750205820280, 0.7120043264817934592 ) ) ;
#176577=CARTESIAN_POINT ( 'NONE',  ( -4.136646265500964148, 6.879818838842817641, -1.082531754730551743 ) ) ;
#176590=ORIENTED_EDGE ( 'NONE', *, *, #83296, .T. ) ;
#176605=CARTESIAN_POINT ( 'NONE',  ( 5.564695703766185275, 5.456842840674144490, 0.000000000000000000 ) ) ;
#176624=CARTESIAN_POINT ( 'NONE',  ( -6.933015448541747006, 9.181880338089085214, 1.599625672291269396 ) ) ;
#176637=ORIENTED_EDGE ( 'NONE', *, *, #38876, .T. ) ;
#176640=CARTESIAN_POINT ( 'NONE',  ( 5.422335090822693715, 5.290755458906732933, 0.000000000000000000 ) ) ;
#176650=CARTESIAN_POINT ( 'NONE',  ( 4.855733865602142707, 8.067643820953190215, 0.9155131637919884380 ) ) ;
#176663=CARTESIAN_POINT ( 'NONE',  ( -5.983791420057156252, 7.107340751733106643, 1.079986564815892613 ) ) ;
#176668=CARTESIAN_POINT ( 'NONE',  ( -5.818384198920079520, 6.817144982608731141, 1.199719254218452935 ) ) ;
#176670=CARTESIAN_POINT ( 'NONE',  ( 4.899292406491845497, 6.809203455697518947, -1.599625672291273171 ) ) ;
#176674=CARTESIAN_POINT ( 'NONE',  ( -7.075376061485238566, 9.347967719856493218, 1.599625672291269396 ) ) ;
#176677=CARTESIAN_POINT ( 'NONE',  ( 6.556249800660121529, 9.806652646482286073, 1.199719254218452047 ) ) ;
#176678=CARTESIAN_POINT ( 'NONE',  ( -3.719872605471121751, 6.605953636083950364, -2.419999999999998597 ) ) ;
#176682=CARTESIAN_POINT ( 'NONE',  ( -5.203215198707511036, 7.836405505866204102, -1.276579466623083858 ) ) ;
#176689=EDGE_CURVE ( 'NONE', #185175, #105328, #176926, .T. ) ;
#176695=EDGE_LOOP ( 'NONE', ( #179990, #37574, #23084, #117762, #31181, #212857, #87815, #127985, #94526, #174561, #211825, #49831, #114635, #204195, #19974, #89183, #141879 ) ) ;
#176699=CARTESIAN_POINT ( 'NONE',  ( 4.421367491832268293, 7.211993602896056288, 1.082531754730549078 ) ) ;
#176704=VERTEX_POINT ( 'NONE', #31754 ) ;
#176717=CARTESIAN_POINT ( 'NONE',  ( 4.050854035433010480, 7.948023151305657841, 0.000000000000000000 ) ) ;
#176766=CARTESIAN_POINT ( 'NONE',  ( -4.570507181138272479, 7.385989907086349504, 1.082531754730549967 ) ) ;
#176774=CARTESIAN_POINT ( 'NONE',  ( -6.231907884136888676, 7.299589282028351001, -1.199719254218453823 ) ) ;
#176779=ORIENTED_EDGE ( 'NONE', *, *, #66529, .T. ) ;
#176784=CARTESIAN_POINT ( 'NONE',  ( -4.847922445338252118, 7.813604065273374921, -1.199719254218453823 ) ) ;
#176787=CARTESIAN_POINT ( 'NONE',  ( 5.323208952783781811, 7.729862296028469970, 1.309151360253474339 ) ) ;
#176792=CARTESIAN_POINT ( 'NONE',  ( 4.342354338126830804, 8.288106837781779035, -0.7998128361456381397 ) ) ;
#176798=CARTESIAN_POINT ( 'NONE',  ( -6.831329296439251131, 9.063246493969506545, -1.599625672291271394 ) ) ;
#176803=CARTESIAN_POINT ( 'NONE',  ( -4.827585214917754719, 7.789877296449459365, -1.199719254218453823 ) ) ;
#176808=CARTESIAN_POINT ( 'NONE',  ( 4.353576723319599218, 8.093273587265928271, -0.7216878364870357165 ) ) ;
#176809=CARTESIAN_POINT ( 'NONE',  ( -5.763624699140882157, 7.817591130454727200, -1.443375672974066548 ) ) ;
#176814=CARTESIAN_POINT ( 'NONE',  ( -5.960744811863571968, 6.983232364376142698, 1.199719254218452935 ) ) ;
#176817=CARTESIAN_POINT ( 'NONE',  ( 4.206772801990143584, 8.129928378955675328, 0.7998128361456271485 ) ) ;
#176847=CARTESIAN_POINT ( 'NONE',  ( 4.615647837050825153, 8.347533190886938570, 0.2882115401751338402 ) ) ;
#176855=CARTESIAN_POINT ( 'NONE',  ( 5.318541398310776103, 9.426991741329731056, -0.7998128361456481317 ) ) ;
#176861=CARTESIAN_POINT ( 'NONE',  ( -4.636404737997885661, 8.342837909782009120, -0.3584692566244596645 ) ) ;
#176868=CARTESIAN_POINT ( 'NONE',  ( -5.465345319640241506, 5.548860092434608760, 0.7216878364870257245 ) ) ;
#176879=CARTESIAN_POINT ( 'NONE',  ( -3.923105346307911745, 5.670318552149568703, -1.599625672291283607 ) ) ;
#176881=CARTESIAN_POINT ( 'NONE',  ( 5.905458427204159477, 9.047396044116986502, 1.199719254218452047 ) ) ;
#176890=CARTESIAN_POINT ( 'NONE',  ( 4.355912491740495440, 8.303924683664389406, 0.000000000000000000 ) ) ;
#176893=CARTESIAN_POINT ( 'NONE',  ( 5.194182247366868843, 8.113610817686430110, 1.082531754730548412 ) ) ;
#176901=CARTESIAN_POINT ( 'NONE',  ( -6.353279334749129426, 6.853861929151015886, 0.6383911273219675664 ) ) ;
#176908=CARTESIAN_POINT ( 'NONE',  ( -5.808742468812186033, 5.741564066561132940, 0.000000000000000000 ) ) ;
#176909=CARTESIAN_POINT ( 'NONE',  ( 6.048345925472178308, 9.110135108809304327, 1.082531754730549967 ) ) ;
#176915=ORIENTED_EDGE ( 'NONE', *, *, #88237, .F. ) ;
#176919=EDGE_LOOP ( 'NONE', ( #105392, #209821, #148147, #48542, #113022 ) ) ;
#176920=CARTESIAN_POINT ( 'NONE',  ( -7.435720902452096936, 7.639705572474380091, 0.000000000000000000 ) ) ;
#176921=CARTESIAN_POINT ( 'NONE',  ( -5.798046968499580345, 6.793418213784815585, 1.199719254218452935 ) ) ;
#176923=CARTESIAN_POINT ( 'NONE',  ( 5.655159470231527763, 9.611786791996525636, -0.7216878364870458196 ) ) ;
#176926=LINE ( 'NONE', #15466, #115236 ) ;
#176927=CARTESIAN_POINT ( 'NONE',  ( 5.090160327287878594, 4.903218234782778850, -0.7998128361456481317 ) ) ;
#176934=CARTESIAN_POINT ( 'NONE',  ( -6.382290003970109815, 6.834844811514095397, -0.5765442458998057962 ) ) ;
#176935=DIRECTION ( 'NONE',  ( 0.000000000000000000, 0.000000000000000000, -1.000000000000000000 ) ) ;
#176944=CARTESIAN_POINT ( 'NONE',  ( -7.391130018105325661, 8.652015104991543026, -1.199719254218452047 ) ) ;
#176962=CARTESIAN_POINT ( 'NONE',  ( 5.234329823327693809, 8.264412672927770487, 1.199719254218451159 ) ) ;
#176996=CARTESIAN_POINT ( 'NONE',  ( 5.076602173674213070, 4.887400388900169368, 0.000000000000000000 ) ) ;
#177026=CARTESIAN_POINT ( 'NONE',  ( -3.955946960137363799, 7.837298230127379917, 0.7998128361456352531 ) ) ;
#177028=CARTESIAN_POINT ( 'NONE',  ( 4.841670253411575864, 8.662716039039905169, -0.7216878364870458196 ) ) ;
#177033=CARTESIAN_POINT ( 'NONE',  ( -5.815521545619021460, 5.749472989502435460, -0.7998128361456362523 ) ) ;
#177039=CARTESIAN_POINT ( 'NONE',  ( -2.810282979782591006, 6.500690253046801814, 0.000000000000000000 ) ) ;
#177041=( BOUNDED_SURFACE ( )  B_SPLINE_SURFACE ( 1, 2, ( 
 ( #45465, #145121, #176518, #206868, #208988, #92092, #44397, #142988, #174407, #191675, #43337, #175463, #27048, #159194, #60624, #74753, #126786, #58499, #210059, #160264, #144064, #124655, #110518, #190611, #140855, #77943, #61698, #127867, #193817, #42270, #111582, #177592, #29204, #41205, #211127, #62751, #173336, #150156, #85134, #84067, #69922, #19055, #20119, #136033, #178660, #167460, #184749, #166387, #46530, #179726, #31345, #51584, #100321, #113722, #17979, #151221, #153340, #112651, #1725, #13989, #30272, #37449, #96357, #202046, #117709, #195975, #133932, #3849, #67782, #129987, #199937, #101385, #183700, #4912, #194892, #146176, #35308, #86204, #47608, #2789, #103527, #70989, #68861, #134980, #200990, #52636, #162412, #80073, #169586, #118764, #36377, #212191, #63829, #53706, #102454, #168520, #152276, #119839, #185818, #21169, #87272, #121993, #125191, #156553, #92638, #8148, #138171, #137102, #120920, #205265, #10277, #191154, #42821, #186893, #190095, #39587, #172805, #187959, #204181, #7058, #203131, #124134, #107861, #105689, #104602, #189036, #91570, #171717, #55837, #88347, #157622, #41749, #108927, #23316, #54773, #38525, #56906, #170649, #174948, #26530, #22236, #173887, #89424, #24377, #155475, #73131, #139234, #154411, #25462, #9219, #123079, #5990, #40674, #75291, #106777, #90490, #72061, #141406, #207414, #158679, #74232, #140325, #206343, #57970, #59033, #44948, #143537, #127334, #111056, #193303, #60103, #28679, #27600, #30827, #211670, #179203, #93700, #177063, #11339, #192219, #13479, #46013, #94766, #63306, #77420, #160814, #209531, #159741, #76352, #12405, #113197, #61173, #78485, #178136, #144602, #162955, #112133, #96904, #14533, #210617, #79555, #129467, #62244, #142459, #128403, #194370, #43882, #114267, #164022, #31887, #97964, #29751, #130521, #80630, #95836, #146722, #161892, #145673, #195451, #47079, #208467, #212740, #64375, #196511, #109996, #48154, #180263, #126262, #176008, #165070, #116377, #167208, #18796, #148820, #201804, #133675, #68608, #84881, #150968, #2532, #16662 ),
 ( #99013, #49201, #66464, #32940, #82747, #199680, #53446, #393, #3598, #35049, #185568, #101120, #132605, #81683, #182365, #115322, #147769, #69675, #131556, #102203, #83807, #198611, #166131, #36119, #33995, #50258, #100069, #51323, #17718, #37198, #15597, #181312, #149899, #52388, #1467, #67533, #135781, #103272, #117451, #183445, #134731, #200738, #197557, #118516, #119585, #184500, #168269, #19869, #85954, #152029, #213785, #65408, #5728, #186643, #104346, #72886, #207164, #154162, #157372, #188784, #124943, #40420, #170390, #169335, #153086, #23058, #42569, #8967, #75040, #4662, #7885, #71807, #205014, #137918, #21979, #39336, #20919, #156302, #140068, #203938, #136848, #6808, #123883, #55586, #88089, #120665, #189848, #73973, #141156, #121741, #172549, #138993, #187708, #105433, #171469, #89175, #155227, #56660, #122823, #70734, #106523, #38269, #41494, #90236, #57725, #24134, #206091, #107607, #202872, #173638, #25211, #91315, #58787, #190905, #87014, #54520, #59852, #108672, #127080, #145425, #126004, #60923, #210359, #209276, #195197, #144358, #96655, #95593, #46834, #109746, #161641, #77164, #174700, #93450, #159488, #176809, #11087, #27348, #143285, #78236, #64131, #146470, #193043, #162708, #128155, #130275, #194115, #175756, #26275, #92391, #28425, #196263, #14280, #80375, #158427, #13236, #44697, #61999, #110804, #94518, #160556, #10027, #79309, #211426, #12164, #76102, #45765, #63056, #111883, #177887, #191965, #129223, #112948, #212489, #29500, #178959, #30574, #142205, #208220, #43631, #115072, #98766, #82493, #164822, #31637, #149, #213542, #2282, #183196, #150722, #65165, #16413, #197313, #163772, #199431, #17475, #148580, #34802, #48954, #66215, #181068, #131320, #47910, #132363, #84631, #32686, #198365, #149641, #50005, #134491, #83559, #35877, #100877, #200494, #116129, #166964, #182117, #114020, #33746, #99824, #165890, #1223, #67285, #133424, #51073, #3355, #180016, #117198, #81443, #97714, #101952, #15350, #52138, #18554, #68358, #118266, #184250, #168019, #19623, #85694, #151782 ) ),
 .UNSPECIFIED., .F., .F., .F. ) 
 B_SPLINE_SURFACE_WITH_KNOTS ( ( 2, 2 ),
 ( 3, 2, 2, 2, 2, 2, 2, 2, 2, 2, 2, 2, 2, 2, 2, 2, 2, 2, 2, 2, 2, 2, 2, 2, 2, 2, 2, 2, 2, 2, 2, 2, 2, 2, 2, 2, 2, 2, 2, 2, 2, 2, 2, 2, 2, 2, 2, 2, 2, 2, 2, 2, 2, 2, 2, 2, 2, 2, 2, 2, 2, 2, 2, 2, 2, 2, 2, 2, 2, 2, 2, 2, 2, 2, 2, 2, 2, 2, 2, 2, 2, 2, 2, 2, 2, 2, 2, 2, 2, 2, 2, 2, 2, 2, 2, 2, 2, 2, 2, 2, 2, 2, 2, 2, 2, 2, 2, 2, 2, 2, 2, 2, 2, 2, 2, 2, 2, 2, 2, 2, 3 ),
 ( 0.000000000000000000, 1.000000000000000000 ),
 ( 0.000000000000000000, 0.008333333333333333218, 0.01666666666666666644, 0.02500000000000000139, 0.03333333333333333287, 0.04166666666666666435, 0.05000000000000000278, 0.05833333333333333426, 0.06666666666666666574, 0.07499999999999999722, 0.08333333333333332871, 0.09166666666666666019, 0.1000000000000000056, 0.1083333333333333370, 0.1166666666666666685, 0.1250000000000000000, 0.1333333333333333315, 0.1416666666666666630, 0.1499999999999999944, 0.1583333333333333259, 0.1666666666666666574, 0.1749999999999999889, 0.1833333333333333204, 0.1916666666666666796, 0.2000000000000000111, 0.2083333333333333426, 0.2166666666666666741, 0.2250000000000000056, 0.2333333333333333370, 0.2416666666666666685, 0.2500000000000000000, 0.2583333333333333592, 0.2666666666666666630, 0.2750000000000000222, 0.2833333333333333259, 0.2916666666666666852, 0.2999999999999999889, 0.3083333333333333481, 0.3166666666666666519, 0.3250000000000000111, 0.3333333333333333148, 0.3416666666666666741, 0.3499999999999999778, 0.3583333333333333370, 0.3666666666666666408, 0.3750000000000000000, 0.3833333333333333592, 0.3916666666666666630, 0.4000000000000000222, 0.4083333333333333259, 0.4166666666666666852, 0.4249999999999999889, 0.4333333333333333481, 0.4416666666666666519, 0.4500000000000000111, 0.4583333333333333148, 0.4666666666666666741, 0.4749999999999999778, 0.4833333333333333370, 0.4916666666666666408, 0.5000000000000000000, 0.5083333333333333037, 0.5166666666666667185, 0.5250000000000000222, 0.5333333333333333259, 0.5416666666666666297, 0.5500000000000000444, 0.5583333333333333481, 0.5666666666666666519, 0.5749999999999999556, 0.5833333333333333703, 0.5916666666666666741, 0.5999999999999999778, 0.6083333333333332815, 0.6166666666666666963, 0.6250000000000000000, 0.6333333333333333037, 0.6416666666666667185, 0.6500000000000000222, 0.6583333333333333259, 0.6666666666666666297, 0.6750000000000000444, 0.6833333333333333481, 0.6916666666666666519, 0.6999999999999999556, 0.7083333333333333703, 0.7166666666666666741, 0.7249999999999999778, 0.7333333333333332815, 0.7416666666666666963, 0.7500000000000000000, 0.7583333333333333037, 0.7666666666666667185, 0.7750000000000000222, 0.7833333333333333259, 0.7916666666666666297, 0.8000000000000000444, 0.8083333333333333481, 0.8166666666666666519, 0.8249999999999999556, 0.8333333333333333703, 0.8416666666666666741, 0.8499999999999999778, 0.8583333333333332815, 0.8666666666666666963, 0.8750000000000000000, 0.8833333333333333037, 0.8916666666666667185, 0.9000000000000000222, 0.9083333333333333259, 0.9166666666666666297, 0.9250000000000000444, 0.9333333333333333481, 0.9416666666666666519, 0.9499999999999999556, 0.9583333333333333703, 0.9666666666666666741, 0.9749999999999999778, 0.9833333333333332815, 0.9916666666666666963, 1.000000000000000000 ),
 .UNSPECIFIED. ) 
 GEOMETRIC_REPRESENTATION_ITEM ( )  RATIONAL_B_SPLINE_SURFACE ( (
 ( 1.000000000000000000, 0.8660254037844387076, 1.000000000000000000, 0.8660254037844387076, 1.000000000000000000, 0.8660254037844387076, 1.000000000000000000, 0.8660254037844387076, 1.000000000000000000, 0.8660254037844387076, 1.000000000000000000, 0.8660254037844387076, 1.000000000000000000, 0.8660254037844387076, 1.000000000000000000, 0.8660254037844387076, 1.000000000000000000, 0.8660254037844387076, 1.000000000000000000, 0.8660254037844387076, 1.000000000000000000, 0.8660254037844387076, 1.000000000000000000, 0.8660254037844387076, 1.000000000000000000, 0.8660254037844387076, 1.000000000000000000, 0.8660254037844387076, 1.000000000000000000, 0.8660254037844387076, 1.000000000000000000, 0.8660254037844387076, 1.000000000000000000, 0.8660254037844387076, 1.000000000000000000, 0.8660254037844387076, 1.000000000000000000, 0.8660254037844387076, 1.000000000000000000, 0.8660254037844387076, 1.000000000000000000, 0.8660254037844387076, 1.000000000000000000, 0.8660254037844387076, 1.000000000000000000, 0.8660254037844387076, 1.000000000000000000, 0.8660254037844387076, 1.000000000000000000, 0.8660254037844387076, 1.000000000000000000, 0.8660254037844387076, 1.000000000000000000, 0.8660254037844387076, 1.000000000000000000, 0.8660254037844387076, 1.000000000000000000, 0.8660254037844387076, 1.000000000000000000, 0.8660254037844387076, 1.000000000000000000, 0.8660254037844387076, 1.000000000000000000, 0.8660254037844387076, 1.000000000000000000, 0.8660254037844387076, 1.000000000000000000, 0.8660254037844387076, 1.000000000000000000, 0.8660254037844387076, 1.000000000000000000, 0.8660254037844387076, 1.000000000000000000, 0.8660254037844387076, 1.000000000000000000, 0.8660254037844387076, 1.000000000000000000, 0.8660254037844387076, 1.000000000000000000, 0.8660254037844387076, 1.000000000000000000, 0.8660254037844387076, 1.000000000000000000, 0.8660254037844387076, 1.000000000000000000, 0.8660254037844387076, 1.000000000000000000, 0.8660254037844387076, 1.000000000000000000, 0.8660254037844387076, 1.000000000000000000, 0.8660254037844387076, 1.000000000000000000, 0.8660254037844387076, 1.000000000000000000, 0.8660254037844387076, 1.000000000000000000, 0.8660254037844387076, 1.000000000000000000, 0.8660254037844387076, 1.000000000000000000, 0.8660254037844387076, 1.000000000000000000, 0.8660254037844387076, 1.000000000000000000, 0.8660254037844387076, 1.000000000000000000, 0.8660254037844387076, 1.000000000000000000, 0.8660254037844387076, 1.000000000000000000, 0.8660254037844387076, 1.000000000000000000, 0.8660254037844387076, 1.000000000000000000, 0.8660254037844387076, 1.000000000000000000, 0.8660254037844387076, 1.000000000000000000, 0.8660254037844387076, 1.000000000000000000, 0.8660254037844387076, 1.000000000000000000, 0.8660254037844387076, 1.000000000000000000, 0.8660254037844387076, 1.000000000000000000, 0.8660254037844387076, 1.000000000000000000, 0.8660254037844387076, 1.000000000000000000, 0.8660254037844387076, 1.000000000000000000, 0.8660254037844387076, 1.000000000000000000, 0.8660254037844387076, 1.000000000000000000, 0.8660254037844387076, 1.000000000000000000, 0.8660254037844387076, 1.000000000000000000, 0.8660254037844387076, 1.000000000000000000, 0.8660254037844387076, 1.000000000000000000, 0.8660254037844387076, 1.000000000000000000, 0.8660254037844387076, 1.000000000000000000, 0.8660254037844387076, 1.000000000000000000, 0.8660254037844387076, 1.000000000000000000, 0.8660254037844387076, 1.000000000000000000, 0.8660254037844387076, 1.000000000000000000, 0.8660254037844387076, 1.000000000000000000, 0.8660254037844387076, 1.000000000000000000, 0.8660254037844387076, 1.000000000000000000, 0.8660254037844387076, 1.000000000000000000, 0.8660254037844387076, 1.000000000000000000, 0.8660254037844387076, 1.000000000000000000, 0.8660254037844387076, 1.000000000000000000, 0.8660254037844387076, 1.000000000000000000, 0.8660254037844387076, 1.000000000000000000, 0.8660254037844387076, 1.000000000000000000, 0.8660254037844387076, 1.000000000000000000, 0.8660254037844387076, 1.000000000000000000, 0.8660254037844387076, 1.000000000000000000, 0.8660254037844387076, 1.000000000000000000, 0.8660254037844387076, 1.000000000000000000, 0.8660254037844387076, 1.000000000000000000, 0.8660254037844387076, 1.000000000000000000, 0.8660254037844387076, 1.000000000000000000, 0.8660254037844387076, 1.000000000000000000, 0.8660254037844387076, 1.000000000000000000, 0.8660254037844387076, 1.000000000000000000, 0.8660254037844387076, 1.000000000000000000, 0.8660254037844387076, 1.000000000000000000, 0.8660254037844387076, 1.000000000000000000, 0.8660254037844387076, 1.000000000000000000, 0.8660254037844387076, 1.000000000000000000, 0.8660254037844387076, 1.000000000000000000, 0.8660254037844387076, 1.000000000000000000, 0.8660254037844387076, 1.000000000000000000, 0.8660254037844387076, 1.000000000000000000, 0.8660254037844387076, 1.000000000000000000, 0.8660254037844387076, 1.000000000000000000, 0.8660254037844387076, 1.000000000000000000, 0.8660254037844387076, 1.000000000000000000, 0.8660254037844387076, 1.000000000000000000, 0.8660254037844387076, 1.000000000000000000, 0.8660254037844387076, 1.000000000000000000, 0.8660254037844387076, 1.000000000000000000, 0.8660254037844387076, 1.000000000000000000, 0.8660254037844387076, 1.000000000000000000, 0.8660254037844387076, 1.000000000000000000, 0.8660254037844387076, 1.000000000000000000),
 ( 1.000000000000000000, 0.8660254037844387076, 1.000000000000000000, 0.8660254037844387076, 1.000000000000000000, 0.8660254037844387076, 1.000000000000000000, 0.8660254037844387076, 1.000000000000000000, 0.8660254037844387076, 1.000000000000000000, 0.8660254037844387076, 1.000000000000000000, 0.8660254037844387076, 1.000000000000000000, 0.8660254037844387076, 1.000000000000000000, 0.8660254037844387076, 1.000000000000000000, 0.8660254037844387076, 1.000000000000000000, 0.8660254037844387076, 1.000000000000000000, 0.8660254037844387076, 1.000000000000000000, 0.8660254037844387076, 1.000000000000000000, 0.8660254037844387076, 1.000000000000000000, 0.8660254037844387076, 1.000000000000000000, 0.8660254037844387076, 1.000000000000000000, 0.8660254037844387076, 1.000000000000000000, 0.8660254037844387076, 1.000000000000000000, 0.8660254037844387076, 1.000000000000000000, 0.8660254037844387076, 1.000000000000000000, 0.8660254037844387076, 1.000000000000000000, 0.8660254037844387076, 1.000000000000000000, 0.8660254037844387076, 1.000000000000000000, 0.8660254037844387076, 1.000000000000000000, 0.8660254037844387076, 1.000000000000000000, 0.8660254037844387076, 1.000000000000000000, 0.8660254037844387076, 1.000000000000000000, 0.8660254037844387076, 1.000000000000000000, 0.8660254037844387076, 1.000000000000000000, 0.8660254037844387076, 1.000000000000000000, 0.8660254037844387076, 1.000000000000000000, 0.8660254037844387076, 1.000000000000000000, 0.8660254037844387076, 1.000000000000000000, 0.8660254037844387076, 1.000000000000000000, 0.8660254037844387076, 1.000000000000000000, 0.8660254037844387076, 1.000000000000000000, 0.8660254037844387076, 1.000000000000000000, 0.8660254037844387076, 1.000000000000000000, 0.8660254037844387076, 1.000000000000000000, 0.8660254037844387076, 1.000000000000000000, 0.8660254037844387076, 1.000000000000000000, 0.8660254037844387076, 1.000000000000000000, 0.8660254037844387076, 1.000000000000000000, 0.8660254037844387076, 1.000000000000000000, 0.8660254037844387076, 1.000000000000000000, 0.8660254037844387076, 1.000000000000000000, 0.8660254037844387076, 1.000000000000000000, 0.8660254037844387076, 1.000000000000000000, 0.8660254037844387076, 1.000000000000000000, 0.8660254037844387076, 1.000000000000000000, 0.8660254037844387076, 1.000000000000000000, 0.8660254037844387076, 1.000000000000000000, 0.8660254037844387076, 1.000000000000000000, 0.8660254037844387076, 1.000000000000000000, 0.8660254037844387076, 1.000000000000000000, 0.8660254037844387076, 1.000000000000000000, 0.8660254037844387076, 1.000000000000000000, 0.8660254037844387076, 1.000000000000000000, 0.8660254037844387076, 1.000000000000000000, 0.8660254037844387076, 1.000000000000000000, 0.8660254037844387076, 1.000000000000000000, 0.8660254037844387076, 1.000000000000000000, 0.8660254037844387076, 1.000000000000000000, 0.8660254037844387076, 1.000000000000000000, 0.8660254037844387076, 1.000000000000000000, 0.8660254037844387076, 1.000000000000000000, 0.8660254037844387076, 1.000000000000000000, 0.8660254037844387076, 1.000000000000000000, 0.8660254037844387076, 1.000000000000000000, 0.8660254037844387076, 1.000000000000000000, 0.8660254037844387076, 1.000000000000000000, 0.8660254037844387076, 1.000000000000000000, 0.8660254037844387076, 1.000000000000000000, 0.8660254037844387076, 1.000000000000000000, 0.8660254037844387076, 1.000000000000000000, 0.8660254037844387076, 1.000000000000000000, 0.8660254037844387076, 1.000000000000000000, 0.8660254037844387076, 1.000000000000000000, 0.8660254037844387076, 1.000000000000000000, 0.8660254037844387076, 1.000000000000000000, 0.8660254037844387076, 1.000000000000000000, 0.8660254037844387076, 1.000000000000000000, 0.8660254037844387076, 1.000000000000000000, 0.8660254037844387076, 1.000000000000000000, 0.8660254037844387076, 1.000000000000000000, 0.8660254037844387076, 1.000000000000000000, 0.8660254037844387076, 1.000000000000000000, 0.8660254037844387076, 1.000000000000000000, 0.8660254037844387076, 1.000000000000000000, 0.8660254037844387076, 1.000000000000000000, 0.8660254037844387076, 1.000000000000000000, 0.8660254037844387076, 1.000000000000000000, 0.8660254037844387076, 1.000000000000000000, 0.8660254037844387076, 1.000000000000000000, 0.8660254037844387076, 1.000000000000000000, 0.8660254037844387076, 1.000000000000000000, 0.8660254037844387076, 1.000000000000000000, 0.8660254037844387076, 1.000000000000000000, 0.8660254037844387076, 1.000000000000000000, 0.8660254037844387076, 1.000000000000000000, 0.8660254037844387076, 1.000000000000000000, 0.8660254037844387076, 1.000000000000000000, 0.8660254037844387076, 1.000000000000000000, 0.8660254037844387076, 1.000000000000000000, 0.8660254037844387076, 1.000000000000000000, 0.8660254037844387076, 1.000000000000000000, 0.8660254037844387076, 1.000000000000000000, 0.8660254037844387076, 1.000000000000000000, 0.8660254037844387076, 1.000000000000000000, 0.8660254037844387076, 1.000000000000000000, 0.8660254037844387076, 1.000000000000000000, 0.8660254037844387076, 1.000000000000000000, 0.8660254037844387076, 1.000000000000000000, 0.8660254037844387076, 1.000000000000000000, 0.8660254037844387076, 1.000000000000000000, 0.8660254037844387076, 1.000000000000000000, 0.8660254037844387076, 1.000000000000000000, 0.8660254037844387076, 1.000000000000000000, 0.8660254037844387076, 1.000000000000000000, 0.8660254037844387076, 1.000000000000000000) ) ) 
 REPRESENTATION_ITEM ( '' )  SURFACE ( )  );
#177047=CARTESIAN_POINT ( 'NONE',  ( -5.529746549527323474, 7.544733289238903851, -1.599625672291271394 ) ) ;
#177056=CARTESIAN_POINT ( 'NONE',  ( -4.553559489343377287, 6.405848385690952718, -1.599625672291271394 ) ) ;
#177059=CARTESIAN_POINT ( 'NONE',  ( -5.316205630334263965, 7.295602216847000498, -1.443375672974066548 ) ) ;
#177061=CARTESIAN_POINT ( 'NONE',  ( -4.434925645001610128, 8.188180662561590495, 0.7216878364870338292 ) ) ;
#177062=CARTESIAN_POINT ( 'NONE',  ( 6.496291879603339758, 7.608037276739255006, 1.199719254218452935 ) ) ;
#177063=CARTESIAN_POINT ( 'NONE',  ( -6.282224075085783177, 8.422623735723785643, 1.599625672291269396 ) ) ;
#177091=AXIS2_PLACEMENT_3D ( 'NONE', #163640, #160427, #14149 ) ;
#177101=CARTESIAN_POINT ( 'NONE',  ( 4.639288533706844575, 8.435234533841581950, -0.4270733708018232822 ) ) ;
#177114=CARTESIAN_POINT ( 'NONE',  ( 5.417364897112183719, 8.477953592343014932, 1.199719254218451159 ) ) ;
#177117=CARTESIAN_POINT ( 'NONE',  ( -3.318713740295064163, 7.093859473644694269, 0.000000000000000000 ) ) ;
#177121=CARTESIAN_POINT ( 'NONE',  ( -7.390603132780795725, 8.755363422066633206, -1.082531754730549967 ) ) ;
#177132=CARTESIAN_POINT ( 'NONE',  ( 3.573456005653643519, 6.326726552307992080, -1.199719254218453823 ) ) ;
#177133=AXIS2_PLACEMENT_3D ( 'NONE', #181923, #165692, #1024 ) ;
#177134=CARTESIAN_POINT ( 'NONE',  ( 5.825163275726873202, 6.825053905550038991, 1.199719254218452047 ) ) ;
#177142=CARTESIAN_POINT ( 'NONE',  ( 5.083381250481017410, 4.895309311841474553, 0.7998128361456352531 ) ) ;
#177148=CARTESIAN_POINT ( 'NONE',  ( 6.710359684120930091, 6.793450817754725257, 0.7998128361456352531 ) ) ;
#177161=CARTESIAN_POINT ( 'NONE',  ( -5.804299160426242388, 6.904675454319632699, -1.082531754730549967 ) ) ;
#177162=CARTESIAN_POINT ( 'NONE',  ( -5.101610940492132151, 9.173906207207963348, -0.7998128361456362523 ) ) ;
#177176=CARTESIAN_POINT ( 'NONE',  ( 6.119526231721748033, 8.232809585132461194, 1.599625672291269396 ) ) ;
#177180=CARTESIAN_POINT ( 'NONE',  ( 5.045042557616584489, 5.058506870073687267, 0.000000000000000000 ) ) ;
#177195=CARTESIAN_POINT ( 'NONE',  ( -4.858757509019059562, 5.629766575900002401, 2.499999999999999556 ) ) ;
#177199=CARTESIAN_POINT ( 'NONE',  ( 6.710359684120930091, 6.793450817754725257, 0.7998128361456352531 ) ) ;
#177202=EDGE_CURVE ( 'NONE', #512, #83383, #157769, .T. ) ;
#177205=CARTESIAN_POINT ( 'NONE',  ( 4.362691568547328202, 8.311833606605697256, -0.7998128361456381397 ) ) ;
#177214=CARTESIAN_POINT ( 'NONE',  ( 7.241463443474815520, 8.581367117876336437, -1.082531754730548412 ) ) ;
#177216=CARTESIAN_POINT ( 'NONE',  ( -7.618755976236585958, 7.853246491889623648, 0.000000000000000000 ) ) ;
#177217=CARTESIAN_POINT ( 'NONE',  ( 5.890091390494168522, 5.836471141856793388, 0.000000000000000000 ) ) ;
#177228=CARTESIAN_POINT ( 'NONE',  ( -5.123001941117347080, 7.070197912760590064, 1.599625672291263179 ) ) ;
#177256=CARTESIAN_POINT ( 'NONE',  ( 4.909461021924244051, 6.821066840368686712, 1.443375672974065660 ) ) ;
#177262=CARTESIAN_POINT ( 'NONE',  ( 5.248414861821569133, 6.256143772614186638, -1.082531754730548412 ) ) ;
#177275=CARTESIAN_POINT ( 'NONE',  ( -5.306037014901836990, 7.283738832175834510, 1.599625672291263179 ) ) ;
#177277=CARTESIAN_POINT ( 'NONE',  ( -6.343235766347277149, 8.493804042195527870, -1.599625672291271394 ) ) ;
#177279=CARTESIAN_POINT ( 'NONE',  ( 7.526184668917440312, 8.913541880892736913, -1.082531754730548412 ) ) ;
#177282=UNCERTAINTY_MEASURE_WITH_UNIT (LENGTH_MEASURE( 1.000000000000000082E-05 ), #210372, 'distance_accuracy_value', 'NONE');
#177283=CARTESIAN_POINT ( 'NONE',  ( -3.816847834374289317, 7.349700740952370914, -0.7361462914088554577 ) ) ;
#177290=CARTESIAN_POINT ( 'NONE',  ( -3.188928480291426837, 8.980740528189164351, -2.451733079074508659 ) ) ;
#177291=CARTESIAN_POINT ( 'NONE',  ( -6.286140498591554326, 7.362860665558790707, 1.199719254218452047 ) ) ;
#177297=CARTESIAN_POINT ( 'NONE',  ( -5.817857314039913241, 5.960124085900898372, 0.000000000000000000 ) ) ;
#177301=CARTESIAN_POINT ( 'NONE',  ( -5.808742468812186033, 5.741564066561132940, 0.000000000000000000 ) ) ;
#177321=CARTESIAN_POINT ( 'NONE',  ( -5.607179047703544583, 8.699403434699558346, 1.199719254218454489 ) ) ;
#177323=CARTESIAN_POINT ( 'NONE',  ( -5.113360211009450040, 5.994616996712990975, -1.199719254218453823 ) ) ;
#177349=CARTESIAN_POINT ( 'NONE',  ( -7.119966945832006289, 8.335658187339330283, 1.199719254218452047 ) ) ;
#177374=CARTESIAN_POINT ( 'NONE',  ( 8.039058738260216330, 8.343599714250547805, -0.7998128361456341429 ) ) ;
#177376=CARTESIAN_POINT ( 'NONE',  ( 7.693325821111733021, 7.940244644243982464, -0.7998128361456341429 ) ) ;
#177377=CARTESIAN_POINT ( 'NONE',  ( 0.000000000000000000, 6.002124920821316323, 0.000000000000000000 ) ) ;
#177389=CARTESIAN_POINT ( 'NONE',  ( 5.825676364550436581, 7.207913871576331566, 1.168708750232345883 ) ) ;
#177391=CARTESIAN_POINT ( 'NONE',  ( 7.512626515748113576, 7.937354821227203594, 0.7216878364870267237 ) ) ;
#177398=CARTESIAN_POINT ( 'NONE',  ( -3.772911886352873445, 7.623757310712140800, 0.7998128361456352531 ) ) ;
#177404=CARTESIAN_POINT ( 'NONE',  ( -4.936577328707246082, 8.773440960218172435, 0.000000000000000000 ) ) ;
#177407=CARTESIAN_POINT ( 'NONE',  ( -4.000799973277850974, 7.681462069183943697, 0.02035690600471253345 ) ) ;
#177408=B_SPLINE_CURVE_WITH_KNOTS ( 'NONE', 3,
 ( #136411, #32495, #66022, #118076, #34618, #84439, #98569, #99629, #1027, #86576, #214393, #100688, #102831, #82299, #35681, #180873 ),
 .UNSPECIFIED., .F., .F.,
 ( 4, 2, 2, 2, 2, 2, 2, 4 ),
 ( 0.4818577711483807979, 0.5128210221889952791, 0.5283026477093025752, 0.5437842732296098713, 0.5592658987499171674, 0.5747475242702243525, 0.5902291497905316486, 0.6057107753108389447 ),
 .UNSPECIFIED. ) ;
#177421=CARTESIAN_POINT ( 'NONE',  ( -6.608673532018475960, 6.674816973635147477, -0.7998128361456361413 ) ) ;
#177423=CARTESIAN_POINT ( 'NONE',  ( 5.671053392266061977, 9.838255734277600695, 0.7998128361456331437 ) ) ;
#177431=AXIS2_PLACEMENT_3D ( 'NONE', #124020, #189985, #157513 ) ;
#177446=CARTESIAN_POINT ( 'NONE',  ( 6.530187263637528439, 7.647581891445782709, -1.199719254218452047 ) ) ;
#177449=CARTESIAN_POINT ( 'NONE',  ( -6.160225556963538018, 6.983552031129079296, 0.9223575212774417498 ) ) ;
#177455=CARTESIAN_POINT ( 'NONE',  ( 4.420840606507738357, 7.315341919971147355, 1.199719254218451159 ) ) ;
#177458=CARTESIAN_POINT ( 'NONE',  ( -5.575940895411126697, 5.849477901847593309, -0.6286834815852658798 ) ) ;
#177468=CARTESIAN_POINT ( 'NONE',  ( 6.048345925472191631, 6.229027465905275562, 0.7216878364870328300 ) ) ;
#177478=CARTESIAN_POINT ( 'NONE',  ( -4.163762573172648196, 7.871823745427799501, 0.000000000000000000 ) ) ;
#177511=CARTESIAN_POINT ( 'NONE',  ( 6.378184920586140727, 6.405913593630768510, 0.000000000000000000 ) ) ;
#177523=CARTESIAN_POINT ( 'NONE',  ( -3.298376509874564988, 7.070132704820777825, 0.000000000000000000 ) ) ;
#177526=CARTESIAN_POINT ( 'NONE',  ( 5.383996397958233260, 5.453953017138946535, -0.7216878364870458196 ) ) ;
#177543=CARTESIAN_POINT ( 'NONE',  ( -5.099275172515603138, 8.002885897026576600, 1.082531754730549967 ) ) ;
#177545=CARTESIAN_POINT ( 'NONE',  ( -3.675669043080673770, 7.302381293653823491, 0.000000000000000000 ) ) ;
#177549=CARTESIAN_POINT ( 'NONE',  ( 4.760321332173959696, 4.726332107057286791, 0.000000000000000000 ) ) ;
#177553=CARTESIAN_POINT ( 'NONE',  ( -4.459788646379888810, 7.974764203887369618, -0.6295236818997522743 ) ) ;
#177578=LINE ( 'NONE', #212179, #212063 ) ;
#177581=CARTESIAN_POINT ( 'NONE',  ( -5.912237504011027767, 9.055304967058290799, 1.199719254218454489 ) ) ;
#177582=CARTESIAN_POINT ( 'NONE',  ( -4.785410049391000342, 8.260660143818395085, 0.8633373473483215710 ) ) ;
#177592=CARTESIAN_POINT ( 'NONE',  ( -5.354544322754380303, 5.211666229493680191, 0.7998128361456281477 ) ) ;
#177595=CARTESIAN_POINT ( 'NONE',  ( -4.359828915246279024, 7.244161613499399799, -1.199719254218455378 ) ) ;
#177608=CARTESIAN_POINT ( 'NONE',  ( 5.061990249855835344, 6.999017606288844284, -1.599625672291273171 ) ) ;
#177636=CARTESIAN_POINT ( 'NONE',  ( 6.204791576909545192, 7.267953590263130259, -1.199719254218452047 ) ) ;
#177637=CARTESIAN_POINT ( 'NONE',  ( 3.386504508363381571, 7.172948703057747011, -0.7998128361456362523 ) ) ;
#177639=CARTESIAN_POINT ( 'NONE',  ( 4.577813143269636065, 5.369812084349879555, -1.199719254218450271 ) ) ;
#177650=CARTESIAN_POINT ( 'NONE',  ( 4.930145672075521013, 8.107674077938057167, 1.051636801887654293 ) ) ;
#177651=CARTESIAN_POINT ( 'NONE',  ( -5.763624699140883934, 6.857221916153382502, -1.082531754730549967 ) ) ;
#177652=CARTESIAN_POINT ( 'NONE',  ( 4.312902262922978736, 5.164712407232485702, -1.082531754730548412 ) ) ;
#177653=( BOUNDED_CURVE ( )  B_SPLINE_CURVE ( 2, ( #85798, #151877, #3452, #119430, #185417, #136696, #169177 ),
 .UNSPECIFIED., .F., .T. ) 
 B_SPLINE_CURVE_WITH_KNOTS ( ( 3, 2, 2, 3 ),
 ( 0.4249999999999999334, 0.4333333333333332926, 0.4416666666666665964, 0.4499999999999999556 ),
 .UNSPECIFIED. ) 
 CURVE ( )  GEOMETRIC_REPRESENTATION_ITEM ( )  RATIONAL_B_SPLINE_CURVE ( ( 1.000000000000000888, 0.8660254037844378194, 1.000000000000000000, 0.8660254037844387076, 1.000000000000000000, 0.8660254037844395958, 0.9999999999999991118 ) ) 
 REPRESENTATION_ITEM ( '' )  );
#177670=CARTESIAN_POINT ( 'NONE',  ( -5.608349667956210816, 5.604589570211684801, -0.4131542205010517166 ) ) ;
#177676=CARTESIAN_POINT ( 'NONE',  ( 5.204350862799327793, 7.165104988056252289, -1.599625672291281386 ) ) ;
#177694=CARTESIAN_POINT ( 'NONE',  ( -7.391130018105325661, 8.652015104991543026, -1.199719254218452047 ) ) ;
#177696=ORIENTED_EDGE ( 'NONE', *, *, #97685, .F. ) ;
#177706=CARTESIAN_POINT ( 'NONE',  ( 5.825163275726873202, 6.825053905550038991, 1.199719254218452047 ) ) ;
#177713=CARTESIAN_POINT ( 'NONE',  ( 4.213551878797002992, 8.137837301896977849, 0.000000000000000000 ) ) ;
#177718=EDGE_CURVE ( 'NONE', #113990, #35662, #39107, .T. ) ;
#177724=CARTESIAN_POINT ( 'NONE',  ( 4.625518323863472503, 8.335144253906971556, 0.3473850511846506839 ) ) ;
#177741=CARTESIAN_POINT ( 'NONE',  ( -4.620296487206990932, 8.612372678375294299, 0.000000000000000000 ) ) ;
#177743=CARTESIAN_POINT ( 'NONE',  ( 6.384963997392946844, 6.413822516572072807, 0.7998128361456352531 ) ) ;
#177747=CARTESIAN_POINT ( 'NONE',  ( -6.882699257592852504, 8.058845884393651460, -1.199719254218452047 ) ) ;
#177751=DIRECTION ( 'NONE',  ( 0.000000000000000000, 0.000000000000000000, 1.000000000000000000 ) ) ;
#177755=CARTESIAN_POINT ( 'NONE',  ( -6.117836340636773507, 7.096790560477957754, -1.125390141808879196 ) ) ;
#177770=EDGE_LOOP ( 'NONE', ( #8779, #23927 ) ) ;
#177773=ORIENTED_EDGE ( 'NONE', *, *, #52019, .F. ) ;
#177774=CARTESIAN_POINT ( 'NONE',  ( 5.560252395380206991, 7.580323442733986283, 1.443375672974065660 ) ) ;
#177793=CARTESIAN_POINT ( 'NONE',  ( 3.901714345682657292, 7.774026846596938434, 0.7998128361456271485 ) ) ;
#177847=CARTESIAN_POINT ( 'NONE',  ( -4.082413651046300274, 6.816547455312373494, 1.082531754730549967 ) ) ;
#177853=CARTESIAN_POINT ( 'NONE',  ( -4.502189528189771472, 7.410248995266807803, -1.199719254218453823 ) ) ;
#177859=EDGE_LOOP ( 'NONE', ( #174120, #14131, #63102, #107195 ) ) ;
#177863=CARTESIAN_POINT ( 'NONE',  ( -3.793249116773374396, 7.647484079536056356, 0.7998128361456352531 ) ) ;
#177865=CARTESIAN_POINT ( 'NONE',  ( 5.703612580814390043, 7.410739916031705121, 1.319003781635886163 ) ) ;
#177870=CARTESIAN_POINT ( 'NONE',  ( 5.611095471209277541, 7.639640364534566075, 1.599625672291268286 ) ) ;
#177876=CARTESIAN_POINT ( 'NONE',  ( -4.858757509019083543, 5.629766575900002401, -2.500000000000000444 ) ) ;
#177877=CARTESIAN_POINT ( 'NONE',  ( -4.679499295372141709, 5.488445928469455559, 1.199719254218452935 ) ) ;
#177881=CARTESIAN_POINT ( 'NONE',  ( -4.450819567036169211, 8.414649604842665553, -0.7998128361456362523 ) ) ;
#177885=CARTESIAN_POINT ( 'NONE',  ( 7.146556367734776316, 7.510272981878305387, 0.7216878364870267237 ) ) ;
#177887=CARTESIAN_POINT ( 'NONE',  ( -5.275531169048895741, 9.168887107283438809, -0.7216878364870338292 ) ) ;
#177891=CARTESIAN_POINT ( 'NONE',  ( -4.773352600463090845, 7.726605912919016106, 1.199719254218452935 ) ) ;
#177894=CARTESIAN_POINT ( 'NONE',  ( 6.364626766972446781, 6.390095747748157251, 0.7998128361456352531 ) ) ;
#177900=CARTESIAN_POINT ( 'NONE',  ( 4.342354338126830804, 8.288106837781777259, -0.7998128361456381397 ) ) ;
#177917=CARTESIAN_POINT ( 'NONE',  ( 5.450602278258352307, 7.609395523180757515, -1.379288001542776865 ) ) ;
#177922=CARTESIAN_POINT ( 'NONE',  ( 4.597294405107005488, 8.370805622008914426, 0.1071034531749150143 ) ) ;
#177930=CARTESIAN_POINT ( 'NONE',  ( 6.017840079619279692, 8.114175741012878973, -1.599625672291281386 ) ) ;
#177936=CARTESIAN_POINT ( 'NONE',  ( -4.619186966818853435, 8.364647258818639131, 0.2498820228645174391 ) ) ;
#177943=CARTESIAN_POINT ( 'NONE',  ( -5.451787166026575981, 5.533042246551999277, 0.000000000000000000 ) ) ;
#177953=CARTESIAN_POINT ( 'NONE',  ( -5.503684012504701961, 5.385662534202396934, 0.000000000000000000 ) ) ;
#177965=CARTESIAN_POINT ( 'NONE',  ( 5.876533236880477240, 5.820653295974182129, 0.7998128361456352531 ) ) ;
#177968=CARTESIAN_POINT ( 'NONE',  ( 5.844973620822844218, 6.952128991449046502, 1.082531754730549967 ) ) ;
#177983=CARTESIAN_POINT ( 'NONE',  ( -5.659602779061863487, 5.567567761852417085, 0.7998128361456281477 ) ) ;
#177986=CARTESIAN_POINT ( 'NONE',  ( 4.309512724297349884, 6.121127159803966933, 1.599625672291261402 ) ) ;
#177995=ORIENTED_EDGE ( 'NONE', *, *, #112332, .F. ) ;
#177996=CARTESIAN_POINT ( 'NONE',  ( -5.315678745009726924, 8.359319748223434487, -1.199719254218453823 ) ) ;
#177997=CARTESIAN_POINT ( 'NONE',  ( 5.993586425693011144, 9.150212042353954800, -1.199719254218452047 ) ) ;
#177999=CARTESIAN_POINT ( 'NONE',  ( 7.485510208076452621, 7.905719128943566432, 0.000000000000000000 ) ) ;
#178003=CARTESIAN_POINT ( 'NONE',  ( 5.076602173674213070, 4.887400388900169368, 0.000000000000000000 ) ) ;
#178009=CARTESIAN_POINT ( 'NONE',  ( -5.095330737579740976, 7.839774693193753308, -1.136590250493845877 ) ) ;
#178016=CARTESIAN_POINT ( 'NONE',  ( -6.583366107887490770, 9.838288338247510367, 1.199719254218452935 ) ) ;
#178035=CARTESIAN_POINT ( 'NONE',  ( 6.866278450678116485, 6.975356045404744521, 0.000000000000000000 ) ) ;
#178068=CARTESIAN_POINT ( 'NONE',  ( 3.054329744828568227, 6.785411478933790264, 0.000000000000000000 ) ) ;
#178100=CARTESIAN_POINT ( 'NONE',  ( -3.969505113751027547, 7.853116076009993840, 1.214306433183764966E-14 ) ) ;
#178103=CARTESIAN_POINT ( 'NONE',  ( 6.333067150914816423, 7.521571443223021625, 1.082531754730549967 ) ) ;
#178108=CARTESIAN_POINT ( 'NONE',  ( -6.330731382938325602, 6.350551133041632212, 0.7998128361456281477 ) ) ;
#178114=CARTESIAN_POINT ( 'NONE',  ( -3.797165540279144214, 6.587721009371067638, 1.199719254218452935 ) ) ;
#178119=CARTESIAN_POINT ( 'NONE',  ( -4.613517410400161722, 8.604463755433990002, -0.7998128361456362523 ) ) ;
#178129=CARTESIAN_POINT ( 'NONE',  ( -5.808742468812186033, 5.741564066561132940, 0.000000000000000000 ) ) ;
#178133=CARTESIAN_POINT ( 'NONE',  ( -4.990809943606269172, 8.836712344267034780, -0.7216878364870338292 ) ) ;
#178134=CARTESIAN_POINT ( 'NONE',  ( -7.729556973122450714, 8.190440354830551328, 0.000000000000000000 ) ) ;
#178135=CARTESIAN_POINT ( 'NONE',  ( 5.840530312436913007, 10.03597880781023299, 0.000000000000000000 ) ) ;
#178136=CARTESIAN_POINT ( 'NONE',  ( -5.447343857640614573, 9.577261277214532242, -0.7998128361456362523 ) ) ;
#178175=CARTESIAN_POINT ( 'NONE',  ( 4.596911992430688265, 8.487755744900498556, -0.08351877912710949092 ) ) ;
#178189=CARTESIAN_POINT ( 'NONE',  ( 7.035755370848908896, 7.173079118937375931, 0.7998128361456352531 ) ) ;
#178192=CARTESIAN_POINT ( 'NONE',  ( -4.573896719763875574, 6.429575154514868274, -1.599625672291271394 ) ) ;
#178195=B_SPLINE_CURVE_WITH_KNOTS ( 'NONE', 3,
 ( #213133, #81020, #195842, #12801, #13869, #47483 ),
 .UNSPECIFIED., .F., .F.,
 ( 4, 2, 4 ),
 ( 0.3194375178873440357, 0.4097251701830488813, 0.5000128224787536713 ),
 .UNSPECIFIED. ) ;
#178197=CARTESIAN_POINT ( 'NONE',  ( -7.227905289416814760, 7.605180057173966723, -0.7216878364870338292 ) ) ;
#178206=ADVANCED_FACE ( 'NONE', ( #57091 ), #42998, .F. ) ;
#178209=CARTESIAN_POINT ( 'NONE',  ( 3.562760505341037831, 7.378580699531681830, -1.734723475976807094E-15 ) ) ;
#178210=CARTESIAN_POINT ( 'NONE',  ( 7.028976294042106332, 7.165170195996068969, 0.000000000000000000 ) ) ;
#178225=CARTESIAN_POINT ( 'NONE',  ( 6.713222337422018349, 7.861122810861019161, -1.199719254218452047 ) ) ;
#178238=CARTESIAN_POINT ( 'NONE',  ( -5.804299160426249493, 5.944306240018289778, -0.7216878364870338292 ) ) ;
#178240=CARTESIAN_POINT ( 'NONE',  ( 4.258669648468268676, 7.982548666606070320, 0.7216878364870257245 ) ) ;
#178242=CARTESIAN_POINT ( 'NONE',  ( -4.888341132428297264, 4.880200397354325759, 0.5250896534725345566 ) ) ;
#178253=CARTESIAN_POINT ( 'NONE',  ( -5.478903473698241378, 9.406154796041011679, -0.7216878364870338292 ) ) ;
#178254=CARTESIAN_POINT ( 'NONE',  ( 7.095713291905693332, 9.371694488680407886, 1.599625672291268286 ) ) ;
#178257=CARTESIAN_POINT ( 'NONE',  ( 4.923019175093585886, 5.876515471431535076, -1.082531754730548412 ) ) ;
#178263=FACE_OUTER_BOUND ( 'NONE', #173331, .T. ) ;
#178270=CARTESIAN_POINT ( 'NONE',  ( -5.608757509019071108, 5.629766575900002401, 7.500000000000000000 ) ) ;
#178273=CARTESIAN_POINT ( 'NONE',  ( -6.111939103702986209, 6.385007292916157873, 0.4240853425246626229 ) ) ;
#178276=CARTESIAN_POINT ( 'NONE',  ( 4.766573523656222555, 7.718696989977711809, 1.199719254218452047 ) ) ;
#178278=CARTESIAN_POINT ( 'NONE',  ( -3.820365424000704557, 7.679119771301277098, -0.7998128361456481317 ) ) ;
#178293=CARTESIAN_POINT ( 'NONE',  ( 6.536439455564155843, 8.719208346281938304, 1.443375672974065660 ) ) ;
#178295=CARTESIAN_POINT ( 'NONE',  ( -6.095272577795516789, 9.268845886473535245, 1.199719254218452047 ) ) ;
#178296=CARTESIAN_POINT ( 'NONE',  ( 4.518610335104485287, 8.493738834255713854, 0.000000000000000000 ) ) ;
#178297=ORIENTED_EDGE ( 'NONE', *, *, #46978, .F. ) ;
#178305=CARTESIAN_POINT ( 'NONE',  ( -4.610654757099099221, 7.536791762327691657, 1.199719254218452935 ) ) ;
#178333=CARTESIAN_POINT ( 'NONE',  ( 4.828112100242277549, 6.726159765073026264, -1.443375672974068769 ) ) ;
#178339=CARTESIAN_POINT ( 'NONE',  ( 4.543390873910903238, 7.354354215321133204, 1.082531754730548412 ) ) ;
#178351=CARTESIAN_POINT ( 'NONE',  ( -5.712781623311813384, 7.758274208654143855, -1.599625672291271394 ) ) ;
#178353=CARTESIAN_POINT ( 'NONE',  ( -7.425025402139490360, 8.691559719698066289, 1.199719254218452047 ) ) ;
#178359=CARTESIAN_POINT ( 'NONE',  ( 8.011942431032855083, 8.311964022485323511, 0.7998128361456291469 ) ) ;
#178365=CARTESIAN_POINT ( 'NONE',  ( -5.098748287191073203, 8.106234214101666780, 1.199719254218452935 ) ) ;
#178371=CARTESIAN_POINT ( 'NONE',  ( -4.448483799059637533, 7.243629294661272588, 1.082531754730549967 ) ) ;
#178374=CARTESIAN_POINT ( 'NONE',  ( -5.309953438407606363, 6.223975762010839574, 1.199719254218452935 ) ) ;
#178393=CARTESIAN_POINT ( 'NONE',  ( -3.146901051703345331, 6.685485303713597283, 0.000000000000000000 ) ) ;
#178395=CARTESIAN_POINT ( 'NONE',  ( -3.983063267364693960, 7.868933921892603323, -0.7998128361456481317 ) ) ;
#178396=ORIENTED_EDGE ( 'NONE', *, *, #27277, .F. ) ;
#178420=CARTESIAN_POINT ( 'NONE',  ( -7.065734331377342414, 8.272386803808890576, -1.199719254218452047 ) ) ;
#178435=CIRCLE ( 'NONE', #161110, 0.08000000000000020983 ) ;
#178447=CARTESIAN_POINT ( 'NONE',  ( 8.167861197590044142, 8.493869250135347215, 0.000000000000000000 ) ) ;
#178448=CARTESIAN_POINT ( 'NONE',  ( -8.014278199453791274, 8.522615118883788199, 1.530808498934192557E-16 ) ) ;
#178460=CARTESIAN_POINT ( 'NONE',  ( 5.871284023695358734, 7.173991544917035945, 1.145568358895364458 ) ) ;
#178462=CARTESIAN_POINT ( 'NONE',  ( 7.187230829020130329, 7.557726520044554697, 0.7216878364870267237 ) ) ;
#178467=CARTESIAN_POINT ( 'NONE',  ( -5.309953438407606363, 6.223975762010839574, 1.199719254218452935 ) ) ;
#178472=CARTESIAN_POINT ( 'NONE',  ( -6.739811759324831897, 7.996106819701333634, -1.082531754730549967 ) ) ;
#178481=CARTESIAN_POINT ( 'NONE',  ( -3.797165540279144214, 6.587721009371067638, 1.199719254218452935 ) ) ;
#178491=CARTESIAN_POINT ( 'NONE',  ( 7.126746022638799971, 8.343567110280638133, 1.199719254218452047 ) ) ;
#178512=CARTESIAN_POINT ( 'NONE',  ( 5.559725510055676168, 8.644040974110419384, 1.199719254218451159 ) ) ;
#178513=CIRCLE ( 'NONE', #151008, 0.08000000000000020983 ) ;
#178514=DIRECTION ( 'NONE',  ( 0.000000000000000000, 1.000000000000000000, 0.000000000000000000 ) ) ;
#178515=CARTESIAN_POINT ( 'NONE',  ( -6.353279334749129426, 6.853861929151015886, 0.6383911273219675664 ) ) ;
#178522=CARTESIAN_POINT ( 'NONE',  ( 4.797606254389322089, 6.690569611577942943, 1.599625672291268286 ) ) ;
#178530=CARTESIAN_POINT ( 'NONE',  ( 5.099275172515607579, 5.121778254122544283, -0.7216878364870458196 ) ) ;
#178532=DIRECTION ( 'NONE',  ( -0.000000000000000000, -0.000000000000000000, -1.000000000000000000 ) ) ;
#178533=CARTESIAN_POINT ( 'NONE',  ( 6.048345925472183637, 8.149765894507963182, 1.443375672974065660 ) ) ;
#178544=CARTESIAN_POINT ( 'NONE',  ( -6.794044374223859428, 7.099008989448849505, 0.000000000000000000 ) ) ;
#178566=AXIS2_PLACEMENT_3D ( 'NONE', #89630, #37657, #87482 ) ;
#178569=CARTESIAN_POINT ( 'NONE',  ( -4.370663978927087356, 5.060324124126027279, 2.420000000000000373 ) ) ;
#178573=LINE ( 'NONE', #65839, #68696 ) ;
#178580=CARTESIAN_POINT ( 'NONE',  ( 5.071631979963703962, 8.074598522336444262, 1.199719254218451159 ) ) ;
#178582=CARTESIAN_POINT ( 'NONE',  ( 4.525389411911321602, 8.501647757197021704, -0.7998128361456381397 ) ) ;
#178594=CARTESIAN_POINT ( 'NONE',  ( -6.400857919427531684, 9.521399101757175742, 1.082531754730549967 ) ) ;
#178597=CARTESIAN_POINT ( 'NONE',  ( 5.411112705185558092, 6.445957923205511086, -1.082531754730548412 ) ) ;
#178613=CARTESIAN_POINT ( 'NONE',  ( -6.509323148336870091, 7.727203440215372865, 1.082531754730549078 ) ) ;
#178614=EDGE_LOOP ( 'NONE', ( #72440, #128042, #183592, #186055 ) ) ;
#178615=CARTESIAN_POINT ( 'NONE',  ( -5.966997003790240228, 6.134120390609613338, -0.7216878364870338292 ) ) ;
#178643=CARTESIAN_POINT ( 'NONE',  ( 5.581281513216643120, 5.830910960256830755, -0.7657042079148683733 ) ) ;
#178651=CARTESIAN_POINT ( 'NONE',  ( -7.208094944320834863, 8.438474185576302133, -1.199719254218452047 ) ) ;
#178652=CARTESIAN_POINT ( 'NONE',  ( -4.594589183792981757, 8.486487934283967860, 0.2047448450237729367 ) ) ;
#178658=DIRECTION ( 'NONE',  ( 2.664535259100375697E-15, 0.000000000000000000, -1.000000000000000000 ) ) ;
#178660=CARTESIAN_POINT ( 'NONE',  ( -5.004894982100124068, 5.868074229652107121, 1.199719254218452935 ) ) ;
#178663=CARTESIAN_POINT ( 'NONE',  ( -3.630551273409382329, 7.457669928944732796, 0.7998128361456352531 ) ) ;
#178673=CARTESIAN_POINT ( 'NONE',  ( 4.278479993564246797, 7.149254538203735798, 1.199719254218452047 ) ) ;
#178698=EDGE_CURVE ( 'NONE', #128658, #207594, #18365, .T. ) ;
#178699=CARTESIAN_POINT ( 'NONE',  ( 6.554440917563797875, 6.611545590104705994, -0.7998128361456481317 ) ) ;
#178700=CARTESIAN_POINT ( 'NONE',  ( 4.329849954717849947, 6.144853928627882489, 1.599625672291262513 ) ) ;
#178702=FACE_OUTER_BOUND ( 'NONE', #77525, .T. ) ;
#178714=CARTESIAN_POINT ( 'NONE',  ( 4.602896574056089207, 8.480248385054199645, 0.1803159889683242367 ) ) ;
#178715=CARTESIAN_POINT ( 'NONE',  ( -6.143253000323532831, 7.300121600866474658, 1.082531754730548412 ) ) ;
#178738=CARTESIAN_POINT ( 'NONE',  ( -5.608478439449225306, 5.609308656285654671, -0.4224404339892348093 ) ) ;
#178745=CARTESIAN_POINT ( 'NONE',  ( 5.391302360089590628, 6.318882837306503575, -1.199719254218452047 ) ) ;
#178756=CARTESIAN_POINT ( 'NONE',  ( -7.065207446497166366, 9.336104335703744539, 0.000000000000000000 ) ) ;
#178766=CARTESIAN_POINT ( 'NONE',  ( -6.583366107887490770, 9.838288338247510367, 1.199719254218452935 ) ) ;
#178778=CARTESIAN_POINT ( 'NONE',  ( 4.505052181490820651, 8.477920988373101707, -0.7998128361456381397 ) ) ;
#178783=CARTESIAN_POINT ( 'NONE',  ( 6.062430963966053632, 7.101866208495718702, -1.199719254218452047 ) ) ;
#178793=CARTESIAN_POINT ( 'NONE',  ( 4.596835240751270035, 8.371391889155539445, -0.09823007671119071693 ) ) ;
#178815=CARTESIAN_POINT ( 'NONE',  ( -4.796552484184649856, 8.818004674849227342, -0.7998128361456362523 ) ) ;
#178817=CARTESIAN_POINT ( 'NONE',  ( 6.412080304620304538, 6.445458208337293549, -0.7998128361456481317 ) ) ;
#178820=CARTESIAN_POINT ( 'NONE',  ( 2.449293598294706414E-16, 0.08000000000000020983, 2.000000000000000000 ) ) ;
#178822=CARTESIAN_POINT ( 'NONE',  ( -5.399890319992785237, 9.521898816625391504, 0.7998128361456291469 ) ) ;
#178842=CARTESIAN_POINT ( 'NONE',  ( 5.303878726007847710, 4.755038592612019777, 2.500000000000000000 ) ) ;
#178848=CARTESIAN_POINT ( 'NONE',  ( 4.584065335196252811, 8.362176967788721882, 0.7216878364870328300 ) ) ;
#178863=CARTESIAN_POINT ( 'NONE',  ( -4.909461021924285795, 6.821066840368686712, 1.443375672974058777 ) ) ;
#178866=CARTESIAN_POINT ( 'NONE',  ( 5.086243903782109221, 5.962981304947771122, -1.199719254218452047 ) ) ;
#178884=CARTESIAN_POINT ( 'NONE',  ( 7.526184668917440312, 8.913541880892736913, -1.082531754730548412 ) ) ;
#178907=CARTESIAN_POINT ( 'NONE',  ( 3.607878275012313285, 6.262922849939428716, 1.082531754730549078 ) ) ;
#178915=CARTESIAN_POINT ( 'NONE',  ( -3.147653791585729444, 8.999999999999998224, -2.419999999999998597 ) ) ;
#178917=CARTESIAN_POINT ( 'NONE',  ( -5.790741006368224753, 5.928488393617260321, 0.7216878364870257245 ) ) ;
#178918=CARTESIAN_POINT ( 'NONE',  ( 4.580108180932601414, 8.499999999999996447, -0.1719113009628105149 ) ) ;
#178923=CARTESIAN_POINT ( 'NONE',  ( -6.771371375382467583, 6.864631124226471037, -0.7998128361456362523 ) ) ;
#178932=CARTESIAN_POINT ( 'NONE',  ( 5.982890925380405456, 10.20206618957764100, 0.000000000000000000 ) ) ;
#178933=CARTESIAN_POINT ( 'NONE',  ( -5.991777542596674166, 5.955104985976372944, 0.000000000000000000 ) ) ;
#178935=ORIENTED_EDGE ( 'NONE', *, *, #115968, .T. ) ;
#178936=CARTESIAN_POINT ( 'NONE',  ( 6.308853223578811509, 6.964933332891984463, 0.9108697706533327443 ) ) ;
#178941=CARTESIAN_POINT ( 'NONE',  ( 6.204791576909545192, 7.267953590263130259, -1.199719254218452047 ) ) ;
#178950=CARTESIAN_POINT ( 'NONE',  ( -5.655686355556086120, 6.627330832017406692, 1.199719254218452935 ) ) ;
#178954=CARTESIAN_POINT ( 'NONE',  ( -5.822300622425855110, 5.757381912443740646, 0.7998128361456281477 ) ) ;
#178957=CARTESIAN_POINT ( 'NONE',  ( 7.336370518326124746, 7.731722824234849689, -0.7216878364870317197 ) ) ;
#178959=CARTESIAN_POINT ( 'NONE',  ( -7.255021596644144921, 7.636815748939187465, 0.7216878364870317197 ) ) ;
#178965=CARTESIAN_POINT ( 'NONE',  ( 5.391302360089590628, 6.318882837306503575, -1.199719254218452047 ) ) ;
#178973=CARTESIAN_POINT ( 'NONE',  ( 4.854701522145073334, 7.821512988214679218, -1.199719254218450271 ) ) ;
#179002=CARTESIAN_POINT ( 'NONE',  ( 7.856023664475727308, 8.130058794835305136, -0.7998128361456341429 ) ) ;
#179004=EDGE_LOOP ( 'NONE', ( #17409, #161632, #109033, #25449 ) ) ;
#179008=CARTESIAN_POINT ( 'NONE',  ( -6.329889402343163773, 6.869280899661572626, -0.6830204514151876349 ) ) ;
#179014=CARTESIAN_POINT ( 'NONE',  ( -3.621436428181653788, 7.239109909604962922, 0.7216878364870338292 ) ) ;
#179024=CARTESIAN_POINT ( 'NONE',  ( -3.980200614063634568, 6.801261928786307642, 1.199719254218452935 ) ) ;
#179026=CARTESIAN_POINT ( 'NONE',  ( 7.635176783151273128, 8.936736330878529699, 1.199719254218452935 ) ) ;
#179029=VERTEX_POINT ( 'NONE', #201766 ) ;
#179034=CARTESIAN_POINT ( 'NONE',  ( 6.039231080244466199, 6.010467446565510130, 0.7998128361456352531 ) ) ;
#179037=CARTESIAN_POINT ( 'NONE',  ( 6.522881301506172846, 6.782652071278222117, -0.7216878364870458196 ) ) ;
#179040=VERTEX_POINT ( 'NONE', #53406 ) ;
#179051=CARTESIAN_POINT ( 'NONE',  ( -5.309953438407606363, 6.223975762010839574, 1.199719254218452935 ) ) ;
#179052=CARTESIAN_POINT ( 'NONE',  ( 3.366167277942881064, 7.149221934233827014, -0.7998128361456362523 ) ) ;
#179063=CARTESIAN_POINT ( 'NONE',  ( -5.855142236255304944, 7.924361590421551860, -1.599625672291271394 ) ) ;
#179064=CARTESIAN_POINT ( 'NONE',  ( 6.692885107001518286, 7.837396042037102717, -1.199719254218452047 ) ) ;
#179077=CARTESIAN_POINT ( 'NONE',  ( -6.449404147558570166, 6.867377544759197150, 0.7074503392771516186 ) ) ;
#179084=DIRECTION ( 'NONE',  ( 0.7592566023652995710, 0.6507913734559650498, 0.000000000000000000 ) ) ;
#179085=CARTESIAN_POINT ( 'NONE',  ( -4.678972410047611774, 5.591794245544547515, 1.082531754730549078 ) ) ;
#179100=CARTESIAN_POINT ( 'NONE',  ( 5.318541398310776103, 9.426991741329731056, -0.7998128361456481317 ) ) ;
#179133=CARTESIAN_POINT ( 'NONE',  ( 3.932747076415766596, 6.745899468197171345, 1.199719254218451159 ) ) ;
#179136=FACE_OUTER_BOUND ( 'NONE', #84261, .T. ) ;
#179165=CARTESIAN_POINT ( 'NONE',  ( -6.303615075710993665, 6.318915441276411471, -0.7998128361456362523 ) ) ;
#179167=CARTESIAN_POINT ( 'NONE',  ( 6.387299765369506055, 7.584842826753462219, -1.082531754730548412 ) ) ;
#179172=CARTESIAN_POINT ( 'NONE',  ( -4.956387674247580755, 7.940146832334256111, 1.199719254218452935 ) ) ;
#179177=CARTESIAN_POINT ( 'NONE',  ( -3.772911886352873445, 7.623757310712140800, 0.7998128361456352531 ) ) ;
#179178=TOROIDAL_SURFACE ( 'NONE', #23605, 3.970406073902761790, 0.08000000000000000167 ) ;
#179183=CARTESIAN_POINT ( 'NONE',  ( -6.231907884136888676, 7.299589282028351001, -1.199719254218453823 ) ) ;
#179196=CARTESIAN_POINT ( 'NONE',  ( -5.469788628470539926, 5.346117919495872783, -0.7998128361456362523 ) ) ;
#179199=CARTESIAN_POINT ( 'NONE',  ( -4.828112100242279325, 8.646898193675708555, -0.7216878364870338292 ) ) ;
#179200=CARTESIAN_POINT ( 'NONE',  ( -7.390603132780803719, 7.794994207765291172, -0.7216878364870338292 ) ) ;
#179201=CARTESIAN_POINT ( 'NONE',  ( 6.607619761813720238, 8.802252036906432764, 1.599625672291268286 ) ) ;
#179203=CARTESIAN_POINT ( 'NONE',  ( -7.306918443122272677, 7.489436036589583345, 0.7998128361456341429 ) ) ;
#179215=ORIENTED_EDGE ( 'NONE', *, *, #190788, .T. ) ;
#179221=CARTESIAN_POINT ( 'NONE',  ( -1.858076449550070564, 2.486042365337548521, -2.481448873923816745 ) ) ;
#179234=CIRCLE ( 'NONE', #16541, 0.08000000000000012657 ) ;
#179241=CARTESIAN_POINT ( 'NONE',  ( 5.213898493288036562, 7.712005038449616379, -1.200564631081424416 ) ) ;
#179257=CARTESIAN_POINT ( 'NONE',  ( 6.737475991348287785, 6.825086509519945999, -0.7998128361456481317 ) ) ;
#179260=CARTESIAN_POINT ( 'NONE',  ( -5.113360211009450040, 5.994616996712990975, -1.199719254218453823 ) ) ;
#179264=CARTESIAN_POINT ( 'NONE',  ( -6.956742217143487395, 8.249192353823097790, 1.082531754730549078 ) ) ;
#179275=CARTESIAN_POINT ( 'NONE',  ( 4.411198876399872404, 6.239761003923544713, -1.599625672291273171 ) ) ;
#179277=CARTESIAN_POINT ( 'NONE',  ( 5.182959862174088883, 9.268813282503625572, 0.7998128361456331437 ) ) ;
#179286=CARTESIAN_POINT ( 'NONE',  ( 3.088225128862704949, 6.824956093640315302, 0.7998128361456281477 ) ) ;
#179292=CARTESIAN_POINT ( 'NONE',  ( 6.875920180786008196, 8.050936961452347163, -1.199719254218452047 ) ) ;
#179306=CARTESIAN_POINT ( 'NONE',  ( -4.611181642423629157, 7.433443445252599702, 1.082531754730549967 ) ) ;
#179307=CARTESIAN_POINT ( 'NONE',  ( 5.885648082108200896, 6.039213315313952002, 0.7216878364870328300 ) ) ;
#179309=CARTESIAN_POINT ( 'NONE',  ( -4.902494178016985060, 4.880919686651536082, 0.5424932267784847717 ) ) ;
#179319=CARTESIAN_POINT ( 'NONE',  ( -7.268579750702160780, 8.613002809641560731, -1.082531754730549967 ) ) ;
#179320=CARTESIAN_POINT ( 'NONE',  ( 7.849244587668864348, 8.122149871893999062, 0.7998128361456291469 ) ) ;
#179323=CARTESIAN_POINT ( 'NONE',  ( 6.021229617800532452, 6.197391773621639288, 0.000000000000000000 ) ) ;
#179341=CARTESIAN_POINT ( 'NONE',  ( 5.143339171537801846, 7.093924681584509173, 1.599625672291269396 ) ) ;
#179343=CARTESIAN_POINT ( 'NONE',  ( -3.481411583659053566, 7.283673624236017830, 0.000000000000000000 ) ) ;
#179354=CARTESIAN_POINT ( 'NONE',  ( 7.078765600110826561, 8.391552967285011988, -1.082531754730548412 ) ) ;
#179356=CARTESIAN_POINT ( 'NONE',  ( -4.945692173934974178, 8.992000979557944973, 0.000000000000000000 ) ) ;
#179357=CARTESIAN_POINT ( 'NONE',  ( 5.180097208873055692, 8.201141289397330780, -1.199719254218450271 ) ) ;
#179366=CARTESIAN_POINT ( 'NONE',  ( -5.098748287191073203, 8.106234214101666780, 1.199719254218452935 ) ) ;
#179396=CARTESIAN_POINT ( 'NONE',  ( 4.367134877377630175, 7.148722219365612141, -1.082531754730548412 ) ) ;
#179397=ORIENTED_EDGE ( 'NONE', *, *, #132097, .T. ) ;
#179402=CARTESIAN_POINT ( 'NONE',  ( 5.275531169048895741, 7.248148678680751189, -1.443375672974078761 ) ) ;
#179414=CARTESIAN_POINT ( 'NONE',  ( -6.805266759416629618, 6.904175738932996964, 0.000000000000000000 ) ) ;
#179416=CARTESIAN_POINT ( 'NONE',  ( -5.752402313948099533, 9.933162809573264695, -0.7998128361456362523 ) ) ;
#179423=CARTESIAN_POINT ( 'NONE',  ( 6.003228155800906407, 10.22579295840155744, 0.000000000000000000 ) ) ;
#179428=CARTESIAN_POINT ( 'NONE',  ( -4.762657100150483380, 8.778460060142702304, 0.000000000000000000 ) ) ;
#179434=CARTESIAN_POINT ( 'NONE',  ( -5.994113311017573054, 6.165756082374834079, 0.7216878364870257245 ) ) ;
#179438=CARTESIAN_POINT ( 'NONE',  ( -5.285699784481336927, 7.260012063351913625, 1.599625672291263179 ) ) ;
#179444=CARTESIAN_POINT ( 'NONE',  ( -5.790741006368233634, 5.928488393617254992, 0.7216878364870203955 ) ) ;
#179456=CARTESIAN_POINT ( 'NONE',  ( -6.149505192250180663, 9.332117270003974951, -1.199719254218452047 ) ) ;
#179459=CARTESIAN_POINT ( 'NONE',  ( -7.130662446144611977, 7.283804040115648526, 0.000000000000000000 ) ) ;
#179478=ORIENTED_EDGE ( 'NONE', *, *, #25456, .F. ) ;
#179481=DIRECTION ( 'NONE',  ( -0.8271092603138155974, 0.5620411653100980676, 1.333541550007727027E-12 ) ) ;
#179486=CARTESIAN_POINT ( 'NONE',  ( -7.795011973214244883, 8.058878488363559356, 0.7998128361456341429 ) ) ;
#179512=CARTESIAN_POINT ( 'NONE',  ( 8.188198428010544205, 8.517596018959260107, 0.000000000000000000 ) ) ;
#179513=CARTESIAN_POINT ( 'NONE',  ( 6.047819040147648373, 9.213483425884394507, 1.199719254218452047 ) ) ;
#179527=CARTESIAN_POINT ( 'NONE',  ( 6.198956711081595294, 6.941498593865138567, 0.8670033951987624610 ) ) ;
#179529=CARTESIAN_POINT ( 'NONE',  ( 4.146814880933355596, 5.931313009212638931, 1.599625672291261402 ) ) ;
#179534=CARTESIAN_POINT ( 'NONE',  ( -4.773352600463090845, 7.726605912919016106, 1.199719254218452935 ) ) ;
#179539=CARTESIAN_POINT ( 'NONE',  ( -6.238160075619175515, 10.29195416494877513, 0.000000000000000000 ) ) ;
#179546=CARTESIAN_POINT ( 'NONE',  ( -5.632486471834530661, 5.535932070087196344, -0.7998128361456362523 ) ) ;
#179556=CARTESIAN_POINT ( 'NONE',  ( 4.329849954717849947, 6.144853928627882489, 1.599625672291262513 ) ) ;
#179579=CARTESIAN_POINT ( 'NONE',  ( 6.367489420273535039, 7.457767740854454708, -1.199719254218452047 ) ) ;
#179581=CARTESIAN_POINT ( 'NONE',  ( -5.130090819275266334, 7.806487709571898748, 1.156910012491520590 ) ) ;
#179587=CARTESIAN_POINT ( 'NONE',  ( 5.716698046817569434, 6.698511138489155137, -1.199719254218452047 ) ) ;
#179594=CARTESIAN_POINT ( 'NONE',  ( 4.923019175537949543, 4.916146257648610352, 0.000000000000000000 ) ) ;
#179597=CARTESIAN_POINT ( 'NONE',  ( 5.506019780925567986, 8.477421273504887722, -1.082531754730548412 ) ) ;
#179602=CARTESIAN_POINT ( 'NONE',  ( 2.449293598294706414E-16, 9.999999999999998224, 2.000000000000000000 ) ) ;
#179608=CARTESIAN_POINT ( 'NONE',  ( -4.326460416536637155, 8.061637896019123062, 0.000000000000000000 ) ) ;
#179615=CARTESIAN_POINT ( 'NONE',  ( 4.245111494854632461, 7.966730820723463502, 0.000000000000000000 ) ) ;
#179645=CARTESIAN_POINT ( 'NONE',  ( 5.987861119090863049, 7.014868056141362551, 1.199719254218452047 ) ) ;
#179647=CARTESIAN_POINT ( 'NONE',  ( 4.538947565524982686, 8.517465603079630299, 0.000000000000000000 ) ) ;
#179659=CARTESIAN_POINT ( 'NONE',  ( -3.363304624641834106, 6.081549941127532222, -1.199719254218452047 ) ) ;
#179662=CARTESIAN_POINT ( 'NONE',  ( 5.248414861821569133, 6.256143772614186638, -1.082531754730548412 ) ) ;
#179675=CARTESIAN_POINT ( 'NONE',  ( -6.794044374223859428, 7.099008989448849505, 0.000000000000000000 ) ) ;
#179677=CARTESIAN_POINT ( 'NONE',  ( -4.163762573172648196, 7.871823745427799501, 0.000000000000000000 ) ) ;
#179680=FACE_OUTER_BOUND ( 'NONE', #83595, .T. ) ;
#179682=CARTESIAN_POINT ( 'NONE',  ( 2.889872605471108802, 6.605953636083950364, -2.420000000000002149 ) ) ;
#179685=CARTESIAN_POINT ( 'NONE',  ( -5.807688785661975217, 6.901678836137074668, -1.092232961817845904 ) ) ;
#179693=B_SPLINE_CURVE_WITH_KNOTS ( 'NONE', 3,
 ( #138754, #22825, #119352, #5498, #118285, #38044 ),
 .UNSPECIFIED., .F., .F.,
 ( 4, 2, 4 ),
 ( 0.0001064780297606581909, 0.0003688581118774151668, 0.0006312381939941720749 ),
 .UNSPECIFIED. ) ;
#179707=CARTESIAN_POINT ( 'NONE',  ( -4.736594563127865420, 6.619389305106191834, -1.599625672291271394 ) ) ;
#179717=CARTESIAN_POINT ( 'NONE',  ( -6.668631453075260396, 8.873432343378178544, -1.599625672291271394 ) ) ;
#179718=CARTESIAN_POINT ( 'NONE',  ( -5.840188366348757931, 7.302172906674928576, 1.289283945506283890 ) ) ;
#179721=ORIENTED_EDGE ( 'NONE', *, *, #130414, .T. ) ;
#179723=CARTESIAN_POINT ( 'NONE',  ( -7.146556367734805626, 9.431011410480991231, 1.443375672974064550 ) ) ;
#179726=CARTESIAN_POINT ( 'NONE',  ( -3.494969737272722643, 7.299491470118629088, -0.7998128361456481317 ) ) ;
#179739=CARTESIAN_POINT ( 'NONE',  ( 4.929271367020211514, 7.908511140569038922, 1.199719254218452047 ) ) ;
#179763=CARTESIAN_POINT ( 'NONE',  ( 5.234329823327693809, 8.264412672927770487, 1.199719254218451159 ) ) ;
#179764=CARTESIAN_POINT ( 'NONE',  ( 5.734172623936983904, 5.654565914206774124, 0.7998128361456352531 ) ) ;
#179766=CARTESIAN_POINT ( 'NONE',  ( 4.903208829997618423, 5.749440385532527564, -1.199719254218450271 ) ) ;
#179776=CARTESIAN_POINT ( 'NONE',  ( 5.371503168974233411, 7.687194297833679357, 1.321221623412481394 ) ) ;
#179777=CARTESIAN_POINT ( 'NONE',  ( -5.438229012412899799, 7.437962829272074750, -1.443375672974066548 ) ) ;
#179803=CARTESIAN_POINT ( 'NONE',  ( 5.825163275726873202, 6.825053905550038991, 1.199719254218452047 ) ) ;
#179813=DIRECTION ( 'NONE',  ( 1.224646799147349509E-16, 0.000000000000000000, -1.000000000000000000 ) ) ;
#179834=CARTESIAN_POINT ( 'NONE',  ( 5.342795052237045539, 8.390955439988655229, -1.199719254218450271 ) ) ;
#179838=CARTESIAN_POINT ( 'NONE',  ( 4.376249722160992839, 8.327651452488305850, 0.000000000000000000 ) ) ;
#179849=CARTESIAN_POINT ( 'NONE',  ( 4.700249516990034238, 8.244041944096728969, -0.6212051699984559860 ) ) ;
#179863=CARTESIAN_POINT ( 'NONE',  ( -5.992450215256712731, 7.101132044915781982, 1.073800501374306382 ) ) ;
#179866=CARTESIAN_POINT ( 'NONE',  ( 2.957086901556340575, 6.464035461875470290, 0.7216878364870257245 ) ) ;
#179867=VERTEX_POINT ( 'NONE', #45720 ) ;
#179871=CARTESIAN_POINT ( 'NONE',  ( -6.363572996767778100, 8.517530811019446091, -1.599625672291271394 ) ) ;
#179873=CARTESIAN_POINT ( 'NONE',  ( 6.900173834712277632, 7.014900660111269559, -0.7998128361456341429 ) ) ;
#179875=CARTESIAN_POINT ( 'NONE',  ( 3.761726504036865926, 7.402781664769409353, 0.2506311418687352521 ) ) ;
#179877=CARTESIAN_POINT ( 'NONE',  ( -7.774674742793745708, 8.035151719539642912, 0.7998128361456341429 ) ) ;
#179885=CARTESIAN_POINT ( 'NONE',  ( -0.3551009713840111437, 2.785693601408736342, -1.969347843778241458 ) ) ;
#179890=ADVANCED_FACE ( 'NONE', ( #29456 ), #125394, .T. ) ;
#179894=EDGE_CURVE ( 'NONE', #93819, #133393, #88100, .T. ) ;
#179902=CARTESIAN_POINT ( 'NONE',  ( 5.668717624289557833, 8.667235424096215723, -1.082531754730548412 ) ) ;
#179918=CARTESIAN_POINT ( 'NONE',  ( -5.478903473698260029, 6.525047153136981137, -1.082531754730549967 ) ) ;
#179920=CARTESIAN_POINT ( 'NONE',  ( 6.561219994370630637, 6.619454513046008515, 0.000000000000000000 ) ) ;
#179934=CARTESIAN_POINT ( 'NONE',  ( -1.886825320689270225, 2.480000000000016858, 2.459652456995881753 ) ) ;
#179962=CARTESIAN_POINT ( 'NONE',  ( -3.719872605471121751, 6.605953636083950364, 2.420000000000000373 ) ) ;
#179974=CARTESIAN_POINT ( 'NONE',  ( -5.492461626867567226, 6.540864998501174199, 1.082531754730549078 ) ) ;
#179980=CARTESIAN_POINT ( 'NONE',  ( -5.960744811863571968, 6.983232364376142698, 1.199719254218452935 ) ) ;
#179985=VERTEX_POINT ( 'NONE', #208093 ) ;
#179987=CARTESIAN_POINT ( 'NONE',  ( 6.994027139803230320, 9.253060644560830994, -1.599625672291267398 ) ) ;
#179988=CARTESIAN_POINT ( 'NONE',  ( -5.818384198920079520, 6.817144982608731141, 1.199719254218452935 ) ) ;
#179990=ORIENTED_EDGE ( 'NONE', *, *, #30406, .F. ) ;
#179991=CARTESIAN_POINT ( 'NONE',  ( 6.509182584184366682, 6.829728176725765820, 0.5468608461018635847 ) ) ;
#179996=CARTESIAN_POINT ( 'NONE',  ( 4.830447868218803897, 8.857549289555754157, -0.7998128361456481317 ) ) ;
#180005=CARTESIAN_POINT ( 'NONE',  ( -3.817502770699643388, 6.611447778194983194, 1.199719254218452935 ) ) ;
#180009=CARTESIAN_POINT ( 'NONE',  ( -6.936931872047518155, 8.122117267924091166, 1.199719254218452047 ) ) ;
#180014=CARTESIAN_POINT ( 'NONE',  ( 5.492461626867537916, 9.421972641405202964, -0.7216878364870458196 ) ) ;
#180016=CARTESIAN_POINT ( 'NONE',  ( -6.522881301506166629, 9.663759714182251770, 1.082531754730549967 ) ) ;
#180022=CARTESIAN_POINT ( 'NONE',  ( 5.529746549527311039, 7.544733289238903851, -1.599625672291281386 ) ) ;
#180025=CARTESIAN_POINT ( 'NONE',  ( -4.940331642637891818, 4.884205503302849749, 0.5202640082965306334 ) ) ;
#180051=CARTESIAN_POINT ( 'NONE',  ( 4.759808938472720463, 8.174556087920027636, -0.7576060450402433144 ) ) ;
#180056=CARTESIAN_POINT ( 'NONE',  ( -2.923191517300036679, 6.424490846909734820, 0.000000000000000000 ) ) ;
#180064=CARTESIAN_POINT ( 'NONE',  ( -5.779986827147332029, 7.257483166437310729, -1.191988747605486010 ) ) ;
#180067=ORIENTED_EDGE ( 'NONE', *, *, #173168, .T. ) ;
#180071=CARTESIAN_POINT ( 'NONE',  ( -5.167065940139584868, 6.161236697318522637, 1.082531754730549078 ) ) ;
#180082=CARTESIAN_POINT ( 'NONE',  ( -3.142457743317409680, 6.888227477170756785, 0.7998128361456352531 ) ) ;
#180086=DIRECTION ( 'NONE',  ( 0.000000000000000000, 1.000000000000000000, 0.000000000000000000 ) ) ;
#180093=CARTESIAN_POINT ( 'NONE',  ( 6.391743074199808916, 6.421731439513382433, -0.7998128361456481317 ) ) ;
#180096=CARTESIAN_POINT ( 'NONE',  ( 6.821160681006788629, 8.091013894996997635, 1.082531754730549967 ) ) ;
#180099=ORIENTED_EDGE ( 'NONE', *, *, #140054, .F. ) ;
#180103=DIRECTION ( 'NONE',  ( 0.000000000000000000, 0.000000000000000000, 1.000000000000000000 ) ) ;
#180111=CARTESIAN_POINT ( 'NONE',  ( -4.773352600463090845, 7.726605912919016106, 1.199719254218452935 ) ) ;
#180112=CARTESIAN_POINT ( 'NONE',  ( 3.770049233051776749, 6.556085317605844232, 1.199719254218451159 ) ) ;
#180122=CARTESIAN_POINT ( 'NONE',  ( -5.101610940492132151, 9.173906207207963348, -0.7998128361456362523 ) ) ;
#180123=CARTESIAN_POINT ( 'NONE',  ( 6.964048179274811012, 8.153752959689313684, 1.199719254218452047 ) ) ;
#180130=CARTESIAN_POINT ( 'NONE',  ( 4.041212305325117882, 6.872442235258051646, -1.199719254218448494 ) ) ;
#180136=CARTESIAN_POINT ( 'NONE',  ( -6.615421019548638704, 6.757903343899189785, 0.08170615477586136433 ) ) ;
#180146=CARTESIAN_POINT ( 'NONE',  ( -8.106849506328558164, 8.422688943663599659, 0.000000000000000000 ) ) ;
#180147=CARTESIAN_POINT ( 'NONE',  ( -5.289089322662584358, 5.343228095960675716, 0.000000000000000000 ) ) ;
#180161=ORIENTED_EDGE ( 'NONE', *, *, #183755, .T. ) ;
#180199=CARTESIAN_POINT ( 'NONE',  ( 7.838022202476093270, 8.316983122409855156, 0.7216878364870267237 ) ) ;
#180200=CARTESIAN_POINT ( 'NONE',  ( -4.828112100242303306, 4.805421336470338645, -0.7216878364870338292 ) ) ;
#180228=CARTESIAN_POINT ( 'NONE',  ( -5.119085517611572378, 8.129960982925583224, 1.199719254218452935 ) ) ;
#180230=CARTESIAN_POINT ( 'NONE',  ( 7.336370518326124746, 7.731722824234849689, -0.7216878364870317197 ) ) ;
#180235=CARTESIAN_POINT ( 'NONE',  ( -6.143779885648060102, 7.196773283791382703, 1.199719254218452047 ) ) ;
#180243=CARTESIAN_POINT ( 'NONE',  ( -4.762657100150483380, 8.778460060142702304, 0.000000000000000000 ) ) ;
#180255=CARTESIAN_POINT ( 'NONE',  ( -4.773352600463090845, 7.726605912919016106, 1.199719254218452935 ) ) ;
#180259=CARTESIAN_POINT ( 'NONE',  ( -7.932929277771797238, 8.427708043588125975, 0.000000000000000000 ) ) ;
#180261=CARTESIAN_POINT ( 'NONE',  ( -7.065207446052813367, 8.375735120883982532, -1.082531754730549967 ) ) ;
#180262=CARTESIAN_POINT ( 'NONE',  ( 7.364013710877980401, 8.620379413226322285, -1.199719254218452047 ) ) ;
#180263=CARTESIAN_POINT ( 'NONE',  ( -6.420668264523499147, 9.648474187656182366, 1.199719254218452935 ) ) ;
#180302=CARTESIAN_POINT ( 'NONE',  ( 6.157602363183391603, 6.969851231138187941, -0.9158007892692658913 ) ) ;
#180315=CARTESIAN_POINT ( 'NONE',  ( 6.688968683495743583, 8.897159112202094988, -1.599625672291283607 ) ) ;
#180318=CARTESIAN_POINT ( 'NONE',  ( -5.679940009482361774, 5.591294530676332641, 0.7998128361456281477 ) ) ;
#180330=CARTESIAN_POINT ( 'NONE',  ( 3.237364818613055473, 6.998952398349030268, -1.734723475976807094E-15 ) ) ;
#180332=CARTESIAN_POINT ( 'NONE',  ( 7.180978637093494044, 8.406838493811077839, -1.199719254218452047 ) ) ;
#180340=CARTESIAN_POINT ( 'NONE',  ( -5.085717018457573957, 8.947437264926888290, 0.7216878364870267237 ) ) ;
#180346=ORIENTED_EDGE ( 'NONE', *, *, #83296, .F. ) ;
#180347=CARTESIAN_POINT ( 'NONE',  ( 6.688968683495743583, 8.897159112202094988, -1.599625672291283607 ) ) ;
#180358=CARTESIAN_POINT ( 'NONE',  ( -6.970300371201519241, 7.304640985922785212, 0.7216878364870317197 ) ) ;
#180359=CARTESIAN_POINT ( 'NONE',  ( 4.692530564105613422, 7.528350520548263702, -1.082531754730548412 ) ) ;
#180368=ORIENTED_EDGE ( 'NONE', *, *, #43321, .T. ) ;
#180370=CARTESIAN_POINT ( 'NONE',  ( -6.292392690518209264, 8.434487120394948079, -1.443375672974066548 ) ) ;
#180371=CARTESIAN_POINT ( 'NONE',  ( 6.933015448541703485, 9.181880338089085214, 1.599625672291268286 ) ) ;
#180375=CARTESIAN_POINT ( 'NONE',  ( 4.787437638956922648, 6.678706226906775179, -1.443375672974068769 ) ) ;
#180377=ORIENTED_EDGE ( 'NONE', *, *, #22239, .F. ) ;
#180393=CARTESIAN_POINT ( 'NONE',  ( -3.494969737272722643, 7.299491470118629088, -0.7998128361456481317 ) ) ;
#180408=CARTESIAN_POINT ( 'NONE',  ( 5.076602173674213070, 4.887400388900169368, 0.000000000000000000 ) ) ;
#180410=CARTESIAN_POINT ( 'NONE',  ( -5.447343857640614573, 9.577261277214532242, -0.7998128361456362523 ) ) ;
#180411=CARTESIAN_POINT ( 'NONE',  ( 4.830447868218803897, 8.857549289555754157, -0.7998128361456481317 ) ) ;
#180419=CARTESIAN_POINT ( 'NONE',  ( -7.110325215724114578, 7.260077271291732082, 0.000000000000000000 ) ) ;
#180444=CARTESIAN_POINT ( 'NONE',  ( 5.566601156340460044, 5.879629814773917218, -0.7777157291131882033 ) ) ;
#180447=CARTESIAN_POINT ( 'NONE',  ( 4.068855497876973537, 7.761098824249525130, -0.7216878364870338292 ) ) ;
#180454=CARTESIAN_POINT ( 'NONE',  ( 3.716343503477301802, 7.349834830783237294, -1.734723475976807094E-15 ) ) ;
#180466=CARTESIAN_POINT ( 'NONE',  ( -6.414942957921379474, 7.513130201443591005, -1.199719254218452047 ) ) ;
#180468=B_SPLINE_CURVE_WITH_KNOTS ( 'NONE', 3,
 ( #160227, #31305, #47570, #177553, #175425, #111544, #45428, #60586, #97380, #129945, #113681, #179685, #163437, #208950, #15017, #147194, #109420, #27010 ),
 .UNSPECIFIED., .F., .F.,
 ( 4, 2, 2, 2, 2, 2, 2, 2, 4 ),
 ( 0.7103161267730502271, 0.7245945595572033104, 0.7388729923413562828, 0.7531514251255093662, 0.7674298579096623385, 0.7817082906938154219, 0.7959867234779685052, 0.8102651562621214776, 0.8245435890462745609 ),
 .UNSPECIFIED. ) ;
#180469=CARTESIAN_POINT ( 'NONE',  ( -6.074935347375019390, 9.245119117649618801, 1.199719254218452047 ) ) ;
#180475=CARTESIAN_POINT ( 'NONE',  ( 5.664274315459256748, 9.830346811336296398, -0.7998128361456481317 ) ) ;
#180479=CARTESIAN_POINT ( 'NONE',  ( 5.011754246625688580, 8.023990808224052529, -1.135194352273690255 ) ) ;
#180480=CARTESIAN_POINT ( 'NONE',  ( -5.887983850084758330, 10.09134126839936840, 0.7998128361456291469 ) ) ;
#180486=CARTESIAN_POINT ( 'NONE',  ( -6.482206841109545259, 6.735198534148810090, 0.7216878364870257245 ) ) ;
#180489=CARTESIAN_POINT ( 'NONE',  ( -5.424143973919053785, 8.485862515284315677, 1.199719254218454489 ) ) ;
#180498=CARTESIAN_POINT ( 'NONE',  ( -3.946832114909622380, 7.618738210787626919, 0.7216878364870227269 ) ) ;
#180506=CARTESIAN_POINT ( 'NONE',  ( -6.607915433898670088, 6.755313035342081385, 0.3810012274577500579 ) ) ;
#180508=DIRECTION ( 'NONE',  ( 0.6507913734559627184, 0.7592566023653016805, 0.000000000000000000 ) ) ;
#180511=CARTESIAN_POINT ( 'NONE',  ( -7.944151662964566540, 8.232874793072271657, 0.000000000000000000 ) ) ;
#180512=CARTESIAN_POINT ( 'NONE',  ( 3.413620815590684199, 7.204584394822967752, 0.7998128361456281477 ) ) ;
#180513=CARTESIAN_POINT ( 'NONE',  ( -4.847922445338252118, 7.813604065273374921, -1.199719254218453823 ) ) ;
#180526=CARTESIAN_POINT ( 'NONE',  ( -5.546112223000226216, 5.929839062422638918, -0.8878705470019981894 ) ) ;
#180530=DIRECTION ( 'NONE',  ( -0.5620411653101037297, -0.8271092603138117116, 0.000000000000000000 ) ) ;
#180535=CARTESIAN_POINT ( 'NONE',  ( -6.119526231721793330, 8.232809585132461194, 1.599625672291263179 ) ) ;
#180560=CARTESIAN_POINT ( 'NONE',  ( 5.571474780572990504, 5.464751763615448787, 0.7998128361456352531 ) ) ;
#180573=CARTESIAN_POINT ( 'NONE',  ( 4.893454165248502186, 8.027304163657891678, -0.9628252682179049282 ) ) ;
#180575=CARTESIAN_POINT ( 'NONE',  ( 7.404161286838808920, 8.771181268467660885, -1.082531754730548412 ) ) ;
#180582=CARTESIAN_POINT ( 'NONE',  ( -6.635789839245807897, 6.706452665400368218, 0.7998128361456341429 ) ) ;
#180587=CARTESIAN_POINT ( 'NONE',  ( -5.750066545527201534, 9.722511713174800008, 0.000000000000000000 ) ) ;
#180591=CARTESIAN_POINT ( 'NONE',  ( -4.001066012398721838, 7.682011088333574378, -6.818990669119789124E-05 ) ) ;
#180596=CARTESIAN_POINT ( 'NONE',  ( -6.120580001926503755, 6.105374521861167914, -0.7998128361456362523 ) ) ;
#180606=CARTESIAN_POINT ( 'NONE',  ( 4.061549535745618833, 6.896169004081968090, -1.199719254218452047 ) ) ;
#180629=CARTESIAN_POINT ( 'NONE',  ( -6.400331034103001748, 9.624747418832267698, 1.199719254218452935 ) ) ;
#180633=CARTESIAN_POINT ( 'NONE',  ( 7.842465510862060896, 8.114240948952696542, 0.000000000000000000 ) ) ;
#180640=CARTESIAN_POINT ( 'NONE',  ( 5.662465432362883355, 6.635239754958710989, 1.199719254218451159 ) ) ;
#180651=CARTESIAN_POINT ( 'NONE',  ( 7.539742822975472158, 7.968990512992423447, -0.7216878364870317197 ) ) ;
#180652=VERTEX_POINT ( 'NONE', #54136 ) ;
#180662=CARTESIAN_POINT ( 'NONE',  ( -7.282137904315833410, 7.668451441222825515, 0.000000000000000000 ) ) ;
#180691=EDGE_LOOP ( 'NONE', ( #153878, #207674 ) ) ;
#180695=CARTESIAN_POINT ( 'NONE',  ( 4.681308178468477799, 8.683552984847038303, 0.000000000000000000 ) ) ;
#180698=CARTESIAN_POINT ( 'NONE',  ( 6.412080304620304538, 6.445458208337293549, -0.7998128361456481317 ) ) ;
#180700=DIRECTION ( 'NONE',  ( 0.6507913734559641616, -0.7592566023653004592, 0.000000000000000000 ) ) ;
#180702=EDGE_CURVE ( 'NONE', #63064, #206426, #77735, .T. ) ;
#180711=CARTESIAN_POINT ( 'NONE',  ( -3.851398154733808088, 6.650992392901508232, -1.199719254218450271 ) ) ;
#180714=CARTESIAN_POINT ( 'NONE',  ( 5.844973620822844218, 6.952128991449046502, 1.082531754730549967 ) ) ;
#180728=CARTESIAN_POINT ( 'NONE',  ( -7.282137904315833410, 7.668451441222825515, 0.000000000000000000 ) ) ;
#180730=CARTESIAN_POINT ( 'NONE',  ( -4.150204419558982671, 7.856005899545188242, 0.7216878364870338292 ) ) ;
#180757=CARTESIAN_POINT ( 'NONE',  ( -5.178288325776719603, 5.006034233019745372, 0.000000000000000000 ) ) ;
#180760=CARTESIAN_POINT ( 'NONE',  ( 3.894033820048811823, 8.999999999999998224, -0.7749999999999996891 ) ) ;
#180765=CARTESIAN_POINT ( 'NONE',  ( -6.587282531393266360, 8.778525268082516320, 1.599625672291269396 ) ) ;
#180766=CARTESIAN_POINT ( 'NONE',  ( -5.780704523637806069, 7.347994962087573079, -1.310296981949153006 ) ) ;
#180768=CARTESIAN_POINT ( 'NONE',  ( 5.094532678321557206, 4.917790403868676385, -0.1305349544365452807 ) ) ;
#180769=ORIENTED_EDGE ( 'NONE', *, *, #134258, .F. ) ;
#180788=CARTESIAN_POINT ( 'NONE',  ( 6.170896192875352959, 7.228408975556602556, 1.199719254218453823 ) ) ;
#180810=CARTESIAN_POINT ( 'NONE',  ( 5.494797395288433250, 9.632623737803665875, 0.000000000000000000 ) ) ;
#180811=CARTESIAN_POINT ( 'NONE',  ( 4.549643065837591038, 7.465611455855944101, -1.199719254218452047 ) ) ;
#180822=CARTESIAN_POINT ( 'NONE',  ( 5.045036709957831711, 4.903268083610561767, 0.3063280728123271568 ) ) ;
#180823=CARTESIAN_POINT ( 'NONE',  ( 4.653539691347775786, 8.417882268172059312, -0.4891605808478947104 ) ) ;
#180825=CARTESIAN_POINT ( 'NONE',  ( -4.923019175093582334, 8.757623114335565617, 0.7216878364870267237 ) ) ;
#180826=CARTESIAN_POINT ( 'NONE',  ( 3.268924434670684498, 6.827845917175511481, -1.734723475976807094E-15 ) ) ;
#180852=CARTESIAN_POINT ( 'NONE',  ( 5.987861119090863049, 7.014868056141362551, 1.199719254218452047 ) ) ;
#180854=CARTESIAN_POINT ( 'NONE',  ( 3.953084306836263995, 6.769626237021087789, 1.199719254218452047 ) ) ;
#180873=CARTESIAN_POINT ( 'NONE',  ( -6.143440778383317813, 6.339971461045375456, 7.509178883279419847E-06 ) ) ;
#180883=CARTESIAN_POINT ( 'NONE',  ( 7.042534447655770080, 7.180988041878682004, -0.7998128361456341429 ) ) ;
#180887=CARTESIAN_POINT ( 'NONE',  ( -6.147489916148834332, 6.992309281770507923, 0.9361876800342925353 ) ) ;
#180888=CARTESIAN_POINT ( 'NONE',  ( 6.723917837734620484, 6.809268663637336516, 0.000000000000000000 ) ) ;
#180899=CARTESIAN_POINT ( 'NONE',  ( 4.599920620972065777, 8.367456947080912144, 0.1478172174028801744 ) ) ;
#180915=DIRECTION ( 'NONE',  ( 0.000000000000000000, 0.000000000000000000, 1.000000000000000000 ) ) ;
#180922=CARTESIAN_POINT ( 'NONE',  ( -7.795011973214244883, 8.058878488363559356, 0.7998128361456341429 ) ) ;
#180924=CARTESIAN_POINT ( 'NONE',  ( 6.496291879603339758, 7.608037276739255006, 1.199719254218452935 ) ) ;
#180932=EDGE_CURVE ( 'NONE', #26714, #130448, #97907, .T. ) ;
#180934=VECTOR ( 'NONE', #180959, 1000.000000000000000 ) ;
#180935=CARTESIAN_POINT ( 'NONE',  ( -6.265495719280979259, 6.992744598377811371, -0.9808356887253886214 ) ) ;
#180952=CARTESIAN_POINT ( 'NONE',  ( 5.234856708652222856, 8.161064355852680308, 1.082531754730549078 ) ) ;
#180959=DIRECTION ( 'NONE',  ( -0.7592566023652995710, -0.6507913734559650498, -0.000000000000000000 ) ) ;
#180967=CARTESIAN_POINT ( 'NONE',  ( -3.689227196694341515, 7.318199139536432973, -0.7216878364870458196 ) ) ;
#180969=CARTESIAN_POINT ( 'NONE',  ( 4.688087255275310561, 8.691461907788344377, -0.7998128361456381397 ) ) ;
#180972=CARTESIAN_POINT ( 'NONE',  ( -7.944151662964566540, 8.232874793072271657, 0.000000000000000000 ) ) ;
#180973=CIRCLE ( 'NONE', #177431, 0.08000000000000041800 ) ;
#180975=CARTESIAN_POINT ( 'NONE',  ( -5.517242166118370150, 5.401480380085008193, 0.7998128361456281477 ) ) ;
#180986=CARTESIAN_POINT ( 'NONE',  ( -3.667411383892738019, 3.520940564220485847, 2.447588313016640704 ) ) ;
#180987=CARTESIAN_POINT ( 'NONE',  ( -0.1216878429548678975, 3.463015919485879834, -1.996294584693599994 ) ) ;
#181020=CARTESIAN_POINT ( 'NONE',  ( 4.065465959251388206, 5.836405933916976707, -1.599625672291269396 ) ) ;
#181027=CARTESIAN_POINT ( 'NONE',  ( -4.136646265500964148, 6.879818838842817641, -1.082531754730551743 ) ) ;
#181035=CARTESIAN_POINT ( 'NONE',  ( -6.557303570864871034, 7.679217583210999010, -1.199719254218452047 ) ) ;
#181043=CARTESIAN_POINT ( 'NONE',  ( -5.661411662158206681, 8.762674818229999829, -1.199719254218452047 ) ) ;
#181045=CARTESIAN_POINT ( 'NONE',  ( 6.400241882075590638, 6.902609158730609096, 0.7749192096189911894 ) ) ;
#181050=CARTESIAN_POINT ( 'NONE',  ( 6.692885107001518286, 7.837396042037102717, -1.199719254218452047 ) ) ;
#181058=CARTESIAN_POINT ( 'NONE',  ( -5.517242166118370150, 5.401480380085008193, 0.7998128361456281477 ) ) ;
#181062=CARTESIAN_POINT ( 'NONE',  ( -4.776215253764153346, 8.794277906025310898, -0.7998128361456362523 ) ) ;
#181066=CARTESIAN_POINT ( 'NONE',  ( 7.471952054462756010, 7.889901283060952508, 0.7216878364870267237 ) ) ;
#181068=CARTESIAN_POINT ( 'NONE',  ( -7.119440060507479018, 8.439006504414422238, 1.082531754730549078 ) ) ;
#181074=CARTESIAN_POINT ( 'NONE',  ( 6.638652492546827766, 7.774124658506663010, 1.199719254218452047 ) ) ;
#181117=CARTESIAN_POINT ( 'NONE',  ( -5.543397514969483630, 7.443247485022737031, -1.247832777738608678 ) ) ;
#181133=B_SPLINE_CURVE_WITH_KNOTS ( 'NONE', 3,
 ( #23591, #60366, #122271, #57179 ),
 .UNSPECIFIED., .F., .F.,
 ( 4, 4 ),
 ( 0.000000000000000000, 0.0007700259059032546743 ),
 .UNSPECIFIED. ) ;
#181135=CARTESIAN_POINT ( 'NONE',  ( -2.844178363816758814, 6.540234867753325076, -0.7998128361456481317 ) ) ;
#181148=CARTESIAN_POINT ( 'NONE',  ( 5.204350862799327793, 7.165104988056252289, -1.599625672291281386 ) ) ;
#181151=CARTESIAN_POINT ( 'NONE',  ( 6.224601922005513543, 7.395028676162137771, -1.082531754730548412 ) ) ;
#181160=AXIS2_PLACEMENT_3D ( 'NONE', #144308, #115013, #78180 ) ;
#181165=CARTESIAN_POINT ( 'NONE',  ( -4.610654757099099221, 7.536791762327691657, 1.199719254218452935 ) ) ;
#181166=CARTESIAN_POINT ( 'NONE',  ( 5.337069745634900997, 6.255611453776062980, 1.199719254218452047 ) ) ;
#181176=CARTESIAN_POINT ( 'NONE',  ( -6.994027139803241866, 9.253060644560830994, -1.599625672291271394 ) ) ;
#181177=CARTESIAN_POINT ( 'NONE',  ( 6.047819040147648373, 9.213483425884394507, 1.199719254218452047 ) ) ;
#181179=CARTESIAN_POINT ( 'NONE',  ( -6.392116398764163598, 6.567141947922926271, -2.438447736784542297 ) ) ;
#181183=CARTESIAN_POINT ( 'NONE',  ( 4.203910148689107729, 7.062256385849379647, -1.199719254218448494 ) ) ;
#181189=CARTESIAN_POINT ( 'NONE',  ( -6.600870636098118638, 6.767368133241304484, -0.2259646751960984468 ) ) ;
#181196=CARTESIAN_POINT ( 'NONE',  ( -3.811250578772981346, 6.500190537660166079, -1.082531754730546636 ) ) ;
#181208=CARTESIAN_POINT ( 'NONE',  ( -4.450244736157934256, 7.987476157872523963, 2.500000000000000444 ) ) ;
#181214=EDGE_CURVE ( 'NONE', #81693, #135497, #23054, .T. ) ;
#181247=CARTESIAN_POINT ( 'NONE',  ( 6.482206841109512396, 9.616306177052839743, -1.082531754730548412 ) ) ;
#181248=CARTESIAN_POINT ( 'NONE',  ( -2.862179826260718762, 6.353310540697199471, 0.000000000000000000 ) ) ;
#181275=CARTESIAN_POINT ( 'NONE',  ( -5.550083779947821760, 7.568460058062819407, -1.599625672291271394 ) ) ;
#181277=CARTESIAN_POINT ( 'NONE',  ( 6.007671464186825183, 8.102312356341712984, 1.443375672974064550 ) ) ;
#181282=CARTESIAN_POINT ( 'NONE',  ( -5.498713818794216834, 8.572860667638675380, -1.199719254218452047 ) ) ;
#181291=CARTESIAN_POINT ( 'NONE',  ( -6.882699257592852504, 8.058845884393651460, -1.199719254218452047 ) ) ;
#181303=CARTESIAN_POINT ( 'NONE',  ( -4.827585214917754719, 7.789877296449459365, -1.199719254218453823 ) ) ;
#181308=CARTESIAN_POINT ( 'NONE',  ( -7.268579750702168774, 7.652633595340216921, -0.7216878364870338292 ) ) ;
#181310=CARTESIAN_POINT ( 'NONE',  ( -6.821160681006823268, 9.051383109298335228, 1.443375672974064550 ) ) ;
#181311=CARTESIAN_POINT ( 'NONE',  ( 6.003228155800906407, 10.22579295840155744, 0.000000000000000000 ) ) ;
#181312=CARTESIAN_POINT ( 'NONE',  ( -5.302647476276252547, 5.359045941843285199, 0.7216878364870257245 ) ) ;
#181332=CARTESIAN_POINT ( 'NONE',  ( -1.870624324079490863, 2.481157652721496021, -2.472014912841812961 ) ) ;
#181333=CARTESIAN_POINT ( 'NONE',  ( 6.225987253121650689, 7.022442755726078900, -1.008712875586889712 ) ) ;
#181352=CARTESIAN_POINT ( 'NONE',  ( 6.321627859881460587, 6.858947107989728842, -0.6823232096292205506 ) ) ;
#181368=ADVANCED_FACE ( 'NONE', ( #210562, #12353, #128353, #66417 ), #95783, .T. ) ;
#181369=CARTESIAN_POINT ( 'NONE',  ( 6.933015448541703485, 9.181880338089085214, 1.599625672291268286 ) ) ;
#181372=CARTESIAN_POINT ( 'NONE',  ( -6.317173229324657413, 6.334733287159020954, 0.000000000000000000 ) ) ;
#181386=CARTESIAN_POINT ( 'NONE',  ( 4.061549535745618833, 6.896169004081968090, -1.199719254218452047 ) ) ;
#181388=CARTESIAN_POINT ( 'NONE',  ( 6.749980374757213575, 8.968339418673846097, 1.599625672291268286 ) ) ;
#181394=CARTESIAN_POINT ( 'NONE',  ( -5.587368702163209910, 9.532697562583475559, 0.000000000000000000 ) ) ;
#181400=CARTESIAN_POINT ( 'NONE',  ( 6.556249800660121529, 9.806652646482286073, 1.199719254218452047 ) ) ;
#181411=CARTESIAN_POINT ( 'NONE',  ( -7.105881907338178038, 7.462819444748888920, -0.7216878364870338292 ) ) ;
#181412=CARTESIAN_POINT ( 'NONE',  ( 4.245111494854632461, 7.966730820723463502, 0.000000000000000000 ) ) ;
#181420=CARTESIAN_POINT ( 'NONE',  ( -5.320648938720212051, 5.172121614787156929, 0.000000000000000000 ) ) ;
#181421=CARTESIAN_POINT ( 'NONE',  ( -5.302647476720585118, 9.200522799567075083, 0.000000000000000000 ) ) ;
#181426=CARTESIAN_POINT ( 'NONE',  ( 5.682275777458854371, 5.801945626556378244, 0.7216878364870328300 ) ) ;
#181445=CARTESIAN_POINT ( 'NONE',  ( -5.829079699232685208, 5.765290835385048496, 0.000000000000000000 ) ) ;
#181458=CARTESIAN_POINT ( 'NONE',  ( 3.715816618597135523, 6.492813934075403637, -1.199719254218453823 ) ) ;
#181461=CARTESIAN_POINT ( 'NONE',  ( 4.369470645354133431, 8.319742529546998000, 0.7998128361456271485 ) ) ;
#181468=EDGE_CURVE ( 'NONE', #198620, #101986, #205733, .T. ) ;
#181496=CARTESIAN_POINT ( 'NONE',  ( 4.095971805104285934, 6.832365301713403838, 1.082531754730549078 ) ) ;
#181501=CARTESIAN_POINT ( 'NONE',  ( 4.588505019226127857, 4.929507493212790692, 0.7728389572207298164 ) ) ;
#181502=CARTESIAN_POINT ( 'NONE',  ( 4.204437033569277560, 7.919277282557212416, 0.000000000000000000 ) ) ;
#181514=CARTESIAN_POINT ( 'NONE',  ( -5.661411662158206681, 8.762674818229999829, -1.199719254218452047 ) ) ;
#181516=CARTESIAN_POINT ( 'NONE',  ( -6.424584688029276514, 8.588711117491191871, 1.599625672291269396 ) ) ;
#181519=CARTESIAN_POINT ( 'NONE',  ( 4.726684935852882852, 4.891486930089099516, -0.8194250277325197951 ) ) ;
#181524=CARTESIAN_POINT ( 'NONE',  ( 6.526270840131753737, 8.707344961610770540, -1.599625672291283607 ) ) ;
#181529=CARTESIAN_POINT ( 'NONE',  ( -5.608755560901242276, 5.628057139458180202, 0.4582055134699433707 ) ) ;
#181530=CARTESIAN_POINT ( 'NONE',  ( -6.074935347375019390, 9.245119117649618801, 1.199719254218452047 ) ) ;
#181536=CARTESIAN_POINT ( 'NONE',  ( -4.800995793014949165, 8.615262501910491366, 0.7216878364870267237 ) ) ;
#181539=CARTESIAN_POINT ( 'NONE',  ( -5.773793314573309132, 7.829454515125894964, 1.599625672291263179 ) ) ;
#181559=CARTESIAN_POINT ( 'NONE',  ( -3.960390268967665328, 6.674186842887300131, 1.082531754730549967 ) ) ;
#181561=CARTESIAN_POINT ( 'NONE',  ( -7.553827861469316396, 8.841829255582865699, -1.199719254218452047 ) ) ;
#181562=CARTESIAN_POINT ( 'NONE',  ( 5.571474780572990504, 5.464751763615448787, 0.7998128361456352531 ) ) ;
#181563=CARTESIAN_POINT ( 'NONE',  ( -6.089547271193396227, 7.133501900260939443, -1.199719254218453823 ) ) ;
#181612=CARTESIAN_POINT ( 'NONE',  ( 2.898410978271408922, 6.603506251283770112, -0.7998128361456362523 ) ) ;
#181624=CARTESIAN_POINT ( 'NONE',  ( 4.678042868546113731, 8.270637144445508682, 0.5573067791126932180 ) ) ;
#181626=CARTESIAN_POINT ( 'NONE',  ( 4.523580528814945545, 5.306540700819438960, 1.199719254218452047 ) ) ;
#181632=CARTESIAN_POINT ( 'NONE',  ( -4.423703259808839938, 8.383013913077441259, 0.7998128361456352531 ) ) ;
#181638=CARTESIAN_POINT ( 'NONE',  ( -7.065207446052813367, 8.375735120883982532, -1.082531754730549967 ) ) ;
#181643=CARTESIAN_POINT ( 'NONE',  ( -4.025218236631250335, 7.648764168548251696, 0.3240912158420958256 ) ) ;
#181647=CARTESIAN_POINT ( 'NONE',  ( 6.875393295905841917, 7.193916064744513506, 0.000000000000000000 ) ) ;
#181650=CARTESIAN_POINT ( 'NONE',  ( -4.878955176071358757, 6.785476686873604280, -1.599625672291271394 ) ) ;
#181660=CARTESIAN_POINT ( 'NONE',  ( 5.273195401072370281, 5.116759154198018855, -0.7998128361456481317 ) ) ;
#181664=ORIENTED_EDGE ( 'NONE', *, *, #212020, .F. ) ;
#181690=CARTESIAN_POINT ( 'NONE',  ( 7.018280793729500644, 8.217024343219755167, -1.199719254218452047 ) ) ;
#181696=CARTESIAN_POINT ( 'NONE',  ( 5.587368702607580673, 5.691220705896524734, -0.7216878364870458196 ) ) ;
#181699=CARTESIAN_POINT ( 'NONE',  ( 5.668717624289557833, 8.667235424096215723, -1.082531754730548412 ) ) ;
#181711=EDGE_CURVE ( 'NONE', #123093, #111396, #197510, .T. ) ;
#181712=CARTESIAN_POINT ( 'NONE',  ( -6.075462232699549325, 9.141770800574526845, 1.082531754730549967 ) ) ;
#181746=CARTESIAN_POINT ( 'NONE',  ( 5.716698046817569434, 6.698511138489155137, -1.199719254218452047 ) ) ;
#181747=CARTESIAN_POINT ( 'NONE',  ( 5.306037014901791693, 7.283738832175834510, 1.599625672291269396 ) ) ;
#181759=CARTESIAN_POINT ( 'NONE',  ( -4.390861645979385663, 6.216034235099629157, -1.599625672291271394 ) ) ;
#181763=CARTESIAN_POINT ( 'NONE',  ( 4.204437033569277560, 7.919277282557212416, 0.000000000000000000 ) ) ;
#181771=CARTESIAN_POINT ( 'NONE',  ( -3.311934663488232733, 7.085950550703385531, -0.7998128361456481317 ) ) ;
#181778=CARTESIAN_POINT ( 'NONE',  ( -7.268579750702168774, 7.652633595340216921, -0.7216878364870338292 ) ) ;
#181780=CARTESIAN_POINT ( 'NONE',  ( -5.506019780925599960, 5.596313630600862510, 0.7216878364870257245 ) ) ;
#181797=CARTESIAN_POINT ( 'NONE',  ( -5.320648938720212051, 5.172121614787156929, 0.000000000000000000 ) ) ;
#181809=CARTESIAN_POINT ( 'NONE',  ( -3.871735385154307263, 6.674719161725423788, -1.199719254218450271 ) ) ;
#181817=FACE_OUTER_BOUND ( 'NONE', #80329, .T. ) ;
#181819=CARTESIAN_POINT ( 'NONE',  ( -5.143355005462953322, 7.892534720870457043, -1.245665949277234841 ) ) ;
#181835=CARTESIAN_POINT ( 'NONE',  ( 6.710359684120930091, 6.793450817754725257, 0.7998128361456352531 ) ) ;
#181842=CARTESIAN_POINT ( 'NONE',  ( -4.274563570058511175, 8.209017608368725405, 0.000000000000000000 ) ) ;
#181859=CARTESIAN_POINT ( 'NONE',  ( 7.015418140428412386, 7.149352350113456822, 0.7998128361456331437 ) ) ;
#181860=CARTESIAN_POINT ( 'NONE',  ( 5.550083779947807550, 7.568460058062819407, -1.599625672291283607 ) ) ;
#181862=CARTESIAN_POINT ( 'NONE',  ( 3.867818961648523235, 7.734482231890414283, 1.040834085586084257E-14 ) ) ;
#181865=CARTESIAN_POINT ( 'NONE',  ( -6.181864745680308637, 5.311701037653689284, -2.438145240001343250 ) ) ;
#181874=CARTESIAN_POINT ( 'NONE',  ( 4.722521264130603136, 8.336029038342307018, -0.7037175076533495055 ) ) ;
#181875=CARTESIAN_POINT ( 'NONE',  ( -6.753369912938502750, 7.051555451282599307, 0.000000000000000000 ) ) ;
#181876=CARTESIAN_POINT ( 'NONE',  ( 3.594320121398666856, 7.207474218358159490, -1.734723475976807094E-15 ) ) ;
#181888=ORIENTED_EDGE ( 'NONE', *, *, #148090, .T. ) ;
#181894=CARTESIAN_POINT ( 'NONE',  ( -1.806654366501805775, 0.000000000000000000, 2.500000000000000444 ) ) ;
#181901=CARTESIAN_POINT ( 'NONE',  ( 5.890091390494168522, 5.836471141856793388, 0.000000000000000000 ) ) ;
#181904=CARTESIAN_POINT ( 'NONE',  ( 5.422335090822693715, 5.290755458906732933, 0.000000000000000000 ) ) ;
#181923=CARTESIAN_POINT ( 'NONE',  ( -4.858757509019071996, 5.629766575900002401, 7.500000000000000000 ) ) ;
#181935=CARTESIAN_POINT ( 'NONE',  ( 4.857564175446106525, 8.889184981320973122, 0.7998128361456331437 ) ) ;
#181940=CARTESIAN_POINT ( 'NONE',  ( -5.998939594393441155, 7.096481464931535754, 1.069142741232721461 ) ) ;
#181941=CARTESIAN_POINT ( 'NONE',  ( 5.013482942003290255, 9.071090208970993274, -0.7998128361456481317 ) ) ;
#181950=CARTESIAN_POINT ( 'NONE',  ( -1.846004154127505403, 8.940320519588478732, 0.7750000000000013545 ) ) ;
#181952=CARTESIAN_POINT ( 'NONE',  ( 4.893454165248502186, 8.027304163657891678, -0.9628252682179049282 ) ) ;
#181963=CARTESIAN_POINT ( 'NONE',  ( 4.723400270955312230, 6.733595400378874274, 1.377748641254195716 ) ) ;
#181974=CARTESIAN_POINT ( 'NONE',  ( -7.632314129850253259, 7.869064337772231355, 0.7998128361456341429 ) ) ;
#181976=CARTESIAN_POINT ( 'NONE',  ( 7.038618024149998043, 8.240751112043669835, -1.199719254218452047 ) ) ;
#181984=DIRECTION ( 'NONE',  ( 0.6507913734559641616, -0.7592566023653004592, 0.000000000000000000 ) ) ;
#181988=CARTESIAN_POINT ( 'NONE',  ( 0.1054570145121075109, 2.614151819895196294, -2.076146791065091701 ) ) ;
#182004=CARTESIAN_POINT ( 'NONE',  ( 5.397554552016212703, 8.350878506444006533, 1.082531754730547524 ) ) ;
#182007=ORIENTED_EDGE ( 'NONE', *, *, #98017, .F. ) ;
#182016=CARTESIAN_POINT ( 'NONE',  ( -5.207740401424942434, 6.208690235484773723, 1.082531754730549078 ) ) ;
#182019=CARTESIAN_POINT ( 'NONE',  ( 6.333594036239346359, 7.418223126147930557, 1.199719254218453823 ) ) ;
#182022=CARTESIAN_POINT ( 'NONE',  ( -6.583366107887490770, 9.838288338247510367, 1.199719254218452935 ) ) ;
#182024=CARTESIAN_POINT ( 'NONE',  ( -4.329849954717889915, 6.144853928627882489, 1.599625672291270506 ) ) ;
#182068=CARTESIAN_POINT ( 'NONE',  ( 4.740510986633625024, 5.559626234941203116, -1.199719254218450271 ) ) ;
#182070=CARTESIAN_POINT ( 'NONE',  ( -4.167966236947438396, 7.861110150953528830, 0.1643318641706831840 ) ) ;
#182074=CARTESIAN_POINT ( 'NONE',  ( -4.787437638956920871, 8.599444655509458357, -0.7216878364870338292 ) ) ;
#182081=CARTESIAN_POINT ( 'NONE',  ( -5.576146316970437944, 9.727530813099326323, 0.000000000000000000 ) ) ;
#182090=CARTESIAN_POINT ( 'NONE',  ( -4.796552484184649856, 8.818004674849227342, -0.7998128361456362523 ) ) ;
#182092=CARTESIAN_POINT ( 'NONE',  ( 4.598366155629488361, 8.485928551783258555, 0.1149073004905968448 ) ) ;
#182097=CARTESIAN_POINT ( 'NONE',  ( 7.452141709366786770, 8.723195411463290583, 1.199719254218452047 ) ) ;
#182106=CARTESIAN_POINT ( 'NONE',  ( -5.829079699232685208, 5.765290835385048496, 0.000000000000000000 ) ) ;
#182110=CARTESIAN_POINT ( 'NONE',  ( -7.259464905474441565, 7.434073576000447048, -0.7998128361456362523 ) ) ;
#182112=FACE_OUTER_BOUND ( 'NONE', #174956, .T. ) ;
#182113=CARTESIAN_POINT ( 'NONE',  ( -3.623772196602547346, 7.449761006003425834, 0.000000000000000000 ) ) ;
#182114=CARTESIAN_POINT ( 'NONE',  ( 4.841670253411575864, 8.662716039039905169, -0.7216878364870458196 ) ) ;
#182117=CARTESIAN_POINT ( 'NONE',  ( -5.912764388891193157, 9.912325863766124456, 0.000000000000000000 ) ) ;
#182124=CARTESIAN_POINT ( 'NONE',  ( 7.028976294042106332, 7.165170195996068969, 0.000000000000000000 ) ) ;
#182138=CARTESIAN_POINT ( 'NONE',  ( 5.894874513638865388, 7.262872338272549300, -1.253420816524719150 ) ) ;
#182151=EDGE_LOOP ( 'NONE', ( #115283, #134467, #19601, #208943, #30394 ) ) ;
#182165=CARTESIAN_POINT ( 'NONE',  ( -5.221311770390402174, 7.721201550036163042, -1.200461426208466076 ) ) ;
#182183=LINE ( 'NONE', #18619, #197791 ) ;
#182187=CARTESIAN_POINT ( 'NONE',  ( -5.818384198920079520, 6.817144982608731141, 1.199719254218452935 ) ) ;
#182189=CARTESIAN_POINT ( 'NONE',  ( 5.854088466050551887, 10.05179665369283981, 0.7998128361456341429 ) ) ;
#182199=VERTEX_POINT ( 'NONE', #23009 ) ;
#182202=CARTESIAN_POINT ( 'NONE',  ( 5.169401708560450004, 9.252995436621013425, 0.000000000000000000 ) ) ;
#182205=CARTESIAN_POINT ( 'NONE',  ( 6.549997608733495902, 7.774656977344789333, -1.082531754730548412 ) ) ;
#182221=CARTESIAN_POINT ( 'NONE',  ( -6.445975688654487001, 6.485002823043819475, -0.7998128361456362523 ) ) ;
#182222=CARTESIAN_POINT ( 'NONE',  ( 3.878514461961128479, 6.682628084666728085, -1.199719254218448494 ) ) ;
#182230=CARTESIAN_POINT ( 'NONE',  ( -6.400331034103001748, 9.624747418832267698, 1.199719254218452935 ) ) ;
#182231=CARTESIAN_POINT ( 'NONE',  ( 7.679767667498067496, 7.924426798361372093, 0.000000000000000000 ) ) ;
#182238=CARTESIAN_POINT ( 'NONE',  ( 3.878514461961128479, 6.682628084666728085, -1.199719254218448494 ) ) ;
#182240=CARTESIAN_POINT ( 'NONE',  ( -0.07171210202241015685, 2.519999999999996021, 2.000000000000000444 ) ) ;
#182245=CARTESIAN_POINT ( 'NONE',  ( -6.035068427865825313, 7.156668563632000435, 1.186355232826277417 ) ) ;
#182255=CARTESIAN_POINT ( 'NONE',  ( -5.112833325684928987, 5.137596099486740897, -0.7216878364870338292 ) ) ;
#182268=CARTESIAN_POINT ( 'NONE',  ( 3.879041346841291649, 7.539648981374564407, 1.040834085586084257E-14 ) ) ;
#182271=VERTEX_POINT ( 'NONE', #77111 ) ;
#182285=CARTESIAN_POINT ( 'NONE',  ( 3.874598038455354665, 7.742391154831718580, -0.7998128361456361413 ) ) ;
#182295=VERTEX_POINT ( 'NONE', #41449 ) ;
#182305=CARTESIAN_POINT ( 'NONE',  ( 4.203910148689107729, 7.062256385849379647, -1.199719254218448494 ) ) ;
#182306=CARTESIAN_POINT ( 'NONE',  ( -5.180624094197616714, 5.216685329418210948, 0.7216878364870257245 ) ) ;
#182319=DIRECTION ( 'NONE',  ( -0.7927788072566357425, 0.000000000000000000, -0.6095094443605826307 ) ) ;
#182322=DIRECTION ( 'NONE',  ( 1.000000000000000000, 2.090028284309406390E-15, 0.000000000000000000 ) ) ;
#182331=ORIENTED_EDGE ( 'NONE', *, *, #130852, .T. ) ;
#182332=CARTESIAN_POINT ( 'NONE',  ( -7.605197822622922210, 7.837428646007010613, -0.7998128361456362523 ) ) ;
#182346=CARTESIAN_POINT ( 'NONE',  ( -7.584860592202423035, 7.813701877183096833, -0.7998128361456362523 ) ) ;
#182353=CARTESIAN_POINT ( 'NONE',  ( 5.225741863424510747, 5.061396693608882558, 0.7998128361456352531 ) ) ;
#182358=CARTESIAN_POINT ( 'NONE',  ( -6.123442655227560927, 7.173046514967467147, 1.199719254218452047 ) ) ;
#182361=CARTESIAN_POINT ( 'NONE',  ( -5.966997003790221576, 9.015228033513643879, -1.082531754730549967 ) ) ;
#182363=CARTESIAN_POINT ( 'NONE',  ( -6.902509602688821744, 8.185920970292658083, -1.082531754730549967 ) ) ;
#182364=CARTESIAN_POINT ( 'NONE',  ( 4.434925645001613681, 5.307073019657559065, -1.082531754730548412 ) ) ;
#182365=CARTESIAN_POINT ( 'NONE',  ( -3.648552735408990166, 6.310376387068841630, -1.082531754730546636 ) ) ;
#182379=CARTESIAN_POINT ( 'NONE',  ( -0.3960368903851408384, 2.881569912824395896, 1.962180772919328353 ) ) ;
#182384=CARTESIAN_POINT ( 'NONE',  ( 6.265786130652515773, 6.994708711910199384, -0.9640221254198673151 ) ) ;
#182392=CARTESIAN_POINT ( 'NONE',  ( 5.639433180129016066, 7.452461152751827633, -1.378512499824318116 ) ) ;
#182407=CARTESIAN_POINT ( 'NONE',  ( 5.583942420111207561, 7.395222456726187943, -1.242479836444350783 ) ) ;
#182422=CARTESIAN_POINT ( 'NONE',  ( 8.174640274396848483, 8.501778173076651512, 0.7998128361456291469 ) ) ;
#182425=CARTESIAN_POINT ( 'NONE',  ( -4.959250327548641479, 9.007818825440551791, -0.7998128361456362523 ) ) ;
#182439=CARTESIAN_POINT ( 'NONE',  ( 5.194709132691408549, 6.089524072008651423, 1.199719254218452935 ) ) ;
#182441=CARTESIAN_POINT ( 'NONE',  ( 5.318541398310776103, 9.426991741329731056, -0.7998128361456481317 ) ) ;
#182447=CARTESIAN_POINT ( 'NONE',  ( -6.495764994278840021, 8.671754808115688107, 1.443375672974064550 ) ) ;
#182453=CARTESIAN_POINT ( 'NONE',  ( 6.003228155800906407, 10.22579295840155744, 0.000000000000000000 ) ) ;
#182466=CARTESIAN_POINT ( 'NONE',  ( -6.292392690518214593, 7.474117906093608710, -1.082531754730549967 ) ) ;
#182467=CARTESIAN_POINT ( 'NONE',  ( 4.584065335196261692, 7.401807753487379848, 1.082531754730549078 ) ) ;
#182477=CARTESIAN_POINT ( 'NONE',  ( -3.623772196602547346, 7.449761006003425834, 0.000000000000000000 ) ) ;
#182478=CARTESIAN_POINT ( 'NONE',  ( -5.641601317062233001, 9.595968946632336127, -0.7216878364870338292 ) ) ;
#182479=CARTESIAN_POINT ( 'NONE',  ( 8.039058738260216330, 8.343599714250547805, -0.7998128361456341429 ) ) ;
#182482=CARTESIAN_POINT ( 'NONE',  ( 5.194182247366878613, 6.192872389083746043, 1.082531754730549078 ) ) ;
#182497=CARTESIAN_POINT ( 'NONE',  ( -5.329149442624137478, 7.114720453792309662, 1.278927581188280760 ) ) ;
#182499=CARTESIAN_POINT ( 'NONE',  ( -5.010620288702242853, 8.003418215864698482, -1.199719254218453823 ) ) ;
#182512=CARTESIAN_POINT ( 'NONE',  ( 4.309512724297349884, 6.121127159803966933, 1.599625672291261402 ) ) ;
#182515=ORIENTED_EDGE ( 'NONE', *, *, #61767, .F. ) ;
#182541=EDGE_LOOP ( 'NONE', ( #152807, #212661, #167559, #201708 ) ) ;
#182553=CARTESIAN_POINT ( 'NONE',  ( 6.048345925472191631, 7.189396680206621149, 1.082531754730549967 ) ) ;
#182559=CARTESIAN_POINT ( 'NONE',  ( 5.682275777458846377, 7.722684055159064975, 1.443375672974064550 ) ) ;
#182569=EDGE_CURVE ( 'NONE', #154238, #38200, #212219, .T. ) ;
#182574=CARTESIAN_POINT ( 'NONE',  ( -5.284646014276622950, 9.387447126623207794, -0.7998128361456362523 ) ) ;
#182585=CARTESIAN_POINT ( 'NONE',  ( 7.862802741282558294, 8.137967717776607657, 0.000000000000000000 ) ) ;
#182591=CARTESIAN_POINT ( 'NONE',  ( -6.505933609711270549, 8.683618192786854095, -1.599625672291271394 ) ) ;
#182597=CARTESIAN_POINT ( 'NONE',  ( -6.455090533882206216, 7.663932056684933158, -1.082531754730549967 ) ) ;
#182600=CARTESIAN_POINT ( 'NONE',  ( -5.098748287191073203, 8.106234214101666780, 1.199719254218452935 ) ) ;
#182615=DIRECTION ( 'NONE',  ( 0.000000000000000000, 0.000000000000000000, 1.000000000000000000 ) ) ;
#182622=CARTESIAN_POINT ( 'NONE',  ( -3.472296738875691346, 6.104744391113324120, 1.082531754730549967 ) ) ;
#182624=CARTESIAN_POINT ( 'NONE',  ( -7.445362632559989535, 8.715286488521982733, 1.199719254218452047 ) ) ;
#182626=CARTESIAN_POINT ( 'NONE',  ( -6.493429226302317225, 6.540365283632955773, 0.7998128361456341429 ) ) ;
#182634=ORIENTED_EDGE ( 'NONE', *, *, #62843, .T. ) ;
#182653=CARTESIAN_POINT ( 'NONE',  ( -5.935437387732586778, 10.14670372898850381, -0.7998128361456362523 ) ) ;
#182681=CARTESIAN_POINT ( 'NONE',  ( 4.411198876399872404, 6.239761003923544713, -1.599625672291273171 ) ) ;
#182696=CARTESIAN_POINT ( 'NONE',  ( 6.943184063974162434, 9.193743722760251202, -1.443375672974064550 ) ) ;
#182703=CARTESIAN_POINT ( 'NONE',  ( -5.529746549527323474, 7.544733289238903851, -1.599625672291271394 ) ) ;
#182710=CARTESIAN_POINT ( 'NONE',  ( -5.763624699140868834, 9.738329559057408602, -0.7216878364870338292 ) ) ;
#182717=CARTESIAN_POINT ( 'NONE',  ( 5.641601317062233001, 7.675230518029648508, -1.443375672974078761 ) ) ;
#182720=CARTESIAN_POINT ( 'NONE',  ( -4.447956913735107598, 7.346977611736363656, 1.199719254218452935 ) ) ;
#182731=CARTESIAN_POINT ( 'NONE',  ( 3.379725431556547477, 7.165039780116438273, -1.734723475976807094E-15 ) ) ;
#182732=CARTESIAN_POINT ( 'NONE',  ( 5.194709132691408549, 6.089524072008651423, 1.199719254218452935 ) ) ;
#182733=ORIENTED_EDGE ( 'NONE', *, *, #70182, .F. ) ;
#182751=CARTESIAN_POINT ( 'NONE',  ( -0.4800000000000244071, 2.999999999999999112, 2.500000000000000444 ) ) ;
#182757=CARTESIAN_POINT ( 'NONE',  ( 7.343676480457483002, 8.596652644402405841, -1.199719254218452047 ) ) ;
#182765=CARTESIAN_POINT ( 'NONE',  ( 6.530187263637528439, 7.647581891445782709, -1.199719254218452047 ) ) ;
#182771=CARTESIAN_POINT ( 'NONE',  ( 5.397554552016226914, 6.430140077841320689, 1.082531754730549078 ) ) ;
#182774=CARTESIAN_POINT ( 'NONE',  ( 6.373741612200162443, 8.529394195690610303, 1.443375672974065660 ) ) ;
#182786=CARTESIAN_POINT ( 'NONE',  ( 6.307155384238837037, 6.868572428096745064, 0.7081091520576547893 ) ) ;
#182787=CARTESIAN_POINT ( 'NONE',  ( -7.295696057929500711, 7.684269287105433222, 0.7216878364870317197 ) ) ;
#182825=CARTESIAN_POINT ( 'NONE',  ( 5.006703865196457492, 9.063181286029688977, 0.000000000000000000 ) ) ;
#182827=CARTESIAN_POINT ( 'NONE',  ( 5.224688093219824303, 7.188831756880171397, -1.599625672291283607 ) ) ;
#182834=FILL_AREA_STYLE ('',( #103739 ) ) ;
#182841=CARTESIAN_POINT ( 'NONE',  ( -5.147255595043616516, 6.034161611419515125, 1.199719254218452935 ) ) ;
#182843=CARTESIAN_POINT ( 'NONE',  ( 5.031484404002878996, 7.923796667095108326, 1.082531754730548412 ) ) ;
#182857=CARTESIAN_POINT ( 'NONE',  ( -5.641601317062233001, 9.595968946632336127, -0.7216878364870338292 ) ) ;
#182859=CARTESIAN_POINT ( 'NONE',  ( -4.828112100242283766, 7.686528979374367410, -1.082531754730549967 ) ) ;
#182885=CARTESIAN_POINT ( 'NONE',  ( -3.142457743317409680, 6.888227477170756785, 0.7998128361456352531 ) ) ;
#182894=( BOUNDED_SURFACE ( )  B_SPLINE_SURFACE ( 1, 2, ( 
 ( #76824, #139734, #77897, #125669, #73635, #140812, #157039, #205758, #75772, #144018, #191631, #127820, #193775, #43295, #23807, #142944, #190571, #44352, #108343, #89912, #60580, #155964, #109415, #90977, #207889, #27004, #174363, #126738, #206824, #7550, #57388, #92049, #192698, #123552, #176474, #25942, #189516, #58458, #158106, #41162, #9695, #107271, #173291, #141880, #24873, #45421, #13944, #82155, #149301, #63779, #80027, #145078, #133088, #882, #12880, #181780, #47563, #198038, #146130, #111537, #177545, #213212, #78956, #33413, #32355, #31297, #212143, #99492, #165549, #29156, #196978, #147187, #95246, #211081, #17142, #83219, #128865, #164485, #161294, #62704, #66948, #49668, #194847, #15007, #48617, #114732, #46480, #112604, #132028, #178615, #30225, #129938, #81098, #96309, #162365, #180730, #179677, #130987, #97372, #163430, #64841, #195926, #115791, #113673, #98420, #16071, #148247, #214249, #65880, #52869, #182859, #87516, #70160, #34477, #202291, #199086, #100549, #116858, #84298, #3023, #53943, #103768, #18214, #36608, #37691, #169819, #69091, #19287, #21406, #4089, #166622, #150383, #151451, #1954, #120080, #50732, #117936, #134156, #101619, #20355, #71227, #68015, #167686, #186056, #200164, #51818, #153581, #152505, #183930, #35542, #135213, #201228, #5150, #119004, #86440, #184982, #137342, #85369, #102694, #168752, #136271, #131666, #1577, #82856, #196622, #116489, #48261, #100178, #16772, #166243, #49313, #163069, #65521, #197669, #114375, #115430, #64488, #13593, #211785, #164130, #181421, #29866, #34106, #180370, #66573, #80744, #31994, #95949, #212851, #198720, #79667, #98075, #133785, #178253, #146832, #505, #67638, #15714, #130630, #63423, #51438, #199793, #145782, #17833, #81799, #182478, #147882, #162004, #129575, #33051, #195562, #83916, #165178, #213898, #99129, #150007, #47198, #113313, #148932, #132715, #179319, #30940, #97015, #14650, #50366, #22087, #183552, #151080, #139096, #55690, #205123, #87125, #54627, #186754, #84989, #18905, #204041, #200842, #167318, #86060, #153195 ),
 ( #117558, #185678, #37307, #201908, #121846, #35159, #103381, #53560, #118623, #52493, #187817, #155332, #69781, #19976, #3705, #2644, #68718, #169443, #4767, #101236, #39443, #119693, #5846, #152137, #21028, #134839, #135890, #138026, #184610, #70844, #72993, #36227, #136960, #154272, #6916, #202987, #120774, #102306, #168379, #38376, #104457, #105537, #170504, #171571, #88198, #71917, #23168, #89284, #160671, #159600, #44811, #25323, #207272, #75154, #92500, #93556, #10136, #57829, #188889, #156409, #122932, #90340, #157485, #41608, #9080, #173746, #172663, #123991, #58903, #144466, #107719, #125056, #76211, #191011, #42679, #143391, #110915, #40530, #158539, #126117, #106634, #108786, #175870, #192077, #61033, #142321, #56766, #174812, #26388, #141264, #209389, #24238, #208331, #59962, #189958, #140179, #127194, #94628, #43743, #91424, #109856, #77279, #11198, #27458, #176921, #193161, #206201, #28536, #7996, #12266, #78343, #74088, #173500, #75972, #90104, #5594, #170260, #40280, #71674, #89039, #137787, #7750, #174568, #57593, #26144, #208089, #205960, #142075, #157237, #56526, #190770, #122686, #92258, #91178, #158304, #123750, #22924, #139933, #189711, #188649, #41364, #9895, #106390, #42432, #8832, #107475, #24002, #59717, #203807, #125876, #25075, #156169, #6680, #38141, #104213, #21845, #74909, #141017, #87953, #55452, #154027, #121604, #187576, #207025, #39201, #105293, #171329, #108538, #155095, #73837, #58656, #124809, #72757, #138854, #204871, #172413, #27210, #160421, #161506, #159352, #147383, #129081, #111741, #62912, #177747, #95457, #13086, #28286, #47769, #12027, #78098, #178822, #65031, #93316, #193976, #79166, #10949, #163633, #14141, #175623, #146333, #43498, #77023, #109618, #143153, #29362, #212347, #113882, #209147, #211288, #196129, #179877, #145282, #112809, #15216, #195052, #60786, #126945, #45624, #192902, #94381, #44558, #46691, #31502, #30434, #97576, #213409, #96520, #81306, #162568, #210219, #130140, #61855, #191835, #80234, #110674, #63988, #176674, #144225, #128022, #149500 ) ),
 .UNSPECIFIED., .F., .F., .T. ) 
 B_SPLINE_SURFACE_WITH_KNOTS ( ( 2, 2 ),
 ( 3, 2, 2, 2, 2, 2, 2, 2, 2, 2, 2, 2, 2, 2, 2, 2, 2, 2, 2, 2, 2, 2, 2, 2, 2, 2, 2, 2, 2, 2, 2, 2, 2, 2, 2, 2, 2, 2, 2, 2, 2, 2, 2, 2, 2, 2, 2, 2, 2, 2, 2, 2, 2, 2, 2, 2, 2, 2, 2, 2, 2, 2, 2, 2, 2, 2, 2, 2, 2, 2, 2, 2, 2, 2, 2, 2, 2, 2, 2, 2, 2, 2, 2, 2, 2, 2, 2, 2, 2, 2, 2, 2, 2, 2, 2, 2, 2, 2, 2, 2, 2, 2, 2, 2, 2, 2, 2, 2, 2, 2, 2, 2, 2, 2, 2, 2, 2, 2, 2, 2, 3 ),
 ( 0.000000000000000000, 1.000000000000000000 ),
 ( 0.000000000000000000, 0.008333333333333333218, 0.01666666666666666644, 0.02500000000000000139, 0.03333333333333333287, 0.04166666666666666435, 0.05000000000000000278, 0.05833333333333333426, 0.06666666666666666574, 0.07499999999999999722, 0.08333333333333332871, 0.09166666666666666019, 0.1000000000000000056, 0.1083333333333333370, 0.1166666666666666685, 0.1250000000000000000, 0.1333333333333333315, 0.1416666666666666630, 0.1499999999999999944, 0.1583333333333333259, 0.1666666666666666574, 0.1749999999999999889, 0.1833333333333333204, 0.1916666666666666796, 0.2000000000000000111, 0.2083333333333333426, 0.2166666666666666741, 0.2250000000000000056, 0.2333333333333333370, 0.2416666666666666685, 0.2500000000000000000, 0.2583333333333333592, 0.2666666666666666630, 0.2750000000000000222, 0.2833333333333333259, 0.2916666666666666852, 0.2999999999999999889, 0.3083333333333333481, 0.3166666666666666519, 0.3250000000000000111, 0.3333333333333333148, 0.3416666666666666741, 0.3499999999999999778, 0.3583333333333333370, 0.3666666666666666408, 0.3750000000000000000, 0.3833333333333333592, 0.3916666666666666630, 0.4000000000000000222, 0.4083333333333333259, 0.4166666666666666852, 0.4249999999999999889, 0.4333333333333333481, 0.4416666666666666519, 0.4500000000000000111, 0.4583333333333333148, 0.4666666666666666741, 0.4749999999999999778, 0.4833333333333333370, 0.4916666666666666408, 0.5000000000000000000, 0.5083333333333333037, 0.5166666666666667185, 0.5250000000000000222, 0.5333333333333333259, 0.5416666666666666297, 0.5500000000000000444, 0.5583333333333333481, 0.5666666666666666519, 0.5749999999999999556, 0.5833333333333333703, 0.5916666666666666741, 0.5999999999999999778, 0.6083333333333332815, 0.6166666666666666963, 0.6250000000000000000, 0.6333333333333333037, 0.6416666666666667185, 0.6500000000000000222, 0.6583333333333333259, 0.6666666666666666297, 0.6750000000000000444, 0.6833333333333333481, 0.6916666666666666519, 0.6999999999999999556, 0.7083333333333333703, 0.7166666666666666741, 0.7249999999999999778, 0.7333333333333332815, 0.7416666666666666963, 0.7500000000000000000, 0.7583333333333333037, 0.7666666666666667185, 0.7750000000000000222, 0.7833333333333333259, 0.7916666666666666297, 0.8000000000000000444, 0.8083333333333333481, 0.8166666666666666519, 0.8249999999999999556, 0.8333333333333333703, 0.8416666666666666741, 0.8499999999999999778, 0.8583333333333332815, 0.8666666666666666963, 0.8750000000000000000, 0.8833333333333333037, 0.8916666666666667185, 0.9000000000000000222, 0.9083333333333333259, 0.9166666666666666297, 0.9250000000000000444, 0.9333333333333333481, 0.9416666666666666519, 0.9499999999999999556, 0.9583333333333333703, 0.9666666666666666741, 0.9749999999999999778, 0.9833333333333332815, 0.9916666666666666963, 1.000000000000000000 ),
 .UNSPECIFIED. ) 
 GEOMETRIC_REPRESENTATION_ITEM ( )  RATIONAL_B_SPLINE_SURFACE ( (
 ( 1.000000000000000000, 0.8660254037844387076, 1.000000000000000000, 0.8660254037844387076, 1.000000000000000000, 0.8660254037844387076, 1.000000000000000000, 0.8660254037844387076, 1.000000000000000000, 0.8660254037844387076, 1.000000000000000000, 0.8660254037844387076, 1.000000000000000000, 0.8660254037844387076, 1.000000000000000000, 0.8660254037844387076, 1.000000000000000000, 0.8660254037844387076, 1.000000000000000000, 0.8660254037844387076, 1.000000000000000000, 0.8660254037844387076, 1.000000000000000000, 0.8660254037844387076, 1.000000000000000000, 0.8660254037844387076, 1.000000000000000000, 0.8660254037844387076, 1.000000000000000000, 0.8660254037844387076, 1.000000000000000000, 0.8660254037844387076, 1.000000000000000000, 0.8660254037844387076, 1.000000000000000000, 0.8660254037844387076, 1.000000000000000000, 0.8660254037844387076, 1.000000000000000000, 0.8660254037844387076, 1.000000000000000000, 0.8660254037844387076, 1.000000000000000000, 0.8660254037844387076, 1.000000000000000000, 0.8660254037844387076, 1.000000000000000000, 0.8660254037844387076, 1.000000000000000000, 0.8660254037844387076, 1.000000000000000000, 0.8660254037844387076, 1.000000000000000000, 0.8660254037844387076, 1.000000000000000000, 0.8660254037844387076, 1.000000000000000000, 0.8660254037844387076, 1.000000000000000000, 0.8660254037844387076, 1.000000000000000000, 0.8660254037844387076, 1.000000000000000000, 0.8660254037844387076, 1.000000000000000000, 0.8660254037844387076, 1.000000000000000000, 0.8660254037844387076, 1.000000000000000000, 0.8660254037844387076, 1.000000000000000000, 0.8660254037844387076, 1.000000000000000000, 0.8660254037844387076, 1.000000000000000000, 0.8660254037844387076, 1.000000000000000000, 0.8660254037844387076, 1.000000000000000000, 0.8660254037844387076, 1.000000000000000000, 0.8660254037844387076, 1.000000000000000000, 0.8660254037844387076, 1.000000000000000000, 0.8660254037844387076, 1.000000000000000000, 0.8660254037844387076, 1.000000000000000000, 0.8660254037844387076, 1.000000000000000000, 0.8660254037844387076, 1.000000000000000000, 0.8660254037844387076, 1.000000000000000000, 0.8660254037844387076, 1.000000000000000000, 0.8660254037844387076, 1.000000000000000000, 0.8660254037844387076, 1.000000000000000000, 0.8660254037844387076, 1.000000000000000000, 0.8660254037844387076, 1.000000000000000000, 0.8660254037844387076, 1.000000000000000000, 0.8660254037844387076, 1.000000000000000000, 0.8660254037844387076, 1.000000000000000000, 0.8660254037844387076, 1.000000000000000000, 0.8660254037844387076, 1.000000000000000000, 0.8660254037844387076, 1.000000000000000000, 0.8660254037844387076, 1.000000000000000000, 0.8660254037844387076, 1.000000000000000000, 0.8660254037844387076, 1.000000000000000000, 0.8660254037844387076, 1.000000000000000000, 0.8660254037844387076, 1.000000000000000000, 0.8660254037844387076, 1.000000000000000000, 0.8660254037844387076, 1.000000000000000000, 0.8660254037844387076, 1.000000000000000000, 0.8660254037844387076, 1.000000000000000000, 0.8660254037844387076, 1.000000000000000000, 0.8660254037844387076, 1.000000000000000000, 0.8660254037844387076, 1.000000000000000000, 0.8660254037844387076, 1.000000000000000000, 0.8660254037844387076, 1.000000000000000000, 0.8660254037844387076, 1.000000000000000000, 0.8660254037844387076, 1.000000000000000000, 0.8660254037844387076, 1.000000000000000000, 0.8660254037844387076, 1.000000000000000000, 0.8660254037844387076, 1.000000000000000000, 0.8660254037844387076, 1.000000000000000000, 0.8660254037844387076, 1.000000000000000000, 0.8660254037844387076, 1.000000000000000000, 0.8660254037844387076, 1.000000000000000000, 0.8660254037844387076, 1.000000000000000000, 0.8660254037844387076, 1.000000000000000000, 0.8660254037844387076, 1.000000000000000000, 0.8660254037844387076, 1.000000000000000000, 0.8660254037844387076, 1.000000000000000000, 0.8660254037844387076, 1.000000000000000000, 0.8660254037844387076, 1.000000000000000000, 0.8660254037844387076, 1.000000000000000000, 0.8660254037844387076, 1.000000000000000000, 0.8660254037844387076, 1.000000000000000000, 0.8660254037844387076, 1.000000000000000000, 0.8660254037844387076, 1.000000000000000000, 0.8660254037844387076, 1.000000000000000000, 0.8660254037844387076, 1.000000000000000000, 0.8660254037844387076, 1.000000000000000000, 0.8660254037844387076, 1.000000000000000000, 0.8660254037844387076, 1.000000000000000000, 0.8660254037844387076, 1.000000000000000000, 0.8660254037844387076, 1.000000000000000000, 0.8660254037844387076, 1.000000000000000000, 0.8660254037844387076, 1.000000000000000000, 0.8660254037844387076, 1.000000000000000000, 0.8660254037844387076, 1.000000000000000000, 0.8660254037844387076, 1.000000000000000000, 0.8660254037844387076, 1.000000000000000000, 0.8660254037844387076, 1.000000000000000000, 0.8660254037844387076, 1.000000000000000000, 0.8660254037844387076, 1.000000000000000000, 0.8660254037844387076, 1.000000000000000000, 0.8660254037844387076, 1.000000000000000000, 0.8660254037844387076, 1.000000000000000000, 0.8660254037844387076, 1.000000000000000000, 0.8660254037844387076, 1.000000000000000000, 0.8660254037844387076, 1.000000000000000000, 0.8660254037844387076, 1.000000000000000000, 0.8660254037844387076, 1.000000000000000000, 0.8660254037844387076, 1.000000000000000000, 0.8660254037844387076, 1.000000000000000000, 0.8660254037844387076, 1.000000000000000000),
 ( 1.000000000000000000, 0.8660254037844387076, 1.000000000000000000, 0.8660254037844387076, 1.000000000000000000, 0.8660254037844387076, 1.000000000000000000, 0.8660254037844387076, 1.000000000000000000, 0.8660254037844387076, 1.000000000000000000, 0.8660254037844387076, 1.000000000000000000, 0.8660254037844387076, 1.000000000000000000, 0.8660254037844387076, 1.000000000000000000, 0.8660254037844387076, 1.000000000000000000, 0.8660254037844387076, 1.000000000000000000, 0.8660254037844387076, 1.000000000000000000, 0.8660254037844387076, 1.000000000000000000, 0.8660254037844387076, 1.000000000000000000, 0.8660254037844387076, 1.000000000000000000, 0.8660254037844387076, 1.000000000000000000, 0.8660254037844387076, 1.000000000000000000, 0.8660254037844387076, 1.000000000000000000, 0.8660254037844387076, 1.000000000000000000, 0.8660254037844387076, 1.000000000000000000, 0.8660254037844387076, 1.000000000000000000, 0.8660254037844387076, 1.000000000000000000, 0.8660254037844387076, 1.000000000000000000, 0.8660254037844387076, 1.000000000000000000, 0.8660254037844387076, 1.000000000000000000, 0.8660254037844387076, 1.000000000000000000, 0.8660254037844387076, 1.000000000000000000, 0.8660254037844387076, 1.000000000000000000, 0.8660254037844387076, 1.000000000000000000, 0.8660254037844387076, 1.000000000000000000, 0.8660254037844387076, 1.000000000000000000, 0.8660254037844387076, 1.000000000000000000, 0.8660254037844387076, 1.000000000000000000, 0.8660254037844387076, 1.000000000000000000, 0.8660254037844387076, 1.000000000000000000, 0.8660254037844387076, 1.000000000000000000, 0.8660254037844387076, 1.000000000000000000, 0.8660254037844387076, 1.000000000000000000, 0.8660254037844387076, 1.000000000000000000, 0.8660254037844387076, 1.000000000000000000, 0.8660254037844387076, 1.000000000000000000, 0.8660254037844387076, 1.000000000000000000, 0.8660254037844387076, 1.000000000000000000, 0.8660254037844387076, 1.000000000000000000, 0.8660254037844387076, 1.000000000000000000, 0.8660254037844387076, 1.000000000000000000, 0.8660254037844387076, 1.000000000000000000, 0.8660254037844387076, 1.000000000000000000, 0.8660254037844387076, 1.000000000000000000, 0.8660254037844387076, 1.000000000000000000, 0.8660254037844387076, 1.000000000000000000, 0.8660254037844387076, 1.000000000000000000, 0.8660254037844387076, 1.000000000000000000, 0.8660254037844387076, 1.000000000000000000, 0.8660254037844387076, 1.000000000000000000, 0.8660254037844387076, 1.000000000000000000, 0.8660254037844387076, 1.000000000000000000, 0.8660254037844387076, 1.000000000000000000, 0.8660254037844387076, 1.000000000000000000, 0.8660254037844387076, 1.000000000000000000, 0.8660254037844387076, 1.000000000000000000, 0.8660254037844387076, 1.000000000000000000, 0.8660254037844387076, 1.000000000000000000, 0.8660254037844387076, 1.000000000000000000, 0.8660254037844387076, 1.000000000000000000, 0.8660254037844387076, 1.000000000000000000, 0.8660254037844387076, 1.000000000000000000, 0.8660254037844387076, 1.000000000000000000, 0.8660254037844387076, 1.000000000000000000, 0.8660254037844387076, 1.000000000000000000, 0.8660254037844387076, 1.000000000000000000, 0.8660254037844387076, 1.000000000000000000, 0.8660254037844387076, 1.000000000000000000, 0.8660254037844387076, 1.000000000000000000, 0.8660254037844387076, 1.000000000000000000, 0.8660254037844387076, 1.000000000000000000, 0.8660254037844387076, 1.000000000000000000, 0.8660254037844387076, 1.000000000000000000, 0.8660254037844387076, 1.000000000000000000, 0.8660254037844387076, 1.000000000000000000, 0.8660254037844387076, 1.000000000000000000, 0.8660254037844387076, 1.000000000000000000, 0.8660254037844387076, 1.000000000000000000, 0.8660254037844387076, 1.000000000000000000, 0.8660254037844387076, 1.000000000000000000, 0.8660254037844387076, 1.000000000000000000, 0.8660254037844387076, 1.000000000000000000, 0.8660254037844387076, 1.000000000000000000, 0.8660254037844387076, 1.000000000000000000, 0.8660254037844387076, 1.000000000000000000, 0.8660254037844387076, 1.000000000000000000, 0.8660254037844387076, 1.000000000000000000, 0.8660254037844387076, 1.000000000000000000, 0.8660254037844387076, 1.000000000000000000, 0.8660254037844387076, 1.000000000000000000, 0.8660254037844387076, 1.000000000000000000, 0.8660254037844387076, 1.000000000000000000, 0.8660254037844387076, 1.000000000000000000, 0.8660254037844387076, 1.000000000000000000, 0.8660254037844387076, 1.000000000000000000, 0.8660254037844387076, 1.000000000000000000, 0.8660254037844387076, 1.000000000000000000, 0.8660254037844387076, 1.000000000000000000, 0.8660254037844387076, 1.000000000000000000, 0.8660254037844387076, 1.000000000000000000, 0.8660254037844387076, 1.000000000000000000, 0.8660254037844387076, 1.000000000000000000, 0.8660254037844387076, 1.000000000000000000, 0.8660254037844387076, 1.000000000000000000, 0.8660254037844387076, 1.000000000000000000, 0.8660254037844387076, 1.000000000000000000, 0.8660254037844387076, 1.000000000000000000, 0.8660254037844387076, 1.000000000000000000, 0.8660254037844387076, 1.000000000000000000, 0.8660254037844387076, 1.000000000000000000, 0.8660254037844387076, 1.000000000000000000, 0.8660254037844387076, 1.000000000000000000, 0.8660254037844387076, 1.000000000000000000, 0.8660254037844387076, 1.000000000000000000, 0.8660254037844387076, 1.000000000000000000, 0.8660254037844387076, 1.000000000000000000) ) ) 
 REPRESENTATION_ITEM ( '' )  SURFACE ( )  );
#182897=CARTESIAN_POINT ( 'NONE',  ( 6.135296122173847344, 5.374195598252329731, -2.500000000000000444 ) ) ;
#182898=CARTESIAN_POINT ( 'NONE',  ( -5.797436685056675643, 7.335035436452395530, -1.304849551618554981 ) ) ;
#182906=CIRCLE ( 'NONE', #44561, 0.4000000000000001332 ) ;
#182916=CARTESIAN_POINT ( 'NONE',  ( 5.468734858265785093, 7.473552982767158070, 1.599625672291269396 ) ) ;
#182938=CARTESIAN_POINT ( 'NONE',  ( 5.830888582329017744, 8.960397891762626799, -1.199719254218452047 ) ) ;
#182939=CARTESIAN_POINT ( 'NONE',  ( 4.766573523656222555, 7.718696989977711809, 1.199719254218452047 ) ) ;
#182941=CARTESIAN_POINT ( 'NONE',  ( 3.542423274920540432, 7.354853930707762721, -1.734723475976807094E-15 ) ) ;
#182955=CARTESIAN_POINT ( 'NONE',  ( 4.708029738644283313, 8.352945002179891887, -0.6661931671527853149 ) ) ;
#182956=CARTESIAN_POINT ( 'NONE',  ( -4.434925645001610128, 8.188180662561590495, 0.7216878364870338292 ) ) ;
#182957=CARTESIAN_POINT ( 'NONE',  ( 3.919715808126649659, 7.587102519540811940, 0.000000000000000000 ) ) ;
#182979=CARTESIAN_POINT ( 'NONE',  ( 3.179715765502636682, 5.975770656120749535, 2.419999999999999485 ) ) ;
#182983=CARTESIAN_POINT ( 'NONE',  ( 7.028976294042106332, 7.165170195996068969, 0.000000000000000000 ) ) ;
#183011=CARTESIAN_POINT ( 'NONE',  ( 7.340813827156391191, 7.528980651296110160, 0.7998128361456281477 ) ) ;
#183015=CARTESIAN_POINT ( 'NONE',  ( -6.081925898509194184, 7.037820769655190212, 1.000852813763454252 ) ) ;
#183016=CARTESIAN_POINT ( 'NONE',  ( 5.365994935958575240, 9.482354201918870018, 0.7998128361456341429 ) ) ;
#183044=CARTESIAN_POINT ( 'NONE',  ( 2.943528747942701695, 6.448217615992859919, 0.000000000000000000 ) ) ;
#183049=CARTESIAN_POINT ( 'NONE',  ( -5.932574734431526942, 9.079031735882207244, 1.199719254218454489 ) ) ;
#183051=CARTESIAN_POINT ( 'NONE',  ( 5.013482942003290255, 9.071090208970993274, -0.7998128361456481317 ) ) ;
#183074=CARTESIAN_POINT ( 'NONE',  ( 7.530627977747744062, 7.750430493652658015, -0.7998128361456341429 ) ) ;
#183083=CARTESIAN_POINT ( 'NONE',  ( 4.927462483923885195, 4.713404084191450849, -0.7998128361456481317 ) ) ;
#183087=ORIENTED_EDGE ( 'NONE', *, *, #149314, .T. ) ;
#183096=CARTESIAN_POINT ( 'NONE',  ( -4.665414256878301025, 6.536345614481700927, -1.443375672974066548 ) ) ;
#183099=CARTESIAN_POINT ( 'NONE',  ( 5.091969210384201361, 8.098325291160362482, 1.199719254218452047 ) ) ;
#183105=CARTESIAN_POINT ( 'NONE',  ( -8.072954122294394352, 8.383144328957069291, -0.7998128361456362523 ) ) ;
#183115=VERTEX_POINT ( 'NONE', #108439 ) ;
#183118=CARTESIAN_POINT ( 'NONE',  ( -0.2255463540285773671, 2.565807686639169471, -1.988980584585362754 ) ) ;
#183148=CARTESIAN_POINT ( 'NONE',  ( 4.258669648468281110, 6.061810238003387141, 1.443375672974058777 ) ) ;
#183153=CARTESIAN_POINT ( 'NONE',  ( 3.366167277942881064, 7.149221934233827014, -0.7998128361456362523 ) ) ;
#183156=CARTESIAN_POINT ( 'NONE',  ( -5.285699784481336927, 7.260012063351913625, 1.599625672291263179 ) ) ;
#183159=ORIENTED_EDGE ( 'NONE', *, *, #71839, .T. ) ;
#183160=CARTESIAN_POINT ( 'NONE',  ( -6.414416072596849538, 7.616478518518682073, -1.082531754730549967 ) ) ;
#183165=VERTEX_POINT ( 'NONE', #209038 ) ;
#183166=CARTESIAN_POINT ( 'NONE',  ( -6.587282531393266360, 8.778525268082516320, 1.599625672291269396 ) ) ;
#183171=ORIENTED_EDGE ( 'NONE', *, *, #13102, .F. ) ;
#183174=CARTESIAN_POINT ( 'NONE',  ( -6.967964602780620353, 7.093989889524320525, 0.000000000000000000 ) ) ;
#183176=CARTESIAN_POINT ( 'NONE',  ( 5.043764445095213489, 7.992138250556588552, 1.161813593947092382 ) ) ;
#183181=CARTESIAN_POINT ( 'NONE',  ( 6.855582950365507244, 8.027210192628430718, -1.199719254218452047 ) ) ;
#183187=CARTESIAN_POINT ( 'NONE',  ( -4.034433228518296666, 6.864533312316751790, -1.199719254218450271 ) ) ;
#183191=CARTESIAN_POINT ( 'NONE',  ( -6.934069218746458318, 7.054445274817795486, -0.7998128361456362523 ) ) ;
#183194=CARTESIAN_POINT ( 'NONE',  ( 7.797347741190739256, 8.269529584243604958, 0.7216878364870267237 ) ) ;
#183196=CARTESIAN_POINT ( 'NONE',  ( -6.956742217143487395, 8.249192353823097790, 1.082531754730549078 ) ) ;
#183202=CARTESIAN_POINT ( 'NONE',  ( 6.343235766347262938, 8.493804042195527870, -1.599625672291281386 ) ) ;
#183216=CARTESIAN_POINT ( 'NONE',  ( 6.304162555737000240, 6.968127521147626346, -0.9177210060461529206 ) ) ;
#183221=CARTESIAN_POINT ( 'NONE',  ( 5.591005849568446706, 5.791977450266268868, -0.7139200525481930182 ) ) ;
#183238=CARTESIAN_POINT ( 'NONE',  ( 4.909461021924244051, 6.821066840368686712, 1.443375672974065660 ) ) ;
#183240=CARTESIAN_POINT ( 'NONE',  ( 8.167861197590044142, 8.493869250135347215, 0.000000000000000000 ) ) ;
#183245=CARTESIAN_POINT ( 'NONE',  ( -6.320392545075788959, 6.875563024200552320, -0.7000339101758262794 ) ) ;
#183263=CARTESIAN_POINT ( 'NONE',  ( -6.317173229324657413, 6.334733287159020954, 0.000000000000000000 ) ) ;
#183277=CARTESIAN_POINT ( 'NONE',  ( 7.530627977747744062, 7.750430493652658015, -0.7998128361456341429 ) ) ;
#183278=CARTESIAN_POINT ( 'NONE',  ( 4.934241560730721510, 4.721313007132757811, 0.000000000000000000 ) ) ;
#183280=CARTESIAN_POINT ( 'NONE',  ( 6.387299765369506055, 7.584842826753462219, -1.082531754730548412 ) ) ;
#183283=EDGE_CURVE ( 'NONE', #142732, #196836, #211421, .T. ) ;
#183294=CARTESIAN_POINT ( 'NONE',  ( -3.949167883330528372, 7.829389307186077396, 1.214306433183764966E-14 ) ) ;
#183295=CARTESIAN_POINT ( 'NONE',  ( 4.529305835417093640, 7.441884687032027657, -1.199719254218450271 ) ) ;
#183303=CARTESIAN_POINT ( 'NONE',  ( -6.050681693448748177, 10.28115541899069463, 0.7998128361456291469 ) ) ;
#183304=CARTESIAN_POINT ( 'NONE',  ( 3.464990776744291345, 6.200183785247111778, 1.199719254218452047 ) ) ;
#183312=CARTESIAN_POINT ( 'NONE',  ( 5.011674058906918638, 5.875983152593414971, 1.199719254218452047 ) ) ;
#183315=CARTESIAN_POINT ( 'NONE',  ( 5.712781623311797397, 7.758274208654143855, -1.599625672291283607 ) ) ;
#183321=CARTESIAN_POINT ( 'NONE',  ( -6.612840081267999714, 6.759580388257274919, -0.1161152146933758927 ) ) ;
#183333=CARTESIAN_POINT ( 'NONE',  ( -3.973948422136981407, 5.729635473950147606, -1.443375672974066548 ) ) ;
#183363=CARTESIAN_POINT ( 'NONE',  ( 5.520104819419390907, 6.469152373191302985, 1.199719254218452935 ) ) ;
#183382=CARTESIAN_POINT ( 'NONE',  ( 0.3985414750882500523, 3.110725714686441989, 2.025316624788002340 ) ) ;
#183384=CARTESIAN_POINT ( 'NONE',  ( 4.030516805012513082, 7.924296382481737844, 0.000000000000000000 ) ) ;
#183385=CARTESIAN_POINT ( 'NONE',  ( -4.340018570150318666, 6.156717313299049366, -1.443375672974066548 ) ) ;
#183410=CARTESIAN_POINT ( 'NONE',  ( -6.414942957921379474, 7.513130201443591005, -1.199719254218452047 ) ) ;
#183413=CARTESIAN_POINT ( 'NONE',  ( 5.844973620822823790, 9.833236634353070826, 0.7216878364870317197 ) ) ;
#183418=CARTESIAN_POINT ( 'NONE',  ( -4.496464221587651799, 5.274905009054215554, 1.199719254218452935 ) ) ;
#183421=CARTESIAN_POINT ( 'NONE',  ( 2.911969131885072670, 6.619324097166378706, 0.000000000000000000 ) ) ;
#183426=CARTESIAN_POINT ( 'NONE',  ( -7.910256278930404505, 8.193330178365746619, -0.7998128361456362523 ) ) ;
#183433=CARTESIAN_POINT ( 'NONE',  ( 4.309512724297349884, 6.121127159803966933, 1.599625672291261402 ) ) ;
#183436=CYLINDRICAL_SURFACE ( 'NONE', #13448, 0.07999999999999972411 ) ;
#183437=CARTESIAN_POINT ( 'NONE',  ( -5.743814354044916470, 6.730146830254374990, -1.199719254218453823 ) ) ;
#183440=CARTESIAN_POINT ( 'NONE',  ( -5.614485009834902840, 9.564333254867113610, 0.7216878364870267237 ) ) ;
#183443=CARTESIAN_POINT ( 'NONE',  ( -7.390603132780795725, 8.755363422066633206, -1.082531754730549967 ) ) ;
#183444=CARTESIAN_POINT ( 'NONE',  ( 4.760321331729593375, 5.686701320840210627, -1.082531754730548412 ) ) ;
#183445=CARTESIAN_POINT ( 'NONE',  ( -4.462041952228954500, 6.299077925724123617, -1.443375672974066548 ) ) ;
#183457=CARTESIAN_POINT ( 'NONE',  ( -0.001670575542712476836, 2.503868101192739282, 2.003409546593375890 ) ) ;
#183461=CARTESIAN_POINT ( 'NONE',  ( -1.833030277982322875, 2.526412122984485364, -2.500000000000015987 ) ) ;
#183462=CARTESIAN_POINT ( 'NONE',  ( 6.567098404289990476, 6.791591158854626720, -0.3517435911668670423 ) ) ;
#183481=CARTESIAN_POINT ( 'NONE',  ( 5.726091835933811325, 7.283405380927965744, -1.209259067671350163 ) ) ;
#183496=CARTESIAN_POINT ( 'NONE',  ( 6.502017186205484300, 9.743381262951846367, -1.199719254218452047 ) ) ;
#183500=CARTESIAN_POINT ( 'NONE',  ( -5.119085517611572378, 8.129960982925583224, 1.199719254218452935 ) ) ;
#183512=CARTESIAN_POINT ( 'NONE',  ( 5.143339171537801846, 7.093924681584509173, 1.599625672291269396 ) ) ;
#183514=CARTESIAN_POINT ( 'NONE',  ( 6.373214726875630731, 9.593111727067046957, 1.199719254218452047 ) ) ;
#183520=CARTESIAN_POINT ( 'NONE',  ( -6.631346530415505036, 7.869564052640446228, 1.082531754730549078 ) ) ;
#183521=ORIENTED_EDGE ( 'NONE', *, *, #80739, .T. ) ;
#183526=CARTESIAN_POINT ( 'NONE',  ( 7.526711554241970248, 8.810193563817646734, -1.199719254218452047 ) ) ;
#183533=CARTESIAN_POINT ( 'NONE',  ( 1.905110947044305725, 8.996536036952683446, 0.7750000000000004663 ) ) ;
#183536=CARTESIAN_POINT ( 'NONE',  ( 5.484430959185961463, 6.043327615839654499, 0.8208683321978844649 ) ) ;
#183540=CARTESIAN_POINT ( 'NONE',  ( -7.132998214565509087, 7.494455136514109661, 0.7216878364870317197 ) ) ;
#183541=CARTESIAN_POINT ( 'NONE',  ( 7.038091139269835317, 7.383730215335837954, 0.000000000000000000 ) ) ;
#183551=CARTESIAN_POINT ( 'NONE',  ( -5.646044625448194410, 5.551749915969804938, 0.000000000000000000 ) ) ;
#183552=CARTESIAN_POINT ( 'NONE',  ( -6.400857919427531684, 9.521399101757175742, 1.082531754730549967 ) ) ;
#183556=CARTESIAN_POINT ( 'NONE',  ( 4.651856102820254968, 7.480896982382013505, -1.082531754730548412 ) ) ;
#183568=CARTESIAN_POINT ( 'NONE',  ( -5.050372967203840879, 7.883769262350217133, 1.105620360010154402 ) ) ;
#183576=CARTESIAN_POINT ( 'NONE',  ( -4.145761110728687804, 8.058748072483927771, -0.7998128361456481317 ) ) ;
#183587=CARTESIAN_POINT ( 'NONE',  ( 3.393283585170187688, 7.180857625999046867, 0.7998128361456271485 ) ) ;
#183592=ORIENTED_EDGE ( 'NONE', *, *, #125545, .F. ) ;
#183597=DIRECTION ( 'NONE',  ( -0.6507913734559641616, -0.7592566023653004592, 0.000000000000000000 ) ) ;
#183617=ORIENTED_EDGE ( 'NONE', *, *, #49896, .F. ) ;
#183624=CARTESIAN_POINT ( 'NONE',  ( 5.511726693494604312, 6.000014001146780629, -0.7850539801177413013 ) ) ;
#183628=CARTESIAN_POINT ( 'NONE',  ( 4.570507181582611267, 8.346359121906111511, 0.000000000000000000 ) ) ;
#183633=CARTESIAN_POINT ( 'NONE',  ( 4.789477563416786765, 4.879958555012922083, 0.4526585511122512284 ) ) ;
#183634=CARTESIAN_POINT ( 'NONE',  ( 5.194182247366868843, 8.113610817686430110, 1.082531754730548412 ) ) ;
#183650=CARTESIAN_POINT ( 'NONE',  ( -7.767895665986912057, 8.027242796598338614, -0.7998128361456362523 ) ) ;
#183659=CARTESIAN_POINT ( 'NONE',  ( -4.625266680917477835, 5.425174544939014964, -1.199719254218453823 ) ) ;
#183661=CARTESIAN_POINT ( 'NONE',  ( 4.217995187182920880, 6.974725914138481642, 1.082531754730549078 ) ) ;
#183668=CARTESIAN_POINT ( 'NONE',  ( -6.261886844665283114, 8.398896966899865646, 1.599625672291269396 ) ) ;
#183674=CARTESIAN_POINT ( 'NONE',  ( -5.641601317062247212, 7.675230518029648508, -1.443375672974066548 ) ) ;
#183677=CARTESIAN_POINT ( 'NONE',  ( -7.286581212701773502, 7.465709267765667789, 0.7998128361456341429 ) ) ;
#183696=CARTESIAN_POINT ( 'NONE',  ( -4.340018570150322219, 5.196348098997705556, -1.082531754730551743 ) ) ;
#183698=CARTESIAN_POINT ( 'NONE',  ( -4.462041952228954500, 6.299077925724123617, -1.443375672974066548 ) ) ;
#183699=CARTESIAN_POINT ( 'NONE',  ( 4.085803189671889157, 5.860132702740892263, -1.599625672291273171 ) ) ;
#183700=CARTESIAN_POINT ( 'NONE',  ( -3.806807270387036368, 7.663301925418665839, 0.000000000000000000 ) ) ;
#183701=CARTESIAN_POINT ( 'NONE',  ( -6.330731382938325602, 6.350551133041632212, 0.7998128361456281477 ) ) ;
#183755=EDGE_CURVE ( 'NONE', #172895, #24495, #116952, .T. ) ;
#183756=CARTESIAN_POINT ( 'NONE',  ( 5.083381250481017410, 4.895309311841474553, 0.7998128361456352531 ) ) ;
#183769=CARTESIAN_POINT ( 'NONE',  ( 4.607663176575717223, 8.357619647684677133, 0.2284409323990380658 ) ) ;
#183773=CARTESIAN_POINT ( 'NONE',  ( 7.024532985656128936, 9.288650798055913427, 1.443375672974065660 ) ) ;
#183776=ORIENTED_EDGE ( 'NONE', *, *, #70214, .F. ) ;
#183777=CARTESIAN_POINT ( 'NONE',  ( -4.925354943514475003, 8.968274210734028529, 0.000000000000000000 ) ) ;
#183784=CARTESIAN_POINT ( 'NONE',  ( -5.899206235277530297, 9.896508017883515862, 0.7216878364870267237 ) ) ;
#183791=CARTESIAN_POINT ( 'NONE',  ( 4.882344714696929877, 8.710169577206153591, -0.7216878364870458196 ) ) ;
#183794=CARTESIAN_POINT ( 'NONE',  ( -5.469788628470539926, 5.346117919495872783, -0.7998128361456362523 ) ) ;
#183805=CARTESIAN_POINT ( 'NONE',  ( 5.391302360089590628, 6.318882837306503575, -1.199719254218452047 ) ) ;
#183806=CARTESIAN_POINT ( 'NONE',  ( 4.411198876399872404, 6.239761003923544713, -1.599625672291273171 ) ) ;
#183831=CARTESIAN_POINT ( 'NONE',  ( 8.167861197590044142, 8.493869250135347215, 0.000000000000000000 ) ) ;
#183834=CARTESIAN_POINT ( 'NONE',  ( 4.435452530326143616, 5.203724702582467998, -1.199719254218452047 ) ) ;
#183839=CARTESIAN_POINT ( 'NONE',  ( 7.028976294042106332, 7.165170195996068969, 0.000000000000000000 ) ) ;
#183843=CARTESIAN_POINT ( 'NONE',  ( 5.573810548993915148, 5.675402860013913475, 0.000000000000000000 ) ) ;
#183847=CARTESIAN_POINT ( 'NONE',  ( 6.536439455564150514, 9.679577560583279450, 1.082531754730549078 ) ) ;
#183858=CARTESIAN_POINT ( 'NONE',  ( 6.039396378094620488, 7.052381734106362821, -1.030794243266313082 ) ) ;
#183859=CARTESIAN_POINT ( 'NONE',  ( -6.780486220610186798, 8.043560357867583832, -1.082531754730549967 ) ) ;
#183865=DIRECTION ( 'NONE',  ( 0.7592566023653044560, -0.6507913734559596097, 8.231876577584280507E-15 ) ) ;
#183890=VERTEX_POINT ( 'NONE', #7387 ) ;
#183894=CARTESIAN_POINT ( 'NONE',  ( 7.028976294042106332, 7.165170195996068969, 0.000000000000000000 ) ) ;
#183896=CARTESIAN_POINT ( 'NONE',  ( 5.176180785367283654, 9.260904359562321275, -0.7998128361456481317 ) ) ;
#183903=( NAMED_UNIT ( * ) PLANE_ANGLE_UNIT ( ) SI_UNIT ( $, .RADIAN. ) );
#183910=CARTESIAN_POINT ( 'NONE',  ( -4.125423880308188629, 8.035021303660014880, -0.7998128361456481317 ) ) ;
#183912=EDGE_CURVE ( 'NONE', #169017, #85779, #27650, .T. ) ;
#183913=CARTESIAN_POINT ( 'NONE',  ( 5.844973620822830895, 8.872867420051733234, 1.082531754730549967 ) ) ;
#183928=CARTESIAN_POINT ( 'NONE',  ( -5.939880696562884310, 9.943961556049767836, 0.7216878364870267237 ) ) ;
#183930=CARTESIAN_POINT ( 'NONE',  ( -6.292392690518214593, 7.474117906093608710, -1.082531754730549967 ) ) ;
#183941=AXIS2_PLACEMENT_3D ( 'NONE', #5389, #42216, #175410 ) ;
#183953=CARTESIAN_POINT ( 'NONE',  ( -4.980641328173854632, 6.904110530993182948, 1.599625672291263179 ) ) ;
#183964=CARTESIAN_POINT ( 'NONE',  ( -4.588266729941921973, 8.494429388143421633, -0.1275441020149002680 ) ) ;
#183982=CARTESIAN_POINT ( 'NONE',  ( 4.877901405866606588, 8.912911750144889567, 0.7998128361456341429 ) ) ;
#183991=FACE_OUTER_BOUND ( 'NONE', #153529, .T. ) ;
#184001=CARTESIAN_POINT ( 'NONE',  ( 5.773793314573267388, 7.829454515125894964, 1.599625672291268286 ) ) ;
#184002=CARTESIAN_POINT ( 'NONE',  ( 5.631432701629774051, 7.663367133358481631, 1.599625672291269396 ) ) ;
#184004=CARTESIAN_POINT ( 'NONE',  ( 5.285699784481295183, 7.260012063351913625, 1.599625672291268286 ) ) ;
#184008=CARTESIAN_POINT ( 'NONE',  ( -4.057819647168310340, 3.809089625685526226, -2.500000000000000888 ) ) ;
#184015=CARTESIAN_POINT ( 'NONE',  ( 4.601768607255383614, 8.481659704624913587, -0.1707596084408805059 ) ) ;
#184016=CARTESIAN_POINT ( 'NONE',  ( -5.980555156959541208, 7.110307450275150210, 1.082531754730549078 ) ) ;
#184017=CARTESIAN_POINT ( 'NONE',  ( 3.770576118376306241, 6.452737000530752276, 1.082531754730549078 ) ) ;
#184038=CARTESIAN_POINT ( 'NONE',  ( -5.289089322662584358, 5.343228095960675716, 0.000000000000000000 ) ) ;
#184043=CARTESIAN_POINT ( 'NONE',  ( 6.343235766347262938, 8.493804042195527870, -1.599625672291281386 ) ) ;
#184051=CARTESIAN_POINT ( 'NONE',  ( 2.547265342226494947E-16, 0.08000000000000020983, -2.080000000000000071 ) ) ;
#184072=CARTESIAN_POINT ( 'NONE',  ( 7.842465510862060896, 8.114240948952696542, 0.000000000000000000 ) ) ;
#184076=CARTESIAN_POINT ( 'NONE',  ( -5.116488771863230589, 7.819496687688390679, 1.149033069458482270 ) ) ;
#184077=CARTESIAN_POINT ( 'NONE',  ( 5.851225812749518695, 8.984124660586543243, -1.199719254218452047 ) ) ;
#184085=CARTESIAN_POINT ( 'NONE',  ( -0.4800000000000000933, 2.999999999999999112, -2.420000000000000373 ) ) ;
#184086=CIRCLE ( 'NONE', #80834, 7.426656976154414558 ) ;
#184094=CARTESIAN_POINT ( 'NONE',  ( -5.398914348987512213, 6.259949555863199677, 2.420000000000001261 ) ) ;
#184103=CARTESIAN_POINT ( 'NONE',  ( 4.475600106286968582, 5.354526557823810151, -1.082531754730548412 ) ) ;
#184107=CARTESIAN_POINT ( 'NONE',  ( -7.944151662964566540, 8.232874793072271657, 0.000000000000000000 ) ) ;
#184109=CARTESIAN_POINT ( 'NONE',  ( 7.361151057576892143, 7.552707420120024828, 0.7998128361456291469 ) ) ;
#184124=CARTESIAN_POINT ( 'NONE',  ( -3.960390268523300339, 7.634556056670224855, 1.214306433183764966E-14 ) ) ;
#184131=CARTESIAN_POINT ( 'NONE',  ( 6.912678218121202534, 9.158153569265168770, 1.599625672291268286 ) ) ;
#184140=CARTESIAN_POINT ( 'NONE',  ( 6.536439455564155843, 8.719208346281938304, 1.443375672974065660 ) ) ;
#184154=CARTESIAN_POINT ( 'NONE',  ( -5.234856708652269042, 7.200695141551334721, 1.443375672974058777 ) ) ;
#184155=VERTEX_POINT ( 'NONE', #14849 ) ;
#184158=CARTESIAN_POINT ( 'NONE',  ( 5.363132282657546490, 8.414682208812571673, -1.199719254218452047 ) ) ;
#184163=CARTESIAN_POINT ( 'NONE',  ( -2.979759899953417612, 6.698413326579433225, 0.7998128361456352531 ) ) ;
#184165=FACE_OUTER_BOUND ( 'NONE', #197287, .T. ) ;
#184177=CARTESIAN_POINT ( 'NONE',  ( -0.1128749944181871995, 2.519999999999980034, -2.000000000000003553 ) ) ;
#184206=CARTESIAN_POINT ( 'NONE',  ( 4.686278372178935392, 5.496354851410763409, 1.199719254218452047 ) ) ;
#184209=CARTESIAN_POINT ( 'NONE',  ( -4.716257332707368910, 6.595662536282280719, -1.599625672291271394 ) ) ;
#184213=CARTESIAN_POINT ( 'NONE',  ( -4.611181641979265500, 8.393812659035525314, 0.000000000000000000 ) ) ;
#184214=DIRECTION ( 'NONE',  ( 0.000000000000000000, 0.000000000000000000, -1.000000000000000000 ) ) ;
#184218=CARTESIAN_POINT ( 'NONE',  ( -7.110325215724114578, 7.260077271291732082, 0.000000000000000000 ) ) ;
#184219=AXIS2_PLACEMENT_3D ( 'NONE', #81285, #147361, #213388 ) ;
#184226=CARTESIAN_POINT ( 'NONE',  ( -5.094831863685302942, 9.165997284266655498, 0.7998128361456291469 ) ) ;
#184228=CARTESIAN_POINT ( 'NONE',  ( 4.597876849858236525, 8.486543085689454813, -0.1053875944492469602 ) ) ;
#184231=DIRECTION ( 'NONE',  ( 0.000000000000000000, 0.000000000000000000, -1.000000000000000000 ) ) ;
#184233=CARTESIAN_POINT ( 'NONE',  ( 6.749980374757213575, 8.968339418673846097, 1.599625672291268286 ) ) ;
#184240=CARTESIAN_POINT ( 'NONE',  ( -6.143779885648060102, 7.196773283791382703, 1.199719254218452047 ) ) ;
#184245=CARTESIAN_POINT ( 'NONE',  ( -6.882699257592852504, 8.058845884393651460, -1.199719254218452047 ) ) ;
#184250=CARTESIAN_POINT ( 'NONE',  ( -7.607533590599451223, 9.008448956188397361, 1.082531754730549078 ) ) ;
#184257=CARTESIAN_POINT ( 'NONE',  ( 5.722423353419669567, 8.833855124701747386, 1.199719254218451159 ) ) ;
#184272=CARTESIAN_POINT ( 'NONE',  ( 5.120401779693986910, 7.917229619699595489, -1.217862772375446712 ) ) ;
#184296=ORIENTED_EDGE ( 'NONE', *, *, #147140, .F. ) ;
#184300=CARTESIAN_POINT ( 'NONE',  ( -6.155278136343885542, 7.070130543739276519, 1.092798041965221900 ) ) ;
#184318=CARTESIAN_POINT ( 'NONE',  ( -5.981082042284069367, 7.006959133200059142, 1.199719254218452935 ) ) ;
#184336=CARTESIAN_POINT ( 'NONE',  ( 4.694866332082116678, 8.699370830729650450, 0.7998128361456341429 ) ) ;
#184340=CARTESIAN_POINT ( 'NONE',  ( 5.844973620822835336, 7.912498205750389424, 1.443375672974064550 ) ) ;
#184346=CARTESIAN_POINT ( 'NONE',  ( -6.326802395788107880, 6.950450678040672514, 0.9045734915664763731 ) ) ;
#184354=CARTESIAN_POINT ( 'NONE',  ( -4.111865726694519552, 8.019203457777400956, 0.000000000000000000 ) ) ;
#184355=CARTESIAN_POINT ( 'NONE',  ( 4.746236293235721604, 7.694970221153795364, 1.199719254218451159 ) ) ;
#184363=CARTESIAN_POINT ( 'NONE',  ( -4.167152111353897403, 5.955039778036558040, 1.599625672291270506 ) ) ;
#184364=CARTESIAN_POINT ( 'NONE',  ( 5.246079093845007257, 5.085123462432798114, 0.7998128361456352531 ) ) ;
#184370=ORIENTED_EDGE ( 'NONE', *, *, #10253, .T. ) ;
#184372=CARTESIAN_POINT ( 'NONE',  ( 6.008198349511364000, 7.038594824965278995, 1.199719254218453823 ) ) ;
#184378=CARTESIAN_POINT ( 'NONE',  ( -4.725015201957559086, 8.329469486225510977, 0.7380969479929339050 ) ) ;
#184383=CARTESIAN_POINT ( 'NONE',  ( 2.972313222866368676, 6.545497292499366182, 0.5012468031770876964 ) ) ;
#184388=CARTESIAN_POINT ( 'NONE',  ( -4.462041952228957165, 5.338708711422782471, -1.082531754730549967 ) ) ;
#184398=CARTESIAN_POINT ( 'NONE',  ( 3.770576118376306241, 6.452737000530752276, 1.082531754730549078 ) ) ;
#184401=CARTESIAN_POINT ( 'NONE',  ( -3.853900823548995991, 8.531065964593981477, 2.447540105570293001 ) ) ;
#184402=CARTESIAN_POINT ( 'NONE',  ( -6.445975688654487001, 6.485002823043819475, -0.7998128361456362523 ) ) ;
#184408=CARTESIAN_POINT ( 'NONE',  ( -5.823017895876262173, 7.308274721394978357, -1.333157625313810879 ) ) ;
#184421=CARTESIAN_POINT ( 'NONE',  ( 4.278479993564246797, 7.149254538203735798, 1.199719254218452047 ) ) ;
#184440=CARTESIAN_POINT ( 'NONE',  ( 0.1939103488286992305, 3.363703174398338547, 1.993194580354152867 ) ) ;
#184442=CARTESIAN_POINT ( 'NONE',  ( 6.066347387471824781, 6.042103138330730872, -0.7998128361456481317 ) ) ;
#184443=CARTESIAN_POINT ( 'NONE',  ( -4.502716413514301408, 7.306900678191715848, -1.082531754730549967 ) ) ;
#184466=CARTESIAN_POINT ( 'NONE',  ( -7.279802135894939852, 7.457800344824362604, -0.7998128361456362523 ) ) ;
#184479=CARTESIAN_POINT ( 'NONE',  ( -5.912237504011027767, 9.055304967058290799, 1.199719254218454489 ) ) ;
#184486=CARTESIAN_POINT ( 'NONE',  ( 3.715816618597135523, 6.492813934075403637, -1.199719254218453823 ) ) ;
#184491=CARTESIAN_POINT ( 'NONE',  ( -5.773793314573309132, 7.829454515125894964, 1.599625672291263179 ) ) ;
#184495=CARTESIAN_POINT ( 'NONE',  ( -6.455090533882193782, 9.584670485287619002, -1.082531754730549967 ) ) ;
#184498=CARTESIAN_POINT ( 'NONE',  ( -7.905812970100109638, 8.396072351304486148, 0.7216878364870317197 ) ) ;
#184499=CARTESIAN_POINT ( 'NONE',  ( 5.221298554594243413, 5.264138866547622975, -0.7216878364870458196 ) ) ;
#184500=CARTESIAN_POINT ( 'NONE',  ( -4.543390873910949423, 6.393985001019784953, 1.443375672974058777 ) ) ;
#184517=CARTESIAN_POINT ( 'NONE',  ( 6.597622414017595638, 6.771646741010207471, 0.1687998040609314243 ) ) ;
#184522=CARTESIAN_POINT ( 'NONE',  ( -3.188928480291423728, 8.980740528189222971, 2.451733079074398969 ) ) ;
#184536=CARTESIAN_POINT ( 'NONE',  ( 6.170003545802125622, 6.961323287618347955, -0.9016653442153206299 ) ) ;
#184555=CARTESIAN_POINT ( 'NONE',  ( 5.826972158823246595, 10.02016096192762085, -0.7998128361456481317 ) ) ;
#184558=CARTESIAN_POINT ( 'NONE',  ( -6.119526231721793330, 8.232809585132461194, 1.599625672291263179 ) ) ;
#184570=CARTESIAN_POINT ( 'NONE',  ( 4.552505719138623341, 8.533283448962240669, 0.7998128361456341429 ) ) ;
#184578=CARTESIAN_POINT ( 'NONE',  ( -6.251718229232856139, 8.387033582228697881, -1.443375672974066548 ) ) ;
#184584=CARTESIAN_POINT ( 'NONE',  ( 5.365994935958575240, 9.482354201918870018, 0.7998128361456341429 ) ) ;
#184594=EDGE_LOOP ( 'NONE', ( #57403, #188495, #33431, #140526 ) ) ;
#184598=CARTESIAN_POINT ( 'NONE',  ( -6.644904684473536882, 6.925012684740138980, 0.7216878364870317197 ) ) ;
#184599=CARTESIAN_POINT ( 'NONE',  ( 4.746763178560241769, 8.551991118380046331, 0.7216878364870328300 ) ) ;
#184601=DIRECTION ( 'NONE',  ( 0.000000000000000000, 0.000000000000000000, -1.000000000000000000 ) ) ;
#184609=CARTESIAN_POINT ( 'NONE',  ( -4.472210567661380587, 6.310941310395290493, 1.599625672291270506 ) ) ;
#184610=CARTESIAN_POINT ( 'NONE',  ( -4.767627293860968507, 5.591261926706423857, -1.199719254218453823 ) ) ;
#184612=CARTESIAN_POINT ( 'NONE',  ( 7.010974831598141499, 7.352094523052197239, -0.7216878364870317197 ) ) ;
#184625=CARTESIAN_POINT ( 'NONE',  ( -4.627894000755552462, 8.353582960325299567, 0.3099817540855500653 ) ) ;
#184629=CARTESIAN_POINT ( 'NONE',  ( -0.1018178655972588748, 3.468664187816145716, -1.997505796056266547 ) ) ;
#184633=CARTESIAN_POINT ( 'NONE',  ( -4.956387674247580755, 7.940146832334256111, 1.199719254218452935 ) ) ;
#184645=CARTESIAN_POINT ( 'NONE',  ( 7.512626515748109135, 8.897724035528543851, 1.082531754730549967 ) ) ;
#184682=CARTESIAN_POINT ( 'NONE',  ( 6.400857919427532572, 6.640291458853147866, -0.7216878364870458196 ) ) ;
#184687=CARTESIAN_POINT ( 'NONE',  ( 5.031484404002867450, 8.884165881396448583, 0.7216878364870317197 ) ) ;
#184701=CARTESIAN_POINT ( 'NONE',  ( -7.282664789195997912, 8.525472337930658284, 1.199719254218452047 ) ) ;
#184710=CARTESIAN_POINT ( 'NONE',  ( 5.031484404002891431, 5.042689024191078673, 0.7216878364870328300 ) ) ;
#184716=CARTESIAN_POINT ( 'NONE',  ( -7.259464905474441565, 7.434073576000447048, -0.7998128361456362523 ) ) ;
#184721=CARTESIAN_POINT ( 'NONE',  ( -6.794044374223859428, 7.099008989448849505, 0.000000000000000000 ) ) ;
#184724=CARTESIAN_POINT ( 'NONE',  ( -7.435720902452096936, 7.639705572474380091, 0.000000000000000000 ) ) ;
#184744=CARTESIAN_POINT ( 'NONE',  ( -3.797692425603673705, 6.484372692295976570, 1.082531754730549967 ) ) ;
#184746=CARTESIAN_POINT ( 'NONE',  ( -5.302647476276252547, 5.359045941843285199, 0.7216878364870257245 ) ) ;
#184748=CARTESIAN_POINT ( 'NONE',  ( 5.923986774528332333, 5.876015756563318426, -0.7998128361456481317 ) ) ;
#184749=CARTESIAN_POINT ( 'NONE',  ( -3.980200614063634568, 6.801261928786307642, 1.199719254218452935 ) ) ;
#184750=CARTESIAN_POINT ( 'NONE',  ( -5.582925393777276035, 9.735439736040634173, 0.7998128361456291469 ) ) ;
#184806=CARTESIAN_POINT ( 'NONE',  ( 4.760848217054122422, 5.583353003765119560, -1.199719254218452047 ) ) ;
#184808=CARTESIAN_POINT ( 'NONE',  ( -3.903294069008378830, 8.999999999999998224, -0.7749999999999979128 ) ) ;
#184819=CARTESIAN_POINT ( 'NONE',  ( 4.644395130292630292, 8.311692339142366492, -0.4369040224408097250 ) ) ;
#184822=CARTESIAN_POINT ( 'NONE',  ( 5.174371902270911150, 6.065797303184739420, 1.199719254218452047 ) ) ;
#184828=CARTESIAN_POINT ( 'NONE',  ( -6.505933609711270549, 8.683618192786854095, -1.599625672291271394 ) ) ;
#184844=CARTESIAN_POINT ( 'NONE',  ( 6.129694847154206983, 8.244672969803623630, -1.443375672974078761 ) ) ;
#184848=CARTESIAN_POINT ( 'NONE',  ( -5.586841817283045408, 8.675676665875643678, 1.199719254218454489 ) ) ;
#184855=VERTEX_POINT ( 'NONE', #159798 ) ;
#184859=CARTESIAN_POINT ( 'NONE',  ( 5.578253857379852576, 5.472660686556754861, -0.7998128361456481317 ) ) ;
#184860=CARTESIAN_POINT ( 'NONE',  ( 4.715203562502613188, 8.723097599553565118, 0.7998128361456341429 ) ) ;
#184881=CARTESIAN_POINT ( 'NONE',  ( 5.348589505275513467, 7.707351500233518671, -1.315919829448284784 ) ) ;
#184885=CARTESIAN_POINT ( 'NONE',  ( 1.886825320689258012, 2.480000000000016858, -2.459652456995881753 ) ) ;
#184888=CARTESIAN_POINT ( 'NONE',  ( 4.869313445963426190, 5.709895770826003414, 1.199719254218452935 ) ) ;
#184893=CARTESIAN_POINT ( 'NONE',  ( 5.006703865196457492, 9.063181286029688977, 0.000000000000000000 ) ) ;
#184898=CARTESIAN_POINT ( 'NONE',  ( 4.258669648468268676, 7.982548666606070320, 0.7216878364870257245 ) ) ;
#184901=CARTESIAN_POINT ( 'NONE',  ( 3.390420931869152721, 6.113185632892752075, -1.199719254218452047 ) ) ;
#184913=CARTESIAN_POINT ( 'NONE',  ( 6.435429789636040177, 6.784273175954743884, -0.4071148367965071735 ) ) ;
#184914=CARTESIAN_POINT ( 'NONE',  ( -6.238160076063538284, 9.331584951165851294, 1.082531754730549967 ) ) ;
#184921=CARTESIAN_POINT ( 'NONE',  ( -5.548322005359108466, 5.928160571233643594, 0.7412397383242540494 ) ) ;
#184945=CARTESIAN_POINT ( 'NONE',  ( 5.508355548902068577, 9.648441583686274470, 0.7998128361456331437 ) ) ;
#184947=CARTESIAN_POINT ( 'NONE',  ( 6.282224075085741433, 8.422623735723785643, 1.599625672291268286 ) ) ;
#184961=CARTESIAN_POINT ( 'NONE',  ( -6.310394152517827315, 6.326824364217716656, 0.7998128361456281477 ) ) ;
#184963=CARTESIAN_POINT ( 'NONE',  ( 5.600926855776875435, 7.627776979863398310, -1.443375672974078761 ) ) ;
#184973=CARTESIAN_POINT ( 'NONE',  ( -3.634467696915153034, 6.397906858779740524, 1.199719254218452935 ) ) ;
#184980=CARTESIAN_POINT ( 'NONE',  ( -5.953438850176548947, 9.959779401932374654, 0.000000000000000000 ) ) ;
#184981=ORIENTED_EDGE ( 'NONE', *, *, #77886, .T. ) ;
#184982=CARTESIAN_POINT ( 'NONE',  ( -4.963693636378939011, 8.805076652501815815, 0.7216878364870267237 ) ) ;
#184992=CARTESIAN_POINT ( 'NONE',  ( 6.204464077730128757, 7.037555732820855781, 1.030856974308017149 ) ) ;
#184994=EDGE_CURVE ( 'NONE', #160443, #65240, #82682, .T. ) ;
#185008=CARTESIAN_POINT ( 'NONE',  ( -6.642568916052639771, 6.714361588341672515, 0.000000000000000000 ) ) ;
#185017=CARTESIAN_POINT ( 'NONE',  ( 2.296870906627769049, 2.697687087511395632, -2.500000000000000444 ) ) ;
#185018=CARTESIAN_POINT ( 'NONE',  ( -4.780157383859068077, 8.266535928781179265, -0.8537241328121815132 ) ) ;
#185042=CARTESIAN_POINT ( 'NONE',  ( 1.844607821789259638, 8.931289555339859021, -0.7749999999999996891 ) ) ;
#185050=CARTESIAN_POINT ( 'NONE',  ( 5.896870467300973750, 5.844380064798101237, 0.7998128361456352531 ) ) ;
#185058=CARTESIAN_POINT ( 'NONE',  ( 5.061990249855835344, 6.999017606288844284, -1.599625672291273171 ) ) ;
#185060=CARTESIAN_POINT ( 'NONE',  ( 4.044074958626150185, 7.940114228364351767, 0.7998128361456271485 ) ) ;
#185073=CARTESIAN_POINT ( 'NONE',  ( 5.788239156490550208, 7.236076679697275083, -1.185412701995581797 ) ) ;
#185075=CARTESIAN_POINT ( 'NONE',  ( -4.950135482320914271, 8.789258806100786359, -0.7216878364870338292 ) ) ;
#185076=CARTESIAN_POINT ( 'NONE',  ( 4.990809943606266508, 6.915973915664348937, -1.443375672974068769 ) ) ;
#185088=ORIENTED_EDGE ( 'NONE', *, *, #200712, .T. ) ;
#185093=CARTESIAN_POINT ( 'NONE',  ( -4.285785955251283141, 8.014184357852876417, 0.000000000000000000 ) ) ;
#185098=CARTESIAN_POINT ( 'NONE',  ( 6.717138760927786834, 6.801359740696030443, -0.7998128361456481317 ) ) ;
#185129=CARTESIAN_POINT ( 'NONE',  ( 7.856023664475727308, 8.130058794835305136, -0.7998128361456341429 ) ) ;
#185160=CARTESIAN_POINT ( 'NONE',  ( 4.340018570150304456, 6.156717313299049366, -1.443375672974068769 ) ) ;
#185166=CARTESIAN_POINT ( 'NONE',  ( -4.327421261425478782, 8.660439569662104375, -0.7750000000000001332 ) ) ;
#185168=CARTESIAN_POINT ( 'NONE',  ( 7.550965208168244125, 7.774157262476569130, -0.7998128361456341429 ) ) ;
#185172=CARTESIAN_POINT ( 'NONE',  ( -3.472296738875691346, 6.104744391113324120, 1.082531754730549967 ) ) ;
#185175=VERTEX_POINT ( 'NONE', #26593 ) ;
#185178=( BOUNDED_SURFACE ( )  B_SPLINE_SURFACE ( 1, 2, ( 
 ( #22473, #153575, #141634, #9450, #55007, #71221, #24618, #173036, #154642, #53938, #186050, #7292, #124363, #41979, #21401, #23548, #88584, #138401, #140562, #90726, #75521, #190320, #204420, #73370, #108089, #25691, #187124, #120074, #171959, #37685, #169813, #6223, #104836, #205504, #188191, #139475, #189267, #170881, #72293, #56075, #39826, #76579, #113428, #159974, #61406, #92863, #210842, #62468, #11578, #77649, #143771, #94996, #63540, #29979, #128630, #111292, #80859, #109163, #209765, #28911, #27837, #127568, #158910, #43050, #78708, #110227, #207642, #176235, #193537, #96065, #161042, #31055, #194597, #45179, #12637, #79780, #144834, #195678, #177297, #46241, #112358, #162117, #178371, #13707, #145892, #211903, #129695, #47314, #26762, #191384, #208701, #179434, #59261, #97131, #10506, #163183, #142691, #14768, #125418, #175174, #60328, #126489, #192452, #44106, #93933, #36345, #150126, #147999, #1699, #146949, #98190, #32105, #151190, #212964, #65632, #134953, #115541, #117682, #130743, #67753, #133903, #199910, #164238, #197783, #15826, #81911, #64602, #180486, #33164, #2762, #50483, #17950, #166360, #149043, #34220, #183674, #131780, #618, #20091, #196736, #35278, #48377, #101355, #181536, #49421, #114489, #165294, #132833, #66686, #200961, #184721, #52608, #116603, #84037, #99245, #51556, #214009, #16888, #198837, #82970, #182597, #100293, #167433, #19025, #85105, #68831, #118737, #102423, #168491, #56879, #120893, #138144, #5961, #40649, #41725, #190073, #69893, #106752, #8120, #104575, #169559, #170620, #154384, #57945, #23286, #87244, #39560, #105662, #152248, #37422, #107835, #153310, #89398, #204154, #186867, #136005, #72032, #124110, #103498, #38497, #24353, #202018, #21141, #119809, #55809, #70963, #172779, #121963, #90462, #155446, #4885, #156529, #137073, #74207, #203098, #187930, #53677, #54743, #73107, #173860, #140302, #189008, #171689, #86178, #139207, #22207, #7030, #206320, #205238, #3821, #88320, #123054, #185788, #128381, #109973, #209507, #160789, #61147, #193280, #44925, #59012 ),
 ( #177039, #12381, #92614, #145651, #78461, #208443, #125169, #113174, #129445, #108903, #191128, #210593, #144579, #126235, #25436, #157601, #111033, #95811, #13457, #207392, #127309, #60077, #175984, #112111, #62223, #47057, #194348, #27577, #28656, #79533, #211647, #174926, #45990, #143511, #178114, #75267, #192195, #42794, #94742, #93676, #29729, #161867, #10256, #141382, #76330, #63283, #26506, #195427, #43859, #159718, #158657, #91542, #9196, #11316, #77395, #142436, #69380, #37978, #4371, #36896, #85653, #55295, #80603, #184209, #3310, #2239, #200450, #133379, #14511, #53158, #84591, #179177, #150678, #101910, #135488, #162930, #67244, #30801, #71515, #51030, #1180, #152791, #20633, #68316, #96880, #146698, #201510, #104051, #170097, #199384, #151740, #134447, #52096, #54230, #86722, #203644, #169036, #118223, #119287, #21683, #87793, #117153, #70441, #185273, #120368, #183156, #35832, #34759, #102978, #167975, #136557, #202578, #166918, #100833, #18512, #186343, #19581, #153867, #5436, #137627, #6515, #124647, #190604, #139768, #205794, #57424, #8663, #191665, #158139, #42262, #24906, #208979, #22760, #123586, #157074, #155997, #189549, #72591, #171170, #206859, #23839, #121445, #89947, #41197, #74743, #105130, #175454, #92082, #7584, #207925, #88877, #75805, #43329, #107304, #204709, #173328, #91012, #93147, #58491, #122522, #140847, #108375, #187414, #138692, #10785, #188485, #174398, #25976, #73669, #154930, #9730, #141913, #56359, #40115, #59547, #125706, #159184, #39045, #172252, #109447, #27038, #106226, #76860, #142979, #60616, #195964, #164523, #131025, #62742, #163466, #177581, #146167, #80065, #129977, #63819, #13981, #31334, #176509, #212182, #47599, #127858, #180765, #113713, #29195, #48652, #32393, #144055, #179717, #178651, #147224, #110509, #95284, #160255, #97411, #128902, #30262, #15046, #45457, #28121, #111573, #213249, #210050, #98459, #12916, #194883, #11856, #81139, #64879, #78996, #145112, #211118, #162403, #197016, #114769, #16108, #96348, #148286, #94215, #46520, #82192, #161332 ) ),
 .UNSPECIFIED., .F., .F., .F. ) 
 B_SPLINE_SURFACE_WITH_KNOTS ( ( 2, 2 ),
 ( 3, 2, 2, 2, 2, 2, 2, 2, 2, 2, 2, 2, 2, 2, 2, 2, 2, 2, 2, 2, 2, 2, 2, 2, 2, 2, 2, 2, 2, 2, 2, 2, 2, 2, 2, 2, 2, 2, 2, 2, 2, 2, 2, 2, 2, 2, 2, 2, 2, 2, 2, 2, 2, 2, 2, 2, 2, 2, 2, 2, 2, 2, 2, 2, 2, 2, 2, 2, 2, 2, 2, 2, 2, 2, 2, 2, 2, 2, 2, 2, 2, 2, 2, 2, 2, 2, 2, 2, 2, 2, 2, 2, 2, 2, 2, 2, 2, 2, 2, 2, 2, 2, 2, 2, 2, 2, 2, 2, 2, 2, 2, 2, 2, 2, 2, 2, 2, 2, 2, 2, 3 ),
 ( 0.000000000000000000, 1.000000000000000000 ),
 ( 0.000000000000000000, 0.008333333333333333218, 0.01666666666666666644, 0.02500000000000000139, 0.03333333333333333287, 0.04166666666666666435, 0.05000000000000000278, 0.05833333333333333426, 0.06666666666666666574, 0.07499999999999999722, 0.08333333333333332871, 0.09166666666666666019, 0.1000000000000000056, 0.1083333333333333370, 0.1166666666666666685, 0.1250000000000000000, 0.1333333333333333315, 0.1416666666666666630, 0.1499999999999999944, 0.1583333333333333259, 0.1666666666666666574, 0.1749999999999999889, 0.1833333333333333204, 0.1916666666666666796, 0.2000000000000000111, 0.2083333333333333426, 0.2166666666666666741, 0.2250000000000000056, 0.2333333333333333370, 0.2416666666666666685, 0.2500000000000000000, 0.2583333333333333592, 0.2666666666666666630, 0.2750000000000000222, 0.2833333333333333259, 0.2916666666666666852, 0.2999999999999999889, 0.3083333333333333481, 0.3166666666666666519, 0.3250000000000000111, 0.3333333333333333148, 0.3416666666666666741, 0.3499999999999999778, 0.3583333333333333370, 0.3666666666666666408, 0.3750000000000000000, 0.3833333333333333592, 0.3916666666666666630, 0.4000000000000000222, 0.4083333333333333259, 0.4166666666666666852, 0.4249999999999999889, 0.4333333333333333481, 0.4416666666666666519, 0.4500000000000000111, 0.4583333333333333148, 0.4666666666666666741, 0.4749999999999999778, 0.4833333333333333370, 0.4916666666666666408, 0.5000000000000000000, 0.5083333333333333037, 0.5166666666666667185, 0.5250000000000000222, 0.5333333333333333259, 0.5416666666666666297, 0.5500000000000000444, 0.5583333333333333481, 0.5666666666666666519, 0.5749999999999999556, 0.5833333333333333703, 0.5916666666666666741, 0.5999999999999999778, 0.6083333333333332815, 0.6166666666666666963, 0.6250000000000000000, 0.6333333333333333037, 0.6416666666666667185, 0.6500000000000000222, 0.6583333333333333259, 0.6666666666666666297, 0.6750000000000000444, 0.6833333333333333481, 0.6916666666666666519, 0.6999999999999999556, 0.7083333333333333703, 0.7166666666666666741, 0.7249999999999999778, 0.7333333333333332815, 0.7416666666666666963, 0.7500000000000000000, 0.7583333333333333037, 0.7666666666666667185, 0.7750000000000000222, 0.7833333333333333259, 0.7916666666666666297, 0.8000000000000000444, 0.8083333333333333481, 0.8166666666666666519, 0.8249999999999999556, 0.8333333333333333703, 0.8416666666666666741, 0.8499999999999999778, 0.8583333333333332815, 0.8666666666666666963, 0.8750000000000000000, 0.8833333333333333037, 0.8916666666666667185, 0.9000000000000000222, 0.9083333333333333259, 0.9166666666666666297, 0.9250000000000000444, 0.9333333333333333481, 0.9416666666666666519, 0.9499999999999999556, 0.9583333333333333703, 0.9666666666666666741, 0.9749999999999999778, 0.9833333333333332815, 0.9916666666666666963, 1.000000000000000000 ),
 .UNSPECIFIED. ) 
 GEOMETRIC_REPRESENTATION_ITEM ( )  RATIONAL_B_SPLINE_SURFACE ( (
 ( 1.000000000000000000, 0.8660254037844387076, 1.000000000000000000, 0.8660254037844387076, 1.000000000000000000, 0.8660254037844387076, 1.000000000000000000, 0.8660254037844387076, 1.000000000000000000, 0.8660254037844387076, 1.000000000000000000, 0.8660254037844387076, 1.000000000000000000, 0.8660254037844387076, 1.000000000000000000, 0.8660254037844387076, 1.000000000000000000, 0.8660254037844387076, 1.000000000000000000, 0.8660254037844387076, 1.000000000000000000, 0.8660254037844387076, 1.000000000000000000, 0.8660254037844387076, 1.000000000000000000, 0.8660254037844387076, 1.000000000000000000, 0.8660254037844387076, 1.000000000000000000, 0.8660254037844387076, 1.000000000000000000, 0.8660254037844387076, 1.000000000000000000, 0.8660254037844387076, 1.000000000000000000, 0.8660254037844387076, 1.000000000000000000, 0.8660254037844387076, 1.000000000000000000, 0.8660254037844387076, 1.000000000000000000, 0.8660254037844387076, 1.000000000000000000, 0.8660254037844387076, 1.000000000000000000, 0.8660254037844387076, 1.000000000000000000, 0.8660254037844387076, 1.000000000000000000, 0.8660254037844387076, 1.000000000000000000, 0.8660254037844387076, 1.000000000000000000, 0.8660254037844387076, 1.000000000000000000, 0.8660254037844387076, 1.000000000000000000, 0.8660254037844387076, 1.000000000000000000, 0.8660254037844387076, 1.000000000000000000, 0.8660254037844387076, 1.000000000000000000, 0.8660254037844387076, 1.000000000000000000, 0.8660254037844387076, 1.000000000000000000, 0.8660254037844387076, 1.000000000000000000, 0.8660254037844387076, 1.000000000000000000, 0.8660254037844387076, 1.000000000000000000, 0.8660254037844387076, 1.000000000000000000, 0.8660254037844387076, 1.000000000000000000, 0.8660254037844387076, 1.000000000000000000, 0.8660254037844387076, 1.000000000000000000, 0.8660254037844387076, 1.000000000000000000, 0.8660254037844387076, 1.000000000000000000, 0.8660254037844387076, 1.000000000000000000, 0.8660254037844387076, 1.000000000000000000, 0.8660254037844387076, 1.000000000000000000, 0.8660254037844387076, 1.000000000000000000, 0.8660254037844387076, 1.000000000000000000, 0.8660254037844387076, 1.000000000000000000, 0.8660254037844387076, 1.000000000000000000, 0.8660254037844387076, 1.000000000000000000, 0.8660254037844387076, 1.000000000000000000, 0.8660254037844387076, 1.000000000000000000, 0.8660254037844387076, 1.000000000000000000, 0.8660254037844387076, 1.000000000000000000, 0.8660254037844387076, 1.000000000000000000, 0.8660254037844387076, 1.000000000000000000, 0.8660254037844387076, 1.000000000000000000, 0.8660254037844387076, 1.000000000000000000, 0.8660254037844387076, 1.000000000000000000, 0.8660254037844387076, 1.000000000000000000, 0.8660254037844387076, 1.000000000000000000, 0.8660254037844387076, 1.000000000000000000, 0.8660254037844387076, 1.000000000000000000, 0.8660254037844387076, 1.000000000000000000, 0.8660254037844387076, 1.000000000000000000, 0.8660254037844387076, 1.000000000000000000, 0.8660254037844387076, 1.000000000000000000, 0.8660254037844387076, 1.000000000000000000, 0.8660254037844387076, 1.000000000000000000, 0.8660254037844387076, 1.000000000000000000, 0.8660254037844387076, 1.000000000000000000, 0.8660254037844387076, 1.000000000000000000, 0.8660254037844387076, 1.000000000000000000, 0.8660254037844387076, 1.000000000000000000, 0.8660254037844387076, 1.000000000000000000, 0.8660254037844387076, 1.000000000000000000, 0.8660254037844387076, 1.000000000000000000, 0.8660254037844387076, 1.000000000000000000, 0.8660254037844387076, 1.000000000000000000, 0.8660254037844387076, 1.000000000000000000, 0.8660254037844387076, 1.000000000000000000, 0.8660254037844387076, 1.000000000000000000, 0.8660254037844387076, 1.000000000000000000, 0.8660254037844387076, 1.000000000000000000, 0.8660254037844387076, 1.000000000000000000, 0.8660254037844387076, 1.000000000000000000, 0.8660254037844387076, 1.000000000000000000, 0.8660254037844387076, 1.000000000000000000, 0.8660254037844387076, 1.000000000000000000, 0.8660254037844387076, 1.000000000000000000, 0.8660254037844387076, 1.000000000000000000, 0.8660254037844387076, 1.000000000000000000, 0.8660254037844387076, 1.000000000000000000, 0.8660254037844387076, 1.000000000000000000, 0.8660254037844387076, 1.000000000000000000, 0.8660254037844387076, 1.000000000000000000, 0.8660254037844387076, 1.000000000000000000, 0.8660254037844387076, 1.000000000000000000, 0.8660254037844387076, 1.000000000000000000, 0.8660254037844387076, 1.000000000000000000, 0.8660254037844387076, 1.000000000000000000, 0.8660254037844387076, 1.000000000000000000, 0.8660254037844387076, 1.000000000000000000, 0.8660254037844387076, 1.000000000000000000, 0.8660254037844387076, 1.000000000000000000, 0.8660254037844387076, 1.000000000000000000, 0.8660254037844387076, 1.000000000000000000, 0.8660254037844387076, 1.000000000000000000, 0.8660254037844387076, 1.000000000000000000, 0.8660254037844387076, 1.000000000000000000, 0.8660254037844387076, 1.000000000000000000, 0.8660254037844387076, 1.000000000000000000, 0.8660254037844387076, 1.000000000000000000, 0.8660254037844387076, 1.000000000000000000, 0.8660254037844387076, 1.000000000000000000, 0.8660254037844387076, 1.000000000000000000, 0.8660254037844387076, 1.000000000000000000, 0.8660254037844387076, 1.000000000000000000, 0.8660254037844387076, 1.000000000000000000, 0.8660254037844387076, 1.000000000000000000),
 ( 1.000000000000000000, 0.8660254037844387076, 1.000000000000000000, 0.8660254037844387076, 1.000000000000000000, 0.8660254037844387076, 1.000000000000000000, 0.8660254037844387076, 1.000000000000000000, 0.8660254037844387076, 1.000000000000000000, 0.8660254037844387076, 1.000000000000000000, 0.8660254037844387076, 1.000000000000000000, 0.8660254037844387076, 1.000000000000000000, 0.8660254037844387076, 1.000000000000000000, 0.8660254037844387076, 1.000000000000000000, 0.8660254037844387076, 1.000000000000000000, 0.8660254037844387076, 1.000000000000000000, 0.8660254037844387076, 1.000000000000000000, 0.8660254037844387076, 1.000000000000000000, 0.8660254037844387076, 1.000000000000000000, 0.8660254037844387076, 1.000000000000000000, 0.8660254037844387076, 1.000000000000000000, 0.8660254037844387076, 1.000000000000000000, 0.8660254037844387076, 1.000000000000000000, 0.8660254037844387076, 1.000000000000000000, 0.8660254037844387076, 1.000000000000000000, 0.8660254037844387076, 1.000000000000000000, 0.8660254037844387076, 1.000000000000000000, 0.8660254037844387076, 1.000000000000000000, 0.8660254037844387076, 1.000000000000000000, 0.8660254037844387076, 1.000000000000000000, 0.8660254037844387076, 1.000000000000000000, 0.8660254037844387076, 1.000000000000000000, 0.8660254037844387076, 1.000000000000000000, 0.8660254037844387076, 1.000000000000000000, 0.8660254037844387076, 1.000000000000000000, 0.8660254037844387076, 1.000000000000000000, 0.8660254037844387076, 1.000000000000000000, 0.8660254037844387076, 1.000000000000000000, 0.8660254037844387076, 1.000000000000000000, 0.8660254037844387076, 1.000000000000000000, 0.8660254037844387076, 1.000000000000000000, 0.8660254037844387076, 1.000000000000000000, 0.8660254037844387076, 1.000000000000000000, 0.8660254037844387076, 1.000000000000000000, 0.8660254037844387076, 1.000000000000000000, 0.8660254037844387076, 1.000000000000000000, 0.8660254037844387076, 1.000000000000000000, 0.8660254037844387076, 1.000000000000000000, 0.8660254037844387076, 1.000000000000000000, 0.8660254037844387076, 1.000000000000000000, 0.8660254037844387076, 1.000000000000000000, 0.8660254037844387076, 1.000000000000000000, 0.8660254037844387076, 1.000000000000000000, 0.8660254037844387076, 1.000000000000000000, 0.8660254037844387076, 1.000000000000000000, 0.8660254037844387076, 1.000000000000000000, 0.8660254037844387076, 1.000000000000000000, 0.8660254037844387076, 1.000000000000000000, 0.8660254037844387076, 1.000000000000000000, 0.8660254037844387076, 1.000000000000000000, 0.8660254037844387076, 1.000000000000000000, 0.8660254037844387076, 1.000000000000000000, 0.8660254037844387076, 1.000000000000000000, 0.8660254037844387076, 1.000000000000000000, 0.8660254037844387076, 1.000000000000000000, 0.8660254037844387076, 1.000000000000000000, 0.8660254037844387076, 1.000000000000000000, 0.8660254037844387076, 1.000000000000000000, 0.8660254037844387076, 1.000000000000000000, 0.8660254037844387076, 1.000000000000000000, 0.8660254037844387076, 1.000000000000000000, 0.8660254037844387076, 1.000000000000000000, 0.8660254037844387076, 1.000000000000000000, 0.8660254037844387076, 1.000000000000000000, 0.8660254037844387076, 1.000000000000000000, 0.8660254037844387076, 1.000000000000000000, 0.8660254037844387076, 1.000000000000000000, 0.8660254037844387076, 1.000000000000000000, 0.8660254037844387076, 1.000000000000000000, 0.8660254037844387076, 1.000000000000000000, 0.8660254037844387076, 1.000000000000000000, 0.8660254037844387076, 1.000000000000000000, 0.8660254037844387076, 1.000000000000000000, 0.8660254037844387076, 1.000000000000000000, 0.8660254037844387076, 1.000000000000000000, 0.8660254037844387076, 1.000000000000000000, 0.8660254037844387076, 1.000000000000000000, 0.8660254037844387076, 1.000000000000000000, 0.8660254037844387076, 1.000000000000000000, 0.8660254037844387076, 1.000000000000000000, 0.8660254037844387076, 1.000000000000000000, 0.8660254037844387076, 1.000000000000000000, 0.8660254037844387076, 1.000000000000000000, 0.8660254037844387076, 1.000000000000000000, 0.8660254037844387076, 1.000000000000000000, 0.8660254037844387076, 1.000000000000000000, 0.8660254037844387076, 1.000000000000000000, 0.8660254037844387076, 1.000000000000000000, 0.8660254037844387076, 1.000000000000000000, 0.8660254037844387076, 1.000000000000000000, 0.8660254037844387076, 1.000000000000000000, 0.8660254037844387076, 1.000000000000000000, 0.8660254037844387076, 1.000000000000000000, 0.8660254037844387076, 1.000000000000000000, 0.8660254037844387076, 1.000000000000000000, 0.8660254037844387076, 1.000000000000000000, 0.8660254037844387076, 1.000000000000000000, 0.8660254037844387076, 1.000000000000000000, 0.8660254037844387076, 1.000000000000000000, 0.8660254037844387076, 1.000000000000000000, 0.8660254037844387076, 1.000000000000000000, 0.8660254037844387076, 1.000000000000000000, 0.8660254037844387076, 1.000000000000000000, 0.8660254037844387076, 1.000000000000000000, 0.8660254037844387076, 1.000000000000000000, 0.8660254037844387076, 1.000000000000000000, 0.8660254037844387076, 1.000000000000000000, 0.8660254037844387076, 1.000000000000000000, 0.8660254037844387076, 1.000000000000000000, 0.8660254037844387076, 1.000000000000000000, 0.8660254037844387076, 1.000000000000000000, 0.8660254037844387076, 1.000000000000000000, 0.8660254037844387076, 1.000000000000000000, 0.8660254037844387076, 1.000000000000000000) ) ) 
 REPRESENTATION_ITEM ( '' )  SURFACE ( )  );
#185191=CARTESIAN_POINT ( 'NONE',  ( 7.517069824134078537, 7.734612647770044092, 0.000000000000000000 ) ) ;
#185200=CARTESIAN_POINT ( 'NONE',  ( 6.021229618244865023, 10.03886863134542828, -0.7216878364870458196 ) ) ;
#185213=CARTESIAN_POINT ( 'NONE',  ( -5.261973015879593873, 8.192700047617899273, 1.082531754730549967 ) ) ;
#185216=CARTESIAN_POINT ( 'NONE',  ( 5.688527969385528849, 8.794310509995222347, -1.199719254218452047 ) ) ;
#185219=CARTESIAN_POINT ( 'NONE',  ( -6.933015448541747006, 9.181880338089085214, 1.599625672291269396 ) ) ;
#185221=CARTESIAN_POINT ( 'NONE',  ( -3.481411583659053566, 7.283673624236017830, 0.000000000000000000 ) ) ;
#185223=CARTESIAN_POINT ( 'NONE',  ( 3.940491328593588971, 7.322805182156911563, -0.8893161052136487887 ) ) ;
#185264=CARTESIAN_POINT ( 'NONE',  ( 5.424670859243587273, 5.501406555305196733, -0.7216878364870458196 ) ) ;
#185269=CARTESIAN_POINT ( 'NONE',  ( -5.173318132066234476, 8.193232366456022930, -1.199719254218453823 ) ) ;
#185273=CARTESIAN_POINT ( 'NONE',  ( -6.310394152517827315, 6.326824364217716656, 0.7998128361456281477 ) ) ;
#185274=CARTESIAN_POINT ( 'NONE',  ( -6.154475385960665790, 6.144919136567696505, 0.000000000000000000 ) ) ;
#185277=CARTESIAN_POINT ( 'NONE',  ( -5.546694241322218666, 8.524874810634301525, 1.082531754730550855 ) ) ;
#185283=CARTESIAN_POINT ( 'NONE',  ( -5.427006627220116286, 9.553534508390610469, -0.7998128361456362523 ) ) ;
#185289=CARTESIAN_POINT ( 'NONE',  ( 3.590748693434304251, 7.344754702231194976, 0.3435062996885069886 ) ) ;
#185291=CARTESIAN_POINT ( 'NONE',  ( -5.875479466675803231, 7.948088359245467416, -1.599625672291271394 ) ) ;
#185293=CARTESIAN_POINT ( 'NONE',  ( 4.873468316212648865, 8.167532512703042258, 0.9812947938723035612 ) ) ;
#185298=CARTESIAN_POINT ( 'NONE',  ( 6.047819040147648373, 9.213483425884394507, 1.199719254218452047 ) ) ;
#185312=CARTESIAN_POINT ( 'NONE',  ( -7.611976899429754084, 7.845337568948314022, 0.7998128361456341429 ) ) ;
#185326=CARTESIAN_POINT ( 'NONE',  ( 6.313256805818848960, 7.394496357324014113, 1.199719254218452047 ) ) ;
#185335=CARTESIAN_POINT ( 'NONE',  ( -4.207966135563093957, 7.175396087857926375, 1.072179110320391260 ) ) ;
#185340=CARTESIAN_POINT ( 'NONE',  ( 5.586791213849657822, 7.504901977030062454, -1.335864709735144817 ) ) ;
#185364=ORIENTED_EDGE ( 'NONE', *, *, #103174, .F. ) ;
#185368=CARTESIAN_POINT ( 'NONE',  ( -6.169688749744446810, 7.059909438329341036, 1.079748085779270950 ) ) ;
#185371=EDGE_CURVE ( 'NONE', #150164, #93524, #185660, .T. ) ;
#185372=VECTOR ( 'NONE', #37425, 1000.000000000000000 ) ;
#185383=EDGE_CURVE ( 'NONE', #130448, #53708, #136236, .T. ) ;
#185389=CARTESIAN_POINT ( 'NONE',  ( -6.303615075710993665, 6.318915441276411471, -0.7998128361456362523 ) ) ;
#185405=CARTESIAN_POINT ( 'NONE',  ( 4.543917759235442944, 5.330267469643351852, 1.199719254218452935 ) ) ;
#185407=CARTESIAN_POINT ( 'NONE',  ( 6.007671464186812749, 10.02305078494439883, 0.7216878364870317197 ) ) ;
#185417=CARTESIAN_POINT ( 'NONE',  ( 5.844973620822844218, 6.952128991449046502, 1.082531754730549967 ) ) ;
#185421=CARTESIAN_POINT ( 'NONE',  ( -7.110325215724114578, 7.260077271291732082, 0.000000000000000000 ) ) ;
#185423=CARTESIAN_POINT ( 'NONE',  ( 4.505052181490820651, 8.477920988373101707, -0.7998128361456381397 ) ) ;
#185432=CARTESIAN_POINT ( 'NONE',  ( -5.164730172163054966, 4.990216387137135889, -0.7998128361456362523 ) ) ;
#185433=CARTESIAN_POINT ( 'NONE',  ( 6.535912570239620578, 9.782925877658371405, 1.199719254218452047 ) ) ;
#185435=SPHERICAL_SURFACE ( 'NONE', #63518, 0.08000000000000000167 ) ;
#185440=CARTESIAN_POINT ( 'NONE',  ( 6.688968683495743583, 8.897159112202094988, -1.599625672291283607 ) ) ;
#185445=CARTESIAN_POINT ( 'NONE',  ( -5.094039349513959536, 7.939876775568885492, 1.214520887661042936 ) ) ;
#185456=CARTESIAN_POINT ( 'NONE',  ( -4.407809337774280856, 7.196175756495025055, 1.082531754730549967 ) ) ;
#185467=CARTESIAN_POINT ( 'NONE',  ( 5.560252395380222090, 5.659585014131299552, 0.7216878364870328300 ) ) ;
#185470=CARTESIAN_POINT ( 'NONE',  ( -4.911796789900812144, 8.952456364851418158, 0.7998128361456291469 ) ) ;
#185481=CARTESIAN_POINT ( 'NONE',  ( 3.250922972226694352, 7.014770244231638863, 0.7998128361456281477 ) ) ;
#185485=CARTESIAN_POINT ( 'NONE',  ( 5.224688093219824303, 7.188831756880171397, -1.599625672291283607 ) ) ;
#185508=CARTESIAN_POINT ( 'NONE',  ( 5.578253857379852576, 5.472660686556754861, -0.7998128361456481317 ) ) ;
#185509=CARTESIAN_POINT ( 'NONE',  ( -5.533136088152923904, 6.588318536667425285, 1.082531754730549078 ) ) ;
#185532=CARTESIAN_POINT ( 'NONE',  ( -7.130662446144611977, 7.283804040115648526, 0.000000000000000000 ) ) ;
#185534=CARTESIAN_POINT ( 'NONE',  ( 7.146556367734771875, 8.470642196179646533, 1.082531754730549967 ) ) ;
#185544=ORIENTED_EDGE ( 'NONE', *, *, #46958, .T. ) ;
#185548=CARTESIAN_POINT ( 'NONE',  ( -7.422162748838431412, 7.623887726591770608, -0.7998128361456362523 ) ) ;
#185560=CARTESIAN_POINT ( 'NONE',  ( -5.413448473606448985, 9.537716662508005427, 0.000000000000000000 ) ) ;
#185563=CARTESIAN_POINT ( 'NONE',  ( -5.144392941742557568, 4.966489618313220333, -0.7998128361456362523 ) ) ;
#185566=CARTESIAN_POINT ( 'NONE',  ( -6.238160075619175515, 10.29195416494877513, 0.000000000000000000 ) ) ;
#185567=CARTESIAN_POINT ( 'NONE',  ( 3.214691819771663628, 6.764574533126651801, -0.7216878364870338292 ) ) ;
#185568=CARTESIAN_POINT ( 'NONE',  ( -3.594320120954326292, 6.247105003538398371, 1.082531754730549967 ) ) ;
#185573=CARTESIAN_POINT ( 'NONE',  ( -4.664887371553763096, 7.600063145858131364, -1.199719254218453823 ) ) ;
#185588=CARTESIAN_POINT ( 'NONE',  ( 5.126881573038487794, 7.911131357477594328, 1.221340741751137493 ) ) ;
#185598=CARTESIAN_POINT ( 'NONE',  ( 5.742760583840166966, 8.857581893525663830, 1.199719254218452047 ) ) ;
#185608=CARTESIAN_POINT ( 'NONE',  ( 5.732961426666957294, 7.278201736375829789, 1.206439608388230500 ) ) ;
#185625=CARTESIAN_POINT ( 'NONE',  ( -5.712781623311813384, 7.758274208654143855, -1.599625672291271394 ) ) ;
#185638=CARTESIAN_POINT ( 'NONE',  ( 4.766573523656222555, 7.718696989977711809, 1.199719254218452047 ) ) ;
#185644=DIRECTION ( 'NONE',  ( 0.000000000000000000, 1.000000000000000000, 0.000000000000000000 ) ) ;
#185645=AXIS2_PLACEMENT_3D ( 'NONE', #34359, #18094, #85245 ) ;
#185650=CARTESIAN_POINT ( 'NONE',  ( 3.228249973385329596, 6.780392379009261283, -1.734723475976807094E-15 ) ) ;
#185651=CARTESIAN_POINT ( 'NONE',  ( 5.606297198005668392, 5.722949621141593113, -0.4987895298722895276 ) ) ;
#185660=LINE ( 'NONE', #37290, #32571 ) ;
#185666=CARTESIAN_POINT ( 'NONE',  ( -6.075462232699549325, 9.141770800574526845, 1.082531754730549967 ) ) ;
#185667=CARTESIAN_POINT ( 'NONE',  ( 4.733205024946604667, 8.536173272497439513, 0.000000000000000000 ) ) ;
#185677=CARTESIAN_POINT ( 'NONE',  ( -4.339491684825780737, 7.220434844675483355, -1.199719254218455378 ) ) ;
#185678=CARTESIAN_POINT ( 'NONE',  ( -2.823841133396259639, 6.516508098929413961, -0.7998128361456481317 ) ) ;
#185680=CARTESIAN_POINT ( 'NONE',  ( 5.343321937117211817, 9.247976336696488886, 0.000000000000000000 ) ) ;
#185691=CARTESIAN_POINT ( 'NONE',  ( -4.768476522361002168, 8.183970109320437558, 0.7579922544750415936 ) ) ;
#185694=CARTESIAN_POINT ( 'NONE',  ( 5.072158865288245444, 5.090142562357324429, 0.7216878364870338292 ) ) ;
#185698=CARTESIAN_POINT ( 'NONE',  ( -5.818384198920079520, 6.817144982608731141, 1.199719254218452935 ) ) ;
#185709=CARTESIAN_POINT ( 'NONE',  ( 5.041653019435334393, 6.975290837464928728, -1.599625672291269396 ) ) ;
#185745=CARTESIAN_POINT ( 'NONE',  ( 4.733205024946604667, 8.536173272497439513, 0.000000000000000000 ) ) ;
#185751=CARTESIAN_POINT ( 'NONE',  ( 5.682275777458841048, 8.683053269460405232, 1.082531754730547524 ) ) ;
#185753=CARTESIAN_POINT ( 'NONE',  ( -3.903950209304078989, 8.999999999999998224, 0.7749999999999996891 ) ) ;
#185766=CARTESIAN_POINT ( 'NONE',  ( -6.474900878978163021, 9.711745571186627402, -1.199719254218452047 ) ) ;
#185783=CARTESIAN_POINT ( 'NONE',  ( -5.167592825464113915, 6.057888380243431570, 1.199719254218452935 ) ) ;
#185788=CARTESIAN_POINT ( 'NONE',  ( -7.431277594066152403, 8.802816960232885179, -1.082531754730549967 ) ) ;
#185792=CARTESIAN_POINT ( 'NONE',  ( -6.454563648557663846, 9.688018802362710957, -1.199719254218452047 ) ) ;
#185806=LINE ( 'NONE', #37439, #186291 ) ;
#185813=CARTESIAN_POINT ( 'NONE',  ( -4.828112100242294424, 5.765790550771681566, -1.082531754730549967 ) ) ;
#185815=CARTESIAN_POINT ( 'NONE',  ( -3.485854892044994102, 7.080931450778859215, -0.7216878364870458196 ) ) ;
#185817=CARTESIAN_POINT ( 'NONE',  ( 6.086684617892325733, 6.065829907154645539, -0.7998128361456481317 ) ) ;
#185818=CARTESIAN_POINT ( 'NONE',  ( -4.685224601974262271, 7.623789914682047808, -1.199719254218453823 ) ) ;
#185819=CARTESIAN_POINT ( 'NONE',  ( -6.794571259104023930, 7.956029886156682274, 1.199719254218452047 ) ) ;
#185873=CARTESIAN_POINT ( 'NONE',  ( 4.278479993564246797, 7.149254538203735798, 1.199719254218452047 ) ) ;
#185875=CARTESIAN_POINT ( 'NONE',  ( -3.912682303000325046, 8.998411203033816363, -0.7749999999999979128 ) ) ;
#185888=CARTESIAN_POINT ( 'NONE',  ( 5.717785742877098620, 7.006476535625818514, 2.500000000000000444 ) ) ;
#185891=CARTESIAN_POINT ( 'NONE',  ( 6.229045230835819069, 6.231917288922055320, -0.7998128361456481317 ) ) ;
#185896=CARTESIAN_POINT ( 'NONE',  ( -5.427006627220116286, 9.553534508390610469, -0.7998128361456362523 ) ) ;
#185901=ORIENTED_EDGE ( 'NONE', *, *, #152381, .T. ) ;
#185908=CARTESIAN_POINT ( 'NONE',  ( 4.489158259456265121, 7.291082831790689056, -1.082531754730548412 ) ) ;
#185912=CARTESIAN_POINT ( 'NONE',  ( 6.563555762791525972, 6.830105609444471426, -0.7216878364870458196 ) ) ;
#185914=CARTESIAN_POINT ( 'NONE',  ( -3.689227196694346400, 6.357829925235092716, -1.082531754730546636 ) ) ;
#185915=CARTESIAN_POINT ( 'NONE',  ( -6.608673532018475960, 6.674816973635147477, -0.7998128361456362523 ) ) ;
#185925=CARTESIAN_POINT ( 'NONE',  ( 3.230585741806197841, 6.991043475407723307, 0.7998128361456271485 ) ) ;
#185926=CARTESIAN_POINT ( 'NONE',  ( 4.688087255275310561, 8.691461907788344377, -0.7998128361456381397 ) ) ;
#185948=CARTESIAN_POINT ( 'NONE',  ( 5.862225131719664972, 7.287605523280396902, -1.268052015211480033 ) ) ;
#185950=ORIENTED_EDGE ( 'NONE', *, *, #169514, .T. ) ;
#185953=CARTESIAN_POINT ( 'NONE',  ( 5.606900530694575835, 7.430539361494464146, 1.295638170384592947 ) ) ;
#185959=CARTESIAN_POINT ( 'NONE',  ( 5.083381250481017410, 4.895309311841474553, 0.7998128361456352531 ) ) ;
#185963=CARTESIAN_POINT ( 'NONE',  ( 7.178115983792402233, 7.339166500704784823, 0.7998128361456281477 ) ) ;
#185964=CARTESIAN_POINT ( 'NONE',  ( -9.336326716892640931, 8.920000000000001705, -2.500000000000000444 ) ) ;
#185968=CARTESIAN_POINT ( 'NONE',  ( 3.445180431648313224, 7.033477913649446300, 0.7216878364870257245 ) ) ;
#185971=CARTESIAN_POINT ( 'NONE',  ( 3.984117037569365305, 5.741498858621315371, 1.599625672291261402 ) ) ;
#185982=CARTESIAN_POINT ( 'NONE',  ( 6.453003701063230402, 6.772902045581084884, 0.3391303328579304277 ) ) ;
#185983=CARTESIAN_POINT ( 'NONE',  ( -5.171509248969888617, 4.998125310078441075, 0.7998128361456281477 ) ) ;
#186010=CARTESIAN_POINT ( 'NONE',  ( -5.983791420057156252, 7.107340751733106643, 1.079986564815892613 ) ) ;
#186016=CARTESIAN_POINT ( 'NONE',  ( 6.313256805818848960, 7.394496357324014113, 1.199719254218452047 ) ) ;
#186018=CARTESIAN_POINT ( 'NONE',  ( 7.862802741282558294, 8.137967717776607657, 0.000000000000000000 ) ) ;
#186024=EDGE_CURVE ( 'NONE', #41882, #85209, #209123, .T. ) ;
#186034=CARTESIAN_POINT ( 'NONE',  ( -5.255720823952942489, 6.160704378480398979, -1.199719254218453823 ) ) ;
#186036=CARTESIAN_POINT ( 'NONE',  ( 6.251718229232841928, 8.387033582228703210, -1.443375672974078761 ) ) ;
#186039=B_SPLINE_CURVE_WITH_KNOTS ( 'NONE', 3,
 ( #109451, #124649, #92085, #127861, #192736, #110512, #160258, #77937, #42264, #30265, #29198, #59549, #210053, #58493 ),
 .UNSPECIFIED., .F., .F.,
 ( 4, 2, 2, 2, 2, 2, 4 ),
 ( 0.001478211208292421830, 0.001788443044005901591, 0.002098674879719381568, 0.002408906715432861112, 0.002719138551146341089, 0.003339602222573304080, 0.003960065894000266637 ),
 .UNSPECIFIED. ) ;
#186047=CARTESIAN_POINT ( 'NONE',  ( -3.688700311369816909, 6.461178242310183784, -1.199719254218450271 ) ) ;
#186050=CARTESIAN_POINT ( 'NONE',  ( -3.472296738875691346, 6.104744391113324120, 1.082531754730549967 ) ) ;
#186052=AXIS2_PLACEMENT_3D ( 'NONE', #156175, #26148, #77027 ) ;
#186054=CARTESIAN_POINT ( 'NONE',  ( -4.930325137224961907, 5.781076077297750970, -1.199719254218453823 ) ) ;
#186055=ORIENTED_EDGE ( 'NONE', *, *, #112616, .F. ) ;
#186056=CARTESIAN_POINT ( 'NONE',  ( -4.800995793014949165, 8.615262501910491366, 0.7216878364870267237 ) ) ;
#186081=CARTESIAN_POINT ( 'NONE',  ( -4.132202957115018727, 8.042930226601317401, 0.000000000000000000 ) ) ;
#186084=CARTESIAN_POINT ( 'NONE',  ( -2.844178363816758814, 6.540234867753325076, -0.7998128361456481317 ) ) ;
#186093=CARTESIAN_POINT ( 'NONE',  ( -5.978723031652583231, 7.198045494411626777, -1.221819409761595088 ) ) ;
#186124=CARTESIAN_POINT ( 'NONE',  ( 3.736153849017632922, 6.516540702899320081, -1.199719254218453823 ) ) ;
#186132=CARTESIAN_POINT ( 'NONE',  ( 5.417364897112183719, 8.477953592343014932, 1.199719254218451159 ) ) ;
#186134=CARTESIAN_POINT ( 'NONE',  ( 6.204791576909545192, 7.267953590263130259, -1.199719254218452047 ) ) ;
#186137=CARTESIAN_POINT ( 'NONE',  ( -3.591468823281545930, 3.560404793497018439, -2.500000000000000444 ) ) ;
#186147=CARTESIAN_POINT ( 'NONE',  ( 6.373787108001086388, 6.824503602047865769, -0.5760177672454840359 ) ) ;
#186149=CARTESIAN_POINT ( 'NONE',  ( -5.438229012412890917, 8.398332043573416783, -1.082531754730549967 ) ) ;
#186150=CARTESIAN_POINT ( 'NONE',  ( 6.102578539926878598, 7.252668063737060855, -1.082531754730548412 ) ) ;
#186168=CARTESIAN_POINT ( 'NONE',  ( -4.787437638956935082, 6.678706226906775179, -1.443375672974066548 ) ) ;
#186173=CARTESIAN_POINT ( 'NONE',  ( 6.530187263637528439, 7.647581891445782709, -1.199719254218452047 ) ) ;
#186201=CARTESIAN_POINT ( 'NONE',  ( 7.178115983792402233, 7.339166500704784823, 0.7998128361456281477 ) ) ;
#186214=CARTESIAN_POINT ( 'NONE',  ( -3.007132747898833447, 6.372410370188839934, -0.7689175719093130912 ) ) ;
#186231=VERTEX_POINT ( 'NONE', #169176 ) ;
#186232=CARTESIAN_POINT ( 'NONE',  ( 5.126391479742934187, 6.113783160189109722, -1.082531754730548412 ) ) ;
#186239=CARTESIAN_POINT ( 'NONE',  ( 6.282224075085741433, 8.422623735723785643, 1.599625672291268286 ) ) ;
#186243=CARTESIAN_POINT ( 'NONE',  ( -3.662110889467009578, 7.286563447771212232, 0.7216878364870338292 ) ) ;
#186251=CARTESIAN_POINT ( 'NONE',  ( -4.462041952228919861, 8.219816354326827224, -0.7216878364870170648 ) ) ;
#186263=CARTESIAN_POINT ( 'NONE',  ( 7.991605200612358573, 8.288237253661408843, 0.7998128361456281477 ) ) ;
#186272=CARTESIAN_POINT ( 'NONE',  ( 5.885648082108177803, 9.880690172519326353, 0.7216878364870317197 ) ) ;
#186283=DIRECTION ( 'NONE',  ( 0.000000000000000000, 0.000000000000000000, -1.000000000000000000 ) ) ;
#186285=CARTESIAN_POINT ( 'NONE',  ( -6.292392690518223475, 6.513748691792265788, -0.7216878364870338292 ) ) ;
#186287=CARTESIAN_POINT ( 'NONE',  ( 7.361151057576892143, 7.552707420120024828, 0.7998128361456291469 ) ) ;
#186291=VECTOR ( 'NONE', #4901, 1000.000000000000000 ) ;
#186293=CARTESIAN_POINT ( 'NONE',  ( -5.815521545619021460, 5.749472989502435460, -0.7998128361456362523 ) ) ;
#186339=CARTESIAN_POINT ( 'NONE',  ( -6.981522756394290319, 7.109807735406931783, 0.7998128361456341429 ) ) ;
#186343=CARTESIAN_POINT ( 'NONE',  ( -6.473091995881817162, 6.516638514809040217, 0.7998128361456281477 ) ) ;
#186344=CARTESIAN_POINT ( 'NONE',  ( -3.820365424000704557, 7.679119771301276209, -0.7998128361456481317 ) ) ;
#186348=CARTESIAN_POINT ( 'NONE',  ( -6.089020385868862739, 8.197219431637373432, -1.443375672974066548 ) ) ;
#186354=CARTESIAN_POINT ( 'NONE',  ( -6.994027139803241866, 9.253060644560830994, -1.599625672291271394 ) ) ;
#186359=EDGE_LOOP ( 'NONE', ( #150610, #45712, #25543, #193926, #51010, #128051 ) ) ;
#186362=CARTESIAN_POINT ( 'NONE',  ( -5.447343857640614573, 9.577261277214532242, -0.7998128361456362523 ) ) ;
#186364=CARTESIAN_POINT ( 'NONE',  ( 4.725438941449205288, 8.332574750205820280, 0.7120043264817934592 ) ) ;
#186369=CARTESIAN_POINT ( 'NONE',  ( 2.925527285498711549, 6.635141943048991742, 0.7998128361456281477 ) ) ;
#186380=CARTESIAN_POINT ( 'NONE',  ( -6.050681693448748177, 10.28115541899069463, 0.7998128361456291469 ) ) ;
#186383=CARTESIAN_POINT ( 'NONE',  ( 3.914023514147235261, 8.998170835453741745, -0.7749999999999996891 ) ) ;
#186392=CARTESIAN_POINT ( 'NONE',  ( 7.343676480457483002, 8.596652644402405841, -1.199719254218452047 ) ) ;
#186407=CARTESIAN_POINT ( 'NONE',  ( 6.184762415132515123, 7.051423785172313607, -1.050594063207562545 ) ) ;
#186435=CARTESIAN_POINT ( 'NONE',  ( -6.081163491871431681, 7.123212080692602477, 1.153528356629534013 ) ) ;
#186439=ORIENTED_EDGE ( 'NONE', *, *, #44801, .T. ) ;
#186455=CARTESIAN_POINT ( 'NONE',  ( -3.630551273409382329, 7.457669928944732796, 0.7998128361456352531 ) ) ;
#186464=( BOUNDED_CURVE ( )  B_SPLINE_CURVE ( 2, ( #152644, #21541, #140704 ),
 .UNSPECIFIED., .F., .T. ) 
 B_SPLINE_CURVE_WITH_KNOTS ( ( 3, 3 ),
 ( 0.2461080272610979280, 0.2500000000000002776 ),
 .UNSPECIFIED. ) 
 CURVE ( )  GEOMETRIC_REPRESENTATION_ITEM ( )  RATIONAL_B_SPLINE_CURVE ( ( 0.9333038493907171995, 0.9374289428588350459, 1.000000000000004441 ) ) 
 REPRESENTATION_ITEM ( '' )  );
#186473=CARTESIAN_POINT ( 'NONE',  ( 4.435452530326143616, 5.203724702582467998, -1.199719254218452047 ) ) ;
#186494=CARTESIAN_POINT ( 'NONE',  ( 4.694866332082116678, 8.699370830729650450, 0.7998128361456341429 ) ) ;
#186505=CARTESIAN_POINT ( 'NONE',  ( -5.113360211009450040, 5.994616996712990975, -1.199719254218453823 ) ) ;
#186506=CARTESIAN_POINT ( 'NONE',  ( 2.925527285498711549, 6.635141943048991742, 0.7998128361456281477 ) ) ;
#186512=CARTESIAN_POINT ( 'NONE',  ( 6.875920180786008196, 8.050936961452347163, -1.199719254218452047 ) ) ;
#186519=MECHANICAL_DESIGN_GEOMETRIC_PRESENTATION_REPRESENTATION('',(#27424),#100098);
#186520=CARTESIAN_POINT ( 'NONE',  ( -4.592595068035599581, 8.488991103336598343, 0.1827531742817755656 ) ) ;
#186529=CARTESIAN_POINT ( 'NONE',  ( -5.112833325684920993, 6.097965313788082931, -1.082531754730549967 ) ) ;
#186539=CARTESIAN_POINT ( 'NONE',  ( 4.936577329151614180, 4.931964103531220722, -0.7216878364870458196 ) ) ;
#186543=CARTESIAN_POINT ( 'NONE',  ( -6.473091995881817162, 6.516638514809040217, 0.7998128361456281477 ) ) ;
#186557=CARTESIAN_POINT ( 'NONE',  ( 4.923546060418115822, 5.773167154356443120, -1.199719254218452047 ) ) ;
#186582=CARTESIAN_POINT ( 'NONE',  ( 0.4138360523464839069, 3.000267424193761467, 2.020124146241416785 ) ) ;
#186584=CARTESIAN_POINT ( 'NONE',  ( -4.909461021924285795, 6.821066840368686712, 1.443375672974058777 ) ) ;
#186608=CARTESIAN_POINT ( 'NONE',  ( -5.986807348886189040, 9.142303119412650503, -1.199719254218452047 ) ) ;
#186610=CARTESIAN_POINT ( 'NONE',  ( 6.333067150914805765, 9.442309871825708356, 1.082531754730549967 ) ) ;
#186623=CARTESIAN_POINT ( 'NONE',  ( -4.842197138736131556, 5.678260079060780008, 1.199719254218452935 ) ) ;
#186629=CARTESIAN_POINT ( 'NONE',  ( 3.718679271898170491, 7.560485927181699317, 0.7998128361456271485 ) ) ;
#186634=CARTESIAN_POINT ( 'NONE',  ( -4.776215253764153346, 8.794277906025310898, -0.7998128361456362523 ) ) ;
#186638=CARTESIAN_POINT ( 'NONE',  ( -4.496464221587651799, 5.274905009054215554, 1.199719254218452935 ) ) ;
#186642=CARTESIAN_POINT ( 'NONE',  ( 3.838366886000300404, 6.531826229425389485, -1.082531754730548412 ) ) ;
#186643=CARTESIAN_POINT ( 'NONE',  ( -5.600926855776901192, 5.707038551260711579, -0.7216878364870338292 ) ) ;
#186648=CARTESIAN_POINT ( 'NONE',  ( -5.181866634007240791, 6.340624232048664766, 1.284222742053082733 ) ) ;
#186651=CARTESIAN_POINT ( 'NONE',  ( 4.415115299905642665, 5.179997933758551554, -1.199719254218450271 ) ) ;
#186661=CARTESIAN_POINT ( 'NONE',  ( 5.720439131930858956, 7.397432110343761025, 1.315134405782365956 ) ) ;
#186670=CARTESIAN_POINT ( 'NONE',  ( 6.333594036239346359, 7.418223126147930557, 1.199719254218453823 ) ) ;
#186680=CARTESIAN_POINT ( 'NONE',  ( 5.542547785767838242, 7.428594929708664196, 1.247761615041423244 ) ) ;
#186697=CARTESIAN_POINT ( 'NONE',  ( -4.606738333593328072, 8.596554832492683929, 0.7998128361456281477 ) ) ;
#186702=LINE ( 'NONE', #4723, #32348 ) ;
#186710=CARTESIAN_POINT ( 'NONE',  ( 5.387385936583818591, 7.378645907471495846, -1.599625672291283607 ) ) ;
#186719=CARTESIAN_POINT ( 'NONE',  ( -5.926322542504860458, 9.928143709648733051, -0.7216878364870338292 ) ) ;
#186724=CARTESIAN_POINT ( 'NONE',  ( 3.377389663135653031, 6.954388683717978026, -0.7216878364870338292 ) ) ;
#186741=CARTESIAN_POINT ( 'NONE',  ( -4.981695098378565945, 4.776675467721892332, -0.7998128361456362523 ) ) ;
#186742=CARTESIAN_POINT ( 'NONE',  ( 6.536439455564168277, 6.798469917679251573, 0.7216878364870328300 ) ) ;
#186745=EDGE_CURVE ( 'NONE', #129277, #92086, #195293, .T. ) ;
#186753=CARTESIAN_POINT ( 'NONE',  ( -6.473091995881817162, 6.516638514809040217, 0.7998128361456281477 ) ) ;
#186754=CARTESIAN_POINT ( 'NONE',  ( -7.919371124158132602, 8.411890197705517380, -0.7216878364870338292 ) ) ;
#186756=CARTESIAN_POINT ( 'NONE',  ( 4.543390873910894356, 8.314723429622471684, 0.7216878364870317197 ) ) ;
#186761=CYLINDRICAL_SURFACE ( 'NONE', #210658, 1.250000000000000000 ) ;
#186762=CARTESIAN_POINT ( 'NONE',  ( -5.337312369484060071, 7.713579007861619985, 1.331290254527866201 ) ) ;
#186766=CARTESIAN_POINT ( 'NONE',  ( -4.764376198328064582, 8.188698463893414825, 0.7498042881181687935 ) ) ;
#186770=CARTESIAN_POINT ( 'NONE',  ( 3.431622278034673901, 7.017660067766835930, -1.734723475976807094E-15 ) ) ;
#186772=VECTOR ( 'NONE', #179084, 1000.000000000000000 ) ;
#186775=CARTESIAN_POINT ( 'NONE',  ( -5.173318132066234476, 8.193232366456022930, -1.199719254218453823 ) ) ;
#186780=B_SPLINE_CURVE_WITH_KNOTS ( 'NONE', 3,
 ( #119329, #136597, #120408, #38020, #186383, #149637, #204750 ),
 .UNSPECIFIED., .F., .F.,
 ( 4, 3, 4 ),
 ( 0.000000000000000000, 2.757963454290271384E-05, 5.739065715766676189E-05 ),
 .UNSPECIFIED. ) ;
#186787=CARTESIAN_POINT ( 'NONE',  ( 4.583538449871731757, 7.505156070562471804, 1.199719254218451159 ) ) ;
#186801=CARTESIAN_POINT ( 'NONE',  ( -5.777182852754558340, 5.912670547734647286, 0.000000000000000000 ) ) ;
#186803=CARTESIAN_POINT ( 'NONE',  ( 2.972313222866368676, 6.545497292499366182, 0.5012468031770876964 ) ) ;
#186823=CARTESIAN_POINT ( 'NONE',  ( 4.746763178560241769, 8.551991118380046331, 0.7216878364870328300 ) ) ;
#186829=CARTESIAN_POINT ( 'NONE',  ( 6.821160681006793070, 7.130644680695653825, 0.7216878364870328300 ) ) ;
#186843=CARTESIAN_POINT ( 'NONE',  ( -5.935437387732586778, 10.14670372898850381, -0.7998128361456362523 ) ) ;
#186854=FACE_OUTER_BOUND ( 'NONE', #13225, .T. ) ;
#186856=CARTESIAN_POINT ( 'NONE',  ( 4.787437638956922648, 6.678706226906775179, -1.443375672974068769 ) ) ;
#186862=CARTESIAN_POINT ( 'NONE',  ( -4.462568837553487100, 5.235360394347691404, -1.199719254218453823 ) ) ;
#186867=CARTESIAN_POINT ( 'NONE',  ( -5.966997003790221576, 9.015228033513643879, -1.082531754730549967 ) ) ;
#186869=CARTESIAN_POINT ( 'NONE',  ( -5.725286006720766707, 9.901527117808042178, 0.7998128361456291469 ) ) ;
#186882=CARTESIAN_POINT ( 'NONE',  ( -4.604929450496978660, 5.401447776115099408, -1.199719254218453823 ) ) ;
#186888=CARTESIAN_POINT ( 'NONE',  ( -4.746763178560296836, 6.631252689777363152, 1.443375672974058777 ) ) ;
#186890=CARTESIAN_POINT ( 'NONE',  ( -5.004368096775595021, 5.971422546727199077, 1.082531754730549078 ) ) ;
#186892=CARTESIAN_POINT ( 'NONE',  ( 4.199993725183334803, 8.122019456014369254, -0.7998128361456362523 ) ) ;
#186893=CARTESIAN_POINT ( 'NONE',  ( -6.466312919074983512, 6.508729591867735031, -0.7998128361456362523 ) ) ;
#186894=CARTESIAN_POINT ( 'NONE',  ( -5.433785704026946384, 9.561443431331920095, 0.000000000000000000 ) ) ;
#186897=DIRECTION ( 'NONE',  ( 0.000000000000000000, -1.000000000000000000, 0.000000000000000000 ) ) ;
#186901=ORIENTED_EDGE ( 'NONE', *, *, #149694, .T. ) ;
#186943=CARTESIAN_POINT ( 'NONE',  ( 2.979851157752180235, 6.482852879502049248, -0.5607284034093787950 ) ) ;
#186951=CARTESIAN_POINT ( 'NONE',  ( 6.059568310664962709, 6.034194215389424798, 0.7998128361456352531 ) ) ;
#186952=CARTESIAN_POINT ( 'NONE',  ( 5.747733515963313167, 7.238988828695343436, -1.232940794674276974 ) ) ;
#186953=CARTESIAN_POINT ( 'NONE',  ( 3.894033820048787398, 8.999999999999998224, 0.7749999999999996891 ) ) ;
#186967=CARTESIAN_POINT ( 'NONE',  ( 3.932747076415766596, 6.745899468197171345, 1.199719254218451159 ) ) ;
#186973=CARTESIAN_POINT ( 'NONE',  ( -7.611976899429754084, 7.845337568948314022, 0.7998128361456341429 ) ) ;
#186978=CARTESIAN_POINT ( 'NONE',  ( 6.059568310664962709, 6.034194215389424798, 0.7998128361456352531 ) ) ;
#186987=EDGE_CURVE ( 'NONE', #142253, #24930, #16853, .T. ) ;
#186991=CARTESIAN_POINT ( 'NONE',  ( 6.861835142292135536, 9.098836647464588978, 1.443375672974065660 ) ) ;
#186993=CARTESIAN_POINT ( 'NONE',  ( -5.167065940583949413, 5.200867483535597913, 0.000000000000000000 ) ) ;
#186994=CARTESIAN_POINT ( 'NONE',  ( -4.599959256786493533, 8.588645909551377855, 0.000000000000000000 ) ) ;
#187005=CARTESIAN_POINT ( 'NONE',  ( 3.878514461961128479, 6.682628084666728085, -1.199719254218448494 ) ) ;
#187006=CARTESIAN_POINT ( 'NONE',  ( 4.766573523656222555, 7.718696989977711809, 1.199719254218452047 ) ) ;
#187023=CARTESIAN_POINT ( 'NONE',  ( 5.269423316188119877, 7.778230059001682406, -1.291559732514224068 ) ) ;
#187029=CARTESIAN_POINT ( 'NONE',  ( 5.722950238744209273, 6.809768379023969587, 1.082531754730549967 ) ) ;
#187032=CARTESIAN_POINT ( 'NONE',  ( 3.464990776744291345, 6.200183785247111778, 1.199719254218452047 ) ) ;
#187037=CARTESIAN_POINT ( 'NONE',  ( 5.508355548902068577, 9.648441583686274470, 0.7998128361456331437 ) ) ;
#187042=CARTESIAN_POINT ( 'NONE',  ( 7.038091139269835317, 7.383730215335837954, 0.000000000000000000 ) ) ;
#187044=CARTESIAN_POINT ( 'NONE',  ( -4.471156797456668386, 8.438376373666578445, -0.7998128361456362523 ) ) ;
#187046=CARTESIAN_POINT ( 'NONE',  ( 7.187230829020129441, 8.518095734345896730, 1.082531754730549967 ) ) ;
#187057=CARTESIAN_POINT ( 'NONE',  ( 6.476386945563378461, 6.757828299745357370, 0.2189195654383000456 ) ) ;
#187058=CARTESIAN_POINT ( 'NONE',  ( -6.116136693540540570, 10.14959355252370266, 0.000000000000000000 ) ) ;
#187091=CARTESIAN_POINT ( 'NONE',  ( 5.936491157937257235, 8.019268665717216749, 1.599625672291268286 ) ) ;
#187093=CARTESIAN_POINT ( 'NONE',  ( 6.176621499477501054, 9.363752961769195693, -1.199719254218452047 ) ) ;
#187106=CARTESIAN_POINT ( 'NONE',  ( -5.822300622425855110, 5.757381912443740646, 0.7998128361456281477 ) ) ;
#187108=CARTESIAN_POINT ( 'NONE',  ( 6.495764994278809823, 6.751016379513001375, 0.7216878364870328300 ) ) ;
#187119=CARTESIAN_POINT ( 'NONE',  ( -5.957882158562513908, 5.915560371269843465, -0.7998128361456362523 ) ) ;
#187121=( BOUNDED_SURFACE ( )  B_SPLINE_SURFACE ( 1, 2, ( 
 ( #199212, #214372, #130066, #30360, #162498, #196059, #83340, #114854, #64961, #81228, #211215, #37535, #47691, #198158, #80157, #115917, #17265, #146263, #113803, #212275, #15142, #97500, #31424, #164612, #66002, #147310, #79091, #112737, #16197, #163557, #213336, #103613, #13014, #145209, #131113, #67072, #181904, #197100, #33538, #48741, #133208, #49791, #62841, #129002, #180854, #32476, #98549, #194979, #82278, #132152, #99610, #165676, #149425, #1008, #46615, #124221, #173975, #123165, #73221, #169668, #23401, #39673, #170737, #104688, #206432, #71074, #91657, #125279, #22323, #137192, #9307, #7150, #121011, #21254, #189126, #190183, #191241, #59122, #154500, #207500, #25549, #141494, #90582, #186978, #40761, #6078, #88436, #42904, #156642, #87360, #204271, #41838, #55925, #8234, #72149, #157710, #140414, #153429, #155568, #74317, #138258, #122082, #38610, #188043, #4998, #105784, #171809, #107949, #203215, #89514, #139328, #205358, #54860, #56992, #106867, #172894, #24469, #58056, #75380, #14622, #159825, #212826, #209618, #211759, #143623, #80717, #26619, #110080, #195533, #146808, #92720, #177148, #196595, #163042, #64462, #158766, #10361, #144689, #160900, #96991, #46100, #95924, #47172, #45034, #145759, #30916, #76438, #94849, #63397, #11428, #176092, #60186, #61260, #142546, #109013, #27690, #130607, #29840, #28765, #175032, #77504, #93789, #127418, #193390, #111148, #208552, #12496, #126345, #129551, #192305, #178225, #210700, #78569, #43964, #62330, #112216, #128489, #194455, #161978, #13568, #79640, #113286, #179292, #48236, #152108, #3678, #2620, #184584, #35134, #84964, #69757, #82830, #197645, #102277, #17807, #101207, #167293, #16745, #114350, #33024, #51412, #83890, #18880, #199767, #148906, #149981, #135861, #180347, #480, #81774, #31968, #168354, #68691, #117532, #134813, #98051, #198696, #200818, #66546, #49290, #132689, #166215, #50340, #164104, #15687, #213873, #116460, #151053, #147854, #133758, #183526, #65495, #131642, #115407, #182453, #1552, #181400, #99101, #19947, #165154, #67613 ),
 ( #34081, #100150, #52469, #86033, #118595, #36202, #122906, #153167, #155307, #57804, #172635, #75125, #187789, #188864, #38350, #104428, #4742, #170475, #185650, #54601, #120749, #7966, #201883, #55663, #121820, #22061, #157456, #88171, #25294, #186724, #9050, #24210, #91395, #107690, #154243, #53532, #5815, #90312, #71890, #173718, #119664, #202960, #74057, #37282, #137999, #70818, #136933, #204017, #123962, #89256, #39418, #105512, #103353, #169417, #171544, #156384, #23139, #140149, #206173, #6889, #72967, #139072, #205097, #56738, #40502, #106607, #189931, #41576, #21001, #87098, #78313, #27431, #192048, #14367, #96741, #162789, #59932, #195281, #95670, #143362, #29582, #11169, #46913, #111965, #125026, #141234, #43711, #93529, #44781, #108757, #159571, #61004, #28506, #13315, #76183, #77245, #144437, #161723, #145507, #94596, #110887, #207243, #209359, #127161, #142291, #208302, #177968, #42647, #63142, #58869, #126087, #174781, #113031, #193132, #92472, #190983, #160639, #79388, #26356, #30655, #109829, #179037, #211505, #158510, #62080, #10110, #12239, #175839, #176893, #210439, #128237, #194200, #45846, #129304, #181151, #1307, #65247, #118352, #213620, #102041, #117282, #184340, #200577, #131397, #35963, #32773, #183280, #115156, #52224, #212576, #81524, #167047, #168110, #197394, #31720, #163855, #49036, #150806, #182205, #132452, #148665, #64215, #80458, #98852, #51160, #97795, #34884, #84718, #147602, #164903, #16496, #82577, #231, #15435, #17556, #67367, #66303, #146556, #180096, #83642, #198450, #50096, #130355, #196347, #47989, #116217, #134576, #100957, #33831, #18639, #99910, #114105, #2370, #165971, #149729, #133511, #199515, #68447, #201639, #38111, #153995, #121574, #106358, #169167, #120504, #171300, #188615, #23970, #187545, #137757, #19709, #87921, #104183, #20762, #86856, #56494, #135619, #156135, #189678, #152921, #53287, #73801, #71644, #185407, #85788, #39176, #40247, #41328, #123717, #4500, #57559, #90072, #205926, #155060, #37025, #105259, #70568, #136687, #107438, #6647, #151868 ) ),
 .UNSPECIFIED., .F., .F., .T. ) 
 B_SPLINE_SURFACE_WITH_KNOTS ( ( 2, 2 ),
 ( 3, 2, 2, 2, 2, 2, 2, 2, 2, 2, 2, 2, 2, 2, 2, 2, 2, 2, 2, 2, 2, 2, 2, 2, 2, 2, 2, 2, 2, 2, 2, 2, 2, 2, 2, 2, 2, 2, 2, 2, 2, 2, 2, 2, 2, 2, 2, 2, 2, 2, 2, 2, 2, 2, 2, 2, 2, 2, 2, 2, 2, 2, 2, 2, 2, 2, 2, 2, 2, 2, 2, 2, 2, 2, 2, 2, 2, 2, 2, 2, 2, 2, 2, 2, 2, 2, 2, 2, 2, 2, 2, 2, 2, 2, 2, 2, 2, 2, 2, 2, 2, 2, 2, 2, 2, 2, 2, 2, 2, 2, 2, 2, 2, 2, 2, 2, 2, 2, 2, 2, 3 ),
 ( 0.000000000000000000, 1.000000000000000000 ),
 ( 0.000000000000000000, 0.008333333333333333218, 0.01666666666666666644, 0.02500000000000000139, 0.03333333333333333287, 0.04166666666666666435, 0.05000000000000000278, 0.05833333333333333426, 0.06666666666666666574, 0.07499999999999999722, 0.08333333333333332871, 0.09166666666666666019, 0.1000000000000000056, 0.1083333333333333370, 0.1166666666666666685, 0.1250000000000000000, 0.1333333333333333315, 0.1416666666666666630, 0.1499999999999999944, 0.1583333333333333259, 0.1666666666666666574, 0.1749999999999999889, 0.1833333333333333204, 0.1916666666666666796, 0.2000000000000000111, 0.2083333333333333426, 0.2166666666666666741, 0.2250000000000000056, 0.2333333333333333370, 0.2416666666666666685, 0.2500000000000000000, 0.2583333333333333592, 0.2666666666666666630, 0.2750000000000000222, 0.2833333333333333259, 0.2916666666666666852, 0.2999999999999999889, 0.3083333333333333481, 0.3166666666666666519, 0.3250000000000000111, 0.3333333333333333148, 0.3416666666666666741, 0.3499999999999999778, 0.3583333333333333370, 0.3666666666666666408, 0.3750000000000000000, 0.3833333333333333592, 0.3916666666666666630, 0.4000000000000000222, 0.4083333333333333259, 0.4166666666666666852, 0.4249999999999999889, 0.4333333333333333481, 0.4416666666666666519, 0.4500000000000000111, 0.4583333333333333148, 0.4666666666666666741, 0.4749999999999999778, 0.4833333333333333370, 0.4916666666666666408, 0.5000000000000000000, 0.5083333333333333037, 0.5166666666666667185, 0.5250000000000000222, 0.5333333333333333259, 0.5416666666666666297, 0.5500000000000000444, 0.5583333333333333481, 0.5666666666666666519, 0.5749999999999999556, 0.5833333333333333703, 0.5916666666666666741, 0.5999999999999999778, 0.6083333333333332815, 0.6166666666666666963, 0.6250000000000000000, 0.6333333333333333037, 0.6416666666666667185, 0.6500000000000000222, 0.6583333333333333259, 0.6666666666666666297, 0.6750000000000000444, 0.6833333333333333481, 0.6916666666666666519, 0.6999999999999999556, 0.7083333333333333703, 0.7166666666666666741, 0.7249999999999999778, 0.7333333333333332815, 0.7416666666666666963, 0.7500000000000000000, 0.7583333333333333037, 0.7666666666666667185, 0.7750000000000000222, 0.7833333333333333259, 0.7916666666666666297, 0.8000000000000000444, 0.8083333333333333481, 0.8166666666666666519, 0.8249999999999999556, 0.8333333333333333703, 0.8416666666666666741, 0.8499999999999999778, 0.8583333333333332815, 0.8666666666666666963, 0.8750000000000000000, 0.8833333333333333037, 0.8916666666666667185, 0.9000000000000000222, 0.9083333333333333259, 0.9166666666666666297, 0.9250000000000000444, 0.9333333333333333481, 0.9416666666666666519, 0.9499999999999999556, 0.9583333333333333703, 0.9666666666666666741, 0.9749999999999999778, 0.9833333333333332815, 0.9916666666666666963, 1.000000000000000000 ),
 .UNSPECIFIED. ) 
 GEOMETRIC_REPRESENTATION_ITEM ( )  RATIONAL_B_SPLINE_SURFACE ( (
 ( 1.000000000000000000, 0.8660254037844387076, 1.000000000000000000, 0.8660254037844387076, 1.000000000000000000, 0.8660254037844387076, 1.000000000000000000, 0.8660254037844387076, 1.000000000000000000, 0.8660254037844387076, 1.000000000000000000, 0.8660254037844387076, 1.000000000000000000, 0.8660254037844387076, 1.000000000000000000, 0.8660254037844387076, 1.000000000000000000, 0.8660254037844387076, 1.000000000000000000, 0.8660254037844387076, 1.000000000000000000, 0.8660254037844387076, 1.000000000000000000, 0.8660254037844387076, 1.000000000000000000, 0.8660254037844387076, 1.000000000000000000, 0.8660254037844387076, 1.000000000000000000, 0.8660254037844387076, 1.000000000000000000, 0.8660254037844387076, 1.000000000000000000, 0.8660254037844387076, 1.000000000000000000, 0.8660254037844387076, 1.000000000000000000, 0.8660254037844387076, 1.000000000000000000, 0.8660254037844387076, 1.000000000000000000, 0.8660254037844387076, 1.000000000000000000, 0.8660254037844387076, 1.000000000000000000, 0.8660254037844387076, 1.000000000000000000, 0.8660254037844387076, 1.000000000000000000, 0.8660254037844387076, 1.000000000000000000, 0.8660254037844387076, 1.000000000000000000, 0.8660254037844387076, 1.000000000000000000, 0.8660254037844387076, 1.000000000000000000, 0.8660254037844387076, 1.000000000000000000, 0.8660254037844387076, 1.000000000000000000, 0.8660254037844387076, 1.000000000000000000, 0.8660254037844387076, 1.000000000000000000, 0.8660254037844387076, 1.000000000000000000, 0.8660254037844387076, 1.000000000000000000, 0.8660254037844387076, 1.000000000000000000, 0.8660254037844387076, 1.000000000000000000, 0.8660254037844387076, 1.000000000000000000, 0.8660254037844387076, 1.000000000000000000, 0.8660254037844387076, 1.000000000000000000, 0.8660254037844387076, 1.000000000000000000, 0.8660254037844387076, 1.000000000000000000, 0.8660254037844387076, 1.000000000000000000, 0.8660254037844387076, 1.000000000000000000, 0.8660254037844387076, 1.000000000000000000, 0.8660254037844387076, 1.000000000000000000, 0.8660254037844387076, 1.000000000000000000, 0.8660254037844387076, 1.000000000000000000, 0.8660254037844387076, 1.000000000000000000, 0.8660254037844387076, 1.000000000000000000, 0.8660254037844387076, 1.000000000000000000, 0.8660254037844387076, 1.000000000000000000, 0.8660254037844387076, 1.000000000000000000, 0.8660254037844387076, 1.000000000000000000, 0.8660254037844387076, 1.000000000000000000, 0.8660254037844387076, 1.000000000000000000, 0.8660254037844387076, 1.000000000000000000, 0.8660254037844387076, 1.000000000000000000, 0.8660254037844387076, 1.000000000000000000, 0.8660254037844387076, 1.000000000000000000, 0.8660254037844387076, 1.000000000000000000, 0.8660254037844387076, 1.000000000000000000, 0.8660254037844387076, 1.000000000000000000, 0.8660254037844387076, 1.000000000000000000, 0.8660254037844387076, 1.000000000000000000, 0.8660254037844387076, 1.000000000000000000, 0.8660254037844387076, 1.000000000000000000, 0.8660254037844387076, 1.000000000000000000, 0.8660254037844387076, 1.000000000000000000, 0.8660254037844387076, 1.000000000000000000, 0.8660254037844387076, 1.000000000000000000, 0.8660254037844387076, 1.000000000000000000, 0.8660254037844387076, 1.000000000000000000, 0.8660254037844387076, 1.000000000000000000, 0.8660254037844387076, 1.000000000000000000, 0.8660254037844387076, 1.000000000000000000, 0.8660254037844387076, 1.000000000000000000, 0.8660254037844387076, 1.000000000000000000, 0.8660254037844387076, 1.000000000000000000, 0.8660254037844387076, 1.000000000000000000, 0.8660254037844387076, 1.000000000000000000, 0.8660254037844387076, 1.000000000000000000, 0.8660254037844387076, 1.000000000000000000, 0.8660254037844387076, 1.000000000000000000, 0.8660254037844387076, 1.000000000000000000, 0.8660254037844387076, 1.000000000000000000, 0.8660254037844387076, 1.000000000000000000, 0.8660254037844387076, 1.000000000000000000, 0.8660254037844387076, 1.000000000000000000, 0.8660254037844387076, 1.000000000000000000, 0.8660254037844387076, 1.000000000000000000, 0.8660254037844387076, 1.000000000000000000, 0.8660254037844387076, 1.000000000000000000, 0.8660254037844387076, 1.000000000000000000, 0.8660254037844387076, 1.000000000000000000, 0.8660254037844387076, 1.000000000000000000, 0.8660254037844387076, 1.000000000000000000, 0.8660254037844387076, 1.000000000000000000, 0.8660254037844387076, 1.000000000000000000, 0.8660254037844387076, 1.000000000000000000, 0.8660254037844387076, 1.000000000000000000, 0.8660254037844387076, 1.000000000000000000, 0.8660254037844387076, 1.000000000000000000, 0.8660254037844387076, 1.000000000000000000, 0.8660254037844387076, 1.000000000000000000, 0.8660254037844387076, 1.000000000000000000, 0.8660254037844387076, 1.000000000000000000, 0.8660254037844387076, 1.000000000000000000, 0.8660254037844387076, 1.000000000000000000, 0.8660254037844387076, 1.000000000000000000, 0.8660254037844387076, 1.000000000000000000, 0.8660254037844387076, 1.000000000000000000, 0.8660254037844387076, 1.000000000000000000, 0.8660254037844387076, 1.000000000000000000, 0.8660254037844387076, 1.000000000000000000, 0.8660254037844387076, 1.000000000000000000, 0.8660254037844387076, 1.000000000000000000, 0.8660254037844387076, 1.000000000000000000, 0.8660254037844387076, 1.000000000000000000, 0.8660254037844387076, 1.000000000000000000, 0.8660254037844387076, 1.000000000000000000),
 ( 1.000000000000000000, 0.8660254037844387076, 1.000000000000000000, 0.8660254037844387076, 1.000000000000000000, 0.8660254037844387076, 1.000000000000000000, 0.8660254037844387076, 1.000000000000000000, 0.8660254037844387076, 1.000000000000000000, 0.8660254037844387076, 1.000000000000000000, 0.8660254037844387076, 1.000000000000000000, 0.8660254037844387076, 1.000000000000000000, 0.8660254037844387076, 1.000000000000000000, 0.8660254037844387076, 1.000000000000000000, 0.8660254037844387076, 1.000000000000000000, 0.8660254037844387076, 1.000000000000000000, 0.8660254037844387076, 1.000000000000000000, 0.8660254037844387076, 1.000000000000000000, 0.8660254037844387076, 1.000000000000000000, 0.8660254037844387076, 1.000000000000000000, 0.8660254037844387076, 1.000000000000000000, 0.8660254037844387076, 1.000000000000000000, 0.8660254037844387076, 1.000000000000000000, 0.8660254037844387076, 1.000000000000000000, 0.8660254037844387076, 1.000000000000000000, 0.8660254037844387076, 1.000000000000000000, 0.8660254037844387076, 1.000000000000000000, 0.8660254037844387076, 1.000000000000000000, 0.8660254037844387076, 1.000000000000000000, 0.8660254037844387076, 1.000000000000000000, 0.8660254037844387076, 1.000000000000000000, 0.8660254037844387076, 1.000000000000000000, 0.8660254037844387076, 1.000000000000000000, 0.8660254037844387076, 1.000000000000000000, 0.8660254037844387076, 1.000000000000000000, 0.8660254037844387076, 1.000000000000000000, 0.8660254037844387076, 1.000000000000000000, 0.8660254037844387076, 1.000000000000000000, 0.8660254037844387076, 1.000000000000000000, 0.8660254037844387076, 1.000000000000000000, 0.8660254037844387076, 1.000000000000000000, 0.8660254037844387076, 1.000000000000000000, 0.8660254037844387076, 1.000000000000000000, 0.8660254037844387076, 1.000000000000000000, 0.8660254037844387076, 1.000000000000000000, 0.8660254037844387076, 1.000000000000000000, 0.8660254037844387076, 1.000000000000000000, 0.8660254037844387076, 1.000000000000000000, 0.8660254037844387076, 1.000000000000000000, 0.8660254037844387076, 1.000000000000000000, 0.8660254037844387076, 1.000000000000000000, 0.8660254037844387076, 1.000000000000000000, 0.8660254037844387076, 1.000000000000000000, 0.8660254037844387076, 1.000000000000000000, 0.8660254037844387076, 1.000000000000000000, 0.8660254037844387076, 1.000000000000000000, 0.8660254037844387076, 1.000000000000000000, 0.8660254037844387076, 1.000000000000000000, 0.8660254037844387076, 1.000000000000000000, 0.8660254037844387076, 1.000000000000000000, 0.8660254037844387076, 1.000000000000000000, 0.8660254037844387076, 1.000000000000000000, 0.8660254037844387076, 1.000000000000000000, 0.8660254037844387076, 1.000000000000000000, 0.8660254037844387076, 1.000000000000000000, 0.8660254037844387076, 1.000000000000000000, 0.8660254037844387076, 1.000000000000000000, 0.8660254037844387076, 1.000000000000000000, 0.8660254037844387076, 1.000000000000000000, 0.8660254037844387076, 1.000000000000000000, 0.8660254037844387076, 1.000000000000000000, 0.8660254037844387076, 1.000000000000000000, 0.8660254037844387076, 1.000000000000000000, 0.8660254037844387076, 1.000000000000000000, 0.8660254037844387076, 1.000000000000000000, 0.8660254037844387076, 1.000000000000000000, 0.8660254037844387076, 1.000000000000000000, 0.8660254037844387076, 1.000000000000000000, 0.8660254037844387076, 1.000000000000000000, 0.8660254037844387076, 1.000000000000000000, 0.8660254037844387076, 1.000000000000000000, 0.8660254037844387076, 1.000000000000000000, 0.8660254037844387076, 1.000000000000000000, 0.8660254037844387076, 1.000000000000000000, 0.8660254037844387076, 1.000000000000000000, 0.8660254037844387076, 1.000000000000000000, 0.8660254037844387076, 1.000000000000000000, 0.8660254037844387076, 1.000000000000000000, 0.8660254037844387076, 1.000000000000000000, 0.8660254037844387076, 1.000000000000000000, 0.8660254037844387076, 1.000000000000000000, 0.8660254037844387076, 1.000000000000000000, 0.8660254037844387076, 1.000000000000000000, 0.8660254037844387076, 1.000000000000000000, 0.8660254037844387076, 1.000000000000000000, 0.8660254037844387076, 1.000000000000000000, 0.8660254037844387076, 1.000000000000000000, 0.8660254037844387076, 1.000000000000000000, 0.8660254037844387076, 1.000000000000000000, 0.8660254037844387076, 1.000000000000000000, 0.8660254037844387076, 1.000000000000000000, 0.8660254037844387076, 1.000000000000000000, 0.8660254037844387076, 1.000000000000000000, 0.8660254037844387076, 1.000000000000000000, 0.8660254037844387076, 1.000000000000000000, 0.8660254037844387076, 1.000000000000000000, 0.8660254037844387076, 1.000000000000000000, 0.8660254037844387076, 1.000000000000000000, 0.8660254037844387076, 1.000000000000000000, 0.8660254037844387076, 1.000000000000000000, 0.8660254037844387076, 1.000000000000000000, 0.8660254037844387076, 1.000000000000000000, 0.8660254037844387076, 1.000000000000000000, 0.8660254037844387076, 1.000000000000000000, 0.8660254037844387076, 1.000000000000000000, 0.8660254037844387076, 1.000000000000000000, 0.8660254037844387076, 1.000000000000000000, 0.8660254037844387076, 1.000000000000000000, 0.8660254037844387076, 1.000000000000000000, 0.8660254037844387076, 1.000000000000000000, 0.8660254037844387076, 1.000000000000000000, 0.8660254037844387076, 1.000000000000000000, 0.8660254037844387076, 1.000000000000000000, 0.8660254037844387076, 1.000000000000000000) ) ) 
 REPRESENTATION_ITEM ( '' )  SURFACE ( )  );
#187124=CARTESIAN_POINT ( 'NONE',  ( -3.689227196694346400, 6.357829925235092716, -1.082531754730546636 ) ) ;
#187129=CARTESIAN_POINT ( 'NONE',  ( -5.144392941742557568, 4.966489618313220333, -0.7998128361456362523 ) ) ;
#187152=ORIENTED_EDGE ( 'NONE', *, *, #84784, .T. ) ;
#187153=CARTESIAN_POINT ( 'NONE',  ( -6.791708605802965870, 6.888357893050385705, -0.7998128361456362523 ) ) ;
#187155=CARTESIAN_POINT ( 'NONE',  ( -3.142457743317409680, 6.888227477170756785, 0.7998128361456352531 ) ) ;
#187179=CARTESIAN_POINT ( 'NONE',  ( 1.802380875475168898, 2.439898602870735456, 2.460315029152825961 ) ) ;
#187185=CARTESIAN_POINT ( 'NONE',  ( 5.817857313595521163, 9.801600942587855414, -0.7216878364870458196 ) ) ;
#187187=CARTESIAN_POINT ( 'NONE',  ( 4.579720705251352442, 8.490788101113528441, 0.3661988261168963588 ) ) ;
#187189=CARTESIAN_POINT ( 'NONE',  ( 1.865214468731738018, 8.973543201141316317, -0.7749999999999996891 ) ) ;
#187194=CARTESIAN_POINT ( 'NONE',  ( -5.586581854188635177, 5.810800913040471194, -0.4357733342581562863 ) ) ;
#187198=CARTESIAN_POINT ( 'NONE',  ( 5.734172623936983904, 5.654565914206774124, 0.7998128361456352531 ) ) ;
#187206=CARTESIAN_POINT ( 'NONE',  ( 5.851225812749518695, 8.984124660586543243, -1.199719254218452047 ) ) ;
#187208=CARTESIAN_POINT ( 'NONE',  ( 5.773793314573267388, 7.829454515125894964, 1.599625672291268286 ) ) ;
#187221=CARTESIAN_POINT ( 'NONE',  ( 6.176125489850557315, 6.957122458884915872, -0.8945188991977878201 ) ) ;
#187224=CARTESIAN_POINT ( 'NONE',  ( 5.478903473698239601, 7.485416367438324059, -1.443375672974078761 ) ) ;
#187232=CARTESIAN_POINT ( 'NONE',  ( -5.157951095356222204, 4.982307464195829816, 0.000000000000000000 ) ) ;
#187235=ORIENTED_EDGE ( 'NONE', *, *, #66529, .F. ) ;
#187244=CARTESIAN_POINT ( 'NONE',  ( -3.784134271545645412, 7.428924060196286483, 0.7216878364870338292 ) ) ;
#187248=CARTESIAN_POINT ( 'NONE',  ( 6.852720297064418986, 6.959538199522133262, 0.7998128361456331437 ) ) ;
#187300=ADVANCED_FACE ( 'NONE', ( #86333 ), #50309, .T. ) ;
#187307=CARTESIAN_POINT ( 'NONE',  ( 5.750066545971570520, 5.881034856487848295, -0.7216878364870458196 ) ) ;
#187314=CARTESIAN_POINT ( 'NONE',  ( 7.472478939787284169, 8.746922180287201698, 1.199719254218452935 ) ) ;
#187318=CARTESIAN_POINT ( 'NONE',  ( -5.492461627311929995, 5.580495784718250363, 0.000000000000000000 ) ) ;
#187338=CARTESIAN_POINT ( 'NONE',  ( 7.693325821111733021, 7.940244644243982464, -0.7998128361456341429 ) ) ;
#187348=CARTESIAN_POINT ( 'NONE',  ( 7.078765600110826561, 8.391552967285011988, -1.082531754730548412 ) ) ;
#187351=ORIENTED_EDGE ( 'NONE', *, *, #104398, .F. ) ;
#187360=CARTESIAN_POINT ( 'NONE',  ( -5.099275172515603138, 8.002885897026576600, 1.082531754730549967 ) ) ;
#187363=CARTESIAN_POINT ( 'NONE',  ( 6.851666526859736983, 9.086973262793417661, -1.599625672291269396 ) ) ;
#187368=CARTESIAN_POINT ( 'NONE',  ( -5.143339171537843590, 7.093924681584509173, 1.599625672291263179 ) ) ;
#187377=CARTESIAN_POINT ( 'NONE',  ( 3.984117037569365305, 5.741498858621315371, 1.599625672291261402 ) ) ;
#187382=DIRECTION ( 'NONE',  ( -0.7592566023653004592, -0.6507913734559639396, -0.000000000000000000 ) ) ;
#187406=CARTESIAN_POINT ( 'NONE',  ( 5.072158865288243668, 6.050511776658669127, 1.082531754730549078 ) ) ;
#187410=CARTESIAN_POINT ( 'NONE',  ( -6.794571259104023930, 7.956029886156682274, 1.199719254218452047 ) ) ;
#187414=CARTESIAN_POINT ( 'NONE',  ( -7.110325215724114578, 7.260077271291732082, 0.000000000000000000 ) ) ;
#187415=CARTESIAN_POINT ( 'NONE',  ( -4.118644803501354978, 8.027112380718707030, 0.7998128361456350310 ) ) ;
#187419=CARTESIAN_POINT ( 'NONE',  ( -7.444835747235459600, 8.818634805597074688, 1.082531754730549078 ) ) ;
#187423=CARTESIAN_POINT ( 'NONE',  ( 2.969872605471105764, 6.605953636083951253, 0.1972538285620730192 ) ) ;
#187427=CARTESIAN_POINT ( 'NONE',  ( -5.354544322754380303, 5.211666229493680191, 0.7998128361456281477 ) ) ;
#187435=CARTESIAN_POINT ( 'NONE',  ( -5.986807348886189040, 9.142303119412650503, -1.199719254218452047 ) ) ;
#187437=CARTESIAN_POINT ( 'NONE',  ( 5.441225816562971218, 7.512442699629209741, -1.249814574298679926 ) ) ;
#187441=CARTESIAN_POINT ( 'NONE',  ( 7.006746397889299871, 6.052176462752766106, 2.500000000000000444 ) ) ;
#187443=CARTESIAN_POINT ( 'NONE',  ( 5.086243903782109221, 5.962981304947771122, -1.199719254218452047 ) ) ;
#187453=CARTESIAN_POINT ( 'NONE',  ( -7.099629715411508890, 8.311931418515415615, 1.199719254218452047 ) ) ;
#187466=CARTESIAN_POINT ( 'NONE',  ( 5.110497557708379546, 4.926945003606695295, -0.7998128361456481317 ) ) ;
#187474=DIRECTION ( 'NONE',  ( -1.000000000000000000, 2.168404344971003504E-14, -0.000000000000000000 ) ) ;
#187479=CARTESIAN_POINT ( 'NONE',  ( 0.04469781632471583888, 2.590841079414101245, 2.082512688130889966 ) ) ;
#187480=CARTESIAN_POINT ( 'NONE',  ( 6.367678427751853221, 6.924687757192571347, 0.8275186136274095272 ) ) ;
#187481=AXIS2_PLACEMENT_3D ( 'NONE', #59143, #157734, #25570 ) ;
#187487=DIRECTION ( 'NONE',  ( -0.7592566023652995710, -0.6507913734559650498, 0.000000000000000000 ) ) ;
#187508=CARTESIAN_POINT ( 'NONE',  ( -5.873358954868365345, 7.276917811852929852, 1.275545277584020365 ) ) ;
#187526=CARTESIAN_POINT ( 'NONE',  ( -5.271087860662956537, 9.371629280740593870, 0.000000000000000000 ) ) ;
#187543=CARTESIAN_POINT ( 'NONE',  ( 3.250922972226694352, 7.014770244231638863, 0.7998128361456281477 ) ) ;
#187545=CARTESIAN_POINT ( 'NONE',  ( 6.278834536460164983, 9.379038488295265097, -1.082531754730548412 ) ) ;
#187551=CARTESIAN_POINT ( 'NONE',  ( 4.734293507696039960, 8.204026701335402905, 0.7038455069194777813 ) ) ;
#187556=EDGE_CURVE ( 'NONE', #117552, #183165, #52330, .T. ) ;
#187560=CARTESIAN_POINT ( 'NONE',  ( 5.123001941117305336, 7.070197912760590064, 1.599625672291268286 ) ) ;
#187570=CARTESIAN_POINT ( 'NONE',  ( -4.980641328173854632, 6.904110530993182948, 1.599625672291263179 ) ) ;
#187572=CARTESIAN_POINT ( 'NONE',  ( 7.842465510862060896, 8.114240948952696542, 0.000000000000000000 ) ) ;
#187576=CARTESIAN_POINT ( 'NONE',  ( -7.110325215724114578, 7.260077271291732082, 0.000000000000000000 ) ) ;
#187578=CARTESIAN_POINT ( 'NONE',  ( 5.956828388357757298, 8.042995434541133193, 1.599625672291269396 ) ) ;
#187584=CARTESIAN_POINT ( 'NONE',  ( -5.137161949866410282, 7.898551110135567654, 1.241398918778359173 ) ) ;
#187594=CARTESIAN_POINT ( 'NONE',  ( -5.451787166026575981, 5.533042246551999277, 0.000000000000000000 ) ) ;
#187603=CARTESIAN_POINT ( 'NONE',  ( 4.760321332173959696, 4.726332107057286791, 0.000000000000000000 ) ) ;
#187606=CARTESIAN_POINT ( 'NONE',  ( 5.017088295346122884, 4.896660802193717466, 0.1179097395585339686 ) ) ;
#187607=CARTESIAN_POINT ( 'NONE',  ( -5.966470118465691641, 9.118576350588734059, -1.199719254218452047 ) ) ;
#187615=CARTESIAN_POINT ( 'NONE',  ( -4.517335436343488553, 8.499999999999996447, 0.7749999999999996891 ) ) ;
#187620=FACE_OUTER_BOUND ( 'NONE', #159446, .T. ) ;
#187625=CARTESIAN_POINT ( 'NONE',  ( 6.062430963966053632, 7.101866208495718702, -1.199719254218452047 ) ) ;
#187636=ORIENTED_EDGE ( 'NONE', *, *, #55665, .T. ) ;
#187647=CARTESIAN_POINT ( 'NONE',  ( -4.882344714696960075, 5.829061934302122161, 1.082531754730549078 ) ) ;
#187670=CARTESIAN_POINT ( 'NONE',  ( -3.133342898089680695, 6.669667457830990465, 0.7216878364870338292 ) ) ;
#187678=CARTESIAN_POINT ( 'NONE',  ( -4.309512724297390740, 6.121127159803966933, 1.599625672291270506 ) ) ;
#187686=CARTESIAN_POINT ( 'NONE',  ( -5.503684012504701961, 5.385662534202396934, 0.000000000000000000 ) ) ;
#187692=CARTESIAN_POINT ( 'NONE',  ( 3.542423274920540432, 7.354853930707762721, -1.734723475976807094E-15 ) ) ;
#187699=CARTESIAN_POINT ( 'NONE',  ( -5.264308783856126439, 9.363720357799287797, -0.7998128361456362523 ) ) ;
#187702=CARTESIAN_POINT ( 'NONE',  ( -3.474632506852224356, 7.275764701294714420, -0.7998128361456481317 ) ) ;
#187707=CARTESIAN_POINT ( 'NONE',  ( 3.079110283634975964, 6.606396074300548982, 0.7216878364870257245 ) ) ;
#187708=CARTESIAN_POINT ( 'NONE',  ( -5.655159470231558849, 6.730679149092498648, 1.082531754730549078 ) ) ;
#187712=CARTESIAN_POINT ( 'NONE',  ( -5.971440312176176768, 5.931378217152456500, 0.000000000000000000 ) ) ;
#187715=CARTESIAN_POINT ( 'NONE',  ( 4.390861645979372341, 6.216034235099629157, -1.599625672291269396 ) ) ;
#187720=CARTESIAN_POINT ( 'NONE',  ( 2.969727409235598969, 6.579374545918310169, -0.3541450170054856184 ) ) ;
#187722=CARTESIAN_POINT ( 'NONE',  ( 6.066347387471824781, 6.042103138330730872, -0.7998128361456481317 ) ) ;
#187726=CARTESIAN_POINT ( 'NONE',  ( 5.703612580814390043, 7.410739916031705121, 1.319003781635886163 ) ) ;
#187734=VECTOR ( 'NONE', #56178, 1000.000000000000000 ) ;
#187737=CARTESIAN_POINT ( 'NONE',  ( 6.444921918449731280, 8.612437886315108315, 1.599625672291268286 ) ) ;
#187740=CARTESIAN_POINT ( 'NONE',  ( 5.899206235721897507, 6.055031161196562373, 0.000000000000000000 ) ) ;
#187747=CARTESIAN_POINT ( 'NONE',  ( 6.326190869690321961, 6.855918622363850190, 0.6739092513716876676 ) ) ;
#187763=CARTESIAN_POINT ( 'NONE',  ( -5.932574734431526942, 9.079031735882207244, 1.199719254218454489 ) ) ;
#187767=DIRECTION ( 'NONE',  ( 0.6507913734559641616, -0.7592566023653004592, 0.000000000000000000 ) ) ;
#187776=CARTESIAN_POINT ( 'NONE',  ( 5.091969210384201361, 8.098325291160362482, 1.199719254218452047 ) ) ;
#187783=( BOUNDED_CURVE ( )  B_SPLINE_CURVE ( 2, ( #14030, #198123, #49754, #130027, #147269, #80116, #115881 ),
 .UNSPECIFIED., .F., .T. ) 
 B_SPLINE_CURVE_WITH_KNOTS ( ( 3, 2, 2, 3 ),
 ( 0.4249999999999998224, 0.4333333333333331261, 0.4416666666666663743, 0.4499999999999996780 ),
 .UNSPECIFIED. ) 
 CURVE ( )  GEOMETRIC_REPRESENTATION_ITEM ( )  RATIONAL_B_SPLINE_CURVE ( ( 1.000000000000002665, 0.8660254037844360431, 1.000000000000000000, 0.8660254037844387076, 1.000000000000000000, 0.8660254037844440367, 0.9999999999999946709 ) ) 
 REPRESENTATION_ITEM ( '' )  );
#187784=CARTESIAN_POINT ( 'NONE',  ( -6.224601922005509991, 10.27613631906616476, 0.7216878364870267237 ) ) ;
#187786=CARTESIAN_POINT ( 'NONE',  ( 4.927462483923885195, 4.713404084191450849, -0.7998128361456481317 ) ) ;
#187789=CARTESIAN_POINT ( 'NONE',  ( 5.045042557616584489, 5.058506870073687267, 0.000000000000000000 ) ) ;
#187800=ORIENTED_EDGE ( 'NONE', *, *, #200712, .F. ) ;
#187804=CARTESIAN_POINT ( 'NONE',  ( -7.431277594066160397, 7.842447745931541370, -0.7216878364870338292 ) ) ;
#187805=CARTESIAN_POINT ( 'NONE',  ( 7.024532985656141371, 7.367912369453226695, 0.7216878364870328300 ) ) ;
#187816=CARTESIAN_POINT ( 'NONE',  ( -5.529746549527323474, 7.544733289238903851, -1.599625672291271394 ) ) ;
#187817=CARTESIAN_POINT ( 'NONE',  ( -3.471769853551161411, 6.208092708188416076, 1.199719254218452935 ) ) ;
#187819=CARTESIAN_POINT ( 'NONE',  ( 6.712695452097489301, 7.964471127936110229, -1.082531754730548412 ) ) ;
#187831=CARTESIAN_POINT ( 'NONE',  ( -4.945771867956824330, 7.989995641179508112, -1.012621479200847441 ) ) ;
#187835=CARTESIAN_POINT ( 'NONE',  ( 3.933273961740286317, 7.602920365423422311, 0.7216878364870257245 ) ) ;
#187839=CARTESIAN_POINT ( 'NONE',  ( -7.767895665986912057, 8.027242796598338614, -0.7998128361456362523 ) ) ;
#187852=CARTESIAN_POINT ( 'NONE',  ( 5.204350862799327793, 7.165104988056252289, -1.599625672291281386 ) ) ;
#187873=EDGE_CURVE ( 'NONE', #189704, #45344, #22649, .T. ) ;
#187888=CARTESIAN_POINT ( 'NONE',  ( 7.187230829020129441, 8.518095734345896730, 1.082531754730549967 ) ) ;
#187889=ORIENTED_EDGE ( 'NONE', *, *, #5202, .F. ) ;
#187894=CARTESIAN_POINT ( 'NONE',  ( 7.499068361690118145, 7.921536974826172361, -0.7216878364870317197 ) ) ;
#187907=CARTESIAN_POINT ( 'NONE',  ( -6.095272577795516789, 9.268845886473535245, 1.199719254218452047 ) ) ;
#187918=CARTESIAN_POINT ( 'NONE',  ( 4.001064729364292916, 6.721640380016713934, -1.082531754730548412 ) ) ;
#187923=VECTOR ( 'NONE', #126068, 1000.000000000000114 ) ;
#187925=CARTESIAN_POINT ( 'NONE',  ( -3.492107083971660586, 6.231819477012331632, 1.199719254218452935 ) ) ;
#187930=CARTESIAN_POINT ( 'NONE',  ( -5.777182853198894463, 9.754147405458438058, 0.7216878364870267237 ) ) ;
#187932=CARTESIAN_POINT ( 'NONE',  ( -1.812896364438562946, 2.514517768406681952, 2.499891510452760368 ) ) ;
#187933=CARTESIAN_POINT ( 'NONE',  ( -8.086512275908061653, 8.398962174839683215, 0.000000000000000000 ) ) ;
#187938=CARTESIAN_POINT ( 'NONE',  ( -3.800028193580205382, 7.655393002477360653, -0.7998128361456481317 ) ) ;
#187954=CARTESIAN_POINT ( 'NONE',  ( -3.987506576194992824, 7.666191748953863794, 0.7216878364870338292 ) ) ;
#187956=CARTESIAN_POINT ( 'NONE',  ( -4.407809337774280856, 7.196175756495025055, 1.082531754730549967 ) ) ;
#187958=CARTESIAN_POINT ( 'NONE',  ( 5.520104819419390907, 6.469152373191302985, 1.199719254218452935 ) ) ;
#187959=CARTESIAN_POINT ( 'NONE',  ( -5.468734858265826837, 7.473552982767158070, 1.599625672291263179 ) ) ;
#187960=CARTESIAN_POINT ( 'NONE',  ( -5.257529707049291900, 9.355811434857983500, 0.7998128361456291469 ) ) ;
#187980=CARTESIAN_POINT ( 'NONE',  ( 5.742760583840166966, 8.857581893525663830, 1.199719254218452047 ) ) ;
#188002=CARTESIAN_POINT ( 'NONE',  ( 5.722423353419669567, 8.833855124701747386, 1.199719254218451159 ) ) ;
#188008=CARTESIAN_POINT ( 'NONE',  ( 6.966220764712146796, 6.002124920821316323, -2.500000000000000444 ) ) ;
#188016=CARTESIAN_POINT ( 'NONE',  ( 6.574778147984297938, 6.635272358928617997, -0.7998128361456481317 ) ) ;
#188033=CARTESIAN_POINT ( 'NONE',  ( 4.095444919779759552, 6.935713618788495793, 1.199719254218451159 ) ) ;
#188039=CARTESIAN_POINT ( 'NONE',  ( -5.101610940492132151, 9.173906207207963348, -0.7998128361456362523 ) ) ;
#188043=CARTESIAN_POINT ( 'NONE',  ( 4.227110032410640095, 8.153655147779589996, 0.7998128361456271485 ) ) ;
#188056=CARTESIAN_POINT ( 'NONE',  ( 7.512626515748113576, 7.937354821227203594, 0.7216878364870267237 ) ) ;
#188057=CARTESIAN_POINT ( 'NONE',  ( -3.797692425603673705, 6.484372692295976570, 1.082531754730549967 ) ) ;
#188058=CARTESIAN_POINT ( 'NONE',  ( -5.424143973919053785, 8.485862515284315677, 1.199719254218454489 ) ) ;
#188065=ORIENTED_EDGE ( 'NONE', *, *, #40506, .F. ) ;
#188071=CARTESIAN_POINT ( 'NONE',  ( 4.206772801990143584, 8.129928378955675328, 0.7998128361456271485 ) ) ;
#188072=CARTESIAN_POINT ( 'NONE',  ( 4.603875680292229156, 7.528882839386387360, 1.199719254218452047 ) ) ;
#188075=CARTESIAN_POINT ( 'NONE',  ( 7.201315867513990554, 8.430565262634994284, -1.199719254218452047 ) ) ;
#188080=CARTESIAN_POINT ( 'NONE',  ( 3.719872605471109761, 6.605953636083950364, -2.500000000000002220 ) ) ;
#188093=CARTESIAN_POINT ( 'NONE',  ( 5.435893244436359240, 5.306573304789342416, -0.7998128361456481317 ) ) ;
#188094=CARTESIAN_POINT ( 'NONE',  ( 4.647606103345025552, 8.407977806742819027, 0.6343139517084724899 ) ) ;
#188099=CARTESIAN_POINT ( 'NONE',  ( 3.223806664999388172, 6.983134552466421674, -0.7998128361456362523 ) ) ;
#188105=CARTESIAN_POINT ( 'NONE',  ( 4.598150373690133463, 5.393538853173795111, -1.199719254218452047 ) ) ;
#188110=CARTESIAN_POINT ( 'NONE',  ( 5.722950238744200391, 7.770137593325314285, 1.443375672974065660 ) ) ;
#188112=CARTESIAN_POINT ( 'NONE',  ( -4.769436176957319695, 8.786368983084006601, 0.7998128361456281477 ) ) ;
#188114=CARTESIAN_POINT ( 'NONE',  ( 3.770049233051776749, 6.556085317605844232, 1.199719254218451159 ) ) ;
#188126=CARTESIAN_POINT ( 'NONE',  ( -2.959422669532919326, 6.674686557755516780, 0.7998128361456352531 ) ) ;
#188136=CARTESIAN_POINT ( 'NONE',  ( 0.4139252888115696472, 3.006731736636585328, -1.957985015624248204 ) ) ;
#188160=CARTESIAN_POINT ( 'NONE',  ( 5.996449078994045223, 10.21788403546024782, 0.7998128361456331437 ) ) ;
#188162=CARTESIAN_POINT ( 'NONE',  ( 7.635176783151273128, 8.936736330878529699, 1.199719254218452935 ) ) ;
#188176=CARTESIAN_POINT ( 'NONE',  ( -4.990283058281743678, 7.979691447040783814, -1.199719254218453823 ) ) ;
#188178=CARTESIAN_POINT ( 'NONE',  ( 6.658462837642799670, 6.940830530104329377, 0.7216878364870328300 ) ) ;
#188187=CARTESIAN_POINT ( 'NONE',  ( -4.797606254389363833, 6.690569611577942943, 1.599625672291263179 ) ) ;
#188191=CARTESIAN_POINT ( 'NONE',  ( -3.797692425603673705, 6.484372692295976570, 1.082531754730549967 ) ) ;
#188194=CARTESIAN_POINT ( 'NONE',  ( -5.659602779061863487, 5.567567761852417085, 0.7998128361456281477 ) ) ;
#188216=CARTESIAN_POINT ( 'NONE',  ( -5.818384198920079520, 6.817144982608731141, 1.199719254218452935 ) ) ;
#188218=CARTESIAN_POINT ( 'NONE',  ( -3.923105346307911745, 5.670318552149568703, -1.599625672291283607 ) ) ;
#188228=CARTESIAN_POINT ( 'NONE',  ( -5.946407990378149933, 7.222024315256661886, -1.239984355232233826 ) ) ;
#188242=CARTESIAN_POINT ( 'NONE',  ( -6.629010762438975135, 6.698543742459062145, -0.7998128361456362523 ) ) ;
#188263=CARTESIAN_POINT ( 'NONE',  ( 4.549643065837591038, 7.465611455855944101, -1.199719254218452047 ) ) ;
#188271=CARTESIAN_POINT ( 'NONE',  ( 7.038618024149998043, 8.240751112043669835, -1.199719254218452047 ) ) ;
#188273=CARTESIAN_POINT ( 'NONE',  ( 5.397027666691686321, 8.454226823519094935, 1.199719254218451159 ) ) ;
#188282=DIRECTION ( 'NONE',  ( 0.000000000000000000, 0.000000000000000000, -1.000000000000000000 ) ) ;
#188285=CARTESIAN_POINT ( 'NONE',  ( -1.806654366501805775, 9.001999999999998892, 2.420000000000000373 ) ) ;
#188286=CARTESIAN_POINT ( 'NONE',  ( 6.011645680221167076, 7.072102904328817274, -1.053258377668888857 ) ) ;
#188288=CARTESIAN_POINT ( 'NONE',  ( 5.641601317062233001, 7.675230518029648508, -1.443375672974078761 ) ) ;
#188296=CARTESIAN_POINT ( 'NONE',  ( -5.320648938720212051, 5.172121614787156929, 0.000000000000000000 ) ) ;
#188297=CARTESIAN_POINT ( 'NONE',  ( 3.686041076052345211, 7.355199913248151589, -0.03413285989870468856 ) ) ;
#188306=CARTESIAN_POINT ( 'NONE',  ( -3.946832114909637479, 7.618738210787614484, 0.7216878364870338292 ) ) ;
#188330=CARTESIAN_POINT ( 'NONE',  ( 5.559725510055676168, 8.644040974110419384, 1.199719254218451159 ) ) ;
#188368=CARTESIAN_POINT ( 'NONE',  ( 3.906157654512984134, 7.571284673658201569, -0.7216878364870338292 ) ) ;
#188380=CARTESIAN_POINT ( 'NONE',  ( -5.207740401424942434, 6.208690235484773723, 1.082531754730549078 ) ) ;
#188397=CARTESIAN_POINT ( 'NONE',  ( -4.036671995544492297, 7.285761072467114019, 0.7944190476826870073 ) ) ;
#188413=CARTESIAN_POINT ( 'NONE',  ( 3.607351389687783794, 6.366271167014519783, 1.199719254218451159 ) ) ;
#188427=CARTESIAN_POINT ( 'NONE',  ( -6.156811154381562012, 6.355570232966157640, 0.7216878364870257245 ) ) ;
#188430=CARTESIAN_POINT ( 'NONE',  ( 5.189738938980948291, 9.276722205444929870, 0.000000000000000000 ) ) ;
#188482=CARTESIAN_POINT ( 'NONE',  ( -5.759181390754928742, 9.941071732514568993, 0.000000000000000000 ) ) ;
#188485=CARTESIAN_POINT ( 'NONE',  ( -6.099189001301292379, 8.209082816308541197, 1.599625672291263179 ) ) ;
#188490=CARTESIAN_POINT ( 'NONE',  ( -6.956742217143487395, 8.249192353823097790, 1.082531754730549078 ) ) ;
#188495=ORIENTED_EDGE ( 'NONE', *, *, #117200, .F. ) ;
#188496=CARTESIAN_POINT ( 'NONE',  ( -4.842197138736131556, 5.678260079060780008, 1.199719254218452935 ) ) ;
#188503=CARTESIAN_POINT ( 'NONE',  ( -6.474900878978163021, 9.711745571186627402, -1.199719254218452047 ) ) ;
#188505=CARTESIAN_POINT ( 'NONE',  ( 5.061762083669725243, 7.855803969722688684, -1.119403510469544782 ) ) ;
#188511=CARTESIAN_POINT ( 'NONE',  ( 5.585032934186686226, 5.480569609498057382, 0.000000000000000000 ) ) ;
#188520=CARTESIAN_POINT ( 'NONE',  ( -8.072954122294394352, 8.383144328957069291, -0.7998128361456362523 ) ) ;
#188534=CARTESIAN_POINT ( 'NONE',  ( 6.587282531393223728, 8.778525268082516320, 1.599625672291268286 ) ) ;
#188549=CARTESIAN_POINT ( 'NONE',  ( 6.578229047358968629, 6.784305542873760864, 0.2988042929856441488 ) ) ;
#188562=ORIENTED_EDGE ( 'NONE', *, *, #106488, .T. ) ;
#188577=CARTESIAN_POINT ( 'NONE',  ( -6.279577920751266973, 6.982973266031838655, 0.9645283542769074181 ) ) ;
#188597=CARTESIAN_POINT ( 'NONE',  ( -5.094831863685302942, 9.165997284266655498, 0.7998128361456291469 ) ) ;
#188613=CARTESIAN_POINT ( 'NONE',  ( 3.386504508363381571, 7.172948703057747011, -0.7998128361456362523 ) ) ;
#188615=CARTESIAN_POINT ( 'NONE',  ( 7.200788982189461507, 8.533913579710086239, -1.082531754730548412 ) ) ;
#188625=CARTESIAN_POINT ( 'NONE',  ( 5.015976829175539109, 7.901154160799176651, 1.084432410706299477 ) ) ;
#188642=EDGE_LOOP ( 'NONE', ( #14790, #7784, #176915, #59564 ) ) ;
#188644=CARTESIAN_POINT ( 'NONE',  ( -4.034433228518296666, 6.864533312316751790, -1.199719254218450271 ) ) ;
#188646=CARTESIAN_POINT ( 'NONE',  ( 5.411639590510088027, 6.342609606130419131, -1.199719254218452047 ) ) ;
#188649=CARTESIAN_POINT ( 'NONE',  ( -6.798487682609798632, 6.896266815991691779, 0.7998128361456341429 ) ) ;
#188652=CARTESIAN_POINT ( 'NONE',  ( 6.526270840131753737, 8.707344961610770540, -1.599625672291283607 ) ) ;
#188656=DIRECTION ( 'NONE',  ( 1.000000000000000000, 0.000000000000000000, 0.000000000000000000 ) ) ;
#188658=B_SPLINE_CURVE_WITH_KNOTS ( 'NONE', 3,
 ( #188397, #40033, #19492, #106145, #172169, #68231 ),
 .UNSPECIFIED., .F., .F.,
 ( 4, 2, 4 ),
 ( 0.000000000000000000, 0.01245272936456226325, 0.02490545872912452649 ),
 .UNSPECIFIED. ) ;
#188659=CARTESIAN_POINT ( 'NONE',  ( -5.435611771797328906, 7.629049766310559200, 1.344574814272103236 ) ) ;
#188669=CARTESIAN_POINT ( 'NONE',  ( -4.570507181138272479, 7.385989907086349504, 1.082531754730549967 ) ) ;
#188678=CARTESIAN_POINT ( 'NONE',  ( 4.909461021924240498, 7.781436054670031410, 1.082531754730549078 ) ) ;
#188682=CARTESIAN_POINT ( 'NONE',  ( -5.413448473606448985, 9.537716662508005427, 0.000000000000000000 ) ) ;
#188684=VERTEX_POINT ( 'NONE', #63967 ) ;
#188700=CARTESIAN_POINT ( 'NONE',  ( 6.574778147984297938, 6.635272358928617109, -0.7998128361456481317 ) ) ;
#188712=VERTEX_POINT ( 'NONE', #211269 ) ;
#188722=CARTESIAN_POINT ( 'NONE',  ( -5.153507786970267013, 8.066157280557016307, -1.082531754730549967 ) ) ;
#188725=AXIS2_PLACEMENT_3D ( 'NONE', #160449, #211316, #12056 ) ;
#188735=EDGE_CURVE ( 'NONE', #183890, #203895, #192566, .T. ) ;
#188745=CARTESIAN_POINT ( 'NONE',  ( -7.445362632559989535, 8.715286488521982733, 1.199719254218452047 ) ) ;
#188746=CARTESIAN_POINT ( 'NONE',  ( -3.383641855062333281, 6.105276709951447778, -1.199719254218452047 ) ) ;
#188751=CARTESIAN_POINT ( 'NONE',  ( -5.469788628470539926, 5.346117919495872783, -0.7998128361456362523 ) ) ;
#188760=CARTESIAN_POINT ( 'NONE',  ( -5.901542003698421190, 10.10715911428198055, 0.000000000000000000 ) ) ;
#188762=CARTESIAN_POINT ( 'NONE',  ( 5.991454128980707949, 7.190850779781567503, -1.201235417510186254 ) ) ;
#188766=CARTESIAN_POINT ( 'NONE',  ( 4.583538449871731757, 7.505156070562471804, 1.199719254218451159 ) ) ;
#188771=CARTESIAN_POINT ( 'NONE',  ( -4.925354943514475003, 8.968274210734028529, 0.000000000000000000 ) ) ;
#188775=CARTESIAN_POINT ( 'NONE',  ( -5.632486471834530661, 5.535932070087196344, -0.7998128361456362523 ) ) ;
#188782=CARTESIAN_POINT ( 'NONE',  ( 5.411112705185558092, 6.445957923205511086, -1.082531754730548412 ) ) ;
#188784=CARTESIAN_POINT ( 'NONE',  ( -3.784134271545645412, 7.428924060196286483, 0.7216878364870338292 ) ) ;
#188786=EDGE_CURVE ( 'NONE', #24495, #198714, #48794, .T. ) ;
#188792=CARTESIAN_POINT ( 'NONE',  ( 5.225741863424510747, 5.061396693608882558, 0.7998128361456352531 ) ) ;
#188793=ORIENTED_EDGE ( 'NONE', *, *, #120455, .T. ) ;
#188805=CARTESIAN_POINT ( 'NONE',  ( 4.930145672075521013, 8.107674077938057167, 1.051636801887654293 ) ) ;
#188811=ORIENTED_EDGE ( 'NONE', *, *, #115920, .F. ) ;
#188815=CARTESIAN_POINT ( 'NONE',  ( 4.701645408888975197, 8.707279753670952971, 0.000000000000000000 ) ) ;
#188825=CARTESIAN_POINT ( 'NONE',  ( 6.137634773950260580, 6.983624353001562923, 0.9378011681944794509 ) ) ;
#188841=CARTESIAN_POINT ( 'NONE',  ( -7.119966945832006289, 8.335658187339330283, 1.199719254218452047 ) ) ;
#188844=FACE_OUTER_BOUND ( 'NONE', #82196, .T. ) ;
#188847=CARTESIAN_POINT ( 'NONE',  ( -3.986493660556410745, 7.309144847462942352, 0.7296485550502177508 ) ) ;
#188854=CARTESIAN_POINT ( 'NONE',  ( 5.365994935958575240, 9.482354201918870018, 0.7998128361456341429 ) ) ;
#188861=CARTESIAN_POINT ( 'NONE',  ( 5.225741863424510747, 5.061396693608882558, 0.7998128361456352531 ) ) ;
#188864=CARTESIAN_POINT ( 'NONE',  ( 5.058600711230250013, 5.074324715956299414, -0.7216878364870458196 ) ) ;
#188870=CARTESIAN_POINT ( 'NONE',  ( -6.486551268120854807, 6.767445667853342783, -0.2095380678983837508 ) ) ;
#188874=ORIENTED_EDGE ( 'NONE', *, *, #101627, .T. ) ;
#188877=CARTESIAN_POINT ( 'NONE',  ( -7.105881907338169157, 8.423188659050232729, -1.082531754730549967 ) ) ;
#188878=CARTESIAN_POINT ( 'NONE',  ( 4.523580528814945545, 5.306540700819438960, 1.199719254218452047 ) ) ;
#188888=CARTESIAN_POINT ( 'NONE',  ( -4.613517410400161722, 8.604463755433990002, -0.7998128361456362523 ) ) ;
#188889=CARTESIAN_POINT ( 'NONE',  ( -4.122561227007127016, 6.967349310553715647, 1.199719254218452935 ) ) ;
#188891=CARTESIAN_POINT ( 'NONE',  ( 5.194182247366861738, 9.073980031987776584, 0.7216878364870317197 ) ) ;
#188897=DIRECTION ( 'NONE',  ( -0.000000000000000000, -0.000000000000000000, -1.000000000000000000 ) ) ;
#188902=CARTESIAN_POINT ( 'NONE',  ( -4.719039639065737646, 8.241789607316443167, 0.6479098462880685805 ) ) ;
#188908=CARTESIAN_POINT ( 'NONE',  ( 5.397554552016226914, 6.430140077841320689, 1.082531754730549078 ) ) ;
#188914=CARTESIAN_POINT ( 'NONE',  ( -7.065734331377342414, 8.272386803808890576, -1.199719254218452047 ) ) ;
#188928=CARTESIAN_POINT ( 'NONE',  ( 4.529305835417093640, 7.441884687032027657, -1.199719254218450271 ) ) ;
#188962=CARTESIAN_POINT ( 'NONE',  ( 7.038091139269835317, 7.383730215335837954, 0.000000000000000000 ) ) ;
#188967=CARTESIAN_POINT ( 'NONE',  ( 7.973603738168424826, 8.475161580717541554, 0.000000000000000000 ) ) ;
#188993=CARTESIAN_POINT ( 'NONE',  ( -5.652823702255029836, 5.559658838911111900, -0.7998128361456362523 ) ) ;
#188995=CARTESIAN_POINT ( 'NONE',  ( 6.021229617800532452, 6.197391773621639288, 0.000000000000000000 ) ) ;
#189001=CARTESIAN_POINT ( 'NONE',  ( -5.004894982100124068, 5.868074229652107121, 1.199719254218452935 ) ) ;
#189008=CARTESIAN_POINT ( 'NONE',  ( -7.756673280794142755, 8.222076047114187602, -0.7216878364870338292 ) ) ;
#189011=CARTESIAN_POINT ( 'NONE',  ( -6.994027139803241866, 9.253060644560830994, -1.599625672291271394 ) ) ;
#189016=CARTESIAN_POINT ( 'NONE',  ( -4.797606254389363833, 6.690569611577942943, 1.599625672291263179 ) ) ;
#189031=CARTESIAN_POINT ( 'NONE',  ( -5.804299160426249493, 5.944306240018289778, -0.7216878364870338292 ) ) ;
#189034=CARTESIAN_POINT ( 'NONE',  ( -6.414416072596849538, 7.616478518518682073, -1.082531754730549967 ) ) ;
#189035=CARTESIAN_POINT ( 'NONE',  ( 7.374709211190586089, 7.568525266002632534, 0.000000000000000000 ) ) ;
#189036=CARTESIAN_POINT ( 'NONE',  ( -6.629010762438975135, 6.698543742459062145, -0.7998128361456362523 ) ) ;
#189052=CARTESIAN_POINT ( 'NONE',  ( 4.094259397040445947, 3.811769539470978962, 2.445515378722424860 ) ) ;
#189057=CARTESIAN_POINT ( 'NONE',  ( 8.039058738260216330, 8.343599714250547805, -0.7998128361456341429 ) ) ;
#189074=AXIS2_PLACEMENT_3D ( 'NONE', #173065, #24645, #28936 ) ;
#189096=CARTESIAN_POINT ( 'NONE',  ( 4.980641328173811999, 6.904110530993182948, 1.599625672291269396 ) ) ;
#189099=CARTESIAN_POINT ( 'NONE',  ( -5.503684012504701961, 5.385662534202396934, 0.000000000000000000 ) ) ;
#189113=CARTESIAN_POINT ( 'NONE',  ( 5.578253857379852576, 5.472660686556754861, -0.7998128361456481317 ) ) ;
#189121=CARTESIAN_POINT ( 'NONE',  ( -5.901542003698421190, 10.10715911428198055, 0.000000000000000000 ) ) ;
#189126=CARTESIAN_POINT ( 'NONE',  ( 5.411639590510088027, 6.342609606130419131, -1.199719254218452047 ) ) ;
#189135=CARTESIAN_POINT ( 'NONE',  ( 5.221298555038576872, 9.105615724271411082, 0.000000000000000000 ) ) ;
#189136=CARTESIAN_POINT ( 'NONE',  ( -4.556949027968976829, 5.449433633119473264, 1.082531754730549078 ) ) ;
#189137=CARTESIAN_POINT ( 'NONE',  ( -6.947627372360122955, 7.070263120700404968, 0.000000000000000000 ) ) ;
#189150=CARTESIAN_POINT ( 'NONE',  ( 5.499767588998890844, 6.445425604367387429, 1.199719254218451159 ) ) ;
#189151=CARTESIAN_POINT ( 'NONE',  ( 4.199993725183334803, 8.122019456014369254, -0.7998128361456362523 ) ) ;
#189154=CARTESIAN_POINT ( 'NONE',  ( 6.230854113932139171, 9.427024345299638952, 1.199719254218452047 ) ) ;
#189169=ADVANCED_FACE ( 'NONE', ( #20523 ), #100723, .T. ) ;
#189171=CARTESIAN_POINT ( 'NONE',  ( 5.408776937209000657, 5.274937613024121674, 0.7998128361456352531 ) ) ;
#189178=CARTESIAN_POINT ( 'NONE',  ( 5.896870467300973750, 5.844380064798101237, 0.7998128361456352531 ) ) ;
#189183=CARTESIAN_POINT ( 'NONE',  ( 5.083381250481017410, 4.895309311841474553, 0.7998128361456352531 ) ) ;
#189184=CARTESIAN_POINT ( 'NONE',  ( 5.459211493810820492, 6.084350935433496588, -0.8767179110168581424 ) ) ;
#189187=CARTESIAN_POINT ( 'NONE',  ( 6.590672070018850803, 7.822110515511036866, -1.082531754730548412 ) ) ;
#189190=CARTESIAN_POINT ( 'NONE',  ( -5.712781623311813384, 7.758274208654143855, -1.599625672291271394 ) ) ;
#189192=CARTESIAN_POINT ( 'NONE',  ( 6.066347387471824781, 6.042103138330730872, -0.7998128361456481317 ) ) ;
#189202=CARTESIAN_POINT ( 'NONE',  ( -6.400857919427531684, 9.521399101757175742, 1.082531754730549967 ) ) ;
#189232=CARTESIAN_POINT ( 'NONE',  ( 4.638297949650961982, 5.544340708415133712, -1.082531754730548412 ) ) ;
#189237=CARTESIAN_POINT ( 'NONE',  ( 7.075376061485196821, 9.347967719856493218, 1.599625672291268286 ) ) ;
#189239=CARTESIAN_POINT ( 'NONE',  ( 5.194182247366881278, 5.232503174782402233, 0.7216878364870328300 ) ) ;
#189244=AXIS2_PLACEMENT_3D ( 'NONE', #8627, #42226, #172217 ) ;
#189251=CARTESIAN_POINT ( 'NONE',  ( -7.096767062110449942, 7.244259425409119046, -0.7998128361456362523 ) ) ;
#189253=CARTESIAN_POINT ( 'NONE',  ( 6.983858524370772258, 9.241197259889668558, 1.443375672974063439 ) ) ;
#189262=CARTESIAN_POINT ( 'NONE',  ( -4.472210567661380587, 6.310941310395290493, 1.599625672291270506 ) ) ;
#189267=CARTESIAN_POINT ( 'NONE',  ( -3.350273356352693188, 6.922752992471175482, 0.000000000000000000 ) ) ;
#189271=CARTESIAN_POINT ( 'NONE',  ( -7.485510208520816278, 8.866088343763324886, 1.082531754730549078 ) ) ;
#189292=CARTESIAN_POINT ( 'NONE',  ( -7.605197822622922210, 7.837428646007010613, -0.7998128361456362523 ) ) ;
#189294=CARTESIAN_POINT ( 'NONE',  ( -5.178288325776719603, 5.006034233019745372, 0.000000000000000000 ) ) ;
#189304=CARTESIAN_POINT ( 'NONE',  ( -6.489832820117282353, 6.840411167308092288, -0.6218019135817691723 ) ) ;
#189320=CARTESIAN_POINT ( 'NONE',  ( -5.468734858265826837, 7.473552982767158070, 1.599625672291263179 ) ) ;
#189327=CARTESIAN_POINT ( 'NONE',  ( 7.810905894804431426, 8.285347430126213553, 0.000000000000000000 ) ) ;
#189336=CARTESIAN_POINT ( 'NONE',  ( -4.616310724566642598, 7.428787828840222041, 1.089621741958981094 ) ) ;
#189340=CARTESIAN_POINT ( 'NONE',  ( 4.064412189046650248, 7.963840997188264659, 0.7998128361456271485 ) ) ;
#189346=CARTESIAN_POINT ( 'NONE',  ( 5.525830126021535449, 8.604496359403894346, -1.199719254218452047 ) ) ;
#189348=CARTESIAN_POINT ( 'NONE',  ( 5.234329823327693809, 8.264412672927770487, 1.199719254218451159 ) ) ;
#189361=CARTESIAN_POINT ( 'NONE',  ( 6.335378924966214242, 6.849830188997488634, 0.6565068261209184852 ) ) ;
#189363=CARTESIAN_POINT ( 'NONE',  ( 5.397554552016216256, 7.390509292142662723, 1.443375672974065660 ) ) ;
#189370=CARTESIAN_POINT ( 'NONE',  ( -4.767627293860968507, 5.591261926706423857, -1.199719254218453823 ) ) ;
#189371=CARTESIAN_POINT ( 'NONE',  ( 3.671470136052636946, 7.354626245547865260, -0.09674656412868055944 ) ) ;
#189373=ORIENTED_EDGE ( 'NONE', *, *, #137043, .T. ) ;
#189381=CARTESIAN_POINT ( 'NONE',  ( -5.790741006368224753, 5.928488393617260321, 0.7216878364870257245 ) ) ;
#189382=LINE ( 'NONE', #59382, #53476 ) ;
#189385=CARTESIAN_POINT ( 'NONE',  ( 5.508355548902068577, 9.648441583686274470, 0.7998128361456331437 ) ) ;
#189386=CARTESIAN_POINT ( 'NONE',  ( 5.078858209280799230, 4.912784287789808246, -0.2022913385141849041 ) ) ;
#189402=CARTESIAN_POINT ( 'NONE',  ( 5.318541398310776103, 9.426991741329731056, -0.7998128361456481317 ) ) ;
#189423=CARTESIAN_POINT ( 'NONE',  ( -7.096767062110449942, 7.244259425409119046, -0.7998128361456362523 ) ) ;
#189444=CARTESIAN_POINT ( 'NONE',  ( 3.919715808126649659, 7.587102519540811940, 0.000000000000000000 ) ) ;
#189449=CARTESIAN_POINT ( 'NONE',  ( -5.921879234118920365, 10.13088588310589699, 0.000000000000000000 ) ) ;
#189452=CARTESIAN_POINT ( 'NONE',  ( -4.723994514485429619, 8.288620342878445513, -0.7462711413273189764 ) ) ;
#189455=CARTESIAN_POINT ( 'NONE',  ( -4.719646871332968452, 5.639247783710797712, 1.082531754730549078 ) ) ;
#189460=CARTESIAN_POINT ( 'NONE',  ( 4.796824973295459316, 8.251456047330133714, 0.8599625132450954279 ) ) ;
#189482=ORIENTED_EDGE ( 'NONE', *, *, #40036, .T. ) ;
#189486=CARTESIAN_POINT ( 'NONE',  ( 4.203910148689107729, 7.062256385849379647, -1.199719254218448494 ) ) ;
#189498=CARTESIAN_POINT ( 'NONE',  ( -6.780486220610184134, 9.003929572168926754, -1.443375672974066548 ) ) ;
#189500=CARTESIAN_POINT ( 'NONE',  ( 7.309781096423290769, 8.557108029695882578, 1.199719254218452935 ) ) ;
#189516=CARTESIAN_POINT ( 'NONE',  ( -3.350273356352693188, 6.922752992471175482, 0.000000000000000000 ) ) ;
#189541=DIRECTION ( 'NONE',  ( 1.000000000000000000, 0.000000000000000000, 0.000000000000000000 ) ) ;
#189546=CARTESIAN_POINT ( 'NONE',  ( -7.119966945832006289, 8.335658187339330283, 1.199719254218452047 ) ) ;
#189549=CARTESIAN_POINT ( 'NONE',  ( -6.231907884136888676, 7.299589282028351001, -1.199719254218453823 ) ) ;
#189555=CARTESIAN_POINT ( 'NONE',  ( -7.255021596644144921, 7.636815748939187465, 0.7216878364870317197 ) ) ;
#189556=EDGE_CURVE ( 'NONE', #6739, #211508, #24531, .T. ) ;
#189559=CARTESIAN_POINT ( 'NONE',  ( -4.864214080903581205, 4.879786425613829692, -0.6392378712632117432 ) ) ;
#189563=CARTESIAN_POINT ( 'NONE',  ( -5.752402313948099533, 9.933162809573264695, -0.7998128361456362523 ) ) ;
#189571=CARTESIAN_POINT ( 'NONE',  ( -6.957269102468015554, 8.145844036748005834, 1.199719254218452047 ) ) ;
#189572=CARTESIAN_POINT ( 'NONE',  ( 4.745935331938881951, 8.308991367555595531, -0.7587592799198628057 ) ) ;
#189575=CARTESIAN_POINT ( 'NONE',  ( 4.450244736158118108, 7.987476157872649196, 2.500000000000000444 ) ) ;
#189577=CARTESIAN_POINT ( 'NONE',  ( 5.969332771766739931, 10.18624834369502885, -0.7998128361456481317 ) ) ;
#189588=CARTESIAN_POINT ( 'NONE',  ( -7.208094944320834863, 8.438474185576302133, -1.199719254218452047 ) ) ;
#189600=CARTESIAN_POINT ( 'NONE',  ( 7.679767667498067496, 7.924426798361372093, 0.000000000000000000 ) ) ;
#189615=CARTESIAN_POINT ( 'NONE',  ( 6.459053645710411296, 6.863086831863287607, 0.6637952124323226455 ) ) ;
#189616=CARTESIAN_POINT ( 'NONE',  ( -5.926322542504884439, 6.086666852443364029, -0.7216878364870338292 ) ) ;
#189638=CIRCLE ( 'NONE', #172339, 0.08000000000000020983 ) ;
#189642=CARTESIAN_POINT ( 'NONE',  ( 5.727393547130178675, 5.646656991265468939, 0.000000000000000000 ) ) ;
#189646=ORIENTED_EDGE ( 'NONE', *, *, #5202, .T. ) ;
#189660=CARTESIAN_POINT ( 'NONE',  ( -6.577640801285370209, 7.702944352034914566, -1.199719254218452047 ) ) ;
#189672=ORIENTED_EDGE ( 'NONE', *, *, #44751, .F. ) ;
#189676=CARTESIAN_POINT ( 'NONE',  ( 3.711900195091365262, 7.552577004240394132, -0.7998128361456362523 ) ) ;
#189678=CARTESIAN_POINT ( 'NONE',  ( 7.363486825553451354, 8.723727730301414240, -1.082531754730548412 ) ) ;
#189688=CARTESIAN_POINT ( 'NONE',  ( 6.137634773950260580, 6.983624353001562923, 0.9378011681944794509 ) ) ;
#189704=VERTEX_POINT ( 'NONE', #88755 ) ;
#189706=CARTESIAN_POINT ( 'NONE',  ( -4.842197138736131556, 5.678260079060780008, 1.199719254218452935 ) ) ;
#189708=CARTESIAN_POINT ( 'NONE',  ( 4.573896719763862251, 6.429575154514868274, -1.599625672291273171 ) ) ;
#189711=CARTESIAN_POINT ( 'NONE',  ( -6.784929528996132220, 6.880448970109080520, 0.000000000000000000 ) ) ;
#189714=VECTOR ( 'NONE', #162740, 1000.000000000000114 ) ;
#189715=CARTESIAN_POINT ( 'NONE',  ( 6.013923656113508542, 9.173938811177871244, -1.199719254218452047 ) ) ;
#189721=CARTESIAN_POINT ( 'NONE',  ( -5.114454317065560751, 7.920171510810852133, -1.228010840421199568 ) ) ;
#189724=EDGE_CURVE ( 'NONE', #199128, #47264, #40000, .T. ) ;
#189729=CARTESIAN_POINT ( 'NONE',  ( -5.329763783503577379, 6.351050847909847086, 1.082531754730549078 ) ) ;
#189737=CARTESIAN_POINT ( 'NONE',  ( 5.722950238744211937, 5.849399164722627553, 0.7216878364870328300 ) ) ;
#189738=CARTESIAN_POINT ( 'NONE',  ( -5.458264003855187951, 7.602368174425947700, -1.382272695577278387 ) ) ;
#189741=CARTESIAN_POINT ( 'NONE',  ( -7.910256278930404505, 8.193330178365746619, -0.7998128361456362523 ) ) ;
#189750=CARTESIAN_POINT ( 'NONE',  ( -4.095971805104331231, 5.871996087412059140, 1.443375672974065660 ) ) ;
#189754=CARTESIAN_POINT ( 'NONE',  ( 4.167806878822868377, 7.207497389070224081, 1.120509907031017605 ) ) ;
#189755=CARTESIAN_POINT ( 'NONE',  ( 3.410758162289653672, 6.136912401716668519, -1.199719254218453823 ) ) ;
#189782=DIRECTION ( 'NONE',  ( 0.7592566023652995710, -0.6507913734559650498, 0.000000000000000000 ) ) ;
#189785=CARTESIAN_POINT ( 'NONE',  ( -6.644904684473536882, 6.925012684740138980, 0.7216878364870317197 ) ) ;
#189808=CARTESIAN_POINT ( 'NONE',  ( -3.296040741453672318, 6.859481608422314025, 0.7216878364870338292 ) ) ;
#189816=CARTESIAN_POINT ( 'NONE',  ( -5.822300622425855110, 5.757381912443740646, 0.7998128361456281477 ) ) ;
#189821=ORIENTED_EDGE ( 'NONE', *, *, #102547, .T. ) ;
#189825=CARTESIAN_POINT ( 'NONE',  ( -4.004454267989906668, 5.765225627445230927, 1.599625672291270506 ) ) ;
#189827=CARTESIAN_POINT ( 'NONE',  ( 5.494857653270467601, 7.581134149042087600, -1.337725346733337872 ) ) ;
#189831=CARTESIAN_POINT ( 'NONE',  ( 4.903208829997618423, 5.749440385532527564, -1.199719254218450271 ) ) ;
#189838=CARTESIAN_POINT ( 'NONE',  ( -7.449279056065764237, 7.655523418356991350, 0.7998128361456341429 ) ) ;
#189842=CARTESIAN_POINT ( 'NONE',  ( -4.930325137224961907, 5.781076077297750970, -1.199719254218453823 ) ) ;
#189847=CARTESIAN_POINT ( 'NONE',  ( 4.380693030546905398, 8.124909279031149012, 0.7216878364870247253 ) ) ;
#189848=CARTESIAN_POINT ( 'NONE',  ( -4.624739795592936353, 7.449261290616792763, -1.082531754730549967 ) ) ;
#189852=CARTESIAN_POINT ( 'NONE',  ( -5.581116510680924847, 6.540332679663050541, -1.199719254218453823 ) ) ;
#189855=CARTESIAN_POINT ( 'NONE',  ( 5.239300017038202917, 5.077214539491492928, 0.000000000000000000 ) ) ;
#189868=CARTESIAN_POINT ( 'NONE',  ( 5.275877007301786215, 7.772378248882220397, 1.293907329011657614 ) ) ;
#189878=CARTESIAN_POINT ( 'NONE',  ( 6.658989722967328717, 7.797851427330578566, 1.199719254218452935 ) ) ;
#189890=CARTESIAN_POINT ( 'NONE',  ( 6.017777097630443883, 7.067734144800174256, 1.048426327298467742 ) ) ;
#189897=CARTESIAN_POINT ( 'NONE',  ( 5.993586425693011144, 9.150212042353954800, -1.199719254218452047 ) ) ;
#189901=CARTESIAN_POINT ( 'NONE',  ( -4.768476522361002168, 8.183970109320437558, 0.7579922544750415936 ) ) ;
#189907=CARTESIAN_POINT ( 'NONE',  ( -7.391130018105325661, 8.652015104991543026, -1.199719254218452047 ) ) ;
#189920=CARTESIAN_POINT ( 'NONE',  ( 7.309781096423290769, 8.557108029695882578, 1.199719254218452935 ) ) ;
#189926=CARTESIAN_POINT ( 'NONE',  ( -6.061904078641520144, 10.08632216847484031, 0.7216878364870267237 ) ) ;
#189928=CARTESIAN_POINT ( 'NONE',  ( 5.415556014015861841, 5.282846535965431300, -0.7998128361456481317 ) ) ;
#189931=CARTESIAN_POINT ( 'NONE',  ( 3.879041346841291649, 7.539648981374564407, 1.040834085586084257E-14 ) ) ;
#189944=CARTESIAN_POINT ( 'NONE',  ( -6.455090533882193782, 9.584670485287619002, -1.082531754730549967 ) ) ;
#189946=CARTESIAN_POINT ( 'NONE',  ( 6.211043768836170820, 9.299949259400630552, 1.082531754730549967 ) ) ;
#189957=CARTESIAN_POINT ( 'NONE',  ( -5.123001941117347080, 7.070197912760590064, 1.599625672291263179 ) ) ;
#189958=CARTESIAN_POINT ( 'NONE',  ( -4.610654757099099221, 7.536791762327691657, 1.199719254218452935 ) ) ;
#189960=CARTESIAN_POINT ( 'NONE',  ( 7.065207446052794715, 9.336104335185329006, -1.443375672974064550 ) ) ;
#189967=DIRECTION ( 'NONE',  ( 0.7592566023653005702, 0.6507913734559639396, 0.000000000000000000 ) ) ;
#189971=CARTESIAN_POINT ( 'NONE',  ( -5.638797120722775169, 7.366710520292286901, -1.234282198493292793 ) ) ;
#189974=CARTESIAN_POINT ( 'NONE',  ( 4.665414256878284149, 6.536345614481700927, -1.443375672974068769 ) ) ;
#189979=CARTESIAN_POINT ( 'NONE',  ( -4.945692173934974178, 8.992000979557944973, 0.000000000000000000 ) ) ;
#189985=DIRECTION ( 'NONE',  ( -0.7592566023652990159, -0.6507913734559659380, 0.000000000000000000 ) ) ;
#189993=EDGE_CURVE ( 'NONE', #161612, #136572, #160136, .T. ) ;
#189994=CARTESIAN_POINT ( 'NONE',  ( 5.174371902270911150, 6.065797303184739420, 1.199719254218452047 ) ) ;
#190001=CYLINDRICAL_SURFACE ( 'NONE', #57462, 0.08000000000000041800 ) ;
#190030=CARTESIAN_POINT ( 'NONE',  ( 5.533136088152891929, 9.469426179571447832, -0.7216878364870458196 ) ) ;
#190035=CARTESIAN_POINT ( 'NONE',  ( 7.634649897826745857, 8.079715433652276957, 0.7216878364870267237 ) ) ;
#190060=CARTESIAN_POINT ( 'NONE',  ( -4.167152111353897403, 5.955039778036558040, 1.599625672291270506 ) ) ;
#190062=CARTESIAN_POINT ( 'NONE',  ( 6.061904078641523697, 7.205214525570814210, -1.082531754730548412 ) ) ;
#190068=CARTESIAN_POINT ( 'NONE',  ( -4.573896719763875574, 6.429575154514868274, -1.599625672291271394 ) ) ;
#190073=CARTESIAN_POINT ( 'NONE',  ( -7.132998214565509087, 7.494455136514109661, 0.7216878364870317197 ) ) ;
#190076=CARTESIAN_POINT ( 'NONE',  ( -5.576146316970437944, 9.727530813099326323, 0.000000000000000000 ) ) ;
#190080=CARTESIAN_POINT ( 'NONE',  ( -3.797165540279144214, 6.587721009371067638, 1.199719254218452935 ) ) ;
#190089=CARTESIAN_POINT ( 'NONE',  ( -4.981695098378565945, 4.776675467721892332, -0.7998128361456362523 ) ) ;
#190091=CARTESIAN_POINT ( 'NONE',  ( -4.312902262922974295, 8.045820050136510915, 0.7216878364870338292 ) ) ;
#190093=CARTESIAN_POINT ( 'NONE',  ( -6.305950843687521790, 7.489935751457798219, 1.082531754730548412 ) ) ;
#190094=CARTESIAN_POINT ( 'NONE',  ( 5.525830126021535449, 8.604496359403894346, -1.199719254218452047 ) ) ;
#190095=CARTESIAN_POINT ( 'NONE',  ( -6.479871072688648148, 6.524547437750345402, 0.000000000000000000 ) ) ;
#190100=FACE_OUTER_BOUND ( 'NONE', #203841, .T. ) ;
#190115=CARTESIAN_POINT ( 'NONE',  ( 5.677832469072920496, 9.846164657218904992, 0.000000000000000000 ) ) ;
#190135=EDGE_CURVE ( 'NONE', #108645, #824, #125133, .T. ) ;
#190153=CARTESIAN_POINT ( 'NONE',  ( 3.874598038455354665, 7.742391154831717692, -0.7998128361456362523 ) ) ;
#190156=CARTESIAN_POINT ( 'NONE',  ( -3.142457743317409680, 6.888227477170756785, 0.7998128361456352531 ) ) ;
#190159=CARTESIAN_POINT ( 'NONE',  ( -6.414416072596849538, 7.616478518518682073, -1.082531754730549967 ) ) ;
#190171=CARTESIAN_POINT ( 'NONE',  ( 6.668631453075247073, 8.873432343378178544, -1.599625672291281386 ) ) ;
#190172=CARTESIAN_POINT ( 'NONE',  ( 5.017399365509065845, 8.011327138806002779, -1.199719254218450271 ) ) ;
#190177=VERTEX_POINT ( 'NONE', #47475 ) ;
#190183=CARTESIAN_POINT ( 'NONE',  ( 4.899292406491845497, 6.809203455697518947, -1.599625672291273171 ) ) ;
#190191=CARTESIAN_POINT ( 'NONE',  ( 6.780486220610169035, 9.003929572168926754, -1.443375672974078761 ) ) ;
#190192=CARTESIAN_POINT ( 'NONE',  ( -4.340018570150322219, 5.196348098997705556, -1.082531754730551743 ) ) ;
#190194=CARTESIAN_POINT ( 'NONE',  ( -5.250750630242457362, 9.347902511916677426, 0.000000000000000000 ) ) ;
#190203=CARTESIAN_POINT ( 'NONE',  ( 5.494797395288433250, 9.632623737803665875, 0.000000000000000000 ) ) ;
#190204=CARTESIAN_POINT ( 'NONE',  ( 4.692003678781083487, 7.631698837623355658, -1.199719254218450271 ) ) ;
#190205=CARTESIAN_POINT ( 'NONE',  ( 5.176180785367283654, 9.260904359562321275, -0.7998128361456481317 ) ) ;
#190208=CARTESIAN_POINT ( 'NONE',  ( 6.282224075085741433, 8.422623735723785643, 1.599625672291268286 ) ) ;
#190227=CARTESIAN_POINT ( 'NONE',  ( 3.725458348705031231, 7.568394850123006279, -1.734723475976807094E-15 ) ) ;
#190231=CARTESIAN_POINT ( 'NONE',  ( 4.389807875774629942, 8.343469298370917997, 0.7998128361456271485 ) ) ;
#190236=CARTESIAN_POINT ( 'NONE',  ( 6.373214726875630731, 9.593111727067046957, 1.199719254218452047 ) ) ;
#190241=ADVANCED_FACE ( 'NONE', ( #197457 ), #192105, .T. ) ;
#190242=CARTESIAN_POINT ( 'NONE',  ( 6.387299765813869712, 6.624473612970537495, 0.000000000000000000 ) ) ;
#190244=CARTESIAN_POINT ( 'NONE',  ( -4.793689830883590020, 7.750332681742931662, 1.199719254218452935 ) ) ;
#190245=CARTESIAN_POINT ( 'NONE',  ( 3.718679271898170491, 7.560485927181699317, 0.7998128361456271485 ) ) ;
#190255=CARTESIAN_POINT ( 'NONE',  ( -7.268579750702160780, 8.613002809641560731, -1.082531754730549967 ) ) ;
#190282=VECTOR ( 'NONE', #113965, 1000.000000000000114 ) ;
#190290=CARTESIAN_POINT ( 'NONE',  ( 6.912678218121202534, 9.158153569265168770, 1.599625672291268286 ) ) ;
#190291=CARTESIAN_POINT ( 'NONE',  ( 4.706088717274906408, 5.623429937309770921, 1.082531754730549078 ) ) ;
#190302=CARTESIAN_POINT ( 'NONE',  ( -6.608673532018475960, 6.674816973635147477, -0.7998128361456362523 ) ) ;
#190304=CARTESIAN_POINT ( 'NONE',  ( 7.648208051440442468, 8.095533279534887328, 0.000000000000000000 ) ) ;
#190314=CARTESIAN_POINT ( 'NONE',  ( -5.635349125135588721, 6.603604063193491136, 1.199719254218452935 ) ) ;
#190320=CARTESIAN_POINT ( 'NONE',  ( -4.095971805104331231, 5.871996087412059140, 1.443375672974065660 ) ) ;
#190325=CARTESIAN_POINT ( 'NONE',  ( -6.102578539926875933, 10.13377570664109051, 0.7216878364870267237 ) ) ;
#190346=CARTESIAN_POINT ( 'NONE',  ( -5.875479466675803231, 7.948088359245467416, -1.599625672291271394 ) ) ;
#190347=CARTESIAN_POINT ( 'NONE',  ( -4.858757509019059562, 5.629766575900002401, 2.420000000000000373 ) ) ;
#190374=CARTESIAN_POINT ( 'NONE',  ( -4.847922445338252118, 7.813604065273374921, -1.199719254218453823 ) ) ;
#190383=CARTESIAN_POINT ( 'NONE',  ( 7.200788982189461507, 8.533913579710086239, -1.082531754730548412 ) ) ;
#190400=CARTESIAN_POINT ( 'NONE',  ( 5.189738938980948291, 9.276722205444929870, 0.000000000000000000 ) ) ;
#190402=CARTESIAN_POINT ( 'NONE',  ( 6.150558962454855561, 7.204682206732687000, 1.199719254218452047 ) ) ;
#190404=B_SPLINE_CURVE_WITH_KNOTS ( 'NONE', 3,
 ( #22833, #88947, #155001, #56434 ),
 .UNSPECIFIED., .F., .F.,
 ( 4, 4 ),
 ( 0.001357288427014568134, 0.001636127605392573552 ),
 .UNSPECIFIED. ) ;
#190416=CARTESIAN_POINT ( 'NONE',  ( 6.353009478083933459, 6.838182937092724956, 0.6209923359970755952 ) ) ;
#190418=CARTESIAN_POINT ( 'NONE',  ( 5.885648082108199119, 6.999582529615296700, 1.082531754730549967 ) ) ;
#190434=CARTESIAN_POINT ( 'NONE',  ( -5.926322542504864899, 8.967774495347393682, -1.082531754730549967 ) ) ;
#190437=CARTESIAN_POINT ( 'NONE',  ( 5.494797395288433250, 9.632623737803665875, 0.000000000000000000 ) ) ;
#190445=CARTESIAN_POINT ( 'NONE',  ( -3.135678666510573365, 6.880318554229450712, 0.000000000000000000 ) ) ;
#190455=CARTESIAN_POINT ( 'NONE',  ( 6.749980374757213575, 8.968339418673846097, 1.599625672291268286 ) ) ;
#190473=CARTESIAN_POINT ( 'NONE',  ( -4.911796789900812144, 8.952456364851418158, 0.7998128361456291469 ) ) ;
#190477=CARTESIAN_POINT ( 'NONE',  ( -6.478676351974181458, 6.772485410396933858, 0.2589597434300341394 ) ) ;
#190495=CARTESIAN_POINT ( 'NONE',  ( 5.614485009834906393, 6.683225611963085733, -1.082531754730548412 ) ) ;
#190507=CARTESIAN_POINT ( 'NONE',  ( -3.851925040058337579, 6.547644075826416277, -1.082531754730546636 ) ) ;
#190510=EDGE_LOOP ( 'NONE', ( #78341, #92504, #45723, #139673 ) ) ;
#190533=CARTESIAN_POINT ( 'NONE',  ( 3.147653791585693028, 8.920000000000001705, 2.499999999999999556 ) ) ;
#190540=CARTESIAN_POINT ( 'NONE',  ( 4.740510986633625024, 5.559626234941203116, -1.199719254218450271 ) ) ;
#190550=CARTESIAN_POINT ( 'NONE',  ( -5.451787166470911217, 9.374519104275787384, 0.7216878364870267237 ) ) ;
#190552=CARTESIAN_POINT ( 'NONE',  ( 3.390947816749319443, 6.970206529600588397, -1.734723475976807094E-15 ) ) ;
#190569=CARTESIAN_POINT ( 'NONE',  ( 3.902768115887398803, 5.646591783325653147, -1.599625672291269396 ) ) ;
#190571=CARTESIAN_POINT ( 'NONE',  ( -4.502716413514313842, 5.386162249589033557, -1.082531754730549967 ) ) ;
#190575=CARTESIAN_POINT ( 'NONE',  ( -3.719872605471121751, 6.605953636083950364, 2.420000000000000373 ) ) ;
#190601=CARTESIAN_POINT ( 'NONE',  ( -7.944151662964566540, 8.232874793072271657, 0.000000000000000000 ) ) ;
#190604=CARTESIAN_POINT ( 'NONE',  ( -4.990283058281743678, 7.979691447040783814, -1.199719254218453823 ) ) ;
#190605=CARTESIAN_POINT ( 'NONE',  ( -4.793689830883590020, 7.750332681742931662, 1.199719254218452935 ) ) ;
#190609=CARTESIAN_POINT ( 'NONE',  ( -5.750066545527201534, 9.722511713174800008, 0.000000000000000000 ) ) ;
#190611=CARTESIAN_POINT ( 'NONE',  ( -3.142457743317409680, 6.888227477170756785, 0.7998128361456352531 ) ) ;
#190614=ORIENTED_EDGE ( 'NONE', *, *, #41407, .F. ) ;
#190615=CARTESIAN_POINT ( 'NONE',  ( -5.738844160334429567, 9.917344963690652548, 0.000000000000000000 ) ) ;
#190623=CARTESIAN_POINT ( 'NONE',  ( -7.306918443122272677, 7.489436036589583345, 0.7998128361456341429 ) ) ;
#190624=EDGE_LOOP ( 'NONE', ( #28101, #2172, #163212, #36855 ) ) ;
#190625=CARTESIAN_POINT ( 'NONE',  ( 5.303225773876714122, 7.631601692149430072, -1.229104931163179426 ) ) ;
#190629=CARTESIAN_POINT ( 'NONE',  ( 3.573456005653643519, 6.326726552307992080, -1.199719254218453823 ) ) ;
#190651=CARTESIAN_POINT ( 'NONE',  ( 4.947799714344386146, 4.737130853015369958, -0.7998128361456481317 ) ) ;
#190663=CARTESIAN_POINT ( 'NONE',  ( 0.4639452589547733985, 2.947031273455551492, 1.945529950462648205 ) ) ;
#190666=DIRECTION ( 'NONE',  ( -0.000000000000000000, -0.000000000000000000, -1.000000000000000000 ) ) ;
#190667=CARTESIAN_POINT ( 'NONE',  ( 5.869365784521903606, 7.282179437329668659, 1.264975801879052453 ) ) ;
#190668=CARTESIAN_POINT ( 'NONE',  ( -5.492461626867567226, 6.540864998501174199, 1.082531754730549078 ) ) ;
#190698=CARTESIAN_POINT ( 'NONE',  ( 3.217027588192558074, 6.975225629525113824, -1.734723475976807094E-15 ) ) ;
#190709=CARTESIAN_POINT ( 'NONE',  ( 8.154303043976348420, 8.478051404252736845, 0.7998128361456281477 ) ) ;
#190718=CARTESIAN_POINT ( 'NONE',  ( -5.336015975430226099, 8.383046517047350932, -1.199719254218453823 ) ) ;
#190732=CARTESIAN_POINT ( 'NONE',  ( 4.061549535745618833, 6.896169004081968090, -1.199719254218452047 ) ) ;
#190741=CARTESIAN_POINT ( 'NONE',  ( 4.822014627293360611, 8.104635198319419587, 0.8657228342519827091 ) ) ;
#190744=CARTESIAN_POINT ( 'NONE',  ( 4.943016831304842817, 7.975319854387232787, 1.017975537214605319 ) ) ;
#190745=CARTESIAN_POINT ( 'NONE',  ( 5.020734711527275351, 8.014512191897464888, 1.145736749330818149 ) ) ;
#190763=LINE ( 'NONE', #42427, #88612 ) ;
#190764=CARTESIAN_POINT ( 'NONE',  ( -5.655686355556086120, 6.627330832017406692, 1.199719254218452935 ) ) ;
#190766=CARTESIAN_POINT ( 'NONE',  ( 5.571474780572990504, 5.464751763615448787, 0.7998128361456352531 ) ) ;
#190770=CARTESIAN_POINT ( 'NONE',  ( -5.098748287191073203, 8.106234214101666780, 1.199719254218452935 ) ) ;
#190773=CARTESIAN_POINT ( 'NONE',  ( 6.393551957296131683, 9.616838495890963401, 1.199719254218452047 ) ) ;
#190778=CARTESIAN_POINT ( 'NONE',  ( -4.818718062179155659, 8.223694781438435797, -0.9201054579500017594 ) ) ;
#190788=EDGE_CURVE ( 'NONE', #153847, #173630, #102053, .T. ) ;
#190797=CARTESIAN_POINT ( 'NONE',  ( 5.234856708652233515, 6.240325927249993576, 1.082531754730549078 ) ) ;
#190800=CARTESIAN_POINT ( 'NONE',  ( -5.427006627220116286, 9.553534508390610469, -0.7998128361456362523 ) ) ;
#190814=CARTESIAN_POINT ( 'NONE',  ( 3.953084306836263995, 6.769626237021087789, 1.199719254218452047 ) ) ;
#190831=ORIENTED_EDGE ( 'NONE', *, *, #213257, .F. ) ;
#190842=CARTESIAN_POINT ( 'NONE',  ( -4.475600106286965918, 8.235634200727838916, 0.7216878364870338292 ) ) ;
#190867=CARTESIAN_POINT ( 'NONE',  ( -5.772739544368596043, 9.956889578397179363, -0.7998128361456362523 ) ) ;
#190872=CARTESIAN_POINT ( 'NONE',  ( -4.146814880933400005, 5.931313009212638931, 1.599625672291270506 ) ) ;
#190881=CARTESIAN_POINT ( 'NONE',  ( -2.830620210203090181, 6.524417021870718258, 0.000000000000000000 ) ) ;
#190883=CARTESIAN_POINT ( 'NONE',  ( 6.142241479726070708, 7.081583759122534794, -1.089790755372788800 ) ) ;
#190887=CARTESIAN_POINT ( 'NONE',  ( 5.337069745634900997, 6.255611453776062980, 1.199719254218452047 ) ) ;
#190893=CARTESIAN_POINT ( 'NONE',  ( -2.844178363816758814, 6.540234867753325076, -0.7998128361456481317 ) ) ;
#190898=CARTESIAN_POINT ( 'NONE',  ( -4.797606254389363833, 6.690569611577942943, 1.599625672291263179 ) ) ;
#190904=CARTESIAN_POINT ( 'NONE',  ( 5.031484404002878996, 7.923796667095108326, 1.082531754730548412 ) ) ;
#190905=CARTESIAN_POINT ( 'NONE',  ( -6.414416072596857532, 6.656109304217339151, -0.7216878364870338292 ) ) ;
#190908=CARTESIAN_POINT ( 'NONE',  ( -4.990283058281743678, 7.979691447040783814, -1.199719254218453823 ) ) ;
#190911=CARTESIAN_POINT ( 'NONE',  ( 3.444653546323793947, 6.176457016423196222, 1.199719254218451159 ) ) ;
#190915=CARTESIAN_POINT ( 'NONE',  ( -4.489620702586434753, 8.251817990458562235, -0.01816452336140990040 ) ) ;
#190919=FILL_AREA_STYLE ('',( #158443 ) ) ;
#190940=CARTESIAN_POINT ( 'NONE',  ( 4.596835240751270035, 8.371391889155539445, -0.09823007671119071693 ) ) ;
#190947=CARTESIAN_POINT ( 'NONE',  ( 6.855582950365507244, 8.027210192628430718, -1.199719254218452047 ) ) ;
#190951=CARTESIAN_POINT ( 'NONE',  ( -4.611386515133914621, 8.374621496872018511, -0.1785149356163841239 ) ) ;
#190957=CARTESIAN_POINT ( 'NONE',  ( -7.065734331377342414, 8.272386803808890576, -1.199719254218452047 ) ) ;
#190970=CARTESIAN_POINT ( 'NONE',  ( 5.040599249230596435, 9.102725900736217568, 0.7998128361456341429 ) ) ;
#190976=AXIS2_PLACEMENT_3D ( 'NONE', #13948, #97376, #142949 ) ;
#190978=ORIENTED_EDGE ( 'NONE', *, *, #201026, .F. ) ;
#190980=CARTESIAN_POINT ( 'NONE',  ( 3.230585741806197841, 6.991043475407723307, 0.7998128361456271485 ) ) ;
#190983=CARTESIAN_POINT ( 'NONE',  ( 4.543390873910894356, 8.314723429622471684, 0.7216878364870317197 ) ) ;
#190984=CARTESIAN_POINT ( 'NONE',  ( 0.02041557226162492300, 2.519999999999982698, -2.000000000000004885 ) ) ;
#190997=CARTESIAN_POINT ( 'NONE',  ( -5.418418667316934112, 6.350518529071726981, -1.199719254218453823 ) ) ;
#190998=CARTESIAN_POINT ( 'NONE',  ( 5.858531774880875176, 9.849054480754103835, -0.7216878364870458196 ) ) ;
#191010=CARTESIAN_POINT ( 'NONE',  ( -6.622231685632140596, 6.690634819517756959, 0.000000000000000000 ) ) ;
#191011=CARTESIAN_POINT ( 'NONE',  ( -3.800028193580205382, 7.655393002477360653, -0.7998128361456481317 ) ) ;
#191027=CARTESIAN_POINT ( 'NONE',  ( -6.087706144486034532, 7.033779493390481363, -0.9955609822858858537 ) ) ;
#191032=CARTESIAN_POINT ( 'NONE',  ( 4.990809943606266508, 6.915973915664348937, -1.443375672974068769 ) ) ;
#191036=CARTESIAN_POINT ( 'NONE',  ( -5.447343857640614573, 9.577261277214532242, -0.7998128361456362523 ) ) ;
#191038=CIRCLE ( 'NONE', #97703, 0.08000000000000020983 ) ;
#191051=CARTESIAN_POINT ( 'NONE',  ( 4.518610335104485287, 8.493738834255713854, 0.000000000000000000 ) ) ;
#191064=TOROIDAL_SURFACE ( 'NONE', #21588, 0.8299999999999999600, 0.08000000000000000167 ) ;
#191067=CARTESIAN_POINT ( 'NONE',  ( 2.970157261343746136, 6.585292010301047938, 0.4235207732182846851 ) ) ;
#191085=CARTESIAN_POINT ( 'NONE',  ( 6.536439455564155843, 8.719208346281938304, 1.443375672974065660 ) ) ;
#191090=CARTESIAN_POINT ( 'NONE',  ( 6.441532379824158383, 9.568852638886589546, -1.082531754730548412 ) ) ;
#191116=CARTESIAN_POINT ( 'NONE',  ( -3.657667580636712934, 7.489305620709952649, -0.7998128361456481317 ) ) ;
#191118=CARTESIAN_POINT ( 'NONE',  ( 6.007671464186834065, 7.141943142040370063, 1.082531754730549967 ) ) ;
#191123=CARTESIAN_POINT ( 'NONE',  ( -5.306037014901836990, 7.283738832175834510, 1.599625672291263179 ) ) ;
#191128=CARTESIAN_POINT ( 'NONE',  ( -3.471769853551161411, 6.208092708188416076, 1.199719254218452935 ) ) ;
#191137=CARTESIAN_POINT ( 'NONE',  ( -4.878955176071358757, 6.785476686873604280, -1.599625672291271394 ) ) ;
#191146=CARTESIAN_POINT ( 'NONE',  ( -5.984998465789844069, 5.947196063035064206, 0.7998128361456281477 ) ) ;
#191149=CARTESIAN_POINT ( 'NONE',  ( -4.828112100242283766, 7.686528979374367410, -1.082531754730549967 ) ) ;
#191150=B_SPLINE_CURVE_WITH_KNOTS ( 'NONE', 3,
 ( #139583, #122340, #73483, #189371, #188297, #4191, #70261, #205610 ),
 .UNSPECIFIED., .F., .F.,
 ( 4, 2, 2, 4 ),
 ( 0.000000000000000000, 0.0001912162707998985305, 0.0003824325415997970610, 0.0007648650831995943387 ),
 .UNSPECIFIED. ) ;
#191151=CARTESIAN_POINT ( 'NONE',  ( -4.787437638956920871, 8.599444655509458357, -0.7216878364870338292 ) ) ;
#191152=CARTESIAN_POINT ( 'NONE',  ( 5.550083779947807550, 7.568460058062819407, -1.599625672291283607 ) ) ;
#191154=CARTESIAN_POINT ( 'NONE',  ( -5.387385936583832802, 7.378645907471495846, -1.599625672291271394 ) ) ;
#191162=ORIENTED_EDGE ( 'NONE', *, *, #22105, .T. ) ;
#191172=CARTESIAN_POINT ( 'NONE',  ( 6.230854113932139171, 9.427024345299638952, 1.199719254218452047 ) ) ;
#191191=CARTESIAN_POINT ( 'NONE',  ( 4.780342502845265074, 8.269896785439653897, -0.8296954209953393278 ) ) ;
#191207=EDGE_CURVE ( 'NONE', #212524, #96867, #19098, .T. ) ;
#191210=CARTESIAN_POINT ( 'NONE',  ( 6.282224075085741433, 8.422623735723785643, 1.599625672291268286 ) ) ;
#191213=CARTESIAN_POINT ( 'NONE',  ( -4.679499295372141709, 5.488445928469455559, 1.199719254218452935 ) ) ;
#191216=CARTESIAN_POINT ( 'NONE',  ( -7.241463443030476732, 7.620997903056574430, 0.000000000000000000 ) ) ;
#191227=CARTESIAN_POINT ( 'NONE',  ( 4.248501033035879004, 6.049946853332221153, -1.599625672291273171 ) ) ;
#191228=CARTESIAN_POINT ( 'NONE',  ( 5.692444392891300886, 7.734547439830227411, -1.599625672291281386 ) ) ;
#191240=ORIENTED_EDGE ( 'NONE', *, *, #200733, .T. ) ;
#191241=CARTESIAN_POINT ( 'NONE',  ( 4.386945222473598527, 7.275797305264619652, -1.199719254218452047 ) ) ;
#191250=CARTESIAN_POINT ( 'NONE',  ( 5.234856708652215751, 9.121433570154021453, 0.7216878364870317197 ) ) ;
#191251=CARTESIAN_POINT ( 'NONE',  ( -6.319508997745553636, 6.545384383557486530, 0.7216878364870257245 ) ) ;
#191252=CARTESIAN_POINT ( 'NONE',  ( -6.343235766347277149, 8.493804042195527870, -1.599625672291271394 ) ) ;
#191263=CARTESIAN_POINT ( 'NONE',  ( 6.229045230835819069, 6.231917288922055320, -0.7998128361456481317 ) ) ;
#191264=CARTESIAN_POINT ( 'NONE',  ( 6.038177310039780643, 8.137902509836795417, -1.599625672291283607 ) ) ;
#191267=CARTESIAN_POINT ( 'NONE',  ( 3.079110283634975964, 6.606396074300548982, 0.7216878364870257245 ) ) ;
#191270=ORIENTED_EDGE ( 'NONE', *, *, #34539, .F. ) ;
#191272=CYLINDRICAL_SURFACE ( 'NONE', #26709, 1.250000000000000000 ) ;
#191283=ORIENTED_EDGE ( 'NONE', *, *, #47045, .T. ) ;
#191284=ORIENTED_EDGE ( 'NONE', *, *, #212227, .F. ) ;
#191288=CARTESIAN_POINT ( 'NONE',  ( 3.874598038455354665, 7.742391154831717692, -0.7998128361456362523 ) ) ;
#191290=EDGE_CURVE ( 'NONE', #184155, #93276, #137295, .T. ) ;
#191293=CARTESIAN_POINT ( 'NONE',  ( 4.050854035433010480, 7.948023151305657841, 0.000000000000000000 ) ) ;
#191297=CARTESIAN_POINT ( 'NONE',  ( 7.343676480457483002, 8.596652644402405841, -1.199719254218452047 ) ) ;
#191298=CARTESIAN_POINT ( 'NONE',  ( 5.411747445213322294, 6.143583536729159356, -0.9474050467834894684 ) ) ;
#191302=CARTESIAN_POINT ( 'NONE',  ( 6.875393295905841917, 7.193916064744513506, 0.000000000000000000 ) ) ;
#191304=CARTESIAN_POINT ( 'NONE',  ( -6.306477729012051725, 7.386587434382707151, 1.199719254218452047 ) ) ;
#191305=CARTESIAN_POINT ( 'NONE',  ( 5.551137550152489553, 5.441024994791534120, 0.7998128361456352531 ) ) ;
#191312=CARTESIAN_POINT ( 'NONE',  ( -5.826172809686546827, 6.253349265757417008, -0.6540019011737445709 ) ) ;
#191315=CARTESIAN_POINT ( 'NONE',  ( -5.041653019435350380, 6.975290837464928728, -1.599625672291271394 ) ) ;
#191351=CARTESIAN_POINT ( 'NONE',  ( -5.064290697676250730, 7.960144884870772763, -1.236948567437242907 ) ) ;
#191352=CARTESIAN_POINT ( 'NONE',  ( 4.462041952228939401, 6.299077925724123617, -1.443375672974068769 ) ) ;
#191363=CARTESIAN_POINT ( 'NONE',  ( -5.978219388983010418, 5.939287140093762574, -0.7998128361456362523 ) ) ;
#191365=CARTESIAN_POINT ( 'NONE',  ( -4.925354943514475003, 8.968274210734028529, 0.000000000000000000 ) ) ;
#191367=CARTESIAN_POINT ( 'NONE',  ( 7.987161891782087686, 8.490979426600148372, -0.7216878364870317197 ) ) ;
#191369=CARTESIAN_POINT ( 'NONE',  ( -3.809009402267528710, 7.350678696556900427, -0.7255371203442788630 ) ) ;
#191377=CARTESIAN_POINT ( 'NONE',  ( -4.176793841461789114, 7.030620694084159794, -1.199719254218455378 ) ) ;
#191384=CARTESIAN_POINT ( 'NONE',  ( -5.966997003790240228, 6.134120390609613338, -0.7216878364870338292 ) ) ;
#191388=CARTESIAN_POINT ( 'NONE',  ( -3.623772196602547346, 7.449761006003425834, 0.000000000000000000 ) ) ;
#191391=UNCERTAINTY_MEASURE_WITH_UNIT (LENGTH_MEASURE( 1.000000000000000082E-05 ), #163404, 'distance_accuracy_value', 'NONE');
#191410=CARTESIAN_POINT ( 'NONE',  ( -7.469616286486262524, 7.679250187180907794, 0.7998128361456341429 ) ) ;
#191413=CARTESIAN_POINT ( 'NONE',  ( -4.118644803501354978, 8.027112380718707030, 0.7998128361456352531 ) ) ;
#191439=CARTESIAN_POINT ( 'NONE',  ( -5.444481204339554736, 8.509589284108232121, 1.199719254218454489 ) ) ;
#191449=CARTESIAN_POINT ( 'NONE',  ( 0.000000000000000000, 5.939655416065874327, 0.000000000000000000 ) ) ;
#191465=CARTESIAN_POINT ( 'NONE',  ( 7.014364370223726830, 9.276787413384745662, -1.599625672291269396 ) ) ;
#191467=CARTESIAN_POINT ( 'NONE',  ( 5.643937085038755797, 9.806620042512378177, -0.7998128361456481317 ) ) ;
#191480=CARTESIAN_POINT ( 'NONE',  ( 5.448178351099921102, 7.506598249424609293, 1.250114376932524252 ) ) ;
#191482=CARTESIAN_POINT ( 'NONE',  ( 7.688882512725796481, 8.142986817701137525, 0.000000000000000000 ) ) ;
#191488=CARTESIAN_POINT ( 'NONE',  ( -4.339491684825780737, 7.220434844675483355, -1.199719254218455378 ) ) ;
#191491=ORIENTED_EDGE ( 'NONE', *, *, #185383, .F. ) ;
#191498=CARTESIAN_POINT ( 'NONE',  ( -6.251718229232856139, 8.387033582228697881, -1.443375672974066548 ) ) ;
#191502=CARTESIAN_POINT ( 'NONE',  ( 7.343676480457483002, 8.596652644402405841, -1.199719254218452047 ) ) ;
#191517=CARTESIAN_POINT ( 'NONE',  ( 6.994027139803230320, 9.253060644560830994, -1.599625672291267398 ) ) ;
#191523=FACE_OUTER_BOUND ( 'NONE', #172118, .T. ) ;
#191536=CARTESIAN_POINT ( 'NONE',  ( -5.966470118465691641, 9.118576350588734059, -1.199719254218452047 ) ) ;
#191539=CARTESIAN_POINT ( 'NONE',  ( 4.830447868218803897, 8.857549289555754157, -0.7998128361456481317 ) ) ;
#191558=CARTESIAN_POINT ( 'NONE',  ( 4.990809943606266508, 6.915973915664348937, -1.443375672974068769 ) ) ;
#191569=CARTESIAN_POINT ( 'NONE',  ( -4.936577329151611515, 7.813071746435248599, 1.082531754730549967 ) ) ;
#191601=CARTESIAN_POINT ( 'NONE',  ( 4.878955176071345434, 6.785476686873604280, -1.599625672291269396 ) ) ;
#191612=CARTESIAN_POINT ( 'NONE',  ( -6.536439455564198475, 8.719208346281938304, 1.443375672974064550 ) ) ;
#191614=CARTESIAN_POINT ( 'NONE',  ( 4.868786560638896255, 5.813244087901094481, 1.082531754730549078 ) ) ;
#191622=DIRECTION ( 'NONE',  ( 0.000000000000000000, 0.000000000000000000, -1.000000000000000000 ) ) ;
#191631=CARTESIAN_POINT ( 'NONE',  ( -3.472296738875691346, 6.104744391113324120, 1.082531754730549967 ) ) ;
#191656=CARTESIAN_POINT ( 'NONE',  ( 5.577698110520374897, 5.843467644431432184, -0.7819401572049750060 ) ) ;
#191662=CARTESIAN_POINT ( 'NONE',  ( -6.607619761813764647, 8.802252036906432764, 1.599625672291269396 ) ) ;
#191665=CARTESIAN_POINT ( 'NONE',  ( -6.635789839245807897, 6.706452665400368218, 0.7998128361456341429 ) ) ;
#191666=CARTESIAN_POINT ( 'NONE',  ( -6.493429226302317225, 6.540365283632955773, 0.7998128361456341429 ) ) ;
#191670=B_SPLINE_CURVE_WITH_KNOTS ( 'NONE', 3,
 ( #162228, #49525, #112465, #212008, #127681, #32214, #129805, #163288, #143884, #96177, #196843, #131888, #164349, #47422, #62571, #64704, #181643, #31162, #113536, #194708, #114600, #45283, #177407, #78817, #165405, #180591 ),
 .UNSPECIFIED., .F., .F.,
 ( 4, 2, 2, 2, 2, 2, 2, 2, 2, 2, 1, 1, 2, 4 ),
 ( 0.1391494940249573542, 0.1534303038895106774, 0.1677111137540640007, 0.1819919236186173239, 0.1962727334831706472, 0.2105535433477239704, 0.2248343532122772659, 0.2391151630768305891, 0.2462555680091072507, 0.2498257704752456232, 0.2516108717083147539, 0.2525034223248493470, 0.2529496976331166436, 0.2533959729413839401 ),
 .UNSPECIFIED. ) ;
#191671=CARTESIAN_POINT ( 'NONE',  ( -5.424670858799220063, 9.342883411992149334, 0.000000000000000000 ) ) ;
#191673=CARTESIAN_POINT ( 'NONE',  ( 6.143253000323500856, 10.18122924377050609, -0.7216878364870458196 ) ) ;
#191675=CARTESIAN_POINT ( 'NONE',  ( -4.004454267989906668, 5.765225627445230927, 1.599625672291270506 ) ) ;
#191679=CARTESIAN_POINT ( 'NONE',  ( -3.644109427023046521, 7.473487774827342278, 0.000000000000000000 ) ) ;
#191693=CARTESIAN_POINT ( 'NONE',  ( 4.386945222473598527, 7.275797305264619652, -1.199719254218452047 ) ) ;
#191718=CARTESIAN_POINT ( 'NONE',  ( 6.527324610336440180, 6.579909898339485252, 0.7998128361456331437 ) ) ;
#191719=CARTESIAN_POINT ( 'NONE',  ( 3.250922972226694352, 7.014770244231638863, 0.7998128361456281477 ) ) ;
#191734=CARTESIAN_POINT ( 'NONE',  ( 6.177100234330334061, 7.056796855232915888, 1.058592334412721936 ) ) ;
#191735=CARTESIAN_POINT ( 'NONE',  ( -4.706088717274938382, 6.583799151611112954, 1.443375672974058777 ) ) ;
#191736=CARTESIAN_POINT ( 'NONE',  ( 3.445180431648323882, 6.073108699348104267, 1.082531754730549078 ) ) ;
#191749=ORIENTED_EDGE ( 'NONE', *, *, #71027, .F. ) ;
#191766=CARTESIAN_POINT ( 'NONE',  ( 3.542423274920540432, 7.354853930707762721, -1.734723475976807094E-15 ) ) ;
#191784=CARTESIAN_POINT ( 'NONE',  ( -5.794130544993808307, 7.853181283949808744, 1.599625672291263179 ) ) ;
#191786=ORIENTED_EDGE ( 'NONE', *, *, #7268, .F. ) ;
#191787=CARTESIAN_POINT ( 'NONE',  ( 1.806654366501771136, 9.001999999999998892, 2.419999999999998597 ) ) ;
#191790=CARTESIAN_POINT ( 'NONE',  ( -4.448483798615272100, 8.203998508444197313, 0.000000000000000000 ) ) ;
#191796=CARTESIAN_POINT ( 'NONE',  ( 4.899292406491845497, 6.809203455697518947, -1.599625672291273171 ) ) ;
#191806=CARTESIAN_POINT ( 'NONE',  ( 5.732961426666957294, 7.278201736375829789, 1.206439608388230500 ) ) ;
#191829=CARTESIAN_POINT ( 'NONE',  ( -5.926849427829407269, 6.943687749669614995, -1.199719254218453823 ) ) ;
#191831=CARTESIAN_POINT ( 'NONE',  ( 5.734172623936983904, 5.654565914206774124, 0.7998128361456352531 ) ) ;
#191835=CARTESIAN_POINT ( 'NONE',  ( -8.072954122294394352, 8.383144328957069291, -0.7998128361456362523 ) ) ;
#191838=DIRECTION ( 'NONE',  ( -0.3281536732072464768, 0.000000000000000000, -0.9446243521954066358 ) ) ;
#191843=CARTESIAN_POINT ( 'NONE',  ( -5.628650723579520232, 7.468463085569896798, -1.343613510788654875 ) ) ;
#191861=CARTESIAN_POINT ( 'NONE',  ( 6.061904079085887354, 6.244845311787889486, 0.000000000000000000 ) ) ;
#191864=CARTESIAN_POINT ( 'NONE',  ( -6.400331034103001748, 9.624747418832267698, 1.199719254218452935 ) ) ;
#191880=CARTESIAN_POINT ( 'NONE',  ( 4.980641328173811999, 6.904110530993182948, 1.599625672291269396 ) ) ;
#191894=ORIENTED_EDGE ( 'NONE', *, *, #8784, .F. ) ;
#191915=VERTEX_POINT ( 'NONE', #160997 ) ;
#191918=CARTESIAN_POINT ( 'NONE',  ( 6.142902043169038429, 7.013529245237516641, 0.9864344219776898237 ) ) ;
#191926=CARTESIAN_POINT ( 'NONE',  ( -5.139949632912262700, 5.169231791251960750, 0.7216878364870257245 ) ) ;
#191932=CARTESIAN_POINT ( 'NONE',  ( -3.461074353238556167, 7.259946855412102273, 0.000000000000000000 ) ) ;
#191940=CARTESIAN_POINT ( 'NONE',  ( -6.140917232347002042, 6.129101290685087911, -0.7998128361456362523 ) ) ;
#191942=CARTESIAN_POINT ( 'NONE',  ( 5.646014316602349759, 7.456765758048159221, -1.329534273556526758 ) ) ;
#191946=CARTESIAN_POINT ( 'NONE',  ( 5.180097208873055692, 8.201141289397330780, -1.199719254218450271 ) ) ;
#191952=CARTESIAN_POINT ( 'NONE',  ( -6.291865805193673111, 9.498204651771386509, -1.199719254218452047 ) ) ;
#191958=CARTESIAN_POINT ( 'NONE',  ( -4.716257332707368910, 6.595662536282280719, -1.599625672291271394 ) ) ;
#191964=CARTESIAN_POINT ( 'NONE',  ( 6.061904078641523697, 7.205214525570814210, -1.082531754730548412 ) ) ;
#191965=CARTESIAN_POINT ( 'NONE',  ( -5.763624699140874164, 8.777960344756069233, -1.082531754730549967 ) ) ;
#191972=CARTESIAN_POINT ( 'NONE',  ( 4.553559489343365740, 6.405848385690952718, -1.599625672291269396 ) ) ;
#191980=CARTESIAN_POINT ( 'NONE',  ( 4.746236293235721604, 7.694970221153795364, 1.199719254218451159 ) ) ;
#192002=CARTESIAN_POINT ( 'NONE',  ( 4.716601407767927689, 8.224641112169805979, 0.6639617910879731522 ) ) ;
#192012=CARTESIAN_POINT ( 'NONE',  ( 6.801350335910821165, 7.963938809097990124, 1.199719254218452047 ) ) ;
#192017=CARTESIAN_POINT ( 'NONE',  ( -4.610539993796915148, 8.375707290415371986, 0.1689211187793551172 ) ) ;
#192024=CARTESIAN_POINT ( 'NONE',  ( -5.284646014276622950, 9.387447126623207794, -0.7998128361456362523 ) ) ;
#192030=CARTESIAN_POINT ( 'NONE',  ( -4.733481511527885210, 4.890303307122107590, -0.5491554243041256722 ) ) ;
#192036=CARTESIAN_POINT ( 'NONE',  ( 7.361151057576892143, 7.552707420120024828, 0.7998128361456291469 ) ) ;
#192045=CARTESIAN_POINT ( 'NONE',  ( 3.390420931869152721, 6.113185632892752075, -1.199719254218452047 ) ) ;
#192048=CARTESIAN_POINT ( 'NONE',  ( 5.858531774436539052, 6.007577623030311287, 0.000000000000000000 ) ) ;
#192049=CARTESIAN_POINT ( 'NONE',  ( 0.04091653908484670782, 2.521406394469414725, -1.999686568719554192 ) ) ;
#192057=CARTESIAN_POINT ( 'NONE',  ( -6.325812300595961446, 6.871976577178664058, 0.6903976412777796945 ) ) ;
#192063=CARTESIAN_POINT ( 'NONE',  ( -4.767627293860968507, 5.591261926706423857, -1.199719254218453823 ) ) ;
#192064=CARTESIAN_POINT ( 'NONE',  ( 7.526184669361807522, 7.953172667109813077, 0.000000000000000000 ) ) ;
#192076=CARTESIAN_POINT ( 'NONE',  ( -7.123883369337781879, 7.275895117174344229, 0.7998128361456341429 ) ) ;
#192077=CARTESIAN_POINT ( 'NONE',  ( -3.935609729716867289, 7.813571461303467913, 0.7998128361456352531 ) ) ;
#192079=CARTESIAN_POINT ( 'NONE',  ( 5.817857313595521163, 9.801600942587855414, -0.7216878364870458196 ) ) ;
#192085=DIRECTION ( 'NONE',  ( 0.000000000000000000, 1.496258514059622730E-16, -1.000000000000000000 ) ) ;
#192090=CARTESIAN_POINT ( 'NONE',  ( -6.290641498436300161, 6.895329709839009169, -0.7498213622291228786 ) ) ;
#192095=CARTESIAN_POINT ( 'NONE',  ( 4.258669648468268676, 7.982548666606070320, 0.7216878364870257245 ) ) ;
#192101=CARTESIAN_POINT ( 'NONE',  ( -6.095272577795516789, 9.268845886473535245, 1.199719254218452047 ) ) ;
#192105=( BOUNDED_SURFACE ( )  B_SPLINE_SURFACE ( 3, 2, ( 
 ( #131456, #167112, #115218 ),
 ( #49098, #32836, #99970 ),
 ( #168169, #199579, #50154 ),
 ( #181208, #166035, #200639 ),
 ( #65307, #51223, #184401 ),
 ( #148724, #31785, #36021 ) ),
 .UNSPECIFIED., .F., .F., .T. ) 
 B_SPLINE_SURFACE_WITH_KNOTS ( ( 4, 2, 4 ),
 ( 3, 3 ),
 ( -6.938893903907228378E-18, 0.002403677751102540304, 0.004807355502205087547 ),
 ( 0.000000000000000000, 1.000000000000000000 ),
 .UNSPECIFIED. ) 
 GEOMETRIC_REPRESENTATION_ITEM ( )  RATIONAL_B_SPLINE_SURFACE ( (
 ( 1.000000000000000000, 0.7789607113619948509, 1.000000000000000000),
 ( 1.000000000000000000, 0.7844575505954650696, 1.000000000000000000),
 ( 1.000000000000000000, 0.7910273759756671907, 1.000000000000000000),
 ( 1.000000000000000000, 0.8087931444444149687, 1.000000000000000000),
 ( 1.000000000000000000, 0.8199986536752983390, 1.000000000000000000),
 ( 1.000000000000000000, 0.8356624583022056463, 1.000000000000000000) ) ) 
 REPRESENTATION_ITEM ( '' )  SURFACE ( )  );
#192118=CARTESIAN_POINT ( 'NONE',  ( 6.475954649182838807, 7.584310507915338562, 1.199719254218452047 ) ) ;
#192136=CARTESIAN_POINT ( 'NONE',  ( -3.824766175154623582, 7.348582304423016964, -0.7466790275774716212 ) ) ;
#192152=CARTESIAN_POINT ( 'NONE',  ( 5.709392085130549077, 9.675058176045386205, 0.000000000000000000 ) ) ;
#192183=CARTESIAN_POINT ( 'NONE',  ( -5.978219388983010418, 5.939287140093762574, -0.7998128361456362523 ) ) ;
#192185=CARTESIAN_POINT ( 'NONE',  ( 6.495764994278809823, 6.751016379513001375, 0.7216878364870328300 ) ) ;
#192190=CARTESIAN_POINT ( 'NONE',  ( -4.305596300791617814, 7.180890229968955651, 1.199719254218452935 ) ) ;
#192194=CARTESIAN_POINT ( 'NONE',  ( 3.719872605471106208, 6.605953636083950364, 7.500000000000000000 ) ) ;
#192195=CARTESIAN_POINT ( 'NONE',  ( -3.298376509874564988, 7.070132704820777825, 0.000000000000000000 ) ) ;
#192197=( BOUNDED_CURVE ( )  B_SPLINE_CURVE ( 2, ( #27966, #7432, #9579, #177421, #15949, #29039, #148126 ),
 .UNSPECIFIED., .F., .T. ) 
 B_SPLINE_CURVE_WITH_KNOTS ( ( 3, 2, 2, 3 ),
 ( 0.5146539602424855531, 0.5166666666666667185, 0.5250000000000000222, 0.5292933853275720857 ),
 .UNSPECIFIED. ) 
 CURVE ( )  GEOMETRIC_REPRESENTATION_ITEM ( )  RATIONAL_B_SPLINE_CURVE ( ( 0.9509142384741717802, 0.9676418163423837759, 1.000000000000000000, 0.8660254037844387076, 1.000000000000000000, 0.9309754521208858380, 0.9330746597073281690 ) ) 
 REPRESENTATION_ITEM ( '' )  );
#192203=CARTESIAN_POINT ( 'NONE',  ( -5.204350862799341115, 7.165104988056252289, -1.599625672291271394 ) ) ;
#192212=CARTESIAN_POINT ( 'NONE',  ( -5.822300622425855110, 5.757381912443740646, 0.7998128361456281477 ) ) ;
#192216=CARTESIAN_POINT ( 'NONE',  ( -5.804299160426237059, 7.865044668620976509, -1.443375672974066548 ) ) ;
#192217=CARTESIAN_POINT ( 'NONE',  ( -4.936577328707246082, 8.773440960218172435, 0.000000000000000000 ) ) ;
#192218=CARTESIAN_POINT ( 'NONE',  ( 5.794130544993763898, 7.853181283949808744, 1.599625672291269396 ) ) ;
#192219=CARTESIAN_POINT ( 'NONE',  ( -5.257529707049291900, 9.355811434857983500, 0.7998128361456291469 ) ) ;
#192227=ORIENTED_EDGE ( 'NONE', *, *, #30501, .T. ) ;
#192238=CARTESIAN_POINT ( 'NONE',  ( 7.635176783151273128, 8.936736330878529699, 1.199719254218452935 ) ) ;
#192244=LINE ( 'NONE', #77444, #11392 ) ;
#192256=CARTESIAN_POINT ( 'NONE',  ( 4.684384365712907616, 8.380862967975740929, 0.5977175665230231028 ) ) ;
#192271=CARTESIAN_POINT ( 'NONE',  ( 5.688527969385528849, 8.794310509995222347, -1.199719254218452047 ) ) ;
#192277=CARTESIAN_POINT ( 'NONE',  ( -6.197485614778184271, 9.284131412999601096, 1.082531754730549967 ) ) ;
#192289=CARTESIAN_POINT ( 'NONE',  ( 6.831329296439236032, 9.063246493969506545, -1.599625672291267398 ) ) ;
#192290=CARTESIAN_POINT ( 'NONE',  ( 5.367048706163317640, 7.354919138647580290, -1.599625672291281386 ) ) ;
#192305=CARTESIAN_POINT ( 'NONE',  ( 7.225569521440261767, 7.394528961293920233, -0.7998128361456341429 ) ) ;
#192309=VECTOR ( 'NONE', #168937, 1000.000000000000000 ) ;
#192318=CARTESIAN_POINT ( 'NONE',  ( -4.150204419558982671, 7.856005899545188242, 0.7216878364870338292 ) ) ;
#192319=CARTESIAN_POINT ( 'NONE',  ( -6.912678218121246942, 9.158153569265168770, 1.599625672291269396 ) ) ;
#192331=CARTESIAN_POINT ( 'NONE',  ( 5.773793314573267388, 7.829454515125894964, 1.599625672291268286 ) ) ;
#192332=CARTESIAN_POINT ( 'NONE',  ( 7.388267364804250725, 7.584343111885245570, -0.7998128361456341429 ) ) ;
#192335=CARTESIAN_POINT ( 'NONE',  ( 5.194182247366881278, 5.232503174782402233, 0.7216878364870328300 ) ) ;
#192354=CARTESIAN_POINT ( 'NONE',  ( 3.386504508363381571, 7.172948703057747011, -0.7998128361456362523 ) ) ;
#192356=CARTESIAN_POINT ( 'NONE',  ( -3.383641855062333281, 6.105276709951447778, -1.199719254218452047 ) ) ;
#192358=CARTESIAN_POINT ( 'NONE',  ( 5.468734858265785093, 7.473552982767158070, 1.599625672291269396 ) ) ;
#192367=B_SPLINE_CURVE_WITH_KNOTS ( 'NONE', 3,
 ( #205937, #159327, #22900, #10924, #76999, #173476, #58632, #155069, #124785, #190745, #158280, #9870, #6658, #28264 ),
 .UNSPECIFIED., .F., .F.,
 ( 4, 2, 2, 2, 2, 2, 4 ),
 ( 0.5000508295171147699, 0.5622958969969490406, 0.6245409644767833113, 0.6556634982167006687, 0.6867860319566181371, 0.7179085656965356055, 0.7490310994364531849 ),
 .UNSPECIFIED. ) ;
#192370=CARTESIAN_POINT ( 'NONE',  ( 7.512626515748113576, 7.937354821227203594, 0.7216878364870267237 ) ) ;
#192372=CARTESIAN_POINT ( 'NONE',  ( -6.607619761813764647, 8.802252036906432764, 1.599625672291269396 ) ) ;
#192373=CARTESIAN_POINT ( 'NONE',  ( 6.052789233858158369, 6.026285292448116948, 0.000000000000000000 ) ) ;
#192385=CARTESIAN_POINT ( 'NONE',  ( -5.646044625448194410, 5.551749915969804938, 0.000000000000000000 ) ) ;
#192410=CIRCLE ( 'NONE', #92117, 0.7500000000000011102 ) ;
#192413=CARTESIAN_POINT ( 'NONE',  ( 3.445180431648323882, 6.073108699348104267, 1.082531754730549078 ) ) ;
#192420=CARTESIAN_POINT ( 'NONE',  ( 6.556249800660121529, 9.806652646482286073, 1.199719254218452047 ) ) ;
#192430=CARTESIAN_POINT ( 'NONE',  ( -4.899292406491858820, 6.809203455697518947, -1.599625672291271394 ) ) ;
#192432=CARTESIAN_POINT ( 'NONE',  ( -4.613517410400161722, 8.604463755433990002, -0.7998128361456362523 ) ) ;
#192434=CARTESIAN_POINT ( 'NONE',  ( 6.143253000323500856, 10.18122924377050609, -0.7216878364870458196 ) ) ;
#192445=CARTESIAN_POINT ( 'NONE',  ( -4.990283058281743678, 7.979691447040783814, -1.199719254218453823 ) ) ;
#192452=CARTESIAN_POINT ( 'NONE',  ( -6.143253000767895600, 6.339752387083549934, 0.000000000000000000 ) ) ;
#192456=CARTESIAN_POINT ( 'NONE',  ( -6.147696309153835692, 6.137010213626392208, 0.7998128361456281477 ) ) ;
#192466=AXIS2_PLACEMENT_3D ( 'NONE', #121216, #6286, #73434 ) ;
#192476=ORIENTED_EDGE ( 'NONE', *, *, #145827, .F. ) ;
#192478=CARTESIAN_POINT ( 'NONE',  ( -5.447343857640614573, 9.577261277214532242, -0.7998128361456362523 ) ) ;
#192480=CARTESIAN_POINT ( 'NONE',  ( -4.573896719763875574, 6.429575154514868274, -1.599625672291271394 ) ) ;
#192489=FACE_OUTER_BOUND ( 'NONE', #190624, .T. ) ;
#192492=ORIENTED_EDGE ( 'NONE', *, *, #122876, .F. ) ;
#192506=CARTESIAN_POINT ( 'NONE',  ( -7.930593509350902792, 8.217056947189661287, -0.7998128361456362523 ) ) ;
#192532=CARTESIAN_POINT ( 'NONE',  ( 7.018280793729500644, 8.217024343219755167, -1.199719254218452047 ) ) ;
#192542=CARTESIAN_POINT ( 'NONE',  ( 6.517945676554362855, 6.748686274690250286, -0.003863832781672048907 ) ) ;
#192546=CARTESIAN_POINT ( 'NONE',  ( 5.176795123377851304, 7.746134302493202561, 1.185296789734613387 ) ) ;
#192548=CARTESIAN_POINT ( 'NONE',  ( 6.156811154381533591, 9.236677875870187293, -1.082531754730548412 ) ) ;
#192554=CARTESIAN_POINT ( 'NONE',  ( -5.581116510680924847, 6.540332679663050541, -1.199719254218453823 ) ) ;
#192562=CARTESIAN_POINT ( 'NONE',  ( -4.950135482320914271, 8.789258806100786359, -0.7216878364870338292 ) ) ;
#192565=CARTESIAN_POINT ( 'NONE',  ( 5.643937085038755797, 9.806620042512378177, -0.7998128361456481317 ) ) ;
#192566=B_SPLINE_CURVE_WITH_KNOTS ( 'NONE', 3,
 ( #146314, #162551, #181963, #61838, #97557, #95438, #66060, #29343 ),
 .UNSPECIFIED., .F., .F.,
 ( 4, 2, 2, 4 ),
 ( 0.000000000000000000, 0.0006610868961727778791, 0.0009916303442591663849, 0.001322173792345555108 ),
 .UNSPECIFIED. ) ;
#192567=CARTESIAN_POINT ( 'NONE',  ( -5.683421429784462298, 6.045756166660654074, -0.6295853902834018800 ) ) ;
#192571=CARTESIAN_POINT ( 'NONE',  ( -2.972980823146582186, 6.690504403638126263, 0.000000000000000000 ) ) ;
#192581=CARTESIAN_POINT ( 'NONE',  ( 4.085803189671889157, 5.860132702740892263, -1.599625672291273171 ) ) ;
#192587=CARTESIAN_POINT ( 'NONE',  ( -5.398914348987512213, 6.259949555863199677, 2.420000000000001261 ) ) ;
#192601=CIRCLE ( 'NONE', #144291, 0.4000000000000001332 ) ;
#192604=CARTESIAN_POINT ( 'NONE',  ( 7.666209513884374438, 7.908608952478760834, 0.7998128361456281477 ) ) ;
#192612=CARTESIAN_POINT ( 'NONE',  ( 5.499767588998890844, 6.445425604367387429, 1.199719254218451159 ) ) ;
#192625=CARTESIAN_POINT ( 'NONE',  ( 6.699137298928158124, 6.988284068270579574, 0.7216878364870328300 ) ) ;
#192635=CARTESIAN_POINT ( 'NONE',  ( -4.828112100242283766, 7.686528979374367410, -1.082531754730549967 ) ) ;
#192646=CARTESIAN_POINT ( 'NONE',  ( -2.428612866367529932E-14, 2.999999999999999112, 7.500000000000000000 ) ) ;
#192656=CARTESIAN_POINT ( 'NONE',  ( -5.346851039111045978, 6.199209027673974859, 1.173132900504408438 ) ) ;
#192662=VERTEX_POINT ( 'NONE', #12905 ) ;
#192666=CARTESIAN_POINT ( 'NONE',  ( 4.041212305325117882, 6.872442235258051646, -1.199719254218448494 ) ) ;
#192678=CARTESIAN_POINT ( 'NONE',  ( -7.282137904315833410, 7.668451441222825515, 0.000000000000000000 ) ) ;
#192681=CARTESIAN_POINT ( 'NONE',  ( 4.136646265500957043, 5.919449624541475607, -1.443375672974068769 ) ) ;
#192698=CARTESIAN_POINT ( 'NONE',  ( -4.719646871332968452, 5.639247783710797712, 1.082531754730549078 ) ) ;
#192713=ORIENTED_EDGE ( 'NONE', *, *, #71694, .T. ) ;
#192730=CARTESIAN_POINT ( 'NONE',  ( -6.257970421159510188, 9.458660037064859694, 1.199719254218452047 ) ) ;
#192734=CARTESIAN_POINT ( 'NONE',  ( -5.196461137543813891, 7.842688287721260032, 1.273345793684066862 ) ) ;
#192735=CARTESIAN_POINT ( 'NONE',  ( -6.303615075710994553, 6.318915441276409695, -0.7998128361456361413 ) ) ;
#192736=CARTESIAN_POINT ( 'NONE',  ( -4.727634349329638219, 8.249773960229633829, 0.6920918352846835431 ) ) ;
#192745=CARTESIAN_POINT ( 'NONE',  ( -3.955946960137363799, 7.837298230127379917, 0.7998128361456352531 ) ) ;
#192759=CARTESIAN_POINT ( 'NONE',  ( 5.194709132691408549, 6.089524072008651423, 1.199719254218452935 ) ) ;
#192771=CARTESIAN_POINT ( 'NONE',  ( 5.078784331656527762, 4.889946239879535028, -0.1287282925451668503 ) ) ;
#192782=CARTESIAN_POINT ( 'NONE',  ( 3.867818961648523235, 7.734482231890414283, 1.040834085586084257E-14 ) ) ;
#192783=CARTESIAN_POINT ( 'NONE',  ( 5.747730777550676073, 5.670383760089384495, 0.000000000000000000 ) ) ;
#192785=CARTESIAN_POINT ( 'NONE',  ( 4.390861645979372341, 6.216034235099629157, -1.599625672291269396 ) ) ;
#192791=DIRECTION ( 'NONE',  ( 0.000000000000000000, 0.000000000000000000, -1.000000000000000000 ) ) ;
#192797=CARTESIAN_POINT ( 'NONE',  ( -2.974698719455045381, 6.690899969729074748, -0.05384663926280564006 ) ) ;
#192798=CARTESIAN_POINT ( 'NONE',  ( 4.797842130449009090, 8.250315290282747682, 0.8618622828703215166 ) ) ;
#192799=CARTESIAN_POINT ( 'NONE',  ( -3.648552735408985725, 7.270745601370182776, -0.7216878364870458196 ) ) ;
#192800=CARTESIAN_POINT ( 'NONE',  ( 3.933273961740298752, 5.682181936820735579, 1.443375672974058777 ) ) ;
#192829=CARTESIAN_POINT ( 'NONE',  ( 4.927462483923885195, 4.713404084191450849, -0.7998128361456481317 ) ) ;
#192847=CARTESIAN_POINT ( 'NONE',  ( -7.442499979258930587, 7.647614495415686164, -0.7998128361456362523 ) ) ;
#192865=CARTESIAN_POINT ( 'NONE',  ( 3.562760505341037831, 7.378580699531681830, -1.734723475976807094E-15 ) ) ;
#192873=CARTESIAN_POINT ( 'NONE',  ( -4.858757509019059562, 5.629766575900002401, 2.420000000000000373 ) ) ;
#192876=CARTESIAN_POINT ( 'NONE',  ( 5.960708871395055120, 7.108654626955757116, 1.090683939682752124 ) ) ;
#192889=ADVANCED_FACE ( 'NONE', ( #204977 ), #175692, .T. ) ;
#192890=CARTESIAN_POINT ( 'NONE',  ( -6.067740968097372622, 7.047743726685476773, 1.013785590662339642 ) ) ;
#192896=CARTESIAN_POINT ( 'NONE',  ( -4.471156797456668386, 8.438376373666578445, -0.7998128361456362523 ) ) ;
#192898=CARTESIAN_POINT ( 'NONE',  ( 5.896870467300973750, 5.844380064798101237, 0.7998128361456352531 ) ) ;
#192902=CARTESIAN_POINT ( 'NONE',  ( -6.831329296439251131, 9.063246493969506545, -1.599625672291271394 ) ) ;
#192905=CARTESIAN_POINT ( 'NONE',  ( 5.854088466050551887, 10.05179665369283981, 0.7998128361456341429 ) ) ;
#192906=CARTESIAN_POINT ( 'NONE',  ( 6.141001612134830978, 5.378507234883239896, -2.500000000000000000 ) ) ;
#192912=CARTESIAN_POINT ( 'NONE',  ( -5.143355005462953322, 7.892534720870457043, -1.245665949277234841 ) ) ;
#192930=CARTESIAN_POINT ( 'NONE',  ( 3.770576118376296471, 7.413106214832098750, 0.7216878364870257245 ) ) ;
#192939=ORIENTED_EDGE ( 'NONE', *, *, #131846, .T. ) ;
#192950=CARTESIAN_POINT ( 'NONE',  ( 5.747730777550676073, 5.670383760089384495, 0.000000000000000000 ) ) ;
#192954=DIRECTION ( 'NONE',  ( -0.7592566023653004592, -0.6507913734559639396, 0.000000000000000000 ) ) ;
#192966=CARTESIAN_POINT ( 'NONE',  ( 3.853570894305305305, 8.531289074211816370, 2.447542183238072155 ) ) ;
#192991=CARTESIAN_POINT ( 'NONE',  ( -5.662713974411738960, 5.571197489760607802, -0.2163730220445139740 ) ) ;
#193000=CARTESIAN_POINT ( 'NONE',  ( -4.543390873910949423, 6.393985001019784953, 1.443375672974058777 ) ) ;
#193007=CARTESIAN_POINT ( 'NONE',  ( -4.586401103172829785, 8.572828063668767484, 0.7998128361456281477 ) ) ;
#193018=CARTESIAN_POINT ( 'NONE',  ( -5.061990249855848667, 6.999017606288844284, -1.599625672291271394 ) ) ;
#193021=CARTESIAN_POINT ( 'NONE',  ( 6.598740849494261873, 6.770918179921630475, -0.1579934589533253664 ) ) ;
#193026=CARTESIAN_POINT ( 'NONE',  ( 4.854701522145073334, 7.821512988214679218, -1.199719254218450271 ) ) ;
#193031=CARTESIAN_POINT ( 'NONE',  ( -5.915100157312088491, 10.12297696016459092, -0.7998128361456362523 ) ) ;
#193038=CARTESIAN_POINT ( 'NONE',  ( -4.288121723672178476, 8.224835454251337552, -0.7998128361456362523 ) ) ;
#193042=CARTESIAN_POINT ( 'NONE',  ( 6.509323147892504657, 6.766834225395614411, 0.000000000000000000 ) ) ;
#193043=CARTESIAN_POINT ( 'NONE',  ( -5.383996397958228819, 8.335060660042973524, 1.082531754730550855 ) ) ;
#193051=CARTESIAN_POINT ( 'NONE',  ( 4.258142763143749399, 7.125527769379820242, 1.199719254218451159 ) ) ;
#193057=CARTESIAN_POINT ( 'NONE',  ( 6.364626766972446781, 6.390095747748158139, 0.7998128361456350310 ) ) ;
#193063=EDGE_CURVE ( 'NONE', #79244, #211530, #51065, .T. ) ;
#193069=CIRCLE ( 'NONE', #206816, 0.08000000000000034861 ) ;
#193084=CARTESIAN_POINT ( 'NONE',  ( 4.624009687016504166, 8.337032093926254106, -0.3390773965592456252 ) ) ;
#193093=CARTESIAN_POINT ( 'NONE',  ( 7.367930134383754215, 7.560616343061329125, -0.7998128361456341429 ) ) ;
#193098=CARTESIAN_POINT ( 'NONE',  ( -4.612386318492403880, 8.373339136000554461, 0.1892495524792922046 ) ) ;
#193105=CARTESIAN_POINT ( 'NONE',  ( -3.811250578772981346, 6.500190537660166079, -1.082531754730546636 ) ) ;
#193118=CARTESIAN_POINT ( 'NONE',  ( -5.113360211009450040, 5.994616996712990975, -1.199719254218453823 ) ) ;
#193120=CARTESIAN_POINT ( 'NONE',  ( 6.984385409695311964, 8.177479728513226576, 1.199719254218452935 ) ) ;
#193129=CARTESIAN_POINT ( 'NONE',  ( 3.379725431556547477, 7.165039780116438273, -1.734723475976807094E-15 ) ) ;
#193132=CARTESIAN_POINT ( 'NONE',  ( 4.516274566683592617, 8.283087737857252719, -0.7216878364870357165 ) ) ;
#193141=CARTESIAN_POINT ( 'NONE',  ( -6.027110718723775129, 7.076430883291389584, 1.047497865993127553 ) ) ;
#193147=CARTESIAN_POINT ( 'NONE',  ( -4.176793841461789114, 7.030620694084159794, -1.199719254218455378 ) ) ;
#193148=CARTESIAN_POINT ( 'NONE',  ( 7.512626515748109135, 8.897724035528543851, 1.082531754730549967 ) ) ;
#193160=CARTESIAN_POINT ( 'NONE',  ( -7.110325215724114578, 7.260077271291732082, 0.000000000000000000 ) ) ;
#193161=CARTESIAN_POINT ( 'NONE',  ( -5.285699784481336927, 7.260012063351913625, 1.599625672291263179 ) ) ;
#193163=CARTESIAN_POINT ( 'NONE',  ( 6.143253000323500856, 10.18122924377050609, -0.7216878364870458196 ) ) ;
#193168=CARTESIAN_POINT ( 'NONE',  ( 4.936577329151614180, 4.931964103531220722, -0.7216878364870458196 ) ) ;
#193175=CARTESIAN_POINT ( 'NONE',  ( -5.622963654236769138, 7.379252650573795869, -1.237363127855268141 ) ) ;
#193184=CARTESIAN_POINT ( 'NONE',  ( -7.795011973214244883, 8.058878488363559356, 0.7998128361456341429 ) ) ;
#193202=CARTESIAN_POINT ( 'NONE',  ( 7.191674137406095291, 7.354984346587396082, 0.000000000000000000 ) ) ;
#193238=CARTESIAN_POINT ( 'NONE',  ( 7.512626515748109135, 8.897724035528543851, 1.082531754730549967 ) ) ;
#193267=CARTESIAN_POINT ( 'NONE',  ( -4.142898457427624415, 6.991076079377632091, 1.199719254218452935 ) ) ;
#193269=CARTESIAN_POINT ( 'NONE',  ( 5.600926855776875435, 7.627776979863398310, -1.443375672974078761 ) ) ;
#193275=CARTESIAN_POINT ( 'NONE',  ( -4.457598643843001973, 8.422558527783969851, 0.000000000000000000 ) ) ;
#193280=CARTESIAN_POINT ( 'NONE',  ( -6.563555762791521531, 9.711213252348503744, 1.082531754730549967 ) ) ;
#193287=CARTESIAN_POINT ( 'NONE',  ( -6.296835998904160014, 6.311006518335105397, 0.000000000000000000 ) ) ;
#193297=CARTESIAN_POINT ( 'NONE',  ( -3.959863383643135393, 6.777535159962392086, 1.199719254218452935 ) ) ;
#193300=CARTESIAN_POINT ( 'NONE',  ( -4.665414256878287702, 8.457084043084382330, -0.7216878364870338292 ) ) ;
#193301=CARTESIAN_POINT ( 'NONE',  ( -6.766928066552171828, 7.067373297165212342, 0.7216878364870317197 ) ) ;
#193302=CARTESIAN_POINT ( 'NONE',  ( 6.658989722967328717, 7.797851427330578566, 1.199719254218452935 ) ) ;
#193303=CARTESIAN_POINT ( 'NONE',  ( -5.121948170912633991, 9.197632976031879792, -0.7998128361456362523 ) ) ;
#193341=CARTESIAN_POINT ( 'NONE',  ( 4.597299534708283453, 8.487268731053720927, 0.09294953129799360392 ) ) ;
#193356=CARTESIAN_POINT ( 'NONE',  ( 7.374709211190586089, 7.568525266002632534, 0.000000000000000000 ) ) ;
#193359=CARTESIAN_POINT ( 'NONE',  ( -3.817502770699643388, 6.611447778194983194, 1.199719254218452935 ) ) ;
#193363=CARTESIAN_POINT ( 'NONE',  ( -6.089020385868856522, 9.157588645938716354, -1.082531754730549967 ) ) ;
#193374=CARTESIAN_POINT ( 'NONE',  ( 7.452141709366786770, 8.723195411463290583, 1.199719254218452047 ) ) ;
#193375=CARTESIAN_POINT ( 'NONE',  ( 5.855142236255289845, 7.924361590421551860, -1.599625672291281386 ) ) ;
#193390=CARTESIAN_POINT ( 'NONE',  ( 5.040599249230596435, 9.102725900736217568, 0.7998128361456341429 ) ) ;
#193402=CARTESIAN_POINT ( 'NONE',  ( -2.862179826260718762, 6.353310540697199471, 0.000000000000000000 ) ) ;
#193405=CARTESIAN_POINT ( 'NONE',  ( -5.655159470675923394, 5.770309935309573923, 0.000000000000000000 ) ) ;
#193406=CARTESIAN_POINT ( 'NONE',  ( -5.887983850084758330, 10.09134126839936840, 0.7998128361456291469 ) ) ;
#193413=VERTEX_POINT ( 'NONE', #85691 ) ;
#193415=CARTESIAN_POINT ( 'NONE',  ( 5.736508391913541338, 6.825586224388162648, -1.082531754730548412 ) ) ;
#193420=CARTESIAN_POINT ( 'NONE',  ( 6.496291879603339758, 7.608037276739255006, 1.199719254218452935 ) ) ;
#193423=CARTESIAN_POINT ( 'NONE',  ( 4.895902867866261055, 4.884510565364971413, -0.7216878364870458196 ) ) ;
#193443=CARTESIAN_POINT ( 'NONE',  ( 5.845500506147374153, 6.848780674373954547, 1.199719254218453823 ) ) ;
#193448=CARTESIAN_POINT ( 'NONE',  ( 6.008198349511364000, 7.038594824965278995, 1.199719254218453823 ) ) ;
#193458=CARTESIAN_POINT ( 'NONE',  ( 6.861835142292135536, 9.098836647464588978, 1.443375672974065660 ) ) ;
#193460=CARTESIAN_POINT ( 'NONE',  ( -5.108390017298964914, 9.181815130149269422, 0.000000000000000000 ) ) ;
#193461=CARTESIAN_POINT ( 'NONE',  ( 4.366607992053101128, 7.252070536440704096, -1.199719254218448494 ) ) ;
#193471=CARTESIAN_POINT ( 'NONE',  ( -5.496904935697871863, 5.377753611261092637, 0.7998128361456281477 ) ) ;
#193485=( GEOMETRIC_REPRESENTATION_CONTEXT ( 3 ) GLOBAL_UNCERTAINTY_ASSIGNED_CONTEXT ( ( #191391 ) ) GLOBAL_UNIT_ASSIGNED_CONTEXT ( ( #163404, #145050, #203331 ) ) REPRESENTATION_CONTEXT ( 'NONE', 'WORKASPACE' ) );
#193500=CARTESIAN_POINT ( 'NONE',  ( 5.289089323106923146, 6.303597310780433283, -1.082531754730548412 ) ) ;
#193506=CARTESIAN_POINT ( 'NONE',  ( 4.868786560638889149, 6.773613302202437403, 1.443375672974065660 ) ) ;
#193517=CARTESIAN_POINT ( 'NONE',  ( -4.847922445338252118, 7.813604065273374921, -1.199719254218453823 ) ) ;
#193519=CARTESIAN_POINT ( 'NONE',  ( -7.045397100956844127, 8.248660034984974132, -1.199719254218452047 ) ) ;
#193521=CARTESIAN_POINT ( 'NONE',  ( 5.506019780481205217, 9.437790487287811558, 0.000000000000000000 ) ) ;
#193530=CARTESIAN_POINT ( 'NONE',  ( -5.152980901645737077, 8.169505597632108262, -1.199719254218453823 ) ) ;
#193537=CARTESIAN_POINT ( 'NONE',  ( -5.207740401424942434, 6.208690235484773723, 1.082531754730549078 ) ) ;
#193541=CARTESIAN_POINT ( 'NONE',  ( -4.960304097753355457, 6.880383762169266504, 1.599625672291263179 ) ) ;
#193560=CARTESIAN_POINT ( 'NONE',  ( -4.959250327548641479, 9.007818825440551791, -0.7998128361456362523 ) ) ;
#193562=CARTESIAN_POINT ( 'NONE',  ( -3.820365424000704557, 7.679119771301277098, -0.7998128361456481317 ) ) ;
#193563=ORIENTED_EDGE ( 'NONE', *, *, #136789, .F. ) ;
#193573=ORIENTED_EDGE ( 'NONE', *, *, #36816, .T. ) ;
#193585=CARTESIAN_POINT ( 'NONE',  ( -6.200875153403786477, 8.327716660428123419, -1.599625672291271394 ) ) ;
#193610=CARTESIAN_POINT ( 'NONE',  ( 7.095713291905693332, 9.371694488680407886, 1.599625672291268286 ) ) ;
#193612=CARTESIAN_POINT ( 'NONE',  ( 7.517069824134078537, 7.734612647770044092, 0.000000000000000000 ) ) ;
#193624=CARTESIAN_POINT ( 'NONE',  ( 5.701630405109389343, 7.302376724489803905, 1.216486997566777584 ) ) ;
#193626=CARTESIAN_POINT ( 'NONE',  ( 7.377044979611483200, 7.779176362401098999, -0.7216878364870317197 ) ) ;
#193631=CARTESIAN_POINT ( 'NONE',  ( -5.147255595043616516, 6.034161611419515125, 1.199719254218452935 ) ) ;
#193637=CARTESIAN_POINT ( 'NONE',  ( -7.092323753280154186, 7.447001598347859463, 0.7216878364870317197 ) ) ;
#193657=CARTESIAN_POINT ( 'NONE',  ( 7.856023664475727308, 8.130058794835305136, -0.7998128361456341429 ) ) ;
#193676=DIRECTION ( 'NONE',  ( 0.000000000000000000, 0.000000000000000000, -1.000000000000000000 ) ) ;
#193678=CARTESIAN_POINT ( 'NONE',  ( -3.650979853707545075, 7.481503272625923628, -0.4052952642843922204 ) ) ;
#193679=CARTESIAN_POINT ( 'NONE',  ( 6.638652492546827766, 7.774124658506663010, 1.199719254218452047 ) ) ;
#193681=CARTESIAN_POINT ( 'NONE',  ( -6.068414747559345734, 7.047288584480712714, 1.012934185448462143 ) ) ;
#193687=CARTESIAN_POINT ( 'NONE',  ( 4.258142763143749399, 7.125527769379820242, 1.199719254218451159 ) ) ;
#193695=CARTESIAN_POINT ( 'NONE',  ( 4.760321332173959696, 4.726332107057286791, 0.000000000000000000 ) ) ;
#193699=CARTESIAN_POINT ( 'NONE',  ( 4.692530564105613422, 7.528350520548263702, -1.082531754730548412 ) ) ;
#193710=EDGE_CURVE ( 'NONE', #63797, #82918, #21920, .T. ) ;
#193711=CARTESIAN_POINT ( 'NONE',  ( -5.099275172515603138, 8.002885897026576600, 1.082531754730549967 ) ) ;
#193743=CARTESIAN_POINT ( 'NONE',  ( 4.420840606507738357, 7.315341919971147355, 1.199719254218451159 ) ) ;
#193754=CARTESIAN_POINT ( 'NONE',  ( -3.284818356260900796, 7.054314858938165678, 0.7998128361456352531 ) ) ;
#193757=CARTESIAN_POINT ( 'NONE',  ( 4.434925645001613681, 5.307073019657559065, -1.082531754730548412 ) ) ;
#193775=CARTESIAN_POINT ( 'NONE',  ( -3.024877669624710386, 6.543124691288523920, 0.000000000000000000 ) ) ;
#193784=DIRECTION ( 'NONE',  ( -0.7592566023653003482, 0.6507913734559641616, 0.000000000000000000 ) ) ;
#193809=CARTESIAN_POINT ( 'NONE',  ( -5.094039349513959536, 7.939876775568885492, 1.214520887661042936 ) ) ;
#193817=CARTESIAN_POINT ( 'NONE',  ( -4.787964524281469458, 5.614988695530339413, -1.199719254218453823 ) ) ;
#193820=CARTESIAN_POINT ( 'NONE',  ( -3.820365424000704557, 7.679119771301277098, -0.7998128361456481317 ) ) ;
#193833=CARTESIAN_POINT ( 'NONE',  ( 4.549643065837591038, 7.465611455855944101, -1.199719254218452047 ) ) ;
#193838=ADVANCED_FACE ( 'NONE', ( #182112 ), #19246, .T. ) ;
#193840=CARTESIAN_POINT ( 'NONE',  ( 0.1949432477380687867, 3.354551554867308827, -2.067633736988962578 ) ) ;
#193855=EDGE_CURVE ( 'NONE', #116214, #86356, #186780, .T. ) ;
#193858=CARTESIAN_POINT ( 'NONE',  ( 5.017399365509065845, 8.011327138806002779, -1.199719254218450271 ) ) ;
#193859=CARTESIAN_POINT ( 'NONE',  ( 4.492547798081839794, 6.334668079219206049, 1.599625672291262513 ) ) ;
#193861=CARTESIAN_POINT ( 'NONE',  ( 4.228163802615382494, 6.026220084508304708, -1.599625672291269396 ) ) ;
#193864=FACE_OUTER_BOUND ( 'NONE', #124539, .T. ) ;
#193867=LINE ( 'NONE', #109504, #127310 ) ;
#193875=CARTESIAN_POINT ( 'NONE',  ( 4.895464504754282409, 8.144056917144915531, 1.010406422583273178 ) ) ;
#193877=CARTESIAN_POINT ( 'NONE',  ( -6.766928066552171828, 7.067373297165212342, 0.7216878364870317197 ) ) ;
#193878=CARTESIAN_POINT ( 'NONE',  ( 4.923019175537949543, 4.916146257648610352, 0.000000000000000000 ) ) ;
#193885=EDGE_CURVE ( 'NONE', #200036, #85668, #27646, .T. ) ;
#193905=CARTESIAN_POINT ( 'NONE',  ( 4.740510986633625024, 5.559626234941203116, -1.199719254218450271 ) ) ;
#193924=CARTESIAN_POINT ( 'NONE',  ( -7.228432174741334038, 8.462200954400218578, -1.199719254218452047 ) ) ;
#193926=ORIENTED_EDGE ( 'NONE', *, *, #200741, .T. ) ;
#193935=CARTESIAN_POINT ( 'NONE',  ( 6.150558962454855561, 7.204682206732687000, 1.199719254218452047 ) ) ;
#193938=ORIENTED_EDGE ( 'NONE', *, *, #1100, .T. ) ;
#193940=EDGE_LOOP ( 'NONE', ( #42974, #33722, #117935, #106248 ) ) ;
#193941=CARTESIAN_POINT ( 'NONE',  ( 4.688087255275310561, 8.691461907788344377, -0.7998128361456381397 ) ) ;
#193951=CARTESIAN_POINT ( 'NONE',  ( 4.612778539632031105, 8.351152097327862123, 0.2683542610703564812 ) ) ;
#193955=B_SPLINE_CURVE_WITH_KNOTS ( 'NONE', 3,
 ( #95237, #161286, #211073, #12872, #128857, #162357 ),
 .UNSPECIFIED., .F., .F.,
 ( 4, 2, 4 ),
 ( 0.8817142480080221167, 0.9367698396229139357, 0.9918254312378057547 ),
 .UNSPECIFIED. ) ;
#193970=CARTESIAN_POINT ( 'NONE',  ( -6.493429226302317225, 6.540365283632955773, 0.7998128361456341429 ) ) ;
#193972=CARTESIAN_POINT ( 'NONE',  ( 6.398522151006641678, 6.429640362454684954, 0.000000000000000000 ) ) ;
#193976=CARTESIAN_POINT ( 'NONE',  ( -5.966470118465691641, 9.118576350588734059, -1.199719254218452047 ) ) ;
#193979=CARTESIAN_POINT ( 'NONE',  ( -6.966220764712148572, 6.002124920821316323, 2.420000000000000373 ) ) ;
#193984=CARTESIAN_POINT ( 'NONE',  ( -5.946407990378149933, 7.222024315256661886, -1.239984355232233826 ) ) ;
#193992=VECTOR ( 'NONE', #192954, 1000.000000000000114 ) ;
#194000=EDGE_LOOP ( 'NONE', ( #139926, #79705, #6536, #158860, #180377 ) ) ;
#194001=CARTESIAN_POINT ( 'NONE',  ( 6.563555762791525972, 6.830105609444471426, -0.7216878364870458196 ) ) ;
#194010=CARTESIAN_POINT ( 'NONE',  ( -4.207966135563093957, 7.175396087857926375, 1.072179110320391260 ) ) ;
#194016=CARTESIAN_POINT ( 'NONE',  ( -5.004368097219957789, 5.011053332944274352, 0.000000000000000000 ) ) ;
#194020=CARTESIAN_POINT ( 'NONE',  ( 6.235824307642648279, 6.239826211863360506, 0.000000000000000000 ) ) ;
#194049=EDGE_LOOP ( 'NONE', ( #44407, #70370 ) ) ;
#194071=CARTESIAN_POINT ( 'NONE',  ( -4.123088111887291518, 7.824370207261548416, 0.000000000000000000 ) ) ;
#194077=ORIENTED_EDGE ( 'NONE', *, *, #165318, .T. ) ;
#194078=CARTESIAN_POINT ( 'NONE',  ( -6.798487682609798632, 6.896266815991691779, 0.7998128361456341429 ) ) ;
#194083=EDGE_LOOP ( 'NONE', ( #93038, #12517, #2055, #37301, #199934, #182007, #28530, #182634, #178935, #22071, #10467, #54240, #197745, #83180, #8914, #184981, #101399, #167607 ) ) ;
#194090=CARTESIAN_POINT ( 'NONE',  ( -4.468294144155606773, 7.370704380560280100, 1.199719254218452935 ) ) ;
#194092=CARTESIAN_POINT ( 'NONE',  ( 5.275877007301786215, 7.772378248882220397, 1.293907329011657614 ) ) ;
#194095=CIRCLE ( 'NONE', #166418, 0.08000000000000041800 ) ;
#194098=CARTESIAN_POINT ( 'NONE',  ( 5.285699784481295183, 7.260012063351913625, 1.599625672291268286 ) ) ;
#194105=CARTESIAN_POINT ( 'NONE',  ( -4.625266680917477835, 5.425174544939014964, -1.199719254218453823 ) ) ;
#194109=CARTESIAN_POINT ( 'NONE',  ( -4.261005416444848315, 8.193199762486115034, 0.7998128361456352531 ) ) ;
#194113=CARTESIAN_POINT ( 'NONE',  ( 5.302647476276220573, 8.240153584747313076, -1.082531754730548412 ) ) ;
#194115=CARTESIAN_POINT ( 'NONE',  ( -5.438229012412890917, 8.398332043573416783, -1.082531754730549967 ) ) ;
#194123=CARTESIAN_POINT ( 'NONE',  ( 4.529305835417093640, 7.441884687032027657, -1.199719254218450271 ) ) ;
#194130=CARTESIAN_POINT ( 'NONE',  ( 5.716698046817569434, 6.698511138489155137, -1.199719254218452047 ) ) ;
#194132=CARTESIAN_POINT ( 'NONE',  ( -1.833030277982346634, 2.531131934864056632, -2.499999999999998668 ) ) ;
#194153=CARTESIAN_POINT ( 'NONE',  ( 4.666668778386947380, 8.284408874816399759, 0.5204741841226891985 ) ) ;
#194162=CARTESIAN_POINT ( 'NONE',  ( 7.191674137406095291, 7.354984346587396082, 0.000000000000000000 ) ) ;
#194167=CARTESIAN_POINT ( 'NONE',  ( -5.050372967203840879, 7.883769262350217133, 1.105620360010154402 ) ) ;
#194169=EDGE_CURVE ( 'NONE', #28052, #148211, #91957, .T. ) ;
#194175=CARTESIAN_POINT ( 'NONE',  ( -7.095713291905736853, 9.371694488680407886, 1.599625672291269396 ) ) ;
#194186=CARTESIAN_POINT ( 'NONE',  ( -5.164730172163054966, 4.990216387137135889, -0.7998128361456362523 ) ) ;
#194190=CARTESIAN_POINT ( 'NONE',  ( -5.608135385276092677, 5.599224824533729716, 0.4022279080854191391 ) ) ;
#194192=DIRECTION ( 'NONE',  ( -0.9829311923673912377, -0.1839735607939864959, 0.000000000000000000 ) ) ;
#194195=ORIENTED_EDGE ( 'NONE', *, *, #21454, .T. ) ;
#194197=CARTESIAN_POINT ( 'NONE',  ( 4.179656494762836516, 8.098292687190454586, -0.7998128361456362523 ) ) ;
#194200=CARTESIAN_POINT ( 'NONE',  ( 6.658462837642799670, 6.940830530104329377, 0.7216878364870328300 ) ) ;
#194209=CARTESIAN_POINT ( 'NONE',  ( -6.041007162748570636, 7.066593642038220935, 1.036256717389577586 ) ) ;
#194216=CARTESIAN_POINT ( 'NONE',  ( -3.461074353238556167, 7.259946855412102273, 0.000000000000000000 ) ) ;
#194217=CARTESIAN_POINT ( 'NONE',  ( 3.932747076415766596, 6.745899468197171345, 1.199719254218451159 ) ) ;
#194228=CARTESIAN_POINT ( 'NONE',  ( -6.882699257592852504, 8.058845884393651460, -1.199719254218452047 ) ) ;
#194229=CARTESIAN_POINT ( 'NONE',  ( 7.340813827156391191, 7.528980651296110160, 0.7998128361456281477 ) ) ;
#194231=CARTESIAN_POINT ( 'NONE',  ( 6.333067150914805765, 9.442309871825708356, 1.082531754730549967 ) ) ;
#194243=CARTESIAN_POINT ( 'NONE',  ( -5.811016664379555330, 7.234075022110222797, -1.179019473189359068 ) ) ;
#194252=CARTESIAN_POINT ( 'NONE',  ( -3.146901051703345331, 6.685485303713597283, 0.000000000000000000 ) ) ;
#194259=LINE ( 'NONE', #127223, #70250 ) ;
#194268=CARTESIAN_POINT ( 'NONE',  ( 5.155843554946782703, 9.237177590738404831, -0.7998128361456481317 ) ) ;
#194271=( BOUNDED_CURVE ( )  B_SPLINE_CURVE ( 2, ( #150850, #118397, #146600, #48034, #184383 ),
 .UNSPECIFIED., .F., .T. ) 
 B_SPLINE_CURVE_WITH_KNOTS ( ( 3, 2, 3 ),
 ( 0.02154092249793660915, 0.02500000000000000139, 0.02797185281523567602 ),
 .UNSPECIFIED. ) 
 CURVE ( )  GEOMETRIC_REPRESENTATION_ITEM ( )  RATIONAL_B_SPLINE_CURVE ( ( 0.9349445691963351734, 0.9443885786059269538, 1.000000000000000000, 0.9522216662880065297, 0.9385209747078349096 ) ) 
 REPRESENTATION_ITEM ( '' )  );
#194283=EDGE_CURVE ( 'NONE', #83383, #190177, #49784, .T. ) ;
#194306=CARTESIAN_POINT ( 'NONE',  ( 7.865138509703455405, 8.348618814175074121, -0.7216878364870317197 ) ) ;
#194335=CARTESIAN_POINT ( 'NONE',  ( -4.606738333593328072, 8.596554832492683929, 0.7998128361456281477 ) ) ;
#194337=CARTESIAN_POINT ( 'NONE',  ( 5.628043163004202931, 8.619781885929965526, -1.082531754730548412 ) ) ;
#194343=CARTESIAN_POINT ( 'NONE',  ( -5.492988512192097161, 6.437516681426083132, 1.199719254218452935 ) ) ;
#194348=CARTESIAN_POINT ( 'NONE',  ( -3.688700311369816909, 6.461178242310183784, -1.199719254218450271 ) ) ;
#194354=CARTESIAN_POINT ( 'NONE',  ( -4.776215253764153346, 8.794277906025310898, -0.7998128361456362523 ) ) ;
#194364=CARTESIAN_POINT ( 'NONE',  ( -5.255720823952942489, 6.160704378480398979, -1.199719254218453823 ) ) ;
#194367=CARTESIAN_POINT ( 'NONE',  ( -6.346625304972878467, 7.537389289624049304, 1.082531754730548412 ) ) ;
#194368=CARTESIAN_POINT ( 'NONE',  ( -6.170369307550858551, 8.292126506933035657, 1.443375672974058777 ) ) ;
#194369=CARTESIAN_POINT ( 'NONE',  ( 7.523848900940885542, 7.742521570711348389, 0.7998128361456291469 ) ) ;
#194370=CARTESIAN_POINT ( 'NONE',  ( -5.610041701004606196, 9.767075427805856691, -0.7998128361456362523 ) ) ;
#194408=CARTESIAN_POINT ( 'NONE',  ( 4.754190777897029818, 8.299541367957775861, -0.7767638722561143183 ) ) ;
#194419=EDGE_CURVE ( 'NONE', #173630, #153847, #28928, .T. ) ;
#194423=CARTESIAN_POINT ( 'NONE',  ( 6.900173834712277632, 7.014900660111269559, -0.7998128361456341429 ) ) ;
#194426=CARTESIAN_POINT ( 'NONE',  ( -5.842637852846353397, 5.781108681267656202, 0.7998128361456281477 ) ) ;
#194430=CARTESIAN_POINT ( 'NONE',  ( -5.275531169048895741, 9.168887107283438809, -0.7216878364870338292 ) ) ;
#194441=CARTESIAN_POINT ( 'NONE',  ( 7.842465510862060896, 8.114240948952696542, 0.000000000000000000 ) ) ;
#194442=CARTESIAN_POINT ( 'NONE',  ( 5.505492895601038938, 8.580769590579979678, -1.199719254218452047 ) ) ;
#194454=ORIENTED_EDGE ( 'NONE', *, *, #59652, .T. ) ;
#194455=CARTESIAN_POINT ( 'NONE',  ( 6.282224075085741433, 8.422623735723785643, 1.599625672291268286 ) ) ;
#194467=DIRECTION ( 'NONE',  ( 0.000000000000000000, 0.000000000000000000, 1.000000000000000000 ) ) ;
#194470=CARTESIAN_POINT ( 'NONE',  ( -4.502716413514301408, 7.306900678191715848, -1.082531754730549967 ) ) ;
#194471=CARTESIAN_POINT ( 'NONE',  ( -6.994027139803241866, 9.253060644560830994, -1.599625672291271394 ) ) ;
#194473=CARTESIAN_POINT ( 'NONE',  ( -4.916039773278787273, 4.881957280557857715, 0.5603013081572870702 ) ) ;
#194483=CARTESIAN_POINT ( 'NONE',  ( 5.515134625708930649, 9.656350506627580543, 0.000000000000000000 ) ) ;
#194486=CARTESIAN_POINT ( 'NONE',  ( 4.760321331729593375, 5.686701320840210627, -1.082531754730548412 ) ) ;
#194503=CARTESIAN_POINT ( 'NONE',  ( 4.603875680292229156, 7.528882839386387360, 1.199719254218452047 ) ) ;
#194504=CARTESIAN_POINT ( 'NONE',  ( -3.332271893908731464, 7.109677319527304640, -0.7998128361456481317 ) ) ;
#194515=CARTESIAN_POINT ( 'NONE',  ( 7.024532985656136930, 8.328281583754568729, 1.082531754730549967 ) ) ;
#194517=CARTESIAN_POINT ( 'NONE',  ( -6.957269102468015554, 8.145844036748005834, 1.199719254218452047 ) ) ;
#194518=CARTESIAN_POINT ( 'NONE',  ( 4.179656494762836516, 8.098292687190454586, -0.7998128361456362523 ) ) ;
#194527=CARTESIAN_POINT ( 'NONE',  ( -4.163763581353360443, 7.871824920094959488, -5.011504818508299590E-05 ) ) ;
#194528=CARTESIAN_POINT ( 'NONE',  ( -4.447956913735107598, 7.346977611736363656, 1.199719254218452935 ) ) ;
#194540=CYLINDRICAL_SURFACE ( 'NONE', #5163, 0.08000000000000020983 ) ;
#194557=CARTESIAN_POINT ( 'NONE',  ( 5.451787166470912993, 6.493411461371761284, -1.082531754730548412 ) ) ;
#194563=CARTESIAN_POINT ( 'NONE',  ( 5.709392084686216506, 5.833581318321598985, -0.7216878364870458196 ) ) ;
#194576=CARTESIAN_POINT ( 'NONE',  ( -5.631432701629818460, 7.663367133358481631, 1.599625672291263179 ) ) ;
#194578=CARTESIAN_POINT ( 'NONE',  ( -6.994027139803241866, 9.253060644560830994, -1.599625672291271394 ) ) ;
#194591=CARTESIAN_POINT ( 'NONE',  ( -6.934069218746458318, 7.054445274817795486, -0.7998128361456362523 ) ) ;
#194597=CARTESIAN_POINT ( 'NONE',  ( -3.838366886444665393, 7.492195444245147939, 0.000000000000000000 ) ) ;
#194600=CARTESIAN_POINT ( 'NONE',  ( -6.445975688654487001, 6.485002823043819475, -0.7998128361456362523 ) ) ;
#194610=VECTOR ( 'NONE', #66013, 1000.000000000000114 ) ;
#194616=CARTESIAN_POINT ( 'NONE',  ( -6.558215298580997832, 6.787841129500100656, 0.5453671684877616777 ) ) ;
#194621=CARTESIAN_POINT ( 'NONE',  ( -3.485854892044998543, 6.120562236477518070, -1.082531754730546636 ) ) ;
#194622=DIRECTION ( 'NONE',  ( 0.000000000000000000, 0.000000000000000000, 1.000000000000000000 ) ) ;
#194623=CARTESIAN_POINT ( 'NONE',  ( -3.481411583659053566, 7.283673624236017830, 0.000000000000000000 ) ) ;
#194650=CARTESIAN_POINT ( 'NONE',  ( -7.442499979258930587, 7.647614495415686164, -0.7998128361456362523 ) ) ;
#194657=CARTESIAN_POINT ( 'NONE',  ( 3.930720324626956863, 8.992102070998166496, 0.7749999999999996891 ) ) ;
#194674=CARTESIAN_POINT ( 'NONE',  ( 6.801350335910821165, 7.963938809097990124, 1.199719254218452047 ) ) ;
#194675=CARTESIAN_POINT ( 'NONE',  ( 4.505997031185814627, 8.479023313017261643, -0.7440749432275711728 ) ) ;
#194679=( BOUNDED_CURVE ( )  B_SPLINE_CURVE ( 2, ( #161249, #45378, #17096, #145032, #95198 ),
 .UNSPECIFIED., .F., .T. ) 
 B_SPLINE_CURVE_WITH_KNOTS ( ( 3, 2, 3 ),
 ( 0.2697076323948381371, 0.2750000000000000222, 0.2818589531839510443 ),
 .UNSPECIFIED. ) 
 CURVE ( )  GEOMETRIC_REPRESENTATION_ITEM ( )  RATIONAL_B_SPLINE_CURVE ( ( 0.9379021630552799582, 0.9149148624488946391, 1.000000000000000000, 0.8897289420062464149, 0.9609804498502303449 ) ) 
 REPRESENTATION_ITEM ( '' )  );
#194690=CARTESIAN_POINT ( 'NONE',  ( 4.855733865602142707, 8.067643820953190215, 0.9155131637919884380 ) ) ;
#194692=CARTESIAN_POINT ( 'NONE',  ( 5.668717624289557833, 8.667235424096215723, -1.082531754730548412 ) ) ;
#194698=CARTESIAN_POINT ( 'NONE',  ( -5.808742468812186033, 5.741564066561132940, 0.000000000000000000 ) ) ;
#194705=CARTESIAN_POINT ( 'NONE',  ( -6.902509602688830626, 7.225551755991315162, -0.7216878364870338292 ) ) ;
#194708=CARTESIAN_POINT ( 'NONE',  ( -4.002183151617731305, 7.677155228057962688, 0.1020948806719407381 ) ) ;
#194713=CARTESIAN_POINT ( 'NONE',  ( -5.334207092333882017, 5.187939460669764635, 0.7998128361456281477 ) ) ;
#194723=CARTESIAN_POINT ( 'NONE',  ( 3.410758162289653672, 6.136912401716668519, -1.199719254218453823 ) ) ;
#194727=VERTEX_POINT ( 'NONE', #194527 ) ;
#194743=CARTESIAN_POINT ( 'NONE',  ( -7.425025402139490360, 8.691559719698066289, 1.199719254218452047 ) ) ;
#194746=CARTESIAN_POINT ( 'NONE',  ( 5.332099551924443404, 9.442809587212341427, 0.000000000000000000 ) ) ;
#194747=FACE_OUTER_BOUND ( 'NONE', #168373, .T. ) ;
#194750=CARTESIAN_POINT ( 'NONE',  ( -6.394499343358424959, 6.826875778244118287, 0.5478302896938479494 ) ) ;
#194756=CARTESIAN_POINT ( 'NONE',  ( 6.215487077222150880, 6.216099443039444949, 0.000000000000000000 ) ) ;
#194763=CARTESIAN_POINT ( 'NONE',  ( 4.014622883422321209, 5.777089012116397804, -1.443375672974068769 ) ) ;
#194765=CIRCLE ( 'NONE', #25168, 4.583333333333340143 ) ;
#194767=CARTESIAN_POINT ( 'NONE',  ( 5.234856708652222856, 8.161064355852680308, 1.082531754730549078 ) ) ;
#194778=CARTESIAN_POINT ( 'NONE',  ( -5.722950238744243023, 7.770137593325314285, 1.443375672974058777 ) ) ;
#194802=CARTESIAN_POINT ( 'NONE',  ( 5.601295902029185036, 5.735459099175467479, 0.6339577218646634815 ) ) ;
#194812=CARTESIAN_POINT ( 'NONE',  ( 6.391743074199808916, 6.421731439513382433, -0.7998128361456481317 ) ) ;
#194814=CARTESIAN_POINT ( 'NONE',  ( 5.712781623311797397, 7.758274208654143855, -1.599625672291283607 ) ) ;
#194824=CARTESIAN_POINT ( 'NONE',  ( -3.149236820124241110, 6.896136400112061970, -0.7998128361456481317 ) ) ;
#194828=CARTESIAN_POINT ( 'NONE',  ( 5.058600711230250013, 5.074324715956299414, -0.7216878364870458196 ) ) ;
#194845=CARTESIAN_POINT ( 'NONE',  ( -4.326460416536637155, 8.061637896019123062, 0.000000000000000000 ) ) ;
#194847=CARTESIAN_POINT ( 'NONE',  ( -4.448483799059637533, 7.243629294661272588, 1.082531754730549967 ) ) ;
#194883=CARTESIAN_POINT ( 'NONE',  ( -7.425025402139490360, 8.691559719698066289, 1.199719254218452047 ) ) ;
#194884=CARTESIAN_POINT ( 'NONE',  ( -5.321855017605967575, 7.728530711523490027, 1.321107644836617467 ) ) ;
#194892=CARTESIAN_POINT ( 'NONE',  ( -4.359828915246279024, 7.244161613499399799, -1.199719254218455378 ) ) ;
#194895=CARTESIAN_POINT ( 'NONE',  ( -5.666381855868691808, 5.575476684793721383, 0.000000000000000000 ) ) ;
#194907=CARTESIAN_POINT ( 'NONE',  ( 4.766573523656222555, 7.718696989977711809, 1.199719254218452047 ) ) ;
#194932=CARTESIAN_POINT ( 'NONE',  ( 4.908934136599710563, 7.884784371745123366, 1.199719254218451159 ) ) ;
#194933=CARTESIAN_POINT ( 'NONE',  ( 5.248941747146098180, 6.152795455539095570, -1.199719254218452047 ) ) ;
#194935=CARTESIAN_POINT ( 'NONE',  ( 5.011674058906918638, 5.875983152593414971, 1.199719254218452047 ) ) ;
#194949=CARTESIAN_POINT ( 'NONE',  ( 4.614865537624940117, 8.465324746759504748, 0.2878883051726736086 ) ) ;
#194950=CARTESIAN_POINT ( 'NONE',  ( -6.427974226210522168, 6.671927150099951298, 0.000000000000000000 ) ) ;
#194964=ORIENTED_EDGE ( 'NONE', *, *, #99445, .T. ) ;
#194977=CARTESIAN_POINT ( 'NONE',  ( 3.718679271898170491, 7.560485927181699317, 0.7998128361456271485 ) ) ;
#194979=CARTESIAN_POINT ( 'NONE',  ( 5.571474780572990504, 5.464751763615448787, 0.7998128361456352531 ) ) ;
#194997=CARTESIAN_POINT ( 'NONE',  ( -6.474900878978163021, 9.711745571186627402, -1.199719254218452047 ) ) ;
#195010=CARTESIAN_POINT ( 'NONE',  ( 6.717138760927786834, 6.801359740696030443, -0.7998128361456481317 ) ) ;
#195017=CARTESIAN_POINT ( 'NONE',  ( 4.875038752565570732, 7.845239757038595663, -1.199719254218452047 ) ) ;
#195026=CARTESIAN_POINT ( 'NONE',  ( 4.871153761480781164, 8.051123856976298399, 0.9350251597124116243 ) ) ;
#195028=CARTESIAN_POINT ( 'NONE',  ( 4.594924845400013780, 8.373833185659544043, 0.04553248676899754321 ) ) ;
#195046=CARTESIAN_POINT ( 'NONE',  ( -4.145761110728687804, 8.058748072483927771, -0.7998128361456481317 ) ) ;
#195048=CARTESIAN_POINT ( 'NONE',  ( 6.170896192875352959, 7.228408975556602556, 1.199719254218453823 ) ) ;
#195049=CARTESIAN_POINT ( 'NONE',  ( -2.277139237642805902, 2.743616490267797747, 2.500000000000000000 ) ) ;
#195052=CARTESIAN_POINT ( 'NONE',  ( -5.725286006720766707, 9.901527117808042178, 0.7998128361456291469 ) ) ;
#195055=VERTEX_POINT ( 'NONE', #1624 ) ;
#195061=CARTESIAN_POINT ( 'NONE',  ( -0.3970953499397937292, 3.114959765369129219, -1.961950730382394870 ) ) ;
#195068=ADVANCED_FACE ( 'NONE', ( #117605 ), #201948, .F. ) ;
#195081=CARTESIAN_POINT ( 'NONE',  ( 5.072158865288222351, 8.931619419562697004, 0.7216878364870317197 ) ) ;
#195097=CARTESIAN_POINT ( 'NONE',  ( -3.838774385731502203, 7.492511168737228111, -0.01748052351197342674 ) ) ;
#195098=CARTESIAN_POINT ( 'NONE',  ( -5.817857314039913241, 5.960124085900898372, 0.000000000000000000 ) ) ;
#195102=CARTESIAN_POINT ( 'NONE',  ( 4.213551878797002992, 8.137837301896977849, 0.000000000000000000 ) ) ;
#195120=CARTESIAN_POINT ( 'NONE',  ( 7.797347741190739256, 8.269529584243604958, 0.7216878364870267237 ) ) ;
#195148=CARTESIAN_POINT ( 'NONE',  ( 4.475600106286968582, 5.354526557823810151, -1.082531754730548412 ) ) ;
#195158=CARTESIAN_POINT ( 'NONE',  ( -5.112833325684916552, 7.058334528089422300, -1.443375672974066548 ) ) ;
#195164=CARTESIAN_POINT ( 'NONE',  ( -5.611095471209320174, 7.639640364534566075, 1.599625672291263179 ) ) ;
#195169=ORIENTED_EDGE ( 'NONE', *, *, #74578, .F. ) ;
#195173=CARTESIAN_POINT ( 'NONE',  ( -4.359828915246279024, 7.244161613499399799, -1.199719254218455378 ) ) ;
#195176=CARTESIAN_POINT ( 'NONE',  ( 6.104935607482663507, 7.108274908414393245, 1.121150977946131722 ) ) ;
#195179=CARTESIAN_POINT ( 'NONE',  ( 2.982514307567902812, 6.468353249220382573, 0.4073410874377252910 ) ) ;
#195181=CARTESIAN_POINT ( 'NONE',  ( 4.857564175446106525, 8.889184981320973122, 0.7998128361456331437 ) ) ;
#195187=CARTESIAN_POINT ( 'NONE',  ( -2.428612866367529932E-14, 8.999999999999998224, 0.7749999999999996891 ) ) ;
#195188=CARTESIAN_POINT ( 'NONE',  ( -4.248501033035892327, 6.049946853332221153, -1.599625672291271394 ) ) ;
#195192=CARTESIAN_POINT ( 'NONE',  ( -3.962726036944197894, 7.845207153068690431, -0.7998128361456481317 ) ) ;
#195195=CARTESIAN_POINT ( 'NONE',  ( 5.628043163004202931, 8.619781885929965526, -1.082531754730548412 ) ) ;
#195197=CARTESIAN_POINT ( 'NONE',  ( -6.089020385868867180, 7.236850217336030511, -1.082531754730549967 ) ) ;
#195203=CARTESIAN_POINT ( 'NONE',  ( 3.881377115262159894, 7.750300077773022878, 0.7998128361456271485 ) ) ;
#195210=CARTESIAN_POINT ( 'NONE',  ( 5.817764947765640571, 7.282435344852455472, -1.374816383645981688 ) ) ;
#195211=ADVANCED_FACE ( 'NONE', ( #8042 ), #190001, .T. ) ;
#195232=CARTESIAN_POINT ( 'NONE',  ( 4.739057715201537846, 8.198473722472776615, 0.7146191656044629248 ) ) ;
#195241=CARTESIAN_POINT ( 'NONE',  ( 5.996449078994045223, 10.21788403546024782, 0.7998128361456331437 ) ) ;
#195247=CARTESIAN_POINT ( 'NONE',  ( -5.005744162364479166, 7.928486884654230238, -1.069363714833789558 ) ) ;
#195254=CARTESIAN_POINT ( 'NONE',  ( -3.458738584817664385, 7.049295759013638474, 0.7216878364870338292 ) ) ;
#195260=B_SPLINE_CURVE_WITH_KNOTS ( 'NONE', 3,
 ( #142079, #192906, #40285, #211292, #98629, #61860, #114933, #18 ),
 .UNSPECIFIED., .F., .F.,
 ( 4, 2, 2, 4 ),
 ( 3.127317220692751914E-18, 0.003102675431456557598, 0.004654013147184835747, 0.006205350862913112595 ),
 .UNSPECIFIED. ) ;
#195266=CARTESIAN_POINT ( 'NONE',  ( -3.871735385154307263, 6.674719161725423788, -1.199719254218450271 ) ) ;
#195277=CARTESIAN_POINT ( 'NONE',  ( 5.041653019435334393, 6.975290837464928728, -1.599625672291269396 ) ) ;
#195281=CARTESIAN_POINT ( 'NONE',  ( 4.028181036591620412, 7.713645286083276709, -0.7216878364870338292 ) ) ;
#195293=B_SPLINE_CURVE_WITH_KNOTS ( 'NONE', 3,
 ( #158281, #106370, #9871, #90084, #156147, #142049 ),
 .UNSPECIFIED., .F., .F.,
 ( 4, 2, 4 ),
 ( 0.000000000000000000, 0.0006264319474642703360, 0.001252863894928540672 ),
 .UNSPECIFIED. ) ;
#195296=CARTESIAN_POINT ( 'NONE',  ( -5.795184315198522285, 5.725746220678519904, -0.7998128361456362523 ) ) ;
#195298=CARTESIAN_POINT ( 'NONE',  ( 4.041212305325117882, 6.872442235258051646, -1.199719254218448494 ) ) ;
#195308=CARTESIAN_POINT ( 'NONE',  ( -7.611976899429754084, 7.845337568948314022, 0.7998128361456341429 ) ) ;
#195309=CARTESIAN_POINT ( 'NONE',  ( 7.028976294042106332, 7.165170195996068969, 0.000000000000000000 ) ) ;
#195313=EDGE_LOOP ( 'NONE', ( #169765, #194454, #173490, #34003, #43186, #106866, #145769, #52741, #180368 ) ) ;
#195323=CARTESIAN_POINT ( 'NONE',  ( -6.616720264197946122, 6.757059058146986708, -0.05018984082068300712 ) ) ;
#195332=CARTESIAN_POINT ( 'NONE',  ( -5.112833325684928987, 5.137596099486740897, -0.7216878364870338292 ) ) ;
#195346=CARTESIAN_POINT ( 'NONE',  ( 7.367930134383754215, 7.560616343061329125, -0.7998128361456341429 ) ) ;
#195381=CARTESIAN_POINT ( 'NONE',  ( 6.373741612200160667, 9.489763409991955001, 1.082531754730549078 ) ) ;
#195408=VECTOR ( 'NONE', #188282, 1000.000000000000000 ) ;
#195415=CARTESIAN_POINT ( 'NONE',  ( -6.306477729012051725, 7.386587434382707151, 1.199719254218452047 ) ) ;
#195417=CARTESIAN_POINT ( 'NONE',  ( 6.821160681006793070, 7.130644680695653825, 0.7216878364870328300 ) ) ;
#195422=CARTESIAN_POINT ( 'NONE',  ( -6.005335696210345020, 5.970922831858983315, 0.7998128361456281477 ) ) ;
#195427=CARTESIAN_POINT ( 'NONE',  ( -3.447516199624892419, 7.244129009529488350, 0.7998128361456352531 ) ) ;
#195433=CARTESIAN_POINT ( 'NONE',  ( -6.947627372360122955, 7.070263120700404968, 0.000000000000000000 ) ) ;
#195443=CARTESIAN_POINT ( 'NONE',  ( -5.147255595043616516, 6.034161611419515125, 1.199719254218452935 ) ) ;
#195447=CARTESIAN_POINT ( 'NONE',  ( -4.489158259900630554, 8.251452046610447510, 0.000000000000000000 ) ) ;
#195448=CARTESIAN_POINT ( 'NONE',  ( -5.411112705185557203, 9.327065566109540740, 0.7216878364870267237 ) ) ;
#195449=CARTESIAN_POINT ( 'NONE',  ( 6.770317605177710085, 8.992066187497757213, 1.599625672291268286 ) ) ;
#195451=CARTESIAN_POINT ( 'NONE',  ( -6.312203035614172286, 9.521931420595302953, -1.199719254218452047 ) ) ;
#195463=ORIENTED_EDGE ( 'NONE', *, *, #82643, .T. ) ;
#195486=CARTESIAN_POINT ( 'NONE',  ( 4.595450297557979624, 8.489593704440707711, 0.02661077391274621617 ) ) ;
#195499=CARTESIAN_POINT ( 'NONE',  ( 7.225569521440261767, 7.394528961293920233, -0.7998128361456341429 ) ) ;
#195502=CARTESIAN_POINT ( 'NONE',  ( -4.359828915246279024, 7.244161613499399799, -1.199719254218455378 ) ) ;
#195506=CARTESIAN_POINT ( 'NONE',  ( -5.736508391913536897, 9.706693867292189637, 0.7216878364870267237 ) ) ;
#195510=DIRECTION ( 'NONE',  ( 0.000000000000000000, 0.000000000000000000, 1.000000000000000000 ) ) ;
#195517=CARTESIAN_POINT ( 'NONE',  ( 3.549202351727371862, 7.362762853649070571, -0.7998128361456362523 ) ) ;
#195519=CARTESIAN_POINT ( 'NONE',  ( 5.155843554946782703, 9.237177590738404831, -0.7998128361456481317 ) ) ;
#195527=CARTESIAN_POINT ( 'NONE',  ( 4.167152111353856547, 5.955039778036558040, 1.599625672291262513 ) ) ;
#195533=CARTESIAN_POINT ( 'NONE',  ( 5.091969210384201361, 8.098325291160362482, 1.199719254218452047 ) ) ;
#195548=CARTESIAN_POINT ( 'NONE',  ( -5.533136088152923904, 6.588318536667425285, 1.082531754730549078 ) ) ;
#195549=CARTESIAN_POINT ( 'NONE',  ( 4.570507181582611267, 8.346359121906111511, 0.000000000000000000 ) ) ;
#195562=CARTESIAN_POINT ( 'NONE',  ( -7.607533591043815768, 8.048079742405473525, 0.000000000000000000 ) ) ;
#195563=CARTESIAN_POINT ( 'NONE',  ( 6.770317605177710085, 8.992066187497757213, 1.599625672291268286 ) ) ;
#195566=CARTESIAN_POINT ( 'NONE',  ( 3.540087506499646874, 7.144202834309300698, -0.7216878364870338292 ) ) ;
#195573=CARTESIAN_POINT ( 'NONE',  ( -1.843739406749240750, 9.999999999999998224, -0.7749999999999996891 ) ) ;
#195580=CARTESIAN_POINT ( 'NONE',  ( -5.853222892721556825, 6.632591286734531799, 0.9264282755401199720 ) ) ;
#195583=CARTESIAN_POINT ( 'NONE',  ( 4.389807875774629942, 8.343469298370917997, 0.7998128361456271485 ) ) ;
#195585=CARTESIAN_POINT ( 'NONE',  ( -4.980641328173854632, 6.904110530993182948, 1.599625672291263179 ) ) ;
#195598=CARTESIAN_POINT ( 'NONE',  ( 5.722950238744198614, 8.730506807626655430, 1.082531754730549967 ) ) ;
#195601=CARTESIAN_POINT ( 'NONE',  ( -5.284646014276622950, 9.387447126623207794, -0.7998128361456362523 ) ) ;
#195602=CARTESIAN_POINT ( 'NONE',  ( 4.342354338126830804, 8.288106837781779035, -0.7998128361456381397 ) ) ;
#195610=CARTESIAN_POINT ( 'NONE',  ( -6.608673532018475960, 6.674816973635147477, -0.7998128361456362523 ) ) ;
#195619=CARTESIAN_POINT ( 'NONE',  ( 4.963960565410041603, 8.060099936542098220, -1.154953748940761971 ) ) ;
#195639=CARTESIAN_POINT ( 'NONE',  ( 3.431622278034673901, 7.017660067766835930, -1.734723475976807094E-15 ) ) ;
#195645=CARTESIAN_POINT ( 'NONE',  ( 5.682275777458851707, 6.762314840857718501, 1.082531754730549078 ) ) ;
#195659=CARTESIAN_POINT ( 'NONE',  ( -4.606738333593328072, 8.596554832492683929, 0.7998128361456281477 ) ) ;
#195661=CARTESIAN_POINT ( 'NONE',  ( -7.611976899429754084, 7.845337568948314022, 0.7998128361456341429 ) ) ;
#195667=CARTESIAN_POINT ( 'NONE',  ( 7.700104897918568447, 7.948153567185284096, 0.000000000000000000 ) ) ;
#195671=CARTESIAN_POINT ( 'NONE',  ( -5.608575705693957580, 5.613253794934144558, 0.4301505824422513502 ) ) ;
#195672=CARTESIAN_POINT ( 'NONE',  ( -6.557303570864871034, 7.679217583210999010, -1.199719254218452047 ) ) ;
#195678=CARTESIAN_POINT ( 'NONE',  ( -5.804299160426249493, 5.944306240018289778, -0.7216878364870338292 ) ) ;
#195681=CARTESIAN_POINT ( 'NONE',  ( -4.664887371553763096, 7.600063145858131364, -1.199719254218453823 ) ) ;
#195698=CARTESIAN_POINT ( 'NONE',  ( -6.589834235204424573, 6.767115956813761102, 0.4477994332492858387 ) ) ;
#195703=CARTESIAN_POINT ( 'NONE',  ( -7.391130018105325661, 8.652015104991543026, -1.199719254218452047 ) ) ;
#195704=CARTESIAN_POINT ( 'NONE',  ( 4.760848217054122422, 5.583353003765119560, -1.199719254218452047 ) ) ;
#195705=CARTESIAN_POINT ( 'NONE',  ( -4.142898457427624415, 6.991076079377632091, 1.199719254218452935 ) ) ;
#195714=CARTESIAN_POINT ( 'NONE',  ( 5.519577934094861860, 6.572500690266394940, 1.082531754730549078 ) ) ;
#195716=ORIENTED_EDGE ( 'NONE', *, *, #141289, .T. ) ;
#195729=CARTESIAN_POINT ( 'NONE',  ( -7.469616286486262524, 7.679250187180907794, 0.7998128361456341429 ) ) ;
#195731=EDGE_CURVE ( 'NONE', #43808, #134523, #44123, .T. ) ;
#195755=CARTESIAN_POINT ( 'NONE',  ( 6.587282531393223728, 8.778525268082516320, 1.599625672291268286 ) ) ;
#195767=CARTESIAN_POINT ( 'NONE',  ( 5.148720134264945791, 7.772403765597828418, 1.171659602702241676 ) ) ;
#195769=CARTESIAN_POINT ( 'NONE',  ( 6.427974226654860956, 7.632296364919712417, -1.082531754730548412 ) ) ;
#195774=CARTESIAN_POINT ( 'NONE',  ( -4.610654757099099221, 7.536791762327691657, 1.199719254218452935 ) ) ;
#195781=CARTESIAN_POINT ( 'NONE',  ( -6.821160681006823268, 9.051383109298335228, 1.443375672974064550 ) ) ;
#195790=CARTESIAN_POINT ( 'NONE',  ( -4.930325137224961907, 5.781076077297750970, -1.199719254218453823 ) ) ;
#195801=CARTESIAN_POINT ( 'NONE',  ( 5.585032934186686226, 5.480569609498057382, 0.000000000000000000 ) ) ;
#195816=CARTESIAN_POINT ( 'NONE',  ( -6.328041841479842056, 6.870487382198048998, 0.6860574420480938240 ) ) ;
#195819=CARTESIAN_POINT ( 'NONE',  ( -5.887983850084758330, 10.09134126839936840, 0.7998128361456291469 ) ) ;
#195822=CARTESIAN_POINT ( 'NONE',  ( 5.169401708560450004, 9.252995436621013425, 0.000000000000000000 ) ) ;
#195825=CARTESIAN_POINT ( 'NONE',  ( -5.214720930002679999, 7.727253977155453590, 1.197825571464938399 ) ) ;
#195832=CARTESIAN_POINT ( 'NONE',  ( 5.987861119090863049, 7.014868056141362551, 1.199719254218452047 ) ) ;
#195842=CARTESIAN_POINT ( 'NONE',  ( -4.715876479964030032, 8.338641909828480081, -0.7613925308670350667 ) ) ;
#195843=CARTESIAN_POINT ( 'NONE',  ( 5.072158865288222351, 8.931619419562697004, 0.7216878364870317197 ) ) ;
#195855=CARTESIAN_POINT ( 'NONE',  ( -6.455090533882213322, 6.703562842383589349, -0.7216878364870338292 ) ) ;
#195889=CARTESIAN_POINT ( 'NONE',  ( 5.879395890181562834, 6.888325289080478697, -1.199719254218452047 ) ) ;
#195891=CARTESIAN_POINT ( 'NONE',  ( 5.682802662783380754, 6.658966523782627434, 1.199719254218452935 ) ) ;
#195906=CARTESIAN_POINT ( 'NONE',  ( -2.959422669532919326, 6.674686557755516780, 0.7998128361456352531 ) ) ;
#195910=CARTESIAN_POINT ( 'NONE',  ( 4.868786560638889149, 6.773613302202437403, 1.443375672974065660 ) ) ;
#195924=CARTESIAN_POINT ( 'NONE',  ( -5.641601317062239218, 8.635599732330991429, -1.082531754730549967 ) ) ;
#195926=CARTESIAN_POINT ( 'NONE',  ( -6.129694847154231852, 6.323934541200937787, -0.7216878364870338292 ) ) ;
#195954=CARTESIAN_POINT ( 'NONE',  ( -5.113360211009450040, 5.994616996712990975, -1.199719254218453823 ) ) ;
#195964=CARTESIAN_POINT ( 'NONE',  ( -7.422162748838431412, 7.623887726591770608, -0.7998128361456362523 ) ) ;
#195965=CARTESIAN_POINT ( 'NONE',  ( -4.589286827423546100, 8.493149336607261901, 0.1385767598228414277 ) ) ;
#195968=CARTESIAN_POINT ( 'NONE',  ( -7.065207446497166366, 9.336104335703744539, 0.000000000000000000 ) ) ;
#195971=CARTESIAN_POINT ( 'NONE',  ( -8.068510813464099485, 8.585886501895810596, 0.7216878364870317197 ) ) ;
#195975=CARTESIAN_POINT ( 'NONE',  ( -5.815521545619021460, 5.749472989502435460, -0.7998128361456362523 ) ) ;
#195988=CARTESIAN_POINT ( 'NONE',  ( 4.389807875774629942, 8.343469298370917997, 0.7998128361456271485 ) ) ;
#196012=CARTESIAN_POINT ( 'NONE',  ( 5.204350862799327793, 7.165104988056252289, -1.599625672291281386 ) ) ;
#196013=CARTESIAN_POINT ( 'NONE',  ( 4.817943484809818600, 6.714296380401858499, 1.599625672291269396 ) ) ;
#196015=CARTESIAN_POINT ( 'NONE',  ( 3.217027588192558074, 6.975225629525113824, -1.734723475976807094E-15 ) ) ;
#196026=CARTESIAN_POINT ( 'NONE',  ( 4.710809438828709617, 8.349644928513606956, 0.6747337923850562635 ) ) ;
#196027=CARTESIAN_POINT ( 'NONE',  ( -5.600926855776894975, 6.667407765562058053, -1.082531754730549967 ) ) ;
#196057=CARTESIAN_POINT ( 'NONE',  ( 6.229045230835819069, 6.231917288922055320, -0.7998128361456481317 ) ) ;
#196059=CARTESIAN_POINT ( 'NONE',  ( 2.898410978271408922, 6.603506251283770112, -0.7998128361456362523 ) ) ;
#196077=CARTESIAN_POINT ( 'NONE',  ( -5.908321080505254841, 10.11506803722328129, 0.7998128361456291469 ) ) ;
#196089=CARTESIAN_POINT ( 'NONE',  ( 6.313256805818848960, 7.394496357324014113, 1.199719254218452047 ) ) ;
#196093=CARTESIAN_POINT ( 'NONE',  ( 5.875479466675786355, 7.948088359245467416, -1.599625672291283607 ) ) ;
#196102=CARTESIAN_POINT ( 'NONE',  ( -1.849150832860085414, 8.949220158640459388, 0.7750000000000013545 ) ) ;
#196103=CARTESIAN_POINT ( 'NONE',  ( 4.678042868546113731, 8.270637144445508682, 0.5573067791126932180 ) ) ;
#196122=VECTOR ( 'NONE', #132279, 1000.000000000000000 ) ;
#196124=CARTESIAN_POINT ( 'NONE',  ( -5.956828388357799042, 8.042995434541133193, 1.599625672291263179 ) ) ;
#196126=CARTESIAN_POINT ( 'NONE',  ( 5.550083779947807550, 7.568460058062819407, -1.599625672291283607 ) ) ;
#196129=CARTESIAN_POINT ( 'NONE',  ( -7.761116589180078407, 8.019333873657032541, 0.000000000000000000 ) ) ;
#196137=CARTESIAN_POINT ( 'NONE',  ( -6.514548575684607989, 6.824011503973982151, -0.5624163230865379948 ) ) ;
#196153=CARTESIAN_POINT ( 'NONE',  ( 7.024532985656141371, 7.367912369453226695, 0.7216878364870328300 ) ) ;
#196156=CARTESIAN_POINT ( 'NONE',  ( -6.563028877466991595, 9.814561569423593923, 1.199719254218452935 ) ) ;
#196167=CARTESIAN_POINT ( 'NONE',  ( -3.874835629217528776, 7.473463894690999254, -0.3237328633659316002 ) ) ;
#196168=CARTESIAN_POINT ( 'NONE',  ( -3.499413046103020175, 7.096749297179887783, 0.7216878364870338292 ) ) ;
#196171=CARTESIAN_POINT ( 'NONE',  ( 5.254667053748194760, 8.288139441751686931, 1.199719254218452047 ) ) ;
#196174=CARTESIAN_POINT ( 'NONE',  ( -10.17567228521070710, -0.02076350362892331880, 2.499999999999999556 ) ) ;
#196200=VERTEX_POINT ( 'NONE', #196704 ) ;
#196221=CARTESIAN_POINT ( 'NONE',  ( -4.164650907004922686, 7.866613389087279806, 0.1028172011370054872 ) ) ;
#196224=CARTESIAN_POINT ( 'NONE',  ( -6.089020385868876062, 6.276481003034692030, -0.7216878364870338292 ) ) ;
#196225=CARTESIAN_POINT ( 'NONE',  ( 4.689424523294686509, 8.358602041046323095, -0.7454045323363467368 ) ) ;
#196230=CARTESIAN_POINT ( 'NONE',  ( -6.134138155540168391, 6.121192367743780949, 0.000000000000000000 ) ) ;
#196236=CARTESIAN_POINT ( 'NONE',  ( -1.854512760316423536, 2.488359591189891251, 2.484105960264900936 ) ) ;
#196237=CARTESIAN_POINT ( 'NONE',  ( -3.969505113751027547, 7.853116076009993840, 1.214306433183764966E-14 ) ) ;
#196240=CARTESIAN_POINT ( 'NONE',  ( 6.148788998471866662, 7.076870205577955986, 1.084632487400632339 ) ) ;
#196245=CARTESIAN_POINT ( 'NONE',  ( 7.015418140428412386, 7.149352350113456822, 0.7998128361456331437 ) ) ;
#196253=CARTESIAN_POINT ( 'NONE',  ( -3.481411583659053566, 7.283673624236017830, 0.000000000000000000 ) ) ;
#196257=CARTESIAN_POINT ( 'NONE',  ( -5.773793314573309132, 7.829454515125894964, 1.599625672291263179 ) ) ;
#196261=CARTESIAN_POINT ( 'NONE',  ( 5.004368096775565711, 8.852530189631227842, -0.7216878364870458196 ) ) ;
#196263=CARTESIAN_POINT ( 'NONE',  ( -6.929625909916163451, 7.257187447756535903, 0.7216878364870317197 ) ) ;
#196269=CARTESIAN_POINT ( 'NONE',  ( 5.204350862799327793, 7.165104988056252289, -1.599625672291281386 ) ) ;
#196272=CARTESIAN_POINT ( 'NONE',  ( -4.921546165693497343, 4.882379070747932204, 0.5514684743740734252 ) ) ;
#196297=CARTESIAN_POINT ( 'NONE',  ( 4.812442952513422689, 8.115120723895499211, -0.8517184758452013282 ) ) ;
#196313=CARTESIAN_POINT ( 'NONE',  ( -5.733196416021622888, 7.293175961584016598, -1.208997762321398550 ) ) ;
#196320=CARTESIAN_POINT ( 'NONE',  ( -4.543390873910949423, 6.393985001019784953, 1.443375672974058777 ) ) ;
#196331=CARTESIAN_POINT ( 'NONE',  ( -5.666381855868691808, 5.575476684793721383, 0.000000000000000000 ) ) ;
#196343=CARTESIAN_POINT ( 'NONE',  ( 5.367048706163317640, 7.354919138647580290, -1.599625672291281386 ) ) ;
#196347=CARTESIAN_POINT ( 'NONE',  ( 6.414416072596830887, 8.576847732820027659, -1.443375672974078761 ) ) ;
#196361=CARTESIAN_POINT ( 'NONE',  ( -5.743814354044916470, 6.730146830254374990, -1.199719254218453823 ) ) ;
#196362=CARTESIAN_POINT ( 'NONE',  ( 3.867818961648523235, 7.734482231890414283, 1.040834085586084257E-14 ) ) ;
#196370=ORIENTED_EDGE ( 'NONE', *, *, #40535, .F. ) ;
#196373=CARTESIAN_POINT ( 'NONE',  ( -5.589704470584107909, 9.743348658981940247, -0.7998128361456362523 ) ) ;
#196374=CARTESIAN_POINT ( 'NONE',  ( 5.345657705538078730, 9.458627433094950021, 0.7998128361456331437 ) ) ;
#196379=ORIENTED_EDGE ( 'NONE', *, *, #189556, .T. ) ;
#196380=CARTESIAN_POINT ( 'NONE',  ( 5.065906673361608270, 5.939254536123854677, -1.199719254218450271 ) ) ;
#196387=CARTESIAN_POINT ( 'NONE',  ( -6.065932567686177279, 7.134227558401057934, 1.164772332933713184 ) ) ;
#196396=CARTESIAN_POINT ( 'NONE',  ( -8.093291352714894415, 8.406871097780989288, -0.7998128361456362523 ) ) ;
#196444=CARTESIAN_POINT ( 'NONE',  ( 4.523580528814945545, 5.306540700819438960, 1.199719254218452047 ) ) ;
#196447=CARTESIAN_POINT ( 'NONE',  ( -4.014622883422336308, 5.777089012116397804, -1.443375672974066548 ) ) ;
#196460=EDGE_CURVE ( 'NONE', #118760, #49550, #106663, .T. ) ;
#196475=ORIENTED_EDGE ( 'NONE', *, *, #65745, .F. ) ;
#196476=CARTESIAN_POINT ( 'NONE',  ( -6.252245114557387851, 7.323316050852266557, -1.199719254218453823 ) ) ;
#196478=CARTESIAN_POINT ( 'NONE',  ( 6.333067150914808430, 8.481940657524365434, 1.443375672974063439 ) ) ;
#196483=CARTESIAN_POINT ( 'NONE',  ( -6.306477729012051725, 7.386587434382707151, 1.199719254218452047 ) ) ;
#196491=CARTESIAN_POINT ( 'NONE',  ( -6.622231685632140596, 6.690634819517756959, 0.000000000000000000 ) ) ;
#196504=CARTESIAN_POINT ( 'NONE',  ( -5.960744811863571968, 6.983232364376142698, 1.199719254218452935 ) ) ;
#196507=CARTESIAN_POINT ( 'NONE',  ( -5.478903473698247595, 8.445785581739666981, -1.082531754730549967 ) ) ;
#196509=CARTESIAN_POINT ( 'NONE',  ( -7.580417283372126391, 8.016444050121833698, 0.7216878364870317197 ) ) ;
#196510=CARTESIAN_POINT ( 'NONE',  ( 7.147083253059300922, 8.367293879104554577, 1.199719254218452935 ) ) ;
#196511=CARTESIAN_POINT ( 'NONE',  ( -7.957709816578236506, 8.248692638954882028, 0.7998128361456341429 ) ) ;
#196530=CARTESIAN_POINT ( 'NONE',  ( -1.842580630436563949, 2.498881177628073491, -2.492971354622253610 ) ) ;
#196537=DIRECTION ( 'NONE',  ( 0.000000000000000000, 0.000000000000000000, -1.000000000000000000 ) ) ;
#196549=CARTESIAN_POINT ( 'NONE',  ( 6.229241538080760421, 6.920885192246182704, -0.8282608007674150397 ) ) ;
#196566=CARTESIAN_POINT ( 'NONE',  ( -3.980200614063634568, 6.801261928786307642, 1.199719254218452935 ) ) ;
#196580=CARTESIAN_POINT ( 'NONE',  ( 4.064412189046650248, 7.963840997188264659, 0.7998128361456271485 ) ) ;
#196582=CARTESIAN_POINT ( 'NONE',  ( 5.169401708560450004, 9.252995436621013425, 0.000000000000000000 ) ) ;
#196595=CARTESIAN_POINT ( 'NONE',  ( 6.723917837734620484, 6.809268663637336516, 0.000000000000000000 ) ) ;
#196610=CARTESIAN_POINT ( 'NONE',  ( -6.482206841109545259, 6.735198534148810090, 0.7216878364870257245 ) ) ;
#196611=CARTESIAN_POINT ( 'NONE',  ( 6.075462232699553766, 6.260663157670496304, -0.7216878364870458196 ) ) ;
#196622=CARTESIAN_POINT ( 'NONE',  ( -6.509323148336870091, 7.727203440215372865, 1.082531754730549078 ) ) ;
#196626=CARTESIAN_POINT ( 'NONE',  ( 5.899206235277530297, 7.015400374979486209, -1.082531754730548412 ) ) ;
#196633=( BOUNDED_SURFACE ( )  B_SPLINE_SURFACE ( 3, 2, ( 
 ( #84385, #151533, #86518 ),
 ( #150472, #68102, #181865 ),
 ( #134238, #51896, #118019 ),
 ( #98510, #184008, #3101 ),
 ( #186137, #69172, #202374 ),
 ( #164572, #152583, #75609 ),
 ( #9535, #173126, #22565 ),
 ( #73462, #42063, #141720 ) ),
 .UNSPECIFIED., .F., .F., .T. ) 
 B_SPLINE_SURFACE_WITH_KNOTS ( ( 4, 2, 2, 4 ),
 ( 3, 3 ),
 ( 0.000000000000000000, 0.003124171923498968943, 0.004686257885248453631, 0.006248343846997937885 ),
 ( 0.000000000000000000, 1.000000000000000000 ),
 .UNSPECIFIED. ) 
 GEOMETRIC_REPRESENTATION_ITEM ( )  RATIONAL_B_SPLINE_SURFACE ( (
 ( 1.000000000000000000, 0.7762074382822432561, 1.000000000000000000),
 ( 1.000000000000000000, 0.7833327749266361106, 1.000000000000000000),
 ( 1.000000000000000000, 0.7920843030290980469, 1.000000000000000000),
 ( 1.000000000000000000, 0.8126253899334039410, 1.000000000000000000),
 ( 1.000000000000000000, 0.8207498793991692132, 1.000000000000000000),
 ( 1.000000000000000000, 0.8408199112011192078, 1.000000000000000000),
 ( 1.000000000000000000, 0.8529121798795707976, 1.000000000000000000),
 ( 1.000000000000000000, 0.8665632151524114146, 1.000000000000000000) ) ) 
 REPRESENTATION_ITEM ( '' )  SURFACE ( )  );
#196645=CARTESIAN_POINT ( 'NONE',  ( -5.503684012504701961, 5.385662534202396934, 0.000000000000000000 ) ) ;
#196656=CARTESIAN_POINT ( 'NONE',  ( 3.217027588192558074, 6.975225629525113824, -1.734723475976807094E-15 ) ) ;
#196658=CARTESIAN_POINT ( 'NONE',  ( -5.932574734431526942, 9.079031735882207244, 1.199719254218454489 ) ) ;
#196659=CARTESIAN_POINT ( 'NONE',  ( 6.367489420273535039, 7.457767740854454708, -1.199719254218452047 ) ) ;
#196668=CARTESIAN_POINT ( 'NONE',  ( -4.773352600463090845, 7.726605912919016106, 1.199719254218452935 ) ) ;
#196671=CARTESIAN_POINT ( 'NONE',  ( -0.3977480831933914440, 3.051780253777475860, 2.024501290749185056 ) ) ;
#196697=CARTESIAN_POINT ( 'NONE',  ( 4.584065335196260804, 6.441438539186039591, 1.443375672974065660 ) ) ;
#196703=CARTESIAN_POINT ( 'NONE',  ( 4.489158259456265121, 7.291082831790689056, -1.082531754730548412 ) ) ;
#196704=CARTESIAN_POINT ( 'NONE',  ( -4.285785955251283141, 8.014184357852876417, 0.000000000000000000 ) ) ;
#196714=CARTESIAN_POINT ( 'NONE',  ( -5.498713818794216834, 8.572860667638675380, -1.199719254218452047 ) ) ;
#196716=CARTESIAN_POINT ( 'NONE',  ( -5.589704470584107909, 9.743348658981940247, -0.7998128361456362523 ) ) ;
#196724=CARTESIAN_POINT ( 'NONE',  ( 7.537407054554579489, 7.758339416593960536, 0.000000000000000000 ) ) ;
#196729=CARTESIAN_POINT ( 'NONE',  ( 4.913571454530422322, 8.125067815752732514, -1.031885869761673069 ) ) ;
#196730=CARTESIAN_POINT ( 'NONE',  ( -6.947627372360122955, 7.070263120700404968, 0.000000000000000000 ) ) ;
#196736=CARTESIAN_POINT ( 'NONE',  ( -6.644904684473536882, 6.925012684740138980, 0.7216878364870317197 ) ) ;
#196740=CARTESIAN_POINT ( 'NONE',  ( -4.586401103172829785, 8.572828063668767484, 0.7998128361456281477 ) ) ;
#196747=CARTESIAN_POINT ( 'NONE',  ( -5.329763783503577379, 6.351050847909847086, 1.082531754730549078 ) ) ;
#196757=CARTESIAN_POINT ( 'NONE',  ( -6.486624235763164492, 6.835203243035253173, 0.7121179707554707861 ) ) ;
#196761=CARTESIAN_POINT ( 'NONE',  ( -6.770317605177755382, 8.992066187497757213, 1.599625672291269396 ) ) ;
#196762=CARTESIAN_POINT ( 'NONE',  ( 5.435893244436359240, 5.306573304789342416, -0.7998128361456481317 ) ) ;
#196763=CARTESIAN_POINT ( 'NONE',  ( -5.875479466675803231, 7.948088359245467416, -1.599625672291271394 ) ) ;
#196787=CARTESIAN_POINT ( 'NONE',  ( -6.095272577795516789, 9.268845886473535245, 1.199719254218452047 ) ) ;
#196812=CARTESIAN_POINT ( 'NONE',  ( 4.598150373690133463, 5.393538853173795111, -1.199719254218452047 ) ) ;
#196814=( BOUNDED_SURFACE ( )  B_SPLINE_SURFACE ( 1, 2, ( 
 ( #84065, #150155, #13732, #1724, #148023, #48404, #66713, #67781, #133931, #31082, #647, #79805, #129720, #117708, #100320, #183699, #65658, #33190, #165321, #63563, #211929, #199936, #163210, #145917, #64628, #131805, #195704, #214033, #96089, #51583, #113453, #15853, #197815, #49447, #146973, #14792, #130767, #196762, #82995, #80883, #212990, #198862, #114517, #180512, #32132, #164264, #115566, #181562, #99273, #81939, #132857, #16915, #149070, #50509, #116631, #20118, #136032, #152275, #151220, #36375, #37448, #123078, #86203, #103526, #203129, #169585, #21168, #121992, #23315, #101384, #70988, #72059, #134979, #184748, #102453, #104601, #39585, #54772, #35307, #87271, #153339, #119837, #187958, #167458, #4911, #185817, #168519, #118763, #105688, #73130, #202045, #3848, #137101, #55836, #204180, #53705, #155473, #120919, #69921, #138170, #19054, #186892, #171716, #85133, #200989, #52635, #68860, #139233, #170648, #7057, #2788, #22234, #38524, #154410, #88346, #5989, #205264, #89423, #56905, #60101, #124133, #156552, #210616, #191152, #208466, #125190, #92637, #160812, #8147, #159740, #74230, #94765, #126260, #140324, #91568, #90489, #57969, #93699, #158678, #10276, #142458, #192218, #206342, #144601, #209530, #25461, #176007, #24375, #143534, #108925, #43881, #40673, #207413, #11338, #177062, #61172, #76351, #173886, #27599, #157621, #190094, #41748, #42820, #9218, #107859, #75290, #193302, #141405, #78484, #77419, #59032, #174947, #26529, #109995, #127333, #44947, #111055, #28678, #12403, #62243, #189035, #106776, #172804, #64374, #146721, #164021, #147768, #97963, #112132, #32938, #13478, #194369, #161891, #14532, #113196, #80629, #30826, #29750, #129466, #130520, #1466, #179201, #196510, #81682, #48152, #114266, #391, #116376, #46012, #15595, #165069, #79554, #63305, #195449, #197556, #132604, #213784, #128402, #180262, #31886, #212738, #66463, #178135, #65407, #131554, #47078, #211669, #198610, #166130, #49200, #96903, #115321, #148819, #82746, #181311, #33994, #99012, #162954, #16661, #95834, #50256 ),
 ( #100068, #145672, #182364, #17717, #83805, #149898, #133674, #187707, #35048, #70733, #153085, #2531, #101119, #89174, #69674, #87013, #3597, #185567, #39335, #167206, #38268, #18795, #105432, #4661, #84879, #184499, #183444, #150967, #186642, #37197, #103271, #20918, #136846, #68607, #23057, #88088, #118515, #54519, #117450, #21978, #201803, #202871, #199679, #85953, #104345, #55585, #154160, #169334, #52387, #5727, #137917, #134730, #120664, #71806, #203937, #170389, #121740, #171468, #119583, #200737, #51322, #135780, #36118, #102201, #168268, #155226, #67531, #19868, #152028, #53445, #174699, #76101, #59851, #209275, #188782, #25210, #143284, #126003, #60921, #92390, #206089, #108671, #26273, #91314, #158426, #107606, #56659, #40419, #207163, #10026, #72885, #77163, #8965, #109745, #123882, #157371, #138992, #41493, #27347, #122822, #75039, #176808, #6807, #189847, #43630, #110803, #141155, #173637, #106522, #94517, #28424, #172548, #127079, #58786, #159487, #124942, #190904, #42568, #142204, #24133, #193042, #208219, #191964, #175755, #44696, #205013, #90235, #156301, #93449, #11086, #7884, #73972, #140067, #57724, #65163, #12163, #194113, #182114, #98764, #33744, #130272, #97712, #15348, #128153, #61997, #32684, #29498, #210358, #129221, #196261, #45763, #212487, #160555, #50003, #148578, #80373, #64129, #47908, #211424, #16411, #195195, #46832, #147519, #78234, #111881, #162706, #114018, #177885, #132361, #197311, #144357, #115070, #95590, #161639, #13234, #79307, #146468, #145423, #131318, #63054, #112945, #178957, #30572, #96653, #14278, #180014, #31635, #163770, #81441, #213540, #48952, #181066, #164820, #82491, #147, #66213, #198363, #116127, #138461, #139537, #199428, #34800, #100875, #172021, #107077, #56133, #190383, #170937, #22537, #187185, #40968, #99822, #88645, #38812, #166962, #183194, #189327, #140624, #55066, #2280, #154703, #123362, #57202, #200492, #8433, #104898, #18552, #205562, #165888, #84629, #173099, #17473, #51071, #117196, #133422, #206636, #23614, #74521, #83557, #89722, #134489 ) ),
 .UNSPECIFIED., .F., .F., .T. ) 
 B_SPLINE_SURFACE_WITH_KNOTS ( ( 2, 2 ),
 ( 3, 2, 2, 2, 2, 2, 2, 2, 2, 2, 2, 2, 2, 2, 2, 2, 2, 2, 2, 2, 2, 2, 2, 2, 2, 2, 2, 2, 2, 2, 2, 2, 2, 2, 2, 2, 2, 2, 2, 2, 2, 2, 2, 2, 2, 2, 2, 2, 2, 2, 2, 2, 2, 2, 2, 2, 2, 2, 2, 2, 2, 2, 2, 2, 2, 2, 2, 2, 2, 2, 2, 2, 2, 2, 2, 2, 2, 2, 2, 2, 2, 2, 2, 2, 2, 2, 2, 2, 2, 2, 2, 2, 2, 2, 2, 2, 2, 2, 2, 2, 2, 2, 2, 2, 2, 2, 2, 2, 2, 2, 2, 2, 2, 2, 2, 2, 2, 2, 2, 2, 3 ),
 ( 0.000000000000000000, 1.000000000000000000 ),
 ( 0.000000000000000000, 0.008333333333333333218, 0.01666666666666666644, 0.02500000000000000139, 0.03333333333333333287, 0.04166666666666666435, 0.05000000000000000278, 0.05833333333333333426, 0.06666666666666666574, 0.07499999999999999722, 0.08333333333333332871, 0.09166666666666666019, 0.1000000000000000056, 0.1083333333333333370, 0.1166666666666666685, 0.1250000000000000000, 0.1333333333333333315, 0.1416666666666666630, 0.1499999999999999944, 0.1583333333333333259, 0.1666666666666666574, 0.1749999999999999889, 0.1833333333333333204, 0.1916666666666666796, 0.2000000000000000111, 0.2083333333333333426, 0.2166666666666666741, 0.2250000000000000056, 0.2333333333333333370, 0.2416666666666666685, 0.2500000000000000000, 0.2583333333333333592, 0.2666666666666666630, 0.2750000000000000222, 0.2833333333333333259, 0.2916666666666666852, 0.2999999999999999889, 0.3083333333333333481, 0.3166666666666666519, 0.3250000000000000111, 0.3333333333333333148, 0.3416666666666666741, 0.3499999999999999778, 0.3583333333333333370, 0.3666666666666666408, 0.3750000000000000000, 0.3833333333333333592, 0.3916666666666666630, 0.4000000000000000222, 0.4083333333333333259, 0.4166666666666666852, 0.4249999999999999889, 0.4333333333333333481, 0.4416666666666666519, 0.4500000000000000111, 0.4583333333333333148, 0.4666666666666666741, 0.4749999999999999778, 0.4833333333333333370, 0.4916666666666666408, 0.5000000000000000000, 0.5083333333333333037, 0.5166666666666667185, 0.5250000000000000222, 0.5333333333333333259, 0.5416666666666666297, 0.5500000000000000444, 0.5583333333333333481, 0.5666666666666666519, 0.5749999999999999556, 0.5833333333333333703, 0.5916666666666666741, 0.5999999999999999778, 0.6083333333333332815, 0.6166666666666666963, 0.6250000000000000000, 0.6333333333333333037, 0.6416666666666667185, 0.6500000000000000222, 0.6583333333333333259, 0.6666666666666666297, 0.6750000000000000444, 0.6833333333333333481, 0.6916666666666666519, 0.6999999999999999556, 0.7083333333333333703, 0.7166666666666666741, 0.7249999999999999778, 0.7333333333333332815, 0.7416666666666666963, 0.7500000000000000000, 0.7583333333333333037, 0.7666666666666667185, 0.7750000000000000222, 0.7833333333333333259, 0.7916666666666666297, 0.8000000000000000444, 0.8083333333333333481, 0.8166666666666666519, 0.8249999999999999556, 0.8333333333333333703, 0.8416666666666666741, 0.8499999999999999778, 0.8583333333333332815, 0.8666666666666666963, 0.8750000000000000000, 0.8833333333333333037, 0.8916666666666667185, 0.9000000000000000222, 0.9083333333333333259, 0.9166666666666666297, 0.9250000000000000444, 0.9333333333333333481, 0.9416666666666666519, 0.9499999999999999556, 0.9583333333333333703, 0.9666666666666666741, 0.9749999999999999778, 0.9833333333333332815, 0.9916666666666666963, 1.000000000000000000 ),
 .UNSPECIFIED. ) 
 GEOMETRIC_REPRESENTATION_ITEM ( )  RATIONAL_B_SPLINE_SURFACE ( (
 ( 1.000000000000000000, 0.8660254037844387076, 1.000000000000000000, 0.8660254037844387076, 1.000000000000000000, 0.8660254037844387076, 1.000000000000000000, 0.8660254037844387076, 1.000000000000000000, 0.8660254037844387076, 1.000000000000000000, 0.8660254037844387076, 1.000000000000000000, 0.8660254037844387076, 1.000000000000000000, 0.8660254037844387076, 1.000000000000000000, 0.8660254037844387076, 1.000000000000000000, 0.8660254037844387076, 1.000000000000000000, 0.8660254037844387076, 1.000000000000000000, 0.8660254037844387076, 1.000000000000000000, 0.8660254037844387076, 1.000000000000000000, 0.8660254037844387076, 1.000000000000000000, 0.8660254037844387076, 1.000000000000000000, 0.8660254037844387076, 1.000000000000000000, 0.8660254037844387076, 1.000000000000000000, 0.8660254037844387076, 1.000000000000000000, 0.8660254037844387076, 1.000000000000000000, 0.8660254037844387076, 1.000000000000000000, 0.8660254037844387076, 1.000000000000000000, 0.8660254037844387076, 1.000000000000000000, 0.8660254037844387076, 1.000000000000000000, 0.8660254037844387076, 1.000000000000000000, 0.8660254037844387076, 1.000000000000000000, 0.8660254037844387076, 1.000000000000000000, 0.8660254037844387076, 1.000000000000000000, 0.8660254037844387076, 1.000000000000000000, 0.8660254037844387076, 1.000000000000000000, 0.8660254037844387076, 1.000000000000000000, 0.8660254037844387076, 1.000000000000000000, 0.8660254037844387076, 1.000000000000000000, 0.8660254037844387076, 1.000000000000000000, 0.8660254037844387076, 1.000000000000000000, 0.8660254037844387076, 1.000000000000000000, 0.8660254037844387076, 1.000000000000000000, 0.8660254037844387076, 1.000000000000000000, 0.8660254037844387076, 1.000000000000000000, 0.8660254037844387076, 1.000000000000000000, 0.8660254037844387076, 1.000000000000000000, 0.8660254037844387076, 1.000000000000000000, 0.8660254037844387076, 1.000000000000000000, 0.8660254037844387076, 1.000000000000000000, 0.8660254037844387076, 1.000000000000000000, 0.8660254037844387076, 1.000000000000000000, 0.8660254037844387076, 1.000000000000000000, 0.8660254037844387076, 1.000000000000000000, 0.8660254037844387076, 1.000000000000000000, 0.8660254037844387076, 1.000000000000000000, 0.8660254037844387076, 1.000000000000000000, 0.8660254037844387076, 1.000000000000000000, 0.8660254037844387076, 1.000000000000000000, 0.8660254037844387076, 1.000000000000000000, 0.8660254037844387076, 1.000000000000000000, 0.8660254037844387076, 1.000000000000000000, 0.8660254037844387076, 1.000000000000000000, 0.8660254037844387076, 1.000000000000000000, 0.8660254037844387076, 1.000000000000000000, 0.8660254037844387076, 1.000000000000000000, 0.8660254037844387076, 1.000000000000000000, 0.8660254037844387076, 1.000000000000000000, 0.8660254037844387076, 1.000000000000000000, 0.8660254037844387076, 1.000000000000000000, 0.8660254037844387076, 1.000000000000000000, 0.8660254037844387076, 1.000000000000000000, 0.8660254037844387076, 1.000000000000000000, 0.8660254037844387076, 1.000000000000000000, 0.8660254037844387076, 1.000000000000000000, 0.8660254037844387076, 1.000000000000000000, 0.8660254037844387076, 1.000000000000000000, 0.8660254037844387076, 1.000000000000000000, 0.8660254037844387076, 1.000000000000000000, 0.8660254037844387076, 1.000000000000000000, 0.8660254037844387076, 1.000000000000000000, 0.8660254037844387076, 1.000000000000000000, 0.8660254037844387076, 1.000000000000000000, 0.8660254037844387076, 1.000000000000000000, 0.8660254037844387076, 1.000000000000000000, 0.8660254037844387076, 1.000000000000000000, 0.8660254037844387076, 1.000000000000000000, 0.8660254037844387076, 1.000000000000000000, 0.8660254037844387076, 1.000000000000000000, 0.8660254037844387076, 1.000000000000000000, 0.8660254037844387076, 1.000000000000000000, 0.8660254037844387076, 1.000000000000000000, 0.8660254037844387076, 1.000000000000000000, 0.8660254037844387076, 1.000000000000000000, 0.8660254037844387076, 1.000000000000000000, 0.8660254037844387076, 1.000000000000000000, 0.8660254037844387076, 1.000000000000000000, 0.8660254037844387076, 1.000000000000000000, 0.8660254037844387076, 1.000000000000000000, 0.8660254037844387076, 1.000000000000000000, 0.8660254037844387076, 1.000000000000000000, 0.8660254037844387076, 1.000000000000000000, 0.8660254037844387076, 1.000000000000000000, 0.8660254037844387076, 1.000000000000000000, 0.8660254037844387076, 1.000000000000000000, 0.8660254037844387076, 1.000000000000000000, 0.8660254037844387076, 1.000000000000000000, 0.8660254037844387076, 1.000000000000000000, 0.8660254037844387076, 1.000000000000000000, 0.8660254037844387076, 1.000000000000000000, 0.8660254037844387076, 1.000000000000000000, 0.8660254037844387076, 1.000000000000000000, 0.8660254037844387076, 1.000000000000000000, 0.8660254037844387076, 1.000000000000000000, 0.8660254037844387076, 1.000000000000000000, 0.8660254037844387076, 1.000000000000000000, 0.8660254037844387076, 1.000000000000000000, 0.8660254037844387076, 1.000000000000000000, 0.8660254037844387076, 1.000000000000000000, 0.8660254037844387076, 1.000000000000000000, 0.8660254037844387076, 1.000000000000000000, 0.8660254037844387076, 1.000000000000000000, 0.8660254037844387076, 1.000000000000000000, 0.8660254037844387076, 1.000000000000000000, 0.8660254037844387076, 1.000000000000000000, 0.8660254037844387076, 1.000000000000000000, 0.8660254037844387076, 1.000000000000000000),
 ( 1.000000000000000000, 0.8660254037844387076, 1.000000000000000000, 0.8660254037844387076, 1.000000000000000000, 0.8660254037844387076, 1.000000000000000000, 0.8660254037844387076, 1.000000000000000000, 0.8660254037844387076, 1.000000000000000000, 0.8660254037844387076, 1.000000000000000000, 0.8660254037844387076, 1.000000000000000000, 0.8660254037844387076, 1.000000000000000000, 0.8660254037844387076, 1.000000000000000000, 0.8660254037844387076, 1.000000000000000000, 0.8660254037844387076, 1.000000000000000000, 0.8660254037844387076, 1.000000000000000000, 0.8660254037844387076, 1.000000000000000000, 0.8660254037844387076, 1.000000000000000000, 0.8660254037844387076, 1.000000000000000000, 0.8660254037844387076, 1.000000000000000000, 0.8660254037844387076, 1.000000000000000000, 0.8660254037844387076, 1.000000000000000000, 0.8660254037844387076, 1.000000000000000000, 0.8660254037844387076, 1.000000000000000000, 0.8660254037844387076, 1.000000000000000000, 0.8660254037844387076, 1.000000000000000000, 0.8660254037844387076, 1.000000000000000000, 0.8660254037844387076, 1.000000000000000000, 0.8660254037844387076, 1.000000000000000000, 0.8660254037844387076, 1.000000000000000000, 0.8660254037844387076, 1.000000000000000000, 0.8660254037844387076, 1.000000000000000000, 0.8660254037844387076, 1.000000000000000000, 0.8660254037844387076, 1.000000000000000000, 0.8660254037844387076, 1.000000000000000000, 0.8660254037844387076, 1.000000000000000000, 0.8660254037844387076, 1.000000000000000000, 0.8660254037844387076, 1.000000000000000000, 0.8660254037844387076, 1.000000000000000000, 0.8660254037844387076, 1.000000000000000000, 0.8660254037844387076, 1.000000000000000000, 0.8660254037844387076, 1.000000000000000000, 0.8660254037844387076, 1.000000000000000000, 0.8660254037844387076, 1.000000000000000000, 0.8660254037844387076, 1.000000000000000000, 0.8660254037844387076, 1.000000000000000000, 0.8660254037844387076, 1.000000000000000000, 0.8660254037844387076, 1.000000000000000000, 0.8660254037844387076, 1.000000000000000000, 0.8660254037844387076, 1.000000000000000000, 0.8660254037844387076, 1.000000000000000000, 0.8660254037844387076, 1.000000000000000000, 0.8660254037844387076, 1.000000000000000000, 0.8660254037844387076, 1.000000000000000000, 0.8660254037844387076, 1.000000000000000000, 0.8660254037844387076, 1.000000000000000000, 0.8660254037844387076, 1.000000000000000000, 0.8660254037844387076, 1.000000000000000000, 0.8660254037844387076, 1.000000000000000000, 0.8660254037844387076, 1.000000000000000000, 0.8660254037844387076, 1.000000000000000000, 0.8660254037844387076, 1.000000000000000000, 0.8660254037844387076, 1.000000000000000000, 0.8660254037844387076, 1.000000000000000000, 0.8660254037844387076, 1.000000000000000000, 0.8660254037844387076, 1.000000000000000000, 0.8660254037844387076, 1.000000000000000000, 0.8660254037844387076, 1.000000000000000000, 0.8660254037844387076, 1.000000000000000000, 0.8660254037844387076, 1.000000000000000000, 0.8660254037844387076, 1.000000000000000000, 0.8660254037844387076, 1.000000000000000000, 0.8660254037844387076, 1.000000000000000000, 0.8660254037844387076, 1.000000000000000000, 0.8660254037844387076, 1.000000000000000000, 0.8660254037844387076, 1.000000000000000000, 0.8660254037844387076, 1.000000000000000000, 0.8660254037844387076, 1.000000000000000000, 0.8660254037844387076, 1.000000000000000000, 0.8660254037844387076, 1.000000000000000000, 0.8660254037844387076, 1.000000000000000000, 0.8660254037844387076, 1.000000000000000000, 0.8660254037844387076, 1.000000000000000000, 0.8660254037844387076, 1.000000000000000000, 0.8660254037844387076, 1.000000000000000000, 0.8660254037844387076, 1.000000000000000000, 0.8660254037844387076, 1.000000000000000000, 0.8660254037844387076, 1.000000000000000000, 0.8660254037844387076, 1.000000000000000000, 0.8660254037844387076, 1.000000000000000000, 0.8660254037844387076, 1.000000000000000000, 0.8660254037844387076, 1.000000000000000000, 0.8660254037844387076, 1.000000000000000000, 0.8660254037844387076, 1.000000000000000000, 0.8660254037844387076, 1.000000000000000000, 0.8660254037844387076, 1.000000000000000000, 0.8660254037844387076, 1.000000000000000000, 0.8660254037844387076, 1.000000000000000000, 0.8660254037844387076, 1.000000000000000000, 0.8660254037844387076, 1.000000000000000000, 0.8660254037844387076, 1.000000000000000000, 0.8660254037844387076, 1.000000000000000000, 0.8660254037844387076, 1.000000000000000000, 0.8660254037844387076, 1.000000000000000000, 0.8660254037844387076, 1.000000000000000000, 0.8660254037844387076, 1.000000000000000000, 0.8660254037844387076, 1.000000000000000000, 0.8660254037844387076, 1.000000000000000000, 0.8660254037844387076, 1.000000000000000000, 0.8660254037844387076, 1.000000000000000000, 0.8660254037844387076, 1.000000000000000000, 0.8660254037844387076, 1.000000000000000000, 0.8660254037844387076, 1.000000000000000000, 0.8660254037844387076, 1.000000000000000000, 0.8660254037844387076, 1.000000000000000000, 0.8660254037844387076, 1.000000000000000000, 0.8660254037844387076, 1.000000000000000000, 0.8660254037844387076, 1.000000000000000000, 0.8660254037844387076, 1.000000000000000000, 0.8660254037844387076, 1.000000000000000000, 0.8660254037844387076, 1.000000000000000000, 0.8660254037844387076, 1.000000000000000000, 0.8660254037844387076, 1.000000000000000000, 0.8660254037844387076, 1.000000000000000000) ) ) 
 REPRESENTATION_ITEM ( '' )  SURFACE ( )  );
#196825=CARTESIAN_POINT ( 'NONE',  ( 4.604167169973131912, 8.362045362587558373, -0.1994984680026238300 ) ) ;
#196827=CARTESIAN_POINT ( 'NONE',  ( 5.225741863424510747, 5.061396693608882558, 0.7998128361456352531 ) ) ;
#196833=CARTESIAN_POINT ( 'NONE',  ( -4.599959256786493533, 8.588645909551377855, 0.000000000000000000 ) ) ;
#196836=VERTEX_POINT ( 'NONE', #158622 ) ;
#196839=CARTESIAN_POINT ( 'NONE',  ( -6.089020385868856522, 9.157588645938716354, -1.082531754730549967 ) ) ;
#196843=CARTESIAN_POINT ( 'NONE',  ( -4.669816416521347158, 7.043937703794544092, 1.217519100783383212 ) ) ;
#196850=CARTESIAN_POINT ( 'NONE',  ( -5.646044625448194410, 5.551749915969804938, 0.000000000000000000 ) ) ;
#196858=CARTESIAN_POINT ( 'NONE',  ( 5.248941747146098180, 6.152795455539095570, -1.199719254218452047 ) ) ;
#196879=CARTESIAN_POINT ( 'NONE',  ( -5.752402313948099533, 9.933162809573264695, -0.7998128361456362523 ) ) ;
#196889=CARTESIAN_POINT ( 'NONE',  ( 4.746236293235721604, 7.694970221153795364, 1.199719254218451159 ) ) ;
#196896=CARTESIAN_POINT ( 'NONE',  ( 4.800995793014950941, 5.734154859006458160, -1.082531754730548412 ) ) ;
#196899=CARTESIAN_POINT ( 'NONE',  ( 7.024532985656136930, 8.328281583754568729, 1.082531754730549967 ) ) ;
#196907=LINE ( 'NONE', #45351, #39740 ) ;
#196910=CARTESIAN_POINT ( 'NONE',  ( -7.119440060951841787, 7.478637290631501067, 0.000000000000000000 ) ) ;
#196935=CARTESIAN_POINT ( 'NONE',  ( 5.594708818112484217, 5.774250729507365953, 0.6894988139244705438 ) ) ;
#196945=CARTESIAN_POINT ( 'NONE',  ( 6.204791576909545192, 7.267953590263130259, -1.199719254218452047 ) ) ;
#196947=CARTESIAN_POINT ( 'NONE',  ( 4.766573523656222555, 7.718696989977711809, 1.199719254218452047 ) ) ;
#196960=CARTESIAN_POINT ( 'NONE',  ( -7.024532985656169792, 9.288650798055913427, 1.443375672974064550 ) ) ;
#196963=CARTESIAN_POINT ( 'NONE',  ( 5.573810548549551491, 6.635772073796838200, -1.082531754730548412 ) ) ;
#196976=CARTESIAN_POINT ( 'NONE',  ( -6.617788377246196951, 7.853746207276256719, -1.082531754730549967 ) ) ;
#196978=CARTESIAN_POINT ( 'NONE',  ( -4.285785955695645910, 7.053815144069948140, 1.082531754730549967 ) ) ;
#196982=DIRECTION ( 'NONE',  ( 0.000000000000000000, 0.000000000000000000, -1.000000000000000000 ) ) ;
#196987=ADVANCED_FACE ( 'NONE', ( #3580 ), #32991, .T. ) ;
#196996=CARTESIAN_POINT ( 'NONE',  ( -3.135678666510573365, 6.880318554229450712, 0.000000000000000000 ) ) ;
#197007=CARTESIAN_POINT ( 'NONE',  ( -5.330290668828105538, 6.247702530834755130, 1.199719254218452935 ) ) ;
#197008=CARTESIAN_POINT ( 'NONE',  ( -5.607373391640464888, 5.677249416569920548, -0.2774322056599042852 ) ) ;
#197010=CARTESIAN_POINT ( 'NONE',  ( 5.427194451788625251, 7.548169490501462242, -1.275334042231127230 ) ) ;
#197016=CARTESIAN_POINT ( 'NONE',  ( -7.533490631048818109, 8.818102486758951031, -1.199719254218452047 ) ) ;
#197017=CARTESIAN_POINT ( 'NONE',  ( -5.426384371074921553, 7.636973626576035734, -1.343385757368668498 ) ) ;
#197021=CARTESIAN_POINT ( 'NONE',  ( -6.238160075619175515, 10.29195416494877513, 0.000000000000000000 ) ) ;
#197036=CARTESIAN_POINT ( 'NONE',  ( 7.374709211190586089, 7.568525266002632534, 0.000000000000000000 ) ) ;
#197059=CARTESIAN_POINT ( 'NONE',  ( 6.801350335910821165, 7.963938809097990124, 1.199719254218452047 ) ) ;
#197060=CARTESIAN_POINT ( 'NONE',  ( 6.333594036239346359, 7.418223126147930557, 1.199719254218453823 ) ) ;
#197062=CARTESIAN_POINT ( 'NONE',  ( 5.225741863424510747, 5.061396693608882558, 0.7998128361456352531 ) ) ;
#197074=CARTESIAN_POINT ( 'NONE',  ( 4.597299534708283453, 8.487268731053720927, 0.09294953129799360392 ) ) ;
#197076=CARTESIAN_POINT ( 'NONE',  ( -6.414416072596857532, 6.656109304217339151, -0.7216878364870338292 ) ) ;
#197077=CARTESIAN_POINT ( 'NONE',  ( 5.912764389335563919, 6.070849007079172743, -0.7216878364870458196 ) ) ;
#197098=CARTESIAN_POINT ( 'NONE',  ( 4.369470645354133431, 8.319742529546998000, 0.7998128361456271485 ) ) ;
#197100=CARTESIAN_POINT ( 'NONE',  ( 5.435893244436359240, 5.306573304789342416, -0.7998128361456481317 ) ) ;
#197121=CARTESIAN_POINT ( 'NONE',  ( -5.610041701004606196, 9.767075427805856691, -0.7998128361456362523 ) ) ;
#197131=CARTESIAN_POINT ( 'NONE',  ( 5.987861119090863049, 7.014868056141362551, 1.199719254218452047 ) ) ;
#197135=CARTESIAN_POINT ( 'NONE',  ( 5.956828388357757298, 8.042995434541133193, 1.599625672291269396 ) ) ;
#197147=CARTESIAN_POINT ( 'NONE',  ( 4.615647837050825153, 8.347533190886938570, 0.2882115401751338402 ) ) ;
#197162=CARTESIAN_POINT ( 'NONE',  ( 0.000000000000000000, 2.480000000000016858, 0.000000000000000000 ) ) ;
#197170=CARTESIAN_POINT ( 'NONE',  ( -5.284646014276622950, 9.387447126623207794, -0.7998128361456362523 ) ) ;
#197172=CARTESIAN_POINT ( 'NONE',  ( 5.417364897112183719, 8.477953592343014932, 1.199719254218451159 ) ) ;
#197174=CARTESIAN_POINT ( 'NONE',  ( 3.840479349152599919, 7.346192795665340114, 0.4818892653144311033 ) ) ;
#197183=CARTESIAN_POINT ( 'NONE',  ( -0.4135277324232147222, 2.752648330311642688, -1.957052666557069109 ) ) ;
#197194=CARTESIAN_POINT ( 'NONE',  ( 1.806654366501771136, 2.518449987798942136, 2.499999999999998668 ) ) ;
#197199=CARTESIAN_POINT ( 'NONE',  ( 7.214347136247488912, 7.589362211809770997, -0.7216878364870317197 ) ) ;
#197205=LINE ( 'NONE', #30465, #180934 ) ;
#197213=CARTESIAN_POINT ( 'NONE',  ( -5.153507786970285665, 5.185049637652990207, -0.7216878364870338292 ) ) ;
#197215=CARTESIAN_POINT ( 'NONE',  ( 5.306037014901791693, 7.283738832175834510, 1.599625672291269396 ) ) ;
#197219=CARTESIAN_POINT ( 'NONE',  ( -5.354544322754380303, 5.211666229493680191, 0.7998128361456281477 ) ) ;
#197229=VERTEX_POINT ( 'NONE', #67120 ) ;
#197231=CARTESIAN_POINT ( 'NONE',  ( -0.2316791905390819806, 3.431749620889657848, -1.989589857879307866 ) ) ;
#197263=CARTESIAN_POINT ( 'NONE',  ( 3.878514461961128479, 6.682628084666728085, -1.199719254218448494 ) ) ;
#197269=CARTESIAN_POINT ( 'NONE',  ( -4.285785955251283141, 8.014184357852876417, 0.000000000000000000 ) ) ;
#197275=CARTESIAN_POINT ( 'NONE',  ( -6.961185525973791144, 7.086080966583015339, 0.7998128361456341429 ) ) ;
#197281=ORIENTED_EDGE ( 'NONE', *, *, #204645, .F. ) ;
#197285=CARTESIAN_POINT ( 'NONE',  ( -4.444040490229335560, 8.406740681901359480, 0.7998128361456352531 ) ) ;
#197287=EDGE_LOOP ( 'NONE', ( #83535, #107441, #43739 ) ) ;
#197288=CARTESIAN_POINT ( 'NONE',  ( 6.090086331970060662, 7.118959255344424086, 1.132899493623270359 ) ) ;
#197293=CARTESIAN_POINT ( 'NONE',  ( 6.801350335910821165, 7.963938809097990124, 1.199719254218452047 ) ) ;
#197299=CIRCLE ( 'NONE', #10519, 0.7500000000000011102 ) ;
#197302=CARTESIAN_POINT ( 'NONE',  ( -4.411198876399886615, 6.239761003923544713, -1.599625672291271394 ) ) ;
#197307=CARTESIAN_POINT ( 'NONE',  ( -6.343235766347277149, 8.493804042195527870, -1.599625672291271394 ) ) ;
#197311=CARTESIAN_POINT ( 'NONE',  ( 7.173672674962134899, 7.541908673643526129, -0.7216878364870317197 ) ) ;
#197313=CARTESIAN_POINT ( 'NONE',  ( -5.587368702163209910, 9.532697562583475559, 0.000000000000000000 ) ) ;
#197319=ADVANCED_FACE ( 'NONE', ( #22637 ), #65791, .T. ) ;
#197320=CARTESIAN_POINT ( 'NONE',  ( 5.611095471209277541, 7.639640364534566075, 1.599625672291268286 ) ) ;
#197328=CARTESIAN_POINT ( 'NONE',  ( -2.978872658371960025, 6.473523904506141236, -0.4823651620584931687 ) ) ;
#197360=CARTESIAN_POINT ( 'NONE',  ( -4.934256961717153445, 8.002024883745839645, -1.000413331142641526 ) ) ;
#197363=ADVANCED_FACE ( 'NONE', ( #98632 ), #138363, .T. ) ;
#197379=CARTESIAN_POINT ( 'NONE',  ( -4.411198876399886615, 6.239761003923544713, -1.599625672291271394 ) ) ;
#197391=CARTESIAN_POINT ( 'NONE',  ( 5.391302360089590628, 6.318882837306503575, -1.199719254218452047 ) ) ;
#197394=CARTESIAN_POINT ( 'NONE',  ( 6.007671464186825183, 8.102312356341712984, 1.443375672974064550 ) ) ;
#197409=CARTESIAN_POINT ( 'NONE',  ( -5.611095471209320174, 7.639640364534566075, 1.599625672291263179 ) ) ;
#197410=CARTESIAN_POINT ( 'NONE',  ( 4.553559489343365740, 6.405848385690952718, -1.599625672291269396 ) ) ;
#197419=CARTESIAN_POINT ( 'NONE',  ( -4.787964524281469458, 5.614988695530339413, -1.199719254218453823 ) ) ;
#197420=CARTESIAN_POINT ( 'NONE',  ( 6.879836604291781121, 6.991173891287354003, -0.7998128361456341429 ) ) ;
#197427=CARTESIAN_POINT ( 'NONE',  ( 4.228163802615382494, 6.026220084508304708, -1.599625672291269396 ) ) ;
#197431=CARTESIAN_POINT ( 'NONE',  ( -0.3265810047278985828, 2.653141922745489989, 1.973618857176524521 ) ) ;
#197435=CARTESIAN_POINT ( 'NONE',  ( -5.840188366348757931, 7.302172906674928576, 1.289283945506283890 ) ) ;
#197445=CARTESIAN_POINT ( 'NONE',  ( -4.963693635934603776, 4.963599794778024155, 0.000000000000000000 ) ) ;
#197457=FACE_OUTER_BOUND ( 'NONE', #137996, .T. ) ;
#197474=CARTESIAN_POINT ( 'NONE',  ( 5.682802662783380754, 6.658966523782627434, 1.199719254218452935 ) ) ;
#197495=CARTESIAN_POINT ( 'NONE',  ( 4.913904330310220558, 4.697586238308844919, 0.000000000000000000 ) ) ;
#197496=CARTESIAN_POINT ( 'NONE',  ( -3.011319516011047082, 6.527306845405913549, 0.7216878364870328300 ) ) ;
#197510=LINE ( 'NONE', #120619, #140078 ) ;
#197522=CARTESIAN_POINT ( 'NONE',  ( -4.630991987519598396, 7.560518531151607213, 1.199719254218452935 ) ) ;
#197524=CARTESIAN_POINT ( 'NONE',  ( 7.485510208076452621, 7.905719128943566432, 0.000000000000000000 ) ) ;
#197529=CARTESIAN_POINT ( 'NONE',  ( -5.284646014276622950, 9.387447126623207794, -0.7998128361456362523 ) ) ;
#197537=CARTESIAN_POINT ( 'NONE',  ( -7.110325215724114578, 7.260077271291732082, 0.000000000000000000 ) ) ;
#197549=CARTESIAN_POINT ( 'NONE',  ( -4.125423880308188629, 8.035021303660014880, -0.7998128361456481317 ) ) ;
#197553=CARTESIAN_POINT ( 'NONE',  ( -7.946487431385463651, 8.443525889470736345, 0.7216878364870317197 ) ) ;
#197555=CARTESIAN_POINT ( 'NONE',  ( -7.715998819508785189, 8.174622508947939181, -0.7216878364870338292 ) ) ;
#197556=CARTESIAN_POINT ( 'NONE',  ( 7.309781096423290769, 8.557108029695882578, 1.199719254218452935 ) ) ;
#197557=CARTESIAN_POINT ( 'NONE',  ( -5.451787166026575981, 5.533042246551999277, 0.000000000000000000 ) ) ;
#197578=CARTESIAN_POINT ( 'NONE',  ( 6.395636025722083673, 6.905704815116233242, -0.7835738547974178125 ) ) ;
#197598=CARTESIAN_POINT ( 'NONE',  ( 5.954584599377941601, 7.113081392617206511, -1.094866876611422235 ) ) ;
#197610=CARTESIAN_POINT ( 'NONE',  ( 6.770317605177710085, 8.992066187497757213, 1.599625672291268286 ) ) ;
#197613=CARTESIAN_POINT ( 'NONE',  ( -3.467853430045390706, 7.267855778353407459, 0.7998128361456352531 ) ) ;
#197617=CARTESIAN_POINT ( 'NONE',  ( -7.146556367734805626, 9.431011410480991231, 1.443375672974064550 ) ) ;
#197627=CARTESIAN_POINT ( 'NONE',  ( 3.223806664999388172, 6.983134552466421674, -0.7998128361456362523 ) ) ;
#197629=CARTESIAN_POINT ( 'NONE',  ( 6.047819040147648373, 9.213483425884394507, 1.199719254218452047 ) ) ;
#197633=CARTESIAN_POINT ( 'NONE',  ( 0.000000000000000000, 8.920000000000001705, 0.000000000000000000 ) ) ;
#197637=CARTESIAN_POINT ( 'NONE',  ( -5.438229012412888252, 9.358701257874761481, -0.7216878364870338292 ) ) ;
#197645=CARTESIAN_POINT ( 'NONE',  ( 7.537407054554579489, 7.758339416593960536, 0.000000000000000000 ) ) ;
#197657=CARTESIAN_POINT ( 'NONE',  ( -5.641601317062239218, 8.635599732330991429, -1.082531754730549967 ) ) ;
#197658=CARTESIAN_POINT ( 'NONE',  ( 4.394251184604957672, 8.140727125432173139, -0.7216878364870357165 ) ) ;
#197669=CARTESIAN_POINT ( 'NONE',  ( -7.105881907338178038, 7.462819444748888920, -0.7216878364870338292 ) ) ;
#197670=CARTESIAN_POINT ( 'NONE',  ( 7.309781096423290769, 8.557108029695882578, 1.199719254218452935 ) ) ;
#197674=CARTESIAN_POINT ( 'NONE',  ( 6.197485614778188712, 6.403023770095574108, -0.7216878364870458196 ) ) ;
#197691=EDGE_CURVE ( 'NONE', #93524, #17896, #139641, .T. ) ;
#197692=CARTESIAN_POINT ( 'NONE',  ( -4.679499295372141709, 5.488445928469455559, 1.199719254218452935 ) ) ;
#197705=CARTESIAN_POINT ( 'NONE',  ( 4.740510986633625024, 5.559626234941203116, -1.199719254218450271 ) ) ;
#197708=CARTESIAN_POINT ( 'NONE',  ( 5.071631979963703962, 8.074598522336444262, 1.199719254218451159 ) ) ;
#197715=CARTESIAN_POINT ( 'NONE',  ( -4.261005416444848315, 8.193199762486115034, 0.7998128361456352531 ) ) ;
#197740=CARTESIAN_POINT ( 'NONE',  ( 5.527114335400765910, 5.971691288924419361, -0.7760601246002347686 ) ) ;
#197741=ADVANCED_FACE ( 'NONE', ( #142891 ), #2378, .T. ) ;
#197744=CARTESIAN_POINT ( 'NONE',  ( 5.397554552016228691, 5.469770863539975991, 0.7216878364870328300 ) ) ;
#197745=ORIENTED_EDGE ( 'NONE', *, *, #81172, .T. ) ;
#197749=CARTESIAN_POINT ( 'NONE',  ( 4.411882113620712254, 5.024994294388632987, 0.9701603416667784474 ) ) ;
#197750=CARTESIAN_POINT ( 'NONE',  ( 5.194182247366869731, 7.153241603385088965, 1.443375672974064550 ) ) ;
#197762=CARTESIAN_POINT ( 'NONE',  ( -6.656127069666307072, 6.730179434224282886, 0.7998128361456341429 ) ) ;
#197764=CARTESIAN_POINT ( 'NONE',  ( -6.505933609711270549, 8.683618192786854095, -1.599625672291271394 ) ) ;
#197771=CARTESIAN_POINT ( 'NONE',  ( 5.677832469072920496, 9.846164657218904992, 0.000000000000000000 ) ) ;
#197776=CARTESIAN_POINT ( 'NONE',  ( -5.608682343087995292, 5.618096023427380459, 0.4395498943386428881 ) ) ;
#197777=CARTESIAN_POINT ( 'NONE',  ( -5.738844160334429567, 9.917344963690652548, 0.000000000000000000 ) ) ;
#197783=CARTESIAN_POINT ( 'NONE',  ( -5.478903473698255588, 7.485416367438324059, -1.443375672974066548 ) ) ;
#197787=CARTESIAN_POINT ( 'NONE',  ( -6.557303570864871034, 7.679217583210999010, -1.199719254218452047 ) ) ;
#197791=VECTOR ( 'NONE', #33810, 1000.000000000000000 ) ;
#197811=CARTESIAN_POINT ( 'NONE',  ( -4.014622883422336308, 5.777089012116397804, -1.443375672974066548 ) ) ;
#197813=CARTESIAN_POINT ( 'NONE',  ( -5.139949632912262700, 5.169231791251960750, 0.7216878364870257245 ) ) ;
#197815=CARTESIAN_POINT ( 'NONE',  ( 3.790386463472274148, 6.579812086429759788, 1.199719254218452047 ) ) ;
#197816=CARTESIAN_POINT ( 'NONE',  ( -4.471156797456668386, 8.438376373666578445, -0.7998128361456362523 ) ) ;
#197817=ORIENTED_EDGE ( 'NONE', *, *, #17110, .F. ) ;
#197827=ORIENTED_EDGE ( 'NONE', *, *, #141289, .F. ) ;
#197831=CARTESIAN_POINT ( 'NONE',  ( -5.521155831633614675, 5.981593978145122392, -0.9474053820182636310 ) ) ;
#197835=CARTESIAN_POINT ( 'NONE',  ( -5.717785742877127042, 7.006476535625795421, -2.500000000000000444 ) ) ;
#197864=CARTESIAN_POINT ( 'NONE',  ( 3.562760505341037831, 7.378580699531681830, -1.734723475976807094E-15 ) ) ;
#197878=CARTESIAN_POINT ( 'NONE',  ( 4.633164669693822901, 8.325607986553848150, 0.3865003237762173471 ) ) ;
#197881=CARTESIAN_POINT ( 'NONE',  ( 4.740510986633625024, 5.559626234941203116, -1.199719254218450271 ) ) ;
#197887=CARTESIAN_POINT ( 'NONE',  ( -4.586401103172829785, 8.572828063668767484, 0.7998128361456281477 ) ) ;
#197892=CARTESIAN_POINT ( 'NONE',  ( -8.054952659850432184, 8.570068656013202002, 0.000000000000000000 ) ) ;
#197901=CARTESIAN_POINT ( 'NONE',  ( -4.125423880308188629, 8.035021303660014880, -0.7998128361456481317 ) ) ;
#197912=CARTESIAN_POINT ( 'NONE',  ( 3.874598038455354665, 7.742391154831717692, -0.7998128361456362523 ) ) ;
#197930=CARTESIAN_POINT ( 'NONE',  ( 0.000000000000000000, 8.920000000000001705, 0.000000000000000000 ) ) ;
#197935=CARTESIAN_POINT ( 'NONE',  ( 5.257115172742783393, 7.717454145000224308, 1.254163143712288653 ) ) ;
#197938=CARTESIAN_POINT ( 'NONE',  ( 6.535912570239620578, 9.782925877658371405, 1.199719254218452047 ) ) ;
#197946=CARTESIAN_POINT ( 'NONE',  ( 7.503511670520385479, 7.718794801887437274, 0.7998128361456281477 ) ) ;
#197953=CARTESIAN_POINT ( 'NONE',  ( 5.126391479742934187, 6.113783160189109722, -1.082531754730548412 ) ) ;
#197956=CARTESIAN_POINT ( 'NONE',  ( 7.512626515748113576, 7.937354821227203594, 0.7216878364870267237 ) ) ;
#197966=CARTESIAN_POINT ( 'NONE',  ( -5.126391479742927970, 8.994890803093138487, 0.7216878364870267237 ) ) ;
#198004=CARTESIAN_POINT ( 'NONE',  ( 5.234329823327693809, 8.264412672927770487, 1.199719254218451159 ) ) ;
#198006=CARTESIAN_POINT ( 'NONE',  ( 5.875479466675786355, 7.948088359245467416, -1.599625672291283607 ) ) ;
#198019=CARTESIAN_POINT ( 'NONE',  ( -5.966997003790217136, 9.975597247814986801, -0.7216878364870338292 ) ) ;
#198022=CARTESIAN_POINT ( 'NONE',  ( 6.034787771414195312, 6.213209619504250547, -0.7216878364870458196 ) ) ;
#198030=CARTESIAN_POINT ( 'NONE',  ( -5.483346782084204563, 5.361935765378481378, 0.000000000000000000 ) ) ;
#198036=CARTESIAN_POINT ( 'NONE',  ( -5.614485009834902840, 9.564333254867113610, 0.7216878364870267237 ) ) ;
#198038=CARTESIAN_POINT ( 'NONE',  ( -4.584065335196305213, 6.441438539186039591, 1.443375672974058777 ) ) ;
#198053=CARTESIAN_POINT ( 'NONE',  ( -2.823841133396259639, 6.516508098929413961, -0.7998128361456481317 ) ) ;
#198064=CARTESIAN_POINT ( 'NONE',  ( -3.806807270387036368, 7.663301925418665839, 0.000000000000000000 ) ) ;
#198076=CARTESIAN_POINT ( 'NONE',  ( 5.345847655232874196, 4.689681438633019894, -2.440353607042919926 ) ) ;
#198077=CARTESIAN_POINT ( 'NONE',  ( -4.624683998644739447, 8.449116153850892985, -0.4091045222319161234 ) ) ;
#198080=ORIENTED_EDGE ( 'NONE', *, *, #197691, .F. ) ;
#198094=CARTESIAN_POINT ( 'NONE',  ( 6.119526231721748033, 8.232809585132461194, 1.599625672291269396 ) ) ;
#198100=CARTESIAN_POINT ( 'NONE',  ( -4.827585214917754719, 7.789877296449459365, -1.199719254218453823 ) ) ;
#198116=CARTESIAN_POINT ( 'NONE',  ( 6.855582950365507244, 8.027210192628430718, -1.199719254218452047 ) ) ;
#198117=CARTESIAN_POINT ( 'NONE',  ( 5.091969210384201361, 8.098325291160362482, 1.199719254218452047 ) ) ;
#198119=CARTESIAN_POINT ( 'NONE',  ( 3.528865121306874464, 7.339036084825155015, -0.7998128361456362523 ) ) ;
#198123=CARTESIAN_POINT ( 'NONE',  ( -6.278834536460208504, 6.497930845391227450, 0.7216878364870173979 ) ) ;
#198131=CARTESIAN_POINT ( 'NONE',  ( 5.088145468715395303, 7.830155539619080507, -1.136959649167136543 ) ) ;
#198133=CARTESIAN_POINT ( 'NONE',  ( -5.438229012412890917, 8.398332043573416783, -1.082531754730549967 ) ) ;
#198134=CARTESIAN_POINT ( 'NONE',  ( 3.933273961740296087, 6.642551151122080277, 1.082531754730549078 ) ) ;
#198156=CARTESIAN_POINT ( 'NONE',  ( 4.692003678781083487, 7.631698837623355658, -1.199719254218450271 ) ) ;
#198158=CARTESIAN_POINT ( 'NONE',  ( 5.110497557708379546, 4.926945003606695295, -0.7998128361456481317 ) ) ;
#198165=CARTESIAN_POINT ( 'NONE',  ( -4.318600669050610463, 4.999583595936805125, 2.499999999999999556 ) ) ;
#198168=LINE ( 'NONE', #214383, #194610 ) ;
#198181=CIRCLE ( 'NONE', #7854, 0.07999999999999982125 ) ;
#198186=CARTESIAN_POINT ( 'NONE',  ( 6.204791576909545192, 7.267953590263130259, -1.199719254218452047 ) ) ;
#198190=CARTESIAN_POINT ( 'NONE',  ( -6.500216601102190239, 6.758717457939978246, 0.07576745652920421903 ) ) ;
#198191=CARTESIAN_POINT ( 'NONE',  ( 6.550524494058025837, 7.671308660269694712, -1.199719254218452047 ) ) ;
#198202=CARTESIAN_POINT ( 'NONE',  ( 4.812442952513422689, 8.115120723895499211, -0.8517184758452013282 ) ) ;
#198217=ORIENTED_EDGE ( 'NONE', *, *, #155093, .T. ) ;
#198223=CARTESIAN_POINT ( 'NONE',  ( -6.526270840131767059, 8.707344961610770540, -1.599625672291271394 ) ) ;
#198225=CARTESIAN_POINT ( 'NONE',  ( 7.062871678076271920, 7.204714810702593120, -0.7998128361456341429 ) ) ;
#198229=CARTESIAN_POINT ( 'NONE',  ( -3.011319516011047082, 6.527306845405913549, 0.7216878364870328300 ) ) ;
#198238=CARTESIAN_POINT ( 'NONE',  ( -6.594145116354495961, 6.771750247812114765, -0.2697605348319087604 ) ) ;
#198254=CARTESIAN_POINT ( 'NONE',  ( 5.370438244788902971, 9.279612028980123384, -0.7216878364870458196 ) ) ;
#198266=CARTESIAN_POINT ( 'NONE',  ( -3.675669043080673770, 7.302381293653823491, 0.000000000000000000 ) ) ;
#198268=CARTESIAN_POINT ( 'NONE',  ( 5.013482942003290255, 9.071090208970993274, -0.7998128361456481317 ) ) ;
#198274=CARTESIAN_POINT ( 'NONE',  ( -4.679499295372141709, 5.488445928469455559, 1.199719254218452935 ) ) ;
#198276=CARTESIAN_POINT ( 'NONE',  ( 3.982994815507484354, 7.308283119008860851, -0.9368446653362592080 ) ) ;
#198284=ORIENTED_EDGE ( 'NONE', *, *, #48644, .F. ) ;
#198285=CARTESIAN_POINT ( 'NONE',  ( -4.285785955251283141, 8.014184357852876417, 0.000000000000000000 ) ) ;
#198319=CARTESIAN_POINT ( 'NONE',  ( 4.095444919779759552, 6.935713618788495793, 1.199719254218451159 ) ) ;
#198325=CARTESIAN_POINT ( 'NONE',  ( -4.787437638956927977, 7.639075441208117212, -1.082531754730549967 ) ) ;
#198331=CARTESIAN_POINT ( 'NONE',  ( -6.934069218746458318, 7.054445274817795486, -0.7998128361456362523 ) ) ;
#198340=CARTESIAN_POINT ( 'NONE',  ( -5.119085517611572378, 8.129960982925583224, 1.199719254218452935 ) ) ;
#198343=CARTESIAN_POINT ( 'NONE',  ( 4.930145672075521013, 8.107674077938057167, 1.051636801887654293 ) ) ;
#198348=CARTESIAN_POINT ( 'NONE',  ( 6.912678218121202534, 9.158153569265168770, 1.599625672291268286 ) ) ;
#198355=CARTESIAN_POINT ( 'NONE',  ( -5.438755897737433287, 6.374245297895642537, -1.199719254218453823 ) ) ;
#198359=CARTESIAN_POINT ( 'NONE',  ( -5.315678745009726924, 8.359319748223434487, -1.199719254218453823 ) ) ;
#198363=CARTESIAN_POINT ( 'NONE',  ( 6.116136693096175136, 9.189224337703940648, -1.082531754730548412 ) ) ;
#198365=CARTESIAN_POINT ( 'NONE',  ( -6.251718229232846369, 9.347402796530044355, -1.082531754730549967 ) ) ;
#198371=CARTESIAN_POINT ( 'NONE',  ( 6.703580607314123085, 6.785541894813420072, 0.000000000000000000 ) ) ;
#198385=CARTESIAN_POINT ( 'NONE',  ( 6.374094191309353619, 6.920300110170956032, -0.8184029421815092187 ) ) ;
#198392=CARTESIAN_POINT ( 'NONE',  ( -5.608135385276092677, 5.599224824533729716, 0.4022279080854191391 ) ) ;
#198400=ORIENTED_EDGE ( 'NONE', *, *, #107183, .F. ) ;
#198402=CARTESIAN_POINT ( 'NONE',  ( 4.637820276784100137, 8.319831082953612622, -0.4078742439591088731 ) ) ;
#198407=DIRECTION ( 'NONE',  ( -1.000000000000000000, 0.000000000000000000, 0.000000000000000000 ) ) ;
#198415=CARTESIAN_POINT ( 'NONE',  ( -5.638797120722775169, 7.366710520292286901, -1.234282198493292793 ) ) ;
#198433=CARTESIAN_POINT ( 'NONE',  ( -5.655686355556086120, 6.627330832017406692, 1.199719254218452935 ) ) ;
#198435=CARTESIAN_POINT ( 'NONE',  ( 7.014364370223726830, 9.276787413384745662, -1.599625672291269396 ) ) ;
#198442=VERTEX_POINT ( 'NONE', #129688 ) ;
#198447=CARTESIAN_POINT ( 'NONE',  ( 4.532168488718122390, 8.509556680138327778, 0.7998128361456271485 ) ) ;
#198450=CARTESIAN_POINT ( 'NONE',  ( 7.322812364712459221, 7.715904978352238430, 0.000000000000000000 ) ) ;
#198465=CARTESIAN_POINT ( 'NONE',  ( -5.367048706163331850, 7.354919138647580290, -1.599625672291271394 ) ) ;
#198466=CARTESIAN_POINT ( 'NONE',  ( 3.691562964670865199, 7.528850235416478576, -0.7998128361456362523 ) ) ;
#198475=CARTESIAN_POINT ( 'NONE',  ( -2.844178363816758814, 6.540234867753325076, -0.7998128361456481317 ) ) ;
#198476=CARTESIAN_POINT ( 'NONE',  ( 5.936491157937257235, 8.019268665717216749, 1.599625672291268286 ) ) ;
#198478=CARTESIAN_POINT ( 'NONE',  ( -5.765600714192150811, 7.067438534624118418, -2.440103264412639472 ) ) ;
#198483=CARTESIAN_POINT ( 'NONE',  ( 4.878955176071345434, 6.785476686873604280, -1.599625672291269396 ) ) ;
#198489=CARTESIAN_POINT ( 'NONE',  ( -6.604009391672221341, 6.765323812321595298, -0.2039879123204788036 ) ) ;
#198497=CARTESIAN_POINT ( 'NONE',  ( -3.458738584817664385, 7.049295759013638474, 0.7216878364870338292 ) ) ;
#198502=FACE_OUTER_BOUND ( 'NONE', #41179, .T. ) ;
#198546=CARTESIAN_POINT ( 'NONE',  ( 0.3372878420078945783, 3.351185588117788328, 1.972345798854260090 ) ) ;
#198547=CARTESIAN_POINT ( 'NONE',  ( 5.228604516725597229, 6.129068686715179126, -1.199719254218450271 ) ) ;
#198548=CARTESIAN_POINT ( 'NONE',  ( -3.174017359375036929, 6.717120995997236221, 0.7216878364870338292 ) ) ;
#198557=EDGE_CURVE ( 'NONE', #97415, #131991, #20503, .T. ) ;
#198564=DIRECTION ( 'NONE',  ( -0.000000000000000000, -0.000000000000000000, -1.000000000000000000 ) ) ;
#198574=CARTESIAN_POINT ( 'NONE',  ( -5.336015975430226099, 8.383046517047350932, -1.199719254218453823 ) ) ;
#198576=CARTESIAN_POINT ( 'NONE',  ( 5.655159470231527763, 9.611786791996525636, -0.7216878364870458196 ) ) ;
#198581=CARTESIAN_POINT ( 'NONE',  ( -5.550083779947821760, 7.568460058062819407, -1.599625672291271394 ) ) ;
#198589=CARTESIAN_POINT ( 'NONE',  ( -6.261886844665283114, 8.398896966899865646, 1.599625672291269396 ) ) ;
#198596=CARTESIAN_POINT ( 'NONE',  ( 3.607351389687783794, 6.366271167014519783, 1.199719254218451159 ) ) ;
#198601=CARTESIAN_POINT ( 'NONE',  ( -6.635789839245807897, 6.706452665400368218, 0.7998128361456341429 ) ) ;
#198603=ADVANCED_FACE ( 'NONE', ( #99238 ), #82962, .T. ) ;
#198607=CARTESIAN_POINT ( 'NONE',  ( -7.485510208520816278, 8.866088343763324886, 1.082531754730549078 ) ) ;
#198609=CARTESIAN_POINT ( 'NONE',  ( -6.956742217143487395, 8.249192353823097790, 1.082531754730549078 ) ) ;
#198610=CARTESIAN_POINT ( 'NONE',  ( 8.011942431032855083, 8.311964022485323511, 0.7998128361456291469 ) ) ;
#198611=CARTESIAN_POINT ( 'NONE',  ( -4.217995187182965289, 6.014356699837137832, 1.443375672974065660 ) ) ;
#198620=VERTEX_POINT ( 'NONE', #177290 ) ;
#198625=CARTESIAN_POINT ( 'NONE',  ( -0.2929755972075621662, 2.708422268617026951, 2.051080643833458783 ) ) ;
#198630=CARTESIAN_POINT ( 'NONE',  ( 6.177100234330334061, 7.056796855232915888, 1.058592334412721936 ) ) ;
#198636=CARTESIAN_POINT ( 'NONE',  ( 5.868043296107601670, 7.273814737382555684, -1.316550679767941157 ) ) ;
#198649=CARTESIAN_POINT ( 'NONE',  ( 6.039396378094620488, 7.052381734106362821, -1.030794243266313082 ) ) ;
#198662=CIRCLE ( 'NONE', #25811, 1.250000000000000444 ) ;
#198663=CARTESIAN_POINT ( 'NONE',  ( 7.876360894896227371, 8.153785563659219804, -0.7998128361456341429 ) ) ;
#198667=CARTESIAN_POINT ( 'NONE',  ( -5.655686355556086120, 6.627330832017406692, 1.199719254218452935 ) ) ;
#198682=CARTESIAN_POINT ( 'NONE',  ( 5.248941747146098180, 6.152795455539095570, -1.199719254218452047 ) ) ;
#198684=CARTESIAN_POINT ( 'NONE',  ( 5.833751235630055376, 10.02806988486892514, 0.7998128361456331437 ) ) ;
#198690=CARTESIAN_POINT ( 'NONE',  ( -7.715998819508785189, 8.174622508947939181, -0.7216878364870338292 ) ) ;
#198696=CARTESIAN_POINT ( 'NONE',  ( 7.862802741282558294, 8.137967717776607657, 0.000000000000000000 ) ) ;
#198702=DIRECTION ( 'NONE',  ( 0.6507913734559640506, -0.7592566023653003482, 0.000000000000000000 ) ) ;
#198709=CARTESIAN_POINT ( 'NONE',  ( -6.617788377246204945, 6.893376992974917350, -0.7216878364870338292 ) ) ;
#198710=CARTESIAN_POINT ( 'NONE',  ( 4.082413651490639062, 7.776916670132135501, 0.000000000000000000 ) ) ;
#198714=VERTEX_POINT ( 'NONE', #61398 ) ;
#198719=CARTESIAN_POINT ( 'NONE',  ( -4.553559489343377287, 6.405848385690952718, -1.599625672291271394 ) ) ;
#198720=CARTESIAN_POINT ( 'NONE',  ( -6.373741612200205076, 8.529394195690610303, 1.443375672974064550 ) ) ;
#198721=CARTESIAN_POINT ( 'NONE',  ( 1.849802594915211928, 2.491750049492945429, -2.487615396287162994 ) ) ;
#198724=CARTESIAN_POINT ( 'NONE',  ( 4.367134876933267407, 8.109091433148536865, 0.000000000000000000 ) ) ;
#198738=CARTESIAN_POINT ( 'NONE',  ( -5.558434366435592189, 6.905725166219703226, 1.208466946602093639 ) ) ;
#198739=CARTESIAN_POINT ( 'NONE',  ( 4.936577329151614180, 4.931964103531220722, -0.7216878364870458196 ) ) ;
#198740=CARTESIAN_POINT ( 'NONE',  ( 4.858757509019057785, 5.629766575900002401, -2.499999999999996891 ) ) ;
#198742=CARTESIAN_POINT ( 'NONE',  ( -4.167152111353897403, 5.955039778036558040, 1.599625672291270506 ) ) ;
#198754=CARTESIAN_POINT ( 'NONE',  ( 5.239300017038202917, 5.077214539491492928, 0.000000000000000000 ) ) ;
#198763=CARTESIAN_POINT ( 'NONE',  ( 7.065207446497155708, 9.336104335703744539, 0.000000000000000000 ) ) ;
#198791=CARTESIAN_POINT ( 'NONE',  ( 4.855228407469603269, 7.718164671139588151, -1.082531754730548412 ) ) ;
#198799=CARTESIAN_POINT ( 'NONE',  ( 6.834718834620487016, 7.146462526578263308, 0.000000000000000000 ) ) ;
#198814=CARTESIAN_POINT ( 'NONE',  ( -6.740338644649361832, 7.892758502626242567, -1.199719254218452047 ) ) ;
#198823=ADVANCED_FACE ( 'NONE', ( #130736 ), #17418, .T. ) ;
#198825=CARTESIAN_POINT ( 'NONE',  ( 3.973948422136968084, 5.729635473950147606, -1.443375672974068769 ) ) ;
#198831=CARTESIAN_POINT ( 'NONE',  ( -5.803772275101700906, 8.928762199997411386, -1.199719254218452047 ) ) ;
#198837=CARTESIAN_POINT ( 'NONE',  ( -5.478903473698247595, 8.445785581739666981, -1.082531754730549967 ) ) ;
#198840=CARTESIAN_POINT ( 'NONE',  ( -6.123442655227560927, 7.173046514967467147, 1.199719254218452047 ) ) ;
#198861=CARTESIAN_POINT ( 'NONE',  ( -5.582925393777276035, 9.735439736040634173, 0.7998128361456291469 ) ) ;
#198862=CARTESIAN_POINT ( 'NONE',  ( 3.386504508363381571, 7.172948703057747011, -0.7998128361456362523 ) ) ;
#198863=CARTESIAN_POINT ( 'NONE',  ( -6.143779885648060102, 7.196773283791382703, 1.199719254218452047 ) ) ;
#198887=CARTESIAN_POINT ( 'NONE',  ( -8.106849506328558164, 8.422688943663599659, 0.000000000000000000 ) ) ;
#198915=CARTESIAN_POINT ( 'NONE',  ( 4.492547798081839794, 6.334668079219206049, 1.599625672291262513 ) ) ;
#198917=CARTESIAN_POINT ( 'NONE',  ( 3.667411383892732246, 3.520940564220482738, -2.447588313016641148 ) ) ;
#198927=CARTESIAN_POINT ( 'NONE',  ( 4.851297196472967421, 8.072458764906237150, -0.9094135686919021522 ) ) ;
#198929=CARTESIAN_POINT ( 'NONE',  ( 5.401997860402196316, 5.267028690082820930, 0.000000000000000000 ) ) ;
#198936=CARTESIAN_POINT ( 'NONE',  ( -5.074494633264801990, 9.142270515442742607, 0.7998128361456291469 ) ) ;
#198938=ORIENTED_EDGE ( 'NONE', *, *, #16357, .F. ) ;
#198942=CARTESIAN_POINT ( 'NONE',  ( -7.119440060507479018, 8.439006504414422238, 1.082531754730549078 ) ) ;
#198950=CARTESIAN_POINT ( 'NONE',  ( 5.072158865288233898, 7.971250205261355859, 1.082531754730549078 ) ) ;
#198953=CARTESIAN_POINT ( 'NONE',  ( -5.659602779061863487, 5.567567761852417085, 0.7998128361456281477 ) ) ;
#198963=CARTESIAN_POINT ( 'NONE',  ( 4.740510986633625024, 5.559626234941203116, -1.199719254218450271 ) ) ;
#198964=CARTESIAN_POINT ( 'NONE',  ( 3.413620815590684199, 7.204584394822967752, 0.7998128361456281477 ) ) ;
#198982=CARTESIAN_POINT ( 'NONE',  ( 3.853720295264306372, 8.531188044730880549, -2.447541241191877770 ) ) ;
#198995=CARTESIAN_POINT ( 'NONE',  ( 6.638652492546827766, 7.774124658506663010, 1.199719254218452047 ) ) ;
#199003=CARTESIAN_POINT ( 'NONE',  ( 5.736508392357904107, 5.865217010605237924, 0.000000000000000000 ) ) ;
#199006=CARTESIAN_POINT ( 'NONE',  ( 5.234856708652215751, 9.121433570154021453, 0.7216878364870317197 ) ) ;
#199007=ORIENTED_EDGE ( 'NONE', *, *, #67389, .F. ) ;
#199017=CARTESIAN_POINT ( 'NONE',  ( -6.509323148336870091, 7.727203440215372865, 1.082531754730549078 ) ) ;
#199024=CARTESIAN_POINT ( 'NONE',  ( 4.260029445439558415, 7.236136616047151193, -2.420000000000000373 ) ) ;
#199041=CARTESIAN_POINT ( 'NONE',  ( 5.858531774436539052, 6.007577623030311287, 0.000000000000000000 ) ) ;
#199053=CARTESIAN_POINT ( 'NONE',  ( 5.481239241674765950, 9.616805891921051952, -0.7998128361456481317 ) ) ;
#199055=CARTESIAN_POINT ( 'NONE',  ( 4.701645408888975197, 8.707279753670952971, 0.000000000000000000 ) ) ;
#199068=CARTESIAN_POINT ( 'NONE',  ( -3.772911886352873445, 7.623757310712140800, 0.7998128361456352531 ) ) ;
#199070=CARTESIAN_POINT ( 'NONE',  ( 4.516274566683592617, 8.283087737857252719, -0.7216878364870357165 ) ) ;
#199073=EDGE_CURVE ( 'NONE', #96770, #203624, #30908, .T. ) ;
#199079=CARTESIAN_POINT ( 'NONE',  ( -5.171509248969888617, 4.998125310078441075, 0.7998128361456281477 ) ) ;
#199084=CARTESIAN_POINT ( 'NONE',  ( -6.292392690518209264, 8.434487120394948079, -1.443375672974066548 ) ) ;
#199086=CARTESIAN_POINT ( 'NONE',  ( -6.319508997745553636, 6.545384383557486530, 0.7216878364870257245 ) ) ;
#199096=CARTESIAN_POINT ( 'NONE',  ( 0.000000000000000000, 6.002124920821316323, 0.000000000000000000 ) ) ;
#199112=CARTESIAN_POINT ( 'NONE',  ( -3.654804927335652209, 6.421633627603656080, 1.199719254218452935 ) ) ;
#199116=FACE_OUTER_BOUND ( 'NONE', #34620, .T. ) ;
#199124=CARTESIAN_POINT ( 'NONE',  ( 2.265485140597475855, 2.737013068702903063, -2.500000000000000444 ) ) ;
#199125=CARTESIAN_POINT ( 'NONE',  ( -4.600441534204600558, 8.479163753367195966, -0.2584006677722027745 ) ) ;
#199128=VERTEX_POINT ( 'NONE', #152344 ) ;
#199143=CARTESIAN_POINT ( 'NONE',  ( 6.713222337422018349, 7.861122810861019161, -1.199719254218452047 ) ) ;
#199148=CARTESIAN_POINT ( 'NONE',  ( 4.608569825152843968, 8.455154480611607681, 0.5018163687887734481 ) ) ;
#199151=CARTESIAN_POINT ( 'NONE',  ( 1.872868072690832220, 8.979822391611987698, -0.7749999999999996891 ) ) ;
#199166=CARTESIAN_POINT ( 'NONE',  ( 5.668190738965027897, 8.770583741171307679, -1.199719254218452047 ) ) ;
#199167=CARTESIAN_POINT ( 'NONE',  ( 4.712340909201580885, 7.655425606447271214, -1.199719254218452047 ) ) ;
#199169=CARTESIAN_POINT ( 'NONE',  ( 4.041212305325117882, 6.872442235258051646, -1.199719254218448494 ) ) ;
#199182=CARTESIAN_POINT ( 'NONE',  ( 4.780342502845265074, 8.269896785439653897, -0.8296954209953393278 ) ) ;
#199183=CARTESIAN_POINT ( 'NONE',  ( -6.089020385868867180, 7.236850217336030511, -1.082531754730549967 ) ) ;
#199184=CARTESIAN_POINT ( 'NONE',  ( 4.258669648468278446, 7.022179452304728287, 1.082531754730549078 ) ) ;
#199206=CARTESIAN_POINT ( 'NONE',  ( -7.041790712887801895, 6.002124920821316323, -2.446252293856579829 ) ) ;
#199211=CARTESIAN_POINT ( 'NONE',  ( 5.342795052237045539, 8.390955439988655229, -1.199719254218450271 ) ) ;
#199212=CARTESIAN_POINT ( 'NONE',  ( 4.934241560730721510, 4.721313007132757811, 0.000000000000000000 ) ) ;
#199242=CARTESIAN_POINT ( 'NONE',  ( 6.587282531393223728, 8.778525268082516320, 1.599625672291268286 ) ) ;
#199246=CARTESIAN_POINT ( 'NONE',  ( -5.804269833667989431, 7.239147048582937671, 1.181955602297209751 ) ) ;
#199247=CARTESIAN_POINT ( 'NONE',  ( 6.713222337422018349, 7.861122810861019161, -1.199719254218452047 ) ) ;
#199260=CARTESIAN_POINT ( 'NONE',  ( 1.844764736977719366, 2.494476015512113509, 2.491383360649020773 ) ) ;
#199279=CARTESIAN_POINT ( 'NONE',  ( 4.773879485787624333, 4.742149952939897162, -0.7216878364870357165 ) ) ;
#199284=CARTESIAN_POINT ( 'NONE',  ( -6.770317605177755382, 8.992066187497757213, 1.599625672291269396 ) ) ;
#199286=CARTESIAN_POINT ( 'NONE',  ( 7.876360894896227371, 8.153785563659219804, -0.7998128361456341429 ) ) ;
#199293=CYLINDRICAL_SURFACE ( 'NONE', #65138, 3.100000000000000089 ) ;
#199297=CARTESIAN_POINT ( 'NONE',  ( -0.2808621375647266660, 2.697699530669510626, -1.982805148454100275 ) ) ;
#199305=CARTESIAN_POINT ( 'NONE',  ( 5.885121196783658526, 9.023669275293071834, 1.199719254218452047 ) ) ;
#199314=CARTESIAN_POINT ( 'NONE',  ( 6.861835142292135536, 9.098836647464588978, 1.443375672974065660 ) ) ;
#199328=CARTESIAN_POINT ( 'NONE',  ( -5.668717624289589807, 5.786127781192186958, 0.7216878364870257245 ) ) ;
#199331=CARTESIAN_POINT ( 'NONE',  ( 4.875038752565570732, 7.845239757038595663, -1.199719254218452047 ) ) ;
#199336=CARTESIAN_POINT ( 'NONE',  ( -5.652823702255029836, 5.559658838911111900, -0.7998128361456362523 ) ) ;
#199345=VERTEX_POINT ( 'NONE', #38596 ) ;
#199381=CARTESIAN_POINT ( 'NONE',  ( 3.054329744828568227, 6.785411478933790264, 0.000000000000000000 ) ) ;
#199383=CARTESIAN_POINT ( 'NONE',  ( -4.171720451616118375, 7.856123832628136405, 0.2051403462137192935 ) ) ;
#199384=CARTESIAN_POINT ( 'NONE',  ( -6.120580001926503755, 6.105374521861167914, -0.7998128361456362523 ) ) ;
#199386=CARTESIAN_POINT ( 'NONE',  ( -1.806654366501805775, 2.518449987798942136, 2.500000000000000444 ) ) ;
#199388=CARTESIAN_POINT ( 'NONE',  ( -6.766928066552171828, 7.067373297165212342, 0.7216878364870317197 ) ) ;
#199394=CARTESIAN_POINT ( 'NONE',  ( -5.237192476628793614, 9.332084666034067055, 0.7998128361456291469 ) ) ;
#199398=ORIENTED_EDGE ( 'NONE', *, *, #31247, .F. ) ;
#199402=CARTESIAN_POINT ( 'NONE',  ( -6.740338644649361832, 7.892758502626242567, -1.199719254218452047 ) ) ;
#199405=CARTESIAN_POINT ( 'NONE',  ( 4.774898309648160755, 8.276035162536045320, 0.8191430224755236189 ) ) ;
#199411=CARTESIAN_POINT ( 'NONE',  ( 6.964048179274811012, 8.153752959689313684, 1.199719254218452047 ) ) ;
#199420=CARTESIAN_POINT ( 'NONE',  ( -5.061990249855848667, 6.999017606288844284, -1.599625672291271394 ) ) ;
#199424=CARTESIAN_POINT ( 'NONE',  ( -5.250750630242457362, 9.347902511916677426, 0.000000000000000000 ) ) ;
#199428=CARTESIAN_POINT ( 'NONE',  ( 6.170369307550816806, 9.252495721234380355, 1.082531754730549967 ) ) ;
#199431=CARTESIAN_POINT ( 'NONE',  ( -6.089020385868856522, 9.157588645938716354, -1.082531754730549967 ) ) ;
#199437=CARTESIAN_POINT ( 'NONE',  ( 6.099189001301251523, 8.209082816308541197, 1.599625672291268286 ) ) ;
#199441=CARTESIAN_POINT ( 'NONE',  ( -4.948193499308641385, 4.885107685699183300, 0.5067794099899626259 ) ) ;
#199447=DIRECTION ( 'NONE',  ( 0.7592566023653044560, 0.6507913734559596097, 0.000000000000000000 ) ) ;
#199451=CARTESIAN_POINT ( 'NONE',  ( 6.038137670975392446, 7.156622065392123311, -1.170913047369964710 ) ) ;
#199473=CARTESIAN_POINT ( 'NONE',  ( 8.018721507839716267, 8.319872945426633137, -0.7998128361456341429 ) ) ;
#199478=CARTESIAN_POINT ( 'NONE',  ( -5.122256578951685846, 7.813849795838854639, -1.152996464563345924 ) ) ;
#199497=CARTESIAN_POINT ( 'NONE',  ( -5.167592825464113915, 6.057888380243431570, 1.199719254218452935 ) ) ;
#199512=CARTESIAN_POINT ( 'NONE',  ( 7.517069824134078537, 7.734612647770044092, 0.000000000000000000 ) ) ;
#199513=CARTESIAN_POINT ( 'NONE',  ( -5.414683845018970487, 6.133484104433280848, 1.108540189933695297 ) ) ;
#199515=CARTESIAN_POINT ( 'NONE',  ( 6.116136693096175136, 9.189224337703940648, -1.082531754730548412 ) ) ;
#199519=AXIS2_PLACEMENT_3D ( 'NONE', #40904, #92861, #107010 ) ;
#199531=CARTESIAN_POINT ( 'NONE',  ( -4.288121723672178476, 8.224835454251337552, -0.7998128361456362523 ) ) ;
#199532=CARTESIAN_POINT ( 'NONE',  ( 5.285699784481295183, 7.260012063351913625, 1.599625672291268286 ) ) ;
#199535=ADVANCED_FACE ( 'NONE', ( #142526 ), #210025, .T. ) ;
#199542=CARTESIAN_POINT ( 'NONE',  ( -8.100070429521727178, 8.414780020722290033, 0.7998128361456341429 ) ) ;
#199543=CARTESIAN_POINT ( 'NONE',  ( 2.898410978271408922, 6.603506251283770112, -0.7998128361456362523 ) ) ;
#199545=CARTESIAN_POINT ( 'NONE',  ( -4.492294583947676223, 8.028511867738769681, -2.499999999999999556 ) ) ;
#199551=CARTESIAN_POINT ( 'NONE',  ( 3.715816618597135523, 6.492813934075403637, -1.199719254218453823 ) ) ;
#199552=CARTESIAN_POINT ( 'NONE',  ( 6.723917837734620484, 6.809268663637336516, 0.000000000000000000 ) ) ;
#199557=CARTESIAN_POINT ( 'NONE',  ( -5.889893629278568632, 7.264407438959931795, 1.268144897863663356 ) ) ;
#199567=CARTESIAN_POINT ( 'NONE',  ( -4.624739795592948788, 5.528522862014106920, -1.082531754730549967 ) ) ;
#199571=CARTESIAN_POINT ( 'NONE',  ( -4.046711340875996044, 3.801480273782240626, 2.499999999999999556 ) ) ;
#199579=CARTESIAN_POINT ( 'NONE',  ( -5.763039058787667201, 7.049721345481766654, 2.499999999999999556 ) ) ;
#199597=CARTESIAN_POINT ( 'NONE',  ( 4.980641328173811999, 6.904110530993182948, 1.599625672291269396 ) ) ;
#199618=CARTESIAN_POINT ( 'NONE',  ( 6.052789233858158369, 6.026285292448116948, 0.000000000000000000 ) ) ;
#199619=CARTESIAN_POINT ( 'NONE',  ( -2.875737979874388284, 6.369128386579808954, -0.7216878364870458196 ) ) ;
#199643=CARTESIAN_POINT ( 'NONE',  ( -7.117104292530948229, 7.267986194233038155, -0.7998128361456362523 ) ) ;
#199650=CARTESIAN_POINT ( 'NONE',  ( -5.008811405605897882, 4.808311159487113073, 0.7998128361456281477 ) ) ;
#199657=CARTESIAN_POINT ( 'NONE',  ( -7.370792787684826486, 8.628288336167626582, -1.199719254218452047 ) ) ;
#199664=CARTESIAN_POINT ( 'NONE',  ( 3.230585741806197841, 6.991043475407723307, 0.7998128361456271485 ) ) ;
#199671=CARTESIAN_POINT ( 'NONE',  ( -4.664887371553763096, 7.600063145858131364, -1.199719254218453823 ) ) ;
#199675=CARTESIAN_POINT ( 'NONE',  ( -5.804299160426224624, 9.785783097223662352, -0.7216878364870338292 ) ) ;
#199678=CARTESIAN_POINT ( 'NONE',  ( -6.075462232255183892, 10.10214001435745246, 0.000000000000000000 ) ) ;
#199679=CARTESIAN_POINT ( 'NONE',  ( 3.553645660113312399, 7.160020680191912845, -1.734723475976807094E-15 ) ) ;
#199680=CARTESIAN_POINT ( 'NONE',  ( -4.950135482320939140, 4.947781948895412008, -0.7216878364870338292 ) ) ;
#199688=VERTEX_POINT ( 'NONE', #152371 ) ;
#199694=CARTESIAN_POINT ( 'NONE',  ( 0.0008036159801554723387, 2.587196701860821957, 2.002358341361919702 ) ) ;
#199699=CARTESIAN_POINT ( 'NONE',  ( 6.374094191309353619, 6.920300110170956032, -0.8184029421815092187 ) ) ;
#199721=CARTESIAN_POINT ( 'NONE',  ( 5.865087380380676230, 7.178575736046542310, -1.148900262672468475 ) ) ;
#199735=AXIS2_PLACEMENT_3D ( 'NONE', #51788, #180700, #32324 ) ;
#199737=CARTESIAN_POINT ( 'NONE',  ( 5.854088466050551887, 10.05179665369283981, 0.7998128361456341429 ) ) ;
#199740=CARTESIAN_POINT ( 'NONE',  ( -6.967964602780620353, 7.093989889524320525, 0.000000000000000000 ) ) ;
#199744=CARTESIAN_POINT ( 'NONE',  ( -7.607533590599451223, 9.008448956188397361, 1.082531754730549078 ) ) ;
#199754=CARTESIAN_POINT ( 'NONE',  ( 4.923546060418115822, 5.773167154356443120, -1.199719254218452047 ) ) ;
#199756=CARTESIAN_POINT ( 'NONE',  ( 6.156284269057003655, 9.340026192945279249, -1.199719254218452047 ) ) ;
#199762=CARTESIAN_POINT ( 'NONE',  ( -5.099275172071237705, 8.963255110809500437, 0.000000000000000000 ) ) ;
#199767=CARTESIAN_POINT ( 'NONE',  ( 7.686546744304875389, 7.932335721302671949, 0.7998128361456291469 ) ) ;
#199780=CARTESIAN_POINT ( 'NONE',  ( -6.672020991700860826, 7.917017590806697314, 1.082531754730549078 ) ) ;
#199781=CARTESIAN_POINT ( 'NONE',  ( 4.584065335196252811, 8.362176967788721882, 0.7216878364870328300 ) ) ;
#199792=CARTESIAN_POINT ( 'NONE',  ( -3.135678666510573365, 6.880318554229450712, 0.000000000000000000 ) ) ;
#199793=CARTESIAN_POINT ( 'NONE',  ( -6.536439455564198475, 8.719208346281938304, 1.443375672974064550 ) ) ;
#199794=CARTESIAN_POINT ( 'NONE',  ( 5.691390622686558487, 9.861982503101517139, 0.7998128361456341429 ) ) ;
#199797=CARTESIAN_POINT ( 'NONE',  ( 4.706088717274896638, 7.544168365912456764, 1.082531754730548412 ) ) ;
#199799=ORIENTED_EDGE ( 'NONE', *, *, #61767, .T. ) ;
#199809=CARTESIAN_POINT ( 'NONE',  ( -5.244114872543307548, 7.700386654371578210, 1.209007019071134170 ) ) ;
#199814=CARTESIAN_POINT ( 'NONE',  ( 3.268924434670684498, 6.827845917175511481, -1.734723475976807094E-15 ) ) ;
#199817=CARTESIAN_POINT ( 'NONE',  ( -4.796552484184649856, 8.818004674849227342, -0.7998128361456362523 ) ) ;
#199831=CARTESIAN_POINT ( 'NONE',  ( 3.902768115887398803, 5.646591783325653147, -1.599625672291269396 ) ) ;
#199857=ORIENTED_EDGE ( 'NONE', *, *, #125435, .T. ) ;
#199868=CARTESIAN_POINT ( 'NONE',  ( 5.939880696562888751, 7.062853913145737295, -1.082531754730548412 ) ) ;
#199874=CARTESIAN_POINT ( 'NONE',  ( 6.495764994278809823, 6.751016379513001375, 0.7216878364870328300 ) ) ;
#199895=CARTESIAN_POINT ( 'NONE',  ( -4.516801452008150086, 5.298631777878131111, 1.199719254218452935 ) ) ;
#199897=CARTESIAN_POINT ( 'NONE',  ( 5.370438244344566847, 5.438135171256338829, 0.000000000000000000 ) ) ;
#199904=CARTESIAN_POINT ( 'NONE',  ( -5.413448473606448985, 9.537716662508005427, 0.000000000000000000 ) ) ;
#199910=CARTESIAN_POINT ( 'NONE',  ( -4.502716413514296079, 8.267269892493059658, -0.7216878364870338292 ) ) ;
#199913=CARTESIAN_POINT ( 'NONE',  ( -4.925354943514475003, 8.968274210734028529, 0.000000000000000000 ) ) ;
#199922=AXIS2_PLACEMENT_3D ( 'NONE', #62013, #47924, #161656 ) ;
#199933=CARTESIAN_POINT ( 'NONE',  ( -3.526529353330355221, 6.168015774643768268, -1.082531754730546636 ) ) ;
#199934=ORIENTED_EDGE ( 'NONE', *, *, #126711, .T. ) ;
#199935=CARTESIAN_POINT ( 'NONE',  ( -3.946832114909637479, 7.618738210787614484, 0.7216878364870338292 ) ) ;
#199936=CARTESIAN_POINT ( 'NONE',  ( 4.167152111353856547, 5.955039778036558040, 1.599625672291262513 ) ) ;
#199937=CARTESIAN_POINT ( 'NONE',  ( -4.305596300791617814, 7.180890229968955651, 1.199719254218452935 ) ) ;
#199938=CARTESIAN_POINT ( 'NONE',  ( -4.945692173934974178, 8.992000979557944973, 0.000000000000000000 ) ) ;
#199963=CARTESIAN_POINT ( 'NONE',  ( 3.179715765502636682, 5.975770656120749535, 2.499999999999999556 ) ) ;
#199976=B_SPLINE_CURVE_WITH_KNOTS ( 'NONE', 3,
 ( #113314, #213899, #33052, #65522, #133786, #150008, #131667, #82857, #99130, #198721, #50367, #67639, #49314, #100179, #51439, #29867 ),
 .UNSPECIFIED., .F., .F.,
 ( 4, 3, 3, 3, 3, 4 ),
 ( 0.000000000000000000, 1.583418202669895186E-05, 3.180857839710038795E-05, 4.638200804740730851E-05, 6.757612010261591353E-05, 9.484161822725196631E-05 ),
 .UNSPECIFIED. ) ;
#199977=AXIS2_PLACEMENT_3D ( 'NONE', #2171, #151674, #134381 ) ;
#199992=CARTESIAN_POINT ( 'NONE',  ( 3.549202351727371862, 7.362762853649070571, -0.7998128361456362523 ) ) ;
#200006=CARTESIAN_POINT ( 'NONE',  ( 4.637309883081485395, 8.320457421531981979, 0.4059539251603030974 ) ) ;
#200009=CARTESIAN_POINT ( 'NONE',  ( 2.878073747850912412, 6.579779482459851003, -0.7998128361456362523 ) ) ;
#200014=CARTESIAN_POINT ( 'NONE',  ( -4.827585214917754719, 7.789877296449459365, -1.199719254218453823 ) ) ;
#200019=FACE_OUTER_BOUND ( 'NONE', #113455, .T. ) ;
#200023=CARTESIAN_POINT ( 'NONE',  ( 4.950135482320912494, 6.868520377498098739, -1.443375672974068769 ) ) ;
#200026=CARTESIAN_POINT ( 'NONE',  ( 6.699137298928158124, 6.988284068270579574, 0.7216878364870328300 ) ) ;
#200029=CARTESIAN_POINT ( 'NONE',  ( -5.041653019435350380, 6.975290837464928728, -1.599625672291271394 ) ) ;
#200036=VERTEX_POINT ( 'NONE', #134021 ) ;
#200042=CARTESIAN_POINT ( 'NONE',  ( 5.890091390494168522, 5.836471141856793388, 0.000000000000000000 ) ) ;
#200043=CARTESIAN_POINT ( 'NONE',  ( 5.435893244436359240, 5.306573304789342416, -0.7998128361456481317 ) ) ;
#200049=ORIENTED_EDGE ( 'NONE', *, *, #161384, .F. ) ;
#200051=CIRCLE ( 'NONE', #41001, 3.970406073902761790 ) ;
#200068=CARTESIAN_POINT ( 'NONE',  ( 7.614839552730775729, 8.913009562054615031, 1.199719254218452047 ) ) ;
#200076=CARTESIAN_POINT ( 'NONE',  ( 4.844006021832467646, 8.873367135438366304, 0.000000000000000000 ) ) ;
#200077=LINE ( 'NONE', #185964, #80652 ) ;
#200081=CARTESIAN_POINT ( 'NONE',  ( 5.912764389335563919, 6.070849007079172743, -0.7216878364870458196 ) ) ;
#200083=CARTESIAN_POINT ( 'NONE',  ( 7.051649292883499953, 7.399548061218447437, -0.7216878364870317197 ) ) ;
#200095=CARTESIAN_POINT ( 'NONE',  ( 6.119462805442048570, 6.996221746119736018, -0.9567421715909133484 ) ) ;
#200096=CARTESIAN_POINT ( 'NONE',  ( -6.672020991700860826, 7.917017590806697314, 1.082531754730549078 ) ) ;
#200100=CARTESIAN_POINT ( 'NONE',  ( 3.177206141917392923, 8.963489737286291614, 2.500000000000000888 ) ) ;
#200131=CARTESIAN_POINT ( 'NONE',  ( 6.692885107001518286, 7.837396042037102717, -1.199719254218452047 ) ) ;
#200132=CARTESIAN_POINT ( 'NONE',  ( -6.251718229232856139, 6.466295153626024472, -0.7216878364870422669 ) ) ;
#200133=CARTESIAN_POINT ( 'NONE',  ( 7.713663051532233972, 7.963971413067895355, -0.7998128361456341429 ) ) ;
#200145=CARTESIAN_POINT ( 'NONE',  ( -5.285699784481336927, 7.260012063351913625, 1.599625672291263179 ) ) ;
#200147=CARTESIAN_POINT ( 'NONE',  ( 5.329763783503544516, 9.232158490813878515, -0.7216878364870458196 ) ) ;
#200156=CARTESIAN_POINT ( 'NONE',  ( -2.986538976760251263, 6.706322249520737522, -0.7998128361456481317 ) ) ;
#200162=CARTESIAN_POINT ( 'NONE',  ( -7.444835747679825033, 7.858265591814152629, 0.000000000000000000 ) ) ;
#200164=CARTESIAN_POINT ( 'NONE',  ( -4.814553946628611136, 8.631080347793099961, 0.000000000000000000 ) ) ;
#200187=CARTESIAN_POINT ( 'NONE',  ( -3.709037541790315640, 6.484905011134099340, -1.199719254218450271 ) ) ;
#200188=CARTESIAN_POINT ( 'NONE',  ( -5.608113461897637819, 5.663683967803710750, -0.3064300721642960190 ) ) ;
#200198=CARTESIAN_POINT ( 'NONE',  ( -4.612885993627734216, 8.463679738117141582, -0.3448095128447264957 ) ) ;
#200200=DIRECTION ( 'NONE',  ( 0.7592566023653005702, 0.6507913734559639396, 0.000000000000000000 ) ) ;
#200216=CARTESIAN_POINT ( 'NONE',  ( 5.875479466675786355, 7.948088359245467416, -1.599625672291283607 ) ) ;
#200229=ADVANCED_FACE ( 'NONE', ( #140431 ), #88389, .T. ) ;
#200239=CARTESIAN_POINT ( 'NONE',  ( 5.508355548902068577, 9.648441583686274470, 0.7998128361456331437 ) ) ;
#200240=CARTESIAN_POINT ( 'NONE',  ( 4.552505719138623341, 8.533283448962240669, 0.7998128361456341429 ) ) ;
#200242=CARTESIAN_POINT ( 'NONE',  ( 5.903649544107831382, 5.852288987739402870, -0.7998128361456481317 ) ) ;
#200243=CARTESIAN_POINT ( 'NONE',  ( -6.326802395788107880, 6.950450678040672514, 0.9045734915664763731 ) ) ;
#200254=CARTESIAN_POINT ( 'NONE',  ( 5.599868899865946936, 7.382462344760764239, -1.240035354157904779 ) ) ;
#200255=CARTESIAN_POINT ( 'NONE',  ( -7.065207446052822249, 7.415365906582643163, -0.7216878364870338292 ) ) ;
#200256=CARTESIAN_POINT ( 'NONE',  ( 5.072158865288243668, 6.050511776658669127, 1.082531754730549078 ) ) ;
#200278=CARTESIAN_POINT ( 'NONE',  ( -5.438229012412911345, 5.517224400669388018, -0.7216878364870338292 ) ) ;
#200283=CARTESIAN_POINT ( 'NONE',  ( 6.367489420273535039, 7.457767740854454708, -1.199719254218452047 ) ) ;
#200312=CARTESIAN_POINT ( 'NONE',  ( 5.318541398310776103, 9.426991741329731056, -0.7998128361456481317 ) ) ;
#200316=CARTESIAN_POINT ( 'NONE',  ( -5.333877144031607287, 7.620261487198364492, 1.234409035313356107 ) ) ;
#200317=CARTESIAN_POINT ( 'NONE',  ( 6.339319342841494453, 9.553567112360518365, -1.199719254218452047 ) ) ;
#200322=AXIS2_PLACEMENT_3D ( 'NONE', #73176, #9264, #23360 ) ;
#200342=CARTESIAN_POINT ( 'NONE',  ( 4.909461021924256485, 4.900328411765999981, 0.7216878364870338292 ) ) ;
#200347=CARTESIAN_POINT ( 'NONE',  ( -7.930593509350902792, 8.217056947189661287, -0.7998128361456362523 ) ) ;
#200349=CARTESIAN_POINT ( 'NONE',  ( 5.664274315459256748, 9.830346811336296398, -0.7998128361456481317 ) ) ;
#200359=( BOUNDED_CURVE ( )  B_SPLINE_CURVE ( 2, ( #71516, #70442, #105131, #2240, #201511, #35833, #104052, #136558, #202579, #186344, #151741, #101911, #53159, #19582, #54231, #154931, #85654, #120369, #138693, #170098, #21684, #204710, #87794, #6516, #119288, #153868, #185274, #56360, #203645, #169037, #121446, #187415, #122523, #40116, #102979, #42263, #59548, #192735, #125707, #94217, #124648, #173329, #190605, #28123, #106227, #27040, #210052, #176511, #108376, #208981, #8664, #191666, #43331, #175456, #109449, #93149, #76862, #7585, #159186, #10787, #24907 ),
 .UNSPECIFIED., .F., .T. ) 
 B_SPLINE_CURVE_WITH_KNOTS ( ( 3, 2, 2, 2, 2, 2, 2, 2, 2, 2, 2, 2, 2, 2, 2, 2, 2, 2, 2, 2, 2, 2, 2, 2, 2, 2, 2, 2, 2, 2, 3 ),
 ( 0.2689266445891022039, 0.2750000000000000222, 0.2833333333333333259, 0.2916666666666666852, 0.2999999999999999889, 0.3083333333333333481, 0.3166666666666666519, 0.3250000000000000111, 0.3333333333333333148, 0.3416666666666666741, 0.3499999999999999778, 0.3583333333333333370, 0.3666666666666666408, 0.3750000000000000000, 0.3833333333333333592, 0.3916666666666666630, 0.4000000000000000222, 0.4083333333333333259, 0.4166666666666667407, 0.4249999999999999889, 0.4333333333333333481, 0.4416666666666666519, 0.4500000000000000111, 0.4583333333333333148, 0.4666666666666666741, 0.4749999999999999778, 0.4833333333333333370, 0.4916666666666666408, 0.5000000000000000000, 0.5083333333333333037, 0.5088011391770072001 ),
 .UNSPECIFIED. ) 
 CURVE ( )  GEOMETRIC_REPRESENTATION_ITEM ( )  RATIONAL_B_SPLINE_CURVE ( ( 0.9470400169073494023, 0.9023589593381649010, 1.000000000000000000, 0.8660254037844387076, 1.000000000000000000, 0.8660254037844387076, 1.000000000000000000, 0.8660254037844387076, 1.000000000000000000, 0.8660254037844387076, 1.000000000000000000, 0.8660254037844387076, 1.000000000000000000, 0.8660254037844387076, 1.000000000000000000, 0.8660254037844387076, 1.000000000000000000, 0.8660254037844387076, 1.000000000000000000, 0.8660254037844387076, 1.000000000000000000, 0.8660254037844387076, 1.000000000000000000, 0.8660254037844387076, 1.000000000000000000, 0.8660254037844387076, 1.000000000000000000, 0.8660254037844387076, 1.000000000000000000, 0.8660254037844387076, 1.000000000000000000, 0.8660254037844387076, 1.000000000000000000, 0.8660254037844387076, 1.000000000000000000, 0.8660254037844387076, 1.000000000000000000, 0.8660254037844387076, 1.000000000000000000, 0.8660254037844387076, 1.000000000000000000, 0.8660254037844387076, 1.000000000000000000, 0.8660254037844387076, 1.000000000000000000, 0.8660254037844387076, 1.000000000000000000, 0.8660254037844387076, 1.000000000000000000, 0.8660254037844387076, 1.000000000000000000, 0.8660254037844387076, 1.000000000000000000, 0.8660254037844387076, 1.000000000000000000, 0.8660254037844387076, 1.000000000000000000, 0.8660254037844387076, 1.000000000000000000, 0.9924791081183812480, 0.9858026123580090339 ) ) 
 REPRESENTATION_ITEM ( '' )  );
#200367=CIRCLE ( 'NONE', #20554, 3.100000000000000089 ) ;
#200373=CARTESIAN_POINT ( 'NONE',  ( 7.343676480457483002, 8.596652644402405841, -1.199719254218452047 ) ) ;
#200382=CARTESIAN_POINT ( 'NONE',  ( 5.722950238744187956, 9.690876021928001904, 0.7216878364870317197 ) ) ;
#200394=CARTESIAN_POINT ( 'NONE',  ( -6.143253000767895600, 6.339752387083549934, 0.000000000000000000 ) ) ;
#200396=CARTESIAN_POINT ( 'NONE',  ( 5.712781623311797397, 7.758274208654143855, -1.599625672291283607 ) ) ;
#200401=CARTESIAN_POINT ( 'NONE',  ( -3.318713740295064163, 7.093859473644694269, 0.000000000000000000 ) ) ;
#200407=AXIS2_PLACEMENT_3D ( 'NONE', #95216, #132002, #161266 ) ;
#200415=CARTESIAN_POINT ( 'NONE',  ( 3.791513125430877373, 7.352524219418101303, -0.3677586026353037996 ) ) ;
#200442=CARTESIAN_POINT ( 'NONE',  ( 3.282482588284323821, 6.843663763058119187, 0.7216878364870257245 ) ) ;
#200447=CARTESIAN_POINT ( 'NONE',  ( 3.230585741806197841, 6.991043475407723307, 0.7998128361456271485 ) ) ;
#200450=CARTESIAN_POINT ( 'NONE',  ( -5.808742468812186033, 5.741564066561132940, 0.000000000000000000 ) ) ;
#200454=CARTESIAN_POINT ( 'NONE',  ( -5.600926855776888758, 7.627776979863398310, -1.443375672974066548 ) ) ;
#200455=CARTESIAN_POINT ( 'NONE',  ( 0.3999999999999758193, 2.999999999999999112, 7.500000000000000000 ) ) ;
#200460=CARTESIAN_POINT ( 'NONE',  ( -6.394605727500880299, 7.489403432619674561, -1.199719254218452047 ) ) ;
#200467=CARTESIAN_POINT ( 'NONE',  ( 3.583694962331215095, 7.343521886800600029, 0.3257169618917153397 ) ) ;
#200469=CARTESIAN_POINT ( 'NONE',  ( -4.633854640820660009, 8.628190524257904670, -0.7998128361456362523 ) ) ;
#200471=CARTESIAN_POINT ( 'NONE',  ( 4.802592184731321545, 8.245026257381830703, 0.8702854636597904259 ) ) ;
#200477=CARTESIAN_POINT ( 'NONE',  ( 5.722423353419669567, 8.833855124701747386, 1.199719254218451159 ) ) ;
#200484=CARTESIAN_POINT ( 'NONE',  ( -5.276058054373441664, 6.184431147304315424, -1.199719254218453823 ) ) ;
#200487=CARTESIAN_POINT ( 'NONE',  ( -5.264308783856126439, 9.363720357799287797, -0.7998128361456362523 ) ) ;
#200488=EDGE_CURVE ( 'NONE', #112565, #164262, #64857, .T. ) ;
#200490=CARTESIAN_POINT ( 'NONE',  ( 5.438229012412886476, 7.437962829272074750, -1.443375672974078316 ) ) ;
#200492=CARTESIAN_POINT ( 'NONE',  ( 6.007671464186812749, 10.02305078494439883, 0.7216878364870317197 ) ) ;
#200494=CARTESIAN_POINT ( 'NONE',  ( -6.821160681006823268, 9.051383109298335228, 1.443375672974064550 ) ) ;
#200501=CARTESIAN_POINT ( 'NONE',  ( 7.191674137406095291, 7.354984346587396082, 0.000000000000000000 ) ) ;
#200502=ORIENTED_EDGE ( 'NONE', *, *, #194169, .F. ) ;
#200510=CARTESIAN_POINT ( 'NONE',  ( -2.428612866367529932E-14, 8.999999999999998224, 2.420000000000000373 ) ) ;
#200514=CARTESIAN_POINT ( 'NONE',  ( 6.533654944624902150, 6.813559398729744032, -0.4760831665120857648 ) ) ;
#200535=CARTESIAN_POINT ( 'NONE',  ( 5.899206235721897507, 6.055031161196562373, 0.000000000000000000 ) ) ;
#200542=CARTESIAN_POINT ( 'NONE',  ( -6.604009391672221341, 6.765323812321595298, -0.2039879123204788036 ) ) ;
#200560=CARTESIAN_POINT ( 'NONE',  ( -3.806807270387036368, 7.663301925418665839, 0.000000000000000000 ) ) ;
#200574=CARTESIAN_POINT ( 'NONE',  ( 6.855582950365507244, 8.027210192628430718, -1.199719254218452047 ) ) ;
#200575=CARTESIAN_POINT ( 'NONE',  ( 3.061108821635398769, 6.793320401875094561, -0.7998128361456362523 ) ) ;
#200577=CARTESIAN_POINT ( 'NONE',  ( 6.333067150914816423, 7.521571443223021625, 1.082531754730549967 ) ) ;
#200590=CARTESIAN_POINT ( 'NONE',  ( -6.231907884136888676, 7.299589282028351001, -1.199719254218453823 ) ) ;
#200591=CARTESIAN_POINT ( 'NONE',  ( 6.052789233858158369, 6.026285292448116948, 0.000000000000000000 ) ) ;
#200597=( BOUNDED_CURVE ( )  B_SPLINE_CURVE ( 2, ( #19664, #134529, #150763, #183238, #151825, #202665, #200535 ),
 .UNSPECIFIED., .F., .T. ) 
 B_SPLINE_CURVE_WITH_KNOTS ( ( 3, 2, 2, 3 ),
 ( 0.3250000000000001776, 0.3333333333333334814, 0.3416666666666667851, 0.3500000000000000888 ),
 .UNSPECIFIED. ) 
 CURVE ( )  GEOMETRIC_REPRESENTATION_ITEM ( )  RATIONAL_B_SPLINE_CURVE ( ( 0.9999999999999973355, 0.8660254037844413721, 1.000000000000000000, 0.8660254037844387076, 1.000000000000000000, 0.8660254037844369313, 1.000000000000001776 ) ) 
 REPRESENTATION_ITEM ( '' )  );
#200601=CARTESIAN_POINT ( 'NONE',  ( -6.749980374757255319, 8.968339418673846097, 1.599625672291269396 ) ) ;
#200602=CARTESIAN_POINT ( 'NONE',  ( 8.005163354226054295, 8.304055099544019214, 0.000000000000000000 ) ) ;
#200604=CARTESIAN_POINT ( 'NONE',  ( 5.736508392357904107, 5.865217010605237924, 0.000000000000000000 ) ) ;
#200608=EDGE_LOOP ( 'NONE', ( #102382, #185901, #134456, #48539, #189672 ) ) ;
#200611=CARTESIAN_POINT ( 'NONE',  ( 5.091969210384201361, 8.098325291160362482, 1.199719254218452047 ) ) ;
#200616=CARTESIAN_POINT ( 'NONE',  ( -4.622835856459495574, 8.451390222604121760, 0.3997878540293615113 ) ) ;
#200628=CARTESIAN_POINT ( 'NONE',  ( -7.445362632559989535, 8.715286488521982733, 1.199719254218452047 ) ) ;
#200636=CARTESIAN_POINT ( 'NONE',  ( 4.584065335196271462, 5.481069324884694005, 1.082531754730549078 ) ) ;
#200639=CARTESIAN_POINT ( 'NONE',  ( -4.496171506534410334, 8.048216686630670580, 2.444650791391992151 ) ) ;
#200647=CARTESIAN_POINT ( 'NONE',  ( -6.642568916052639771, 6.714361588341672515, 0.000000000000000000 ) ) ;
#200650=CARTESIAN_POINT ( 'NONE',  ( 8.014278199453780616, 8.522615118883788199, 0.000000000000000000 ) ) ;
#200655=CARTESIAN_POINT ( 'NONE',  ( 5.574337433874081427, 6.532423756721743580, -1.199719254218452047 ) ) ;
#200675=CARTESIAN_POINT ( 'NONE',  ( -0.1115135314127749661, 3.398037119535586292, 2.078540374709471283 ) ) ;
#200677=CARTESIAN_POINT ( 'NONE',  ( 5.174371902270911150, 6.065797303184739420, 1.199719254218452047 ) ) ;
#200678=CARTESIAN_POINT ( 'NONE',  ( -4.001064729808656573, 7.682009594836471500, 1.214306433183764966E-14 ) ) ;
#200701=B_SPLINE_CURVE_WITH_KNOTS ( 'NONE', 3,
 ( #19103, #68906, #119889, #88397, #69970, #202098 ),
 .UNSPECIFIED., .F., .F.,
 ( 4, 2, 4 ),
 ( 0.000000000000000000, 0.0005322801792318878960, 0.001064560358463775792 ),
 .UNSPECIFIED. ) ;
#200703=CARTESIAN_POINT ( 'NONE',  ( -4.945692173934974178, 8.992000979557944973, 0.000000000000000000 ) ) ;
#200712=EDGE_CURVE ( 'NONE', #85779, #80427, #121105, .T. ) ;
#200717=CARTESIAN_POINT ( 'NONE',  ( -5.749539660647037032, 8.865490816466966351, 1.199719254218454489 ) ) ;
#200724=CARTESIAN_POINT ( 'NONE',  ( 4.146814880933355596, 5.931313009212638931, 1.599625672291261402 ) ) ;
#200729=CARTESIAN_POINT ( 'NONE',  ( -6.798487682609798632, 6.896266815991691779, 0.7998128361456341429 ) ) ;
#200732=CARTESIAN_POINT ( 'NONE',  ( -6.129694847154211423, 9.205042184104968328, -1.082531754730549967 ) ) ;
#200733=EDGE_CURVE ( 'NONE', #136449, #65494, #1851, .T. ) ;
#200737=CARTESIAN_POINT ( 'NONE',  ( 5.682275777458854371, 5.801945626556378244, 0.7216878364870328300 ) ) ;
#200738=CARTESIAN_POINT ( 'NONE',  ( -5.438229012412911345, 5.517224400669388018, -0.7216878364870338292 ) ) ;
#200741=EDGE_CURVE ( 'NONE', #160913, #202042, #13058, .T. ) ;
#200753=CARTESIAN_POINT ( 'NONE',  ( 0.3596124336656087994, 2.795337124577100152, 2.035015742620380319 ) ) ;
#200758=CARTESIAN_POINT ( 'NONE',  ( 6.536750166778501736, 6.811520125210166476, 0.4662371894542677864 ) ) ;
#200765=ORIENTED_EDGE ( 'NONE', *, *, #111897, .F. ) ;
#200777=CARTESIAN_POINT ( 'NONE',  ( 5.559975706299111309, 7.414571502401146930, -1.245397951563255834 ) ) ;
#200792=CARTESIAN_POINT ( 'NONE',  ( 7.309781096423290769, 8.557108029695882578, 1.199719254218452935 ) ) ;
#200795=CARTESIAN_POINT ( 'NONE',  ( -6.631873415740034083, 7.766215735565355160, 1.199719254218452047 ) ) ;
#200799=CARTESIAN_POINT ( 'NONE',  ( -6.685579144870156476, 9.853573864773576219, 1.082531754730549967 ) ) ;
#200806=CARTESIAN_POINT ( 'NONE',  ( 6.900173834712277632, 7.014900660111269559, -0.7998128361456341429 ) ) ;
#200814=CARTESIAN_POINT ( 'NONE',  ( -7.566859129758459979, 8.000626204239226880, 0.000000000000000000 ) ) ;
#200818=CARTESIAN_POINT ( 'NONE',  ( 7.876360894896227371, 8.153785563659219804, -0.7998128361456341429 ) ) ;
#200830=CARTESIAN_POINT ( 'NONE',  ( -6.617788377246196951, 7.853746207276256719, -1.082531754730549967 ) ) ;
#200831=CARTESIAN_POINT ( 'NONE',  ( 5.207740401424913124, 9.089797878388800711, -0.7216878364870458196 ) ) ;
#200837=FACE_OUTER_BOUND ( 'NONE', #26092, .T. ) ;
#200841=CARTESIAN_POINT ( 'NONE',  ( -5.822300622425855110, 5.757381912443740646, 0.7998128361456281477 ) ) ;
#200842=CARTESIAN_POINT ( 'NONE',  ( -7.024532985656169792, 9.288650798055913427, 1.443375672974064550 ) ) ;
#200845=CARTESIAN_POINT ( 'NONE',  ( 5.465345319640213972, 8.429967735338637524, -1.082531754730548412 ) ) ;
#200853=B_SPLINE_CURVE_WITH_KNOTS ( 'NONE', 3,
 ( #2847, #184808, #185875, #37511, #152333, #150212, #153400 ),
 .UNSPECIFIED., .F., .F.,
 ( 4, 3, 4 ),
 ( 0.000000000000000000, 2.778074687866575757E-05, 5.739355541035052121E-05 ),
 .UNSPECIFIED. ) ;
#200860=CARTESIAN_POINT ( 'NONE',  ( -4.864640111294652236, 8.076240785039992431, 0.9165970657895030627 ) ) ;
#200867=CARTESIAN_POINT ( 'NONE',  ( 4.773879485787624333, 4.742149952939897162, -0.7216878364870357165 ) ) ;
#200870=CARTESIAN_POINT ( 'NONE',  ( -6.168033539574333979, 6.160736982450306876, 0.7998128361456281477 ) ) ;
#200882=CARTESIAN_POINT ( 'NONE',  ( 3.040771591214902259, 6.769593633051179005, -0.7998128361456362523 ) ) ;
#200918=CARTESIAN_POINT ( 'NONE',  ( 5.343321937561575474, 8.287607122913563273, -1.082531754730548412 ) ) ;
#200923=CARTESIAN_POINT ( 'NONE',  ( 5.899206235277530297, 7.015400374979486209, -1.082531754730548412 ) ) ;
#200937=CARTESIAN_POINT ( 'NONE',  ( -6.444921918449773024, 8.612437886315108315, 1.599625672291269396 ) ) ;
#200948=CARTESIAN_POINT ( 'NONE',  ( 5.194182247366878613, 6.192872389083746043, 1.082531754730549078 ) ) ;
#200955=CARTESIAN_POINT ( 'NONE',  ( -6.936931872047518155, 8.122117267924091166, 1.199719254218452047 ) ) ;
#200961=CARTESIAN_POINT ( 'NONE',  ( -6.780486220610195680, 7.083191143566240910, -0.7216878364870338292 ) ) ;
#200964=CARTESIAN_POINT ( 'NONE',  ( -6.343235766347277149, 8.493804042195527870, -1.599625672291271394 ) ) ;
#200984=CARTESIAN_POINT ( 'NONE',  ( -5.153507786970285665, 5.185049637652990207, -0.7216878364870338292 ) ) ;
#200987=CARTESIAN_POINT ( 'NONE',  ( -4.123088111887291518, 7.824370207261548416, 0.000000000000000000 ) ) ;
#200989=CARTESIAN_POINT ( 'NONE',  ( 4.766573523656222555, 7.718696989977711809, 1.199719254218452047 ) ) ;
#200990=CARTESIAN_POINT ( 'NONE',  ( -3.969505113751027547, 7.853116076009993840, 1.214306433183764966E-14 ) ) ;
#200991=CARTESIAN_POINT ( 'NONE',  ( -5.661411662158206681, 8.762674818229999829, -1.199719254218452047 ) ) ;
#201017=CARTESIAN_POINT ( 'NONE',  ( -8.120407659942227241, 8.438506789546210030, 0.7998128361456341429 ) ) ;
#201022=AXIS2_PLACEMENT_3D ( 'NONE', #62336, #212831, #48242 ) ;
#201026=EDGE_CURVE ( 'NONE', #71404, #38200, #201170, .T. ) ;
#201044=ORIENTED_EDGE ( 'NONE', *, *, #175741, .T. ) ;
#201047=CARTESIAN_POINT ( 'NONE',  ( 5.032011289327418702, 5.899709921417326974, 1.199719254218452935 ) ) ;
#201061=CARTESIAN_POINT ( 'NONE',  ( 4.596835240751270035, 8.371391889155539445, -0.09823007671119071693 ) ) ;
#201064=CARTESIAN_POINT ( 'NONE',  ( 6.319508997745523438, 9.426492026461511742, -1.082531754730548412 ) ) ;
#201071=CARTESIAN_POINT ( 'NONE',  ( -5.773793314573309132, 7.829454515125894964, 1.599625672291263179 ) ) ;
#201076=AXIS2_PLACEMENT_3D ( 'NONE', #130787, #179481, #180530 ) ;
#201084=CARTESIAN_POINT ( 'NONE',  ( 7.038091139269835317, 7.383730215335837954, 0.000000000000000000 ) ) ;
#201087=CARTESIAN_POINT ( 'NONE',  ( -6.611536185319534908, 7.742488966741438716, 1.199719254218452047 ) ) ;
#201099=CARTESIAN_POINT ( 'NONE',  ( 5.551137550152489553, 5.441024994791534120, 0.7998128361456352531 ) ) ;
#201100=CARTESIAN_POINT ( 'NONE',  ( 5.091969210384201361, 8.098325291160362482, 1.199719254218452047 ) ) ;
#201127=CARTESIAN_POINT ( 'NONE',  ( 6.318982112420993502, 9.529840343536603697, -1.199719254218452047 ) ) ;
#201130=CARTESIAN_POINT ( 'NONE',  ( 4.329849954717849947, 6.144853928627882489, 1.599625672291262513 ) ) ;
#201135=CARTESIAN_POINT ( 'NONE',  ( 7.340813827156391191, 7.528980651296110160, 0.7998128361456281477 ) ) ;
#201140=CARTESIAN_POINT ( 'NONE',  ( 5.397554552016228691, 5.469770863539975991, 0.7216878364870328300 ) ) ;
#201142=EDGE_CURVE ( 'NONE', #206605, #180652, #22778, .T. ) ;
#201144=CARTESIAN_POINT ( 'NONE',  ( 7.702440666339465558, 8.158804663583751449, -0.7216878364870317197 ) ) ;
#201155=CARTESIAN_POINT ( 'NONE',  ( 6.491225937077876651, 6.748298437306541331, 0.07656069123261090292 ) ) ;
#201156=CARTESIAN_POINT ( 'NONE',  ( -6.129694847154211423, 9.205042184104968328, -1.082531754730549967 ) ) ;
#201170=B_SPLINE_CURVE_WITH_KNOTS ( 'NONE', 3,
 ( #42953, #73269, #109062, #122129, #39724, #141539 ),
 .UNSPECIFIED., .F., .F.,
 ( 4, 2, 4 ),
 ( 0.000000000000000000, 0.002403937268455931617, 0.004807874536911863235 ),
 .UNSPECIFIED. ) ;
#201191=CARTESIAN_POINT ( 'NONE',  ( 6.424584688029230328, 8.588711117491191871, 1.599625672291268286 ) ) ;
#201193=CARTESIAN_POINT ( 'NONE',  ( 5.501576472095266901, 9.640532660744973725, -0.7998128361456481317 ) ) ;
#201208=CARTESIAN_POINT ( 'NONE',  ( -6.283277845290492714, 6.295188672452495915, -0.7998128361456362523 ) ) ;
#201211=CARTESIAN_POINT ( 'NONE',  ( 7.322812364712459221, 7.715904978352238430, 0.000000000000000000 ) ) ;
#201220=CARTESIAN_POINT ( 'NONE',  ( -4.146814880933400005, 5.931313009212638931, 1.599625672291270506 ) ) ;
#201223=DIRECTION ( 'NONE',  ( -1.000000000000000000, 0.000000000000000000, 0.000000000000000000 ) ) ;
#201226=CARTESIAN_POINT ( 'NONE',  ( -7.105881907338178038, 7.462819444748888920, -0.7216878364870338292 ) ) ;
#201228=CARTESIAN_POINT ( 'NONE',  ( -6.807602527837528505, 7.114826835331461652, 0.7216878364870317197 ) ) ;
#201251=CARTESIAN_POINT ( 'NONE',  ( -4.956387674247580755, 7.940146832334256111, 1.199719254218452935 ) ) ;
#201261=CARTESIAN_POINT ( 'NONE',  ( -4.882431421883429046, 8.154724402237897962, -1.012048471081774093 ) ) ;
#201273=CARTESIAN_POINT ( 'NONE',  ( 3.147653791585713901, 8.920000000000001705, -2.500000000000002220 ) ) ;
#201284=CARTESIAN_POINT ( 'NONE',  ( 1.849150832860071647, 8.949220158640459388, -0.7749999999999996891 ) ) ;
#201299=CARTESIAN_POINT ( 'NONE',  ( 5.342795052237045539, 8.390955439988655229, -1.199719254218450271 ) ) ;
#201300=CARTESIAN_POINT ( 'NONE',  ( 5.224688093219824303, 7.188831756880171397, -1.599625672291283607 ) ) ;
#201302=CARTESIAN_POINT ( 'NONE',  ( 4.529305835417093640, 7.441884687032027657, -1.199719254218450271 ) ) ;
#201315=CARTESIAN_POINT ( 'NONE',  ( 5.528015674651411970, 7.440572265265038787, -1.248273786418591103 ) ) ;
#201317=CARTESIAN_POINT ( 'NONE',  ( -5.438229012412899799, 7.437962829272074750, -1.443375672974066548 ) ) ;
#201318=CARTESIAN_POINT ( 'NONE',  ( 3.933273961740286317, 7.602920365423422311, 0.7216878364870257245 ) ) ;
#201335=ORIENTED_EDGE ( 'NONE', *, *, #167354, .F. ) ;
#201338=CARTESIAN_POINT ( 'NONE',  ( -5.519577934094894722, 7.532869904567736974, 1.443375672974058777 ) ) ;
#201343=CARTESIAN_POINT ( 'NONE',  ( 5.234329823327693809, 8.264412672927770487, 1.199719254218451159 ) ) ;
#201364=ORIENTED_EDGE ( 'NONE', *, *, #19121, .T. ) ;
#201372=CARTESIAN_POINT ( 'NONE',  ( 7.991605200612358573, 8.288237253661408843, 0.7998128361456281477 ) ) ;
#201385=AXIS2_PLACEMENT_3D ( 'NONE', #59713, #141015, #125873 ) ;
#201402=EDGE_LOOP ( 'NONE', ( #13074, #134532, #85239, #209235, #101234, #89437 ) ) ;
#201403=CARTESIAN_POINT ( 'NONE',  ( 4.095971805104285934, 6.832365301713403838, 1.082531754730549078 ) ) ;
#201408=CARTESIAN_POINT ( 'NONE',  ( -7.469616286486262524, 7.679250187180907794, 0.7998128361456341429 ) ) ;
#201410=CARTESIAN_POINT ( 'NONE',  ( 5.528692779322568640, 9.672168352510192690, 0.7998128361456341429 ) ) ;
#201419=FACE_OUTER_BOUND ( 'NONE', #186359, .T. ) ;
#201432=CARTESIAN_POINT ( 'NONE',  ( 6.535912570239620578, 9.782925877658371405, 1.199719254218452047 ) ) ;
#201441=CARTESIAN_POINT ( 'NONE',  ( 7.187230829020129441, 8.518095734345896730, 1.082531754730549967 ) ) ;
#201453=CARTESIAN_POINT ( 'NONE',  ( -4.340018570150306232, 8.077455741901736985, -0.7216878364870338292 ) ) ;
#201456=CARTESIAN_POINT ( 'NONE',  ( 7.523848900940885542, 7.742521570711348389, 0.7998128361456291469 ) ) ;
#201459=CARTESIAN_POINT ( 'NONE',  ( -7.608060475923978494, 8.905100639113307182, 1.199719254218452047 ) ) ;
#201461=CARTESIAN_POINT ( 'NONE',  ( -4.085803189671902480, 5.860132702740892263, -1.599625672291271394 ) ) ;
#201474=DIRECTION ( 'NONE',  ( 0.000000000000000000, 0.000000000000000000, -1.000000000000000000 ) ) ;
#201476=CARTESIAN_POINT ( 'NONE',  ( -0.4716924744713574813, 3.050499071788768113, -1.943633845707283703 ) ) ;
#201503=CARTESIAN_POINT ( 'NONE',  ( 3.743459811148990291, 7.381470523066878009, -0.7216878364870338292 ) ) ;
#201510=CARTESIAN_POINT ( 'NONE',  ( -4.502189528189771472, 7.410248995266807803, -1.199719254218453823 ) ) ;
#201511=CARTESIAN_POINT ( 'NONE',  ( -5.330290668828105538, 6.247702530834755130, 1.199719254218452935 ) ) ;
#201514=CARTESIAN_POINT ( 'NONE',  ( -6.468648687051513413, 7.679749902049126220, 1.082531754730549078 ) ) ;
#201515=EDGE_CURVE ( 'NONE', #93276, #189704, #71799, .T. ) ;
#201517=CARTESIAN_POINT ( 'NONE',  ( -4.827553558169476844, 4.879519697517697985, -0.5995761563960356755 ) ) ;
#201520=VERTEX_POINT ( 'NONE', #201926 ) ;
#201521=CARTESIAN_POINT ( 'NONE',  ( -5.424143973919053785, 8.485862515284315677, 1.199719254218454489 ) ) ;
#201529=CARTESIAN_POINT ( 'NONE',  ( -6.818824913030298696, 6.919993584815607335, 0.7998128361456341429 ) ) ;
#201531=CARTESIAN_POINT ( 'NONE',  ( 4.632842592818133376, 8.443130954262043630, -0.3954830847591808696 ) ) ;
#201536=CARTESIAN_POINT ( 'NONE',  ( 7.205232291019763480, 7.370802192470005565, -0.7998128361456341429 ) ) ;
#201549=CARTESIAN_POINT ( 'NONE',  ( -7.923814432544069142, 8.209148024248356990, 0.000000000000000000 ) ) ;
#201562=CARTESIAN_POINT ( 'NONE',  ( 7.530627977747744062, 7.750430493652658015, -0.7998128361456341429 ) ) ;
#201572=DIRECTION ( 'NONE',  ( -0.6507913734559596097, 0.7592566023653043450, 0.000000000000000000 ) ) ;
#201576=CARTESIAN_POINT ( 'NONE',  ( 5.092389439195339484, 7.944299729584391123, -1.199137415704543130 ) ) ;
#201586=CARTESIAN_POINT ( 'NONE',  ( -0.3866901564497978727, 3.102326550341739875, 2.027579305719746205 ) ) ;
#201603=CARTESIAN_POINT ( 'NONE',  ( -6.606716786301501720, 6.763562328987043237, 0.1806677948501221598 ) ) ;
#201620=CARTESIAN_POINT ( 'NONE',  ( -5.842637852846353397, 5.781108681267656202, 0.7998128361456281477 ) ) ;
#201622=ORIENTED_EDGE ( 'NONE', *, *, #25508, .T. ) ;
#201639=CARTESIAN_POINT ( 'NONE',  ( 5.668717623845194176, 9.627604637879139560, 0.000000000000000000 ) ) ;
#201652=CARTESIAN_POINT ( 'NONE',  ( -5.576146316970437944, 9.727530813099326323, 0.000000000000000000 ) ) ;
#201655=CARTESIAN_POINT ( 'NONE',  ( 5.987861119090863049, 7.014868056141362551, 1.199719254218452047 ) ) ;
#201665=CARTESIAN_POINT ( 'NONE',  ( -7.747558435566414659, 8.003516027774422170, -0.7998128361456362523 ) ) ;
#201666=CARTESIAN_POINT ( 'NONE',  ( 6.831329296439236032, 9.063246493969506545, -1.599625672291267398 ) ) ;
#201673=CARTESIAN_POINT ( 'NONE',  ( 7.147083253059300922, 8.367293879104554577, 1.199719254218452935 ) ) ;
#201676=CARTESIAN_POINT ( 'NONE',  ( -2.428612866367529932E-14, 2.999999999999999112, 2.420000000000000373 ) ) ;
#201679=CARTESIAN_POINT ( 'NONE',  ( -4.749858536263919184, 8.300932276130108534, 0.7929127856809523589 ) ) ;
#201690=CARTESIAN_POINT ( 'NONE',  ( -3.323157048681004699, 6.891117300187535655, -0.7216878364870458196 ) ) ;
#201702=CARTESIAN_POINT ( 'NONE',  ( 4.909461021924254709, 5.860697626067345567, 1.082531754730549078 ) ) ;
#201705=CARTESIAN_POINT ( 'NONE',  ( -7.096767062110449942, 7.244259425409119046, -0.7998128361456362523 ) ) ;
#201708=ORIENTED_EDGE ( 'NONE', *, *, #115282, .T. ) ;
#201719=CARTESIAN_POINT ( 'NONE',  ( 4.248501033035879004, 6.049946853332221153, -1.599625672291273171 ) ) ;
#201744=CARTESIAN_POINT ( 'NONE',  ( 3.867818961648523235, 7.734482231890414283, 1.040834085586084257E-14 ) ) ;
#201745=CARTESIAN_POINT ( 'NONE',  ( -4.746763178560296836, 6.631252689777363152, 1.443375672974058777 ) ) ;
#201766=CARTESIAN_POINT ( 'NONE',  ( 4.787437623848783907, 6.678706240755900581, -1.249999999999999334 ) ) ;
#201769=CARTESIAN_POINT ( 'NONE',  ( -7.065734331377342414, 8.272386803808890576, -1.199719254218452047 ) ) ;
#201784=CARTESIAN_POINT ( 'NONE',  ( -7.611976899429754084, 7.845337568948314022, 0.7998128361456341429 ) ) ;
#201796=CARTESIAN_POINT ( 'NONE',  ( -5.855142236255304944, 7.924361590421551860, -1.599625672291271394 ) ) ;
#201799=CARTESIAN_POINT ( 'NONE',  ( -3.447516199624892419, 7.244129009529488350, 0.7998128361456352531 ) ) ;
#201802=CARTESIAN_POINT ( 'NONE',  ( -6.061904078641520144, 10.08632216847484031, 0.7216878364870267237 ) ) ;
#201803=CARTESIAN_POINT ( 'NONE',  ( 4.001064729364292916, 6.721640380016713934, -1.082531754730548412 ) ) ;
#201804=CARTESIAN_POINT ( 'NONE',  ( -8.106849506328558164, 8.422688943663599659, 0.000000000000000000 ) ) ;
#201821=CARTESIAN_POINT ( 'NONE',  ( 0.2653090297881668391, 2.688473650299893158, -2.056485102041657242 ) ) ;
#201822=CARTESIAN_POINT ( 'NONE',  ( 6.344829475870412239, 6.940264737885684987, 0.8615092103797560297 ) ) ;
#201842=CARTESIAN_POINT ( 'NONE',  ( 5.825676364550436581, 7.207913871576331566, 1.168708750232345883 ) ) ;
#201861=CARTESIAN_POINT ( 'NONE',  ( -7.117104292530948229, 7.267986194233038155, -0.7998128361456362523 ) ) ;
#201871=CARTESIAN_POINT ( 'NONE',  ( 4.538947565524982686, 8.517465603079630299, 0.000000000000000000 ) ) ;
#201877=CARTESIAN_POINT ( 'NONE',  ( -5.750066545527201534, 9.722511713174800008, 0.000000000000000000 ) ) ;
#201883=CARTESIAN_POINT ( 'NONE',  ( 4.706088717274906408, 5.623429937309770921, 1.082531754730549078 ) ) ;
#201884=CARTESIAN_POINT ( 'NONE',  ( 0.000000000000000000, 8.999999999999998224, 0.000000000000000000 ) ) ;
#201895=CARTESIAN_POINT ( 'NONE',  ( -6.617788377246193399, 8.814115421577600529, -1.443375672974066548 ) ) ;
#201897=CARTESIAN_POINT ( 'NONE',  ( 6.699137298928158124, 6.988284068270579574, 0.7216878364870328300 ) ) ;
#201903=CARTESIAN_POINT ( 'NONE',  ( 4.367134876933267407, 8.109091433148536865, 0.000000000000000000 ) ) ;
#201907=CARTESIAN_POINT ( 'NONE',  ( -3.800028193580205382, 7.655393002477360653, -0.7998128361456481317 ) ) ;
#201908=CARTESIAN_POINT ( 'NONE',  ( -3.902768115887413014, 5.646591783325653147, -1.599625672291283607 ) ) ;
#201910=CARTESIAN_POINT ( 'NONE',  ( 7.146556367734776316, 7.510272981878305387, 0.7216878364870267237 ) ) ;
#201922=CARTESIAN_POINT ( 'NONE',  ( -4.603364586660168456, 8.384938909114524108, 0.004600842637982396899 ) ) ;
#201926=CARTESIAN_POINT ( 'NONE',  ( -5.514013019825418915, 5.994650414344389056, -0.9619886414689113874 ) ) ;
#201928=CARTESIAN_POINT ( 'NONE',  ( -6.805266759416629618, 6.904175738932996964, 0.000000000000000000 ) ) ;
#201941=CARTESIAN_POINT ( 'NONE',  ( 4.960304097753311936, 6.880383762169266504, 1.599625672291268286 ) ) ;
#201948=CYLINDRICAL_SURFACE ( 'NONE', #78324, 1.250000000000000000 ) ;
#201977=CARTESIAN_POINT ( 'NONE',  ( 5.885648082108199119, 6.999582529615296700, 1.082531754730549967 ) ) ;
#201981=CARTESIAN_POINT ( 'NONE',  ( 4.882939164911702434, 4.877617891921787852, 0.1515561221680329362 ) ) ;
#201982=CARTESIAN_POINT ( 'NONE',  ( 6.549997608733495902, 7.774656977344789333, -1.082531754730548412 ) ) ;
#201995=CARTESIAN_POINT ( 'NONE',  ( -6.957269102468015554, 8.145844036748005834, 1.199719254218452047 ) ) ;
#202005=CARTESIAN_POINT ( 'NONE',  ( -3.383641855062333281, 6.105276709951447778, -1.199719254218452047 ) ) ;
#202007=CARTESIAN_POINT ( 'NONE',  ( 4.543390873910906791, 6.393985001019784953, 1.443375672974065660 ) ) ;
#202013=CARTESIAN_POINT ( 'NONE',  ( -4.004454267989906668, 5.765225627445230927, 1.599625672291270506 ) ) ;
#202018=CARTESIAN_POINT ( 'NONE',  ( -6.536439455564198475, 8.719208346281938304, 1.443375672974064550 ) ) ;
#202021=CARTESIAN_POINT ( 'NONE',  ( -5.966470118465691641, 9.118576350588734059, -1.199719254218452047 ) ) ;
#202041=CARTESIAN_POINT ( 'NONE',  ( -3.336715202739028552, 6.906935146588564223, 0.7216878364870338292 ) ) ;
#202042=VERTEX_POINT ( 'NONE', #49898 ) ;
#202043=CARTESIAN_POINT ( 'NONE',  ( -5.492461626867567226, 6.540864998501174199, 1.082531754730549078 ) ) ;
#202045=CARTESIAN_POINT ( 'NONE',  ( 4.050854035433010480, 7.948023151305657841, 0.000000000000000000 ) ) ;
#202046=CARTESIAN_POINT ( 'NONE',  ( -4.736594563127865420, 6.619389305106191834, -1.599625672291271394 ) ) ;
#202047=CARTESIAN_POINT ( 'NONE',  ( -7.767895665986912057, 8.027242796598338614, -0.7998128361456362523 ) ) ;
#202098=CARTESIAN_POINT ( 'NONE',  ( -4.913752204202785023, 4.881785571126718182, -0.5639616748225815268 ) ) ;
#202106=CARTESIAN_POINT ( 'NONE',  ( 5.411639590510088027, 6.342609606130419131, -1.199719254218452047 ) ) ;
#202123=CARTESIAN_POINT ( 'NONE',  ( 6.066347387471824781, 6.042103138330730872, -0.7998128361456481317 ) ) ;
#202129=CARTESIAN_POINT ( 'NONE',  ( -7.422162748838431412, 7.623887726591770608, -0.7998128361456362523 ) ) ;
#202134=ORIENTED_EDGE ( 'NONE', *, *, #33948, .T. ) ;
#202145=CARTESIAN_POINT ( 'NONE',  ( 5.885648082108190238, 7.959951743916638733, 1.443375672974065660 ) ) ;
#202149=CARTESIAN_POINT ( 'NONE',  ( -6.784929528996132220, 6.880448970109080520, 0.000000000000000000 ) ) ;
#202158=EDGE_LOOP ( 'NONE', ( #162558, #35057, #119691, #182515 ) ) ;
#202162=CARTESIAN_POINT ( 'NONE',  ( 4.903208829997618423, 5.749440385532527564, -1.199719254218450271 ) ) ;
#202163=CARTESIAN_POINT ( 'NONE',  ( 6.723917837734620484, 6.809268663637336516, 0.000000000000000000 ) ) ;
#202183=CARTESIAN_POINT ( 'NONE',  ( 5.413027408713817046, 7.651055653456078076, -1.328921179265474262 ) ) ;
#202192=CARTESIAN_POINT ( 'NONE',  ( 5.096939404094710468, 4.911127157724081371, 0.000000000000000000 ) ) ;
#202197=CARTESIAN_POINT ( 'NONE',  ( 5.692444392891300886, 7.734547439830227411, -1.599625672291281386 ) ) ;
#202204=CARTESIAN_POINT ( 'NONE',  ( 5.234856708652233515, 6.240325927249993576, 1.082531754730549078 ) ) ;
#202207=CARTESIAN_POINT ( 'NONE',  ( 4.913904330310220558, 4.697586238308844919, 0.000000000000000000 ) ) ;
#202219=CARTESIAN_POINT ( 'NONE',  ( 6.492506472431533560, 6.747478052702773788, -0.04572756507489894595 ) ) ;
#202220=CARTESIAN_POINT ( 'NONE',  ( -3.471769853551161411, 6.208092708188416076, 1.199719254218452935 ) ) ;
#202229=CARTESIAN_POINT ( 'NONE',  ( -0.004145910806160996512, 3.413539372451380949, -2.083557531367431270 ) ) ;
#202252=ORIENTED_EDGE ( 'NONE', *, *, #196460, .T. ) ;
#202256=CARTESIAN_POINT ( 'NONE',  ( 5.169401708560450004, 9.252995436621013425, 0.000000000000000000 ) ) ;
#202258=CARTESIAN_POINT ( 'NONE',  ( 7.201315867513990554, 8.430565262634994284, -1.199719254218452047 ) ) ;
#202260=CARTESIAN_POINT ( 'NONE',  ( -0.1265553566730630297, 3.463015919485879834, -2.076146368081344118 ) ) ;
#202271=CARTESIAN_POINT ( 'NONE',  ( -3.623772196602547346, 7.449761006003425834, 0.000000000000000000 ) ) ;
#202273=CARTESIAN_POINT ( 'NONE',  ( 4.841670253411575864, 8.662716039039905169, -0.7216878364870458196 ) ) ;
#202282=CARTESIAN_POINT ( 'NONE',  ( -4.821859908315634158, 5.654533310236863564, 1.199719254218452935 ) ) ;
#202289=CARTESIAN_POINT ( 'NONE',  ( -2.986538976760251263, 6.706322249520737522, -0.7998128361456481317 ) ) ;
#202291=CARTESIAN_POINT ( 'NONE',  ( -6.305950844131887223, 6.529566537674873494, 0.000000000000000000 ) ) ;
#202317=CARTESIAN_POINT ( 'NONE',  ( -6.005335696210345020, 5.970922831858983315, 0.7998128361456281477 ) ) ;
#202320=EDGE_CURVE ( 'NONE', #758, #28052, #47736, .T. ) ;
#202326=CARTESIAN_POINT ( 'NONE',  ( 6.180809796670631684, 5.328980321105058593, -2.499999999999329425 ) ) ;
#202327=CARTESIAN_POINT ( 'NONE',  ( -6.358822508390924888, 6.928531665952419871, -0.8607971499900844981 ) ) ;
#202338=CARTESIAN_POINT ( 'NONE',  ( 2.281615103653998666, 2.664038801896126962, 2.456549816139060649 ) ) ;
#202346=EDGE_CURVE ( 'NONE', #105328, #193413, #41134, .T. ) ;
#202358=CARTESIAN_POINT ( 'NONE',  ( 3.400062661977048428, 7.188766548940353829, -1.734723475976807094E-15 ) ) ;
#202368=CARTESIAN_POINT ( 'NONE',  ( 7.700104897918568447, 7.948153567185284096, 0.000000000000000000 ) ) ;
#202370=CARTESIAN_POINT ( 'NONE',  ( 4.960304097753311936, 6.880383762169266504, 1.599625672291268286 ) ) ;
#202374=CARTESIAN_POINT ( 'NONE',  ( -3.633158051037565617, 3.497935290439206923, -2.447764745243742546 ) ) ;
#202383=CARTESIAN_POINT ( 'NONE',  ( 5.551963943121584144, 7.421064284658021037, -1.246246109899084020 ) ) ;
#202385=CARTESIAN_POINT ( 'NONE',  ( -4.624739795592931912, 8.409630504918133909, -0.7216878364870338292 ) ) ;
#202386=CARTESIAN_POINT ( 'NONE',  ( 6.265276383290871109, 7.442482214328385304, -1.082531754730548412 ) ) ;
#202393=LINE ( 'NONE', #104944, #187734 ) ;
#202402=CARTESIAN_POINT ( 'NONE',  ( -4.299344108864949554, 8.030002203735486788, -0.7216878364870338292 ) ) ;
#202403=DIRECTION ( 'NONE',  ( -0.6507913734559627184, -0.7592566023653016805, 0.000000000000000000 ) ) ;
#202407=CARTESIAN_POINT ( 'NONE',  ( 6.866278450678116485, 6.975356045404744521, 0.000000000000000000 ) ) ;
#202429=ORIENTED_EDGE ( 'NONE', *, *, #27277, .T. ) ;
#202432=DIRECTION ( 'NONE',  ( 0.000000000000000000, 1.000000000000000000, 0.000000000000000000 ) ) ;
#202436=CARTESIAN_POINT ( 'NONE',  ( 6.855582950365507244, 8.027210192628430718, -1.199719254218452047 ) ) ;
#202447=CARTESIAN_POINT ( 'NONE',  ( -3.005201095308074777, 6.378479170349286242, -0.7606738891400167679 ) ) ;
#202463=DIRECTION ( 'NONE',  ( -0.7592566023652995710, 0.6507913734559650498, 0.000000000000000000 ) ) ;
#202465=( BOUNDED_CURVE ( )  B_SPLINE_CURVE ( 2, ( #184124, #35746, #4285, #168949, #101821, #167888, #19489 ),
 .UNSPECIFIED., .F., .T. ) 
 B_SPLINE_CURVE_WITH_KNOTS ( ( 3, 2, 2, 3 ),
 ( 0.3000000000000002109, 0.3083333333333335147, 0.3166666666666667629, 0.3250000000000000666 ),
 .UNSPECIFIED. ) 
 CURVE ( )  GEOMETRIC_REPRESENTATION_ITEM ( )  RATIONAL_B_SPLINE_CURVE ( ( 0.9999999999999964473, 0.8660254037844422603, 1.000000000000000000, 0.8660254037844387076, 1.000000000000000000, 0.8660254037844378194, 1.000000000000000888 ) ) 
 REPRESENTATION_ITEM ( '' )  );
#202467=CARTESIAN_POINT ( 'NONE',  ( 3.607878275012302627, 7.223292064240769861, 0.7216878364870257245 ) ) ;
#202475=CARTESIAN_POINT ( 'NONE',  ( 7.212011367826596242, 7.378711115411311638, 0.000000000000000000 ) ) ;
#202480=CARTESIAN_POINT ( 'NONE',  ( -5.045042558060949034, 6.018876084893449274, 1.082531754730549078 ) ) ;
#202485=CARTESIAN_POINT ( 'NONE',  ( 0.000000000000000000, 9.001999999999998892, 0.000000000000000000 ) ) ;
#202489=CARTESIAN_POINT ( 'NONE',  ( -4.913752204202785023, 4.881785571126718182, -0.5639616748225815268 ) ) ;
#202500=CARTESIAN_POINT ( 'NONE',  ( 5.833751235630055376, 10.02806988486892514, 0.7998128361456331437 ) ) ;
#202510=CARTESIAN_POINT ( 'NONE',  ( 7.241463443474815520, 8.581367117876336437, -1.082531754730548412 ) ) ;
#202522=CARTESIAN_POINT ( 'NONE',  ( -6.346625304972878467, 7.537389289624049304, 1.082531754730548412 ) ) ;
#202524=CARTESIAN_POINT ( 'NONE',  ( 6.607619761813720238, 8.802252036906432764, 1.599625672291268286 ) ) ;
#202529=CARTESIAN_POINT ( 'NONE',  ( -5.276058054373441664, 6.184431147304315424, -1.199719254218453823 ) ) ;
#202545=FACE_OUTER_BOUND ( 'NONE', #95048, .T. ) ;
#202570=CARTESIAN_POINT ( 'NONE',  ( 5.397554552016228691, 5.469770863539975991, 0.7216878364870328300 ) ) ;
#202574=CARTESIAN_POINT ( 'NONE',  ( -4.932134020321308654, 8.976183133675331050, 0.7998128361456291469 ) ) ;
#202578=CARTESIAN_POINT ( 'NONE',  ( -5.367048706163331850, 7.354919138647580290, -1.599625672291271394 ) ) ;
#202579=CARTESIAN_POINT ( 'NONE',  ( -3.806807270387036368, 7.663301925418665839, 0.000000000000000000 ) ) ;
#202583=CARTESIAN_POINT ( 'NONE',  ( -5.099275172071237705, 8.963255110809500437, 0.000000000000000000 ) ) ;
#202589=CARTESIAN_POINT ( 'NONE',  ( -3.923105346307911745, 5.670318552149568703, -1.599625672291283607 ) ) ;
#202597=CARTESIAN_POINT ( 'NONE',  ( -8.106849506328558164, 8.422688943663599659, 0.000000000000000000 ) ) ;
#202599=CARTESIAN_POINT ( 'NONE',  ( 4.605689926069578277, 8.476745573306274650, -0.2140288463435610078 ) ) ;
#202604=CARTESIAN_POINT ( 'NONE',  ( 5.110497557708379546, 4.926945003606695295, -0.7998128361456481317 ) ) ;
#202618=CARTESIAN_POINT ( 'NONE',  ( -6.291865805193673111, 9.498204651771386509, -1.199719254218452047 ) ) ;
#202631=CARTESIAN_POINT ( 'NONE',  ( 7.354371980770088690, 7.544798497178720531, 0.000000000000000000 ) ) ;
#202646=CARTESIAN_POINT ( 'NONE',  ( 6.053423048675670159, 7.145495228771222784, -1.160209803801291795 ) ) ;
#202653=CARTESIAN_POINT ( 'NONE',  ( -2.974866045527320590, 6.692355909712924600, 0.04048647387576057716 ) ) ;
#202665=CARTESIAN_POINT ( 'NONE',  ( 5.885648082108208889, 6.039213315313944896, 0.7216878364870273899 ) ) ;
#202668=CARTESIAN_POINT ( 'NONE',  ( -5.593777659986292505, 7.397990072842402398, -1.241664499109219166 ) ) ;
#202674=CARTESIAN_POINT ( 'NONE',  ( -6.612576056032890115, 6.759750829040511277, 0.1256891304984939506 ) ) ;
#202694=CARTESIAN_POINT ( 'NONE',  ( -6.479871072688648148, 6.524547437750345402, 0.000000000000000000 ) ) ;
#202710=CARTESIAN_POINT ( 'NONE',  ( 5.096939404094710468, 4.911127157724081371, 0.000000000000000000 ) ) ;
#202726=CARTESIAN_POINT ( 'NONE',  ( 5.499767588998890844, 6.445425604367387429, 1.199719254218451159 ) ) ;
#202737=CARTESIAN_POINT ( 'NONE',  ( -3.871735385154307263, 6.674719161725423788, -1.199719254218450271 ) ) ;
#202738=CARTESIAN_POINT ( 'NONE',  ( 4.760848217054122422, 5.583353003765119560, -1.199719254218452047 ) ) ;
#202744=CARTESIAN_POINT ( 'NONE',  ( 7.201315867513990554, 8.430565262634994284, -1.199719254218452047 ) ) ;
#202749=CARTESIAN_POINT ( 'NONE',  ( -4.900510728191886933, 8.135641830034209931, 1.034109914766440541 ) ) ;
#202758=CARTESIAN_POINT ( 'NONE',  ( -3.648552735408985725, 7.270745601370182776, -0.7216878364870458196 ) ) ;
#202770=CARTESIAN_POINT ( 'NONE',  ( 3.390947817193682656, 6.009837315817661008, -1.082531754730549967 ) ) ;
#202774=CARTESIAN_POINT ( 'NONE',  ( -5.529746549527323474, 7.544733289238903851, -1.599625672291271394 ) ) ;
#202784=CARTESIAN_POINT ( 'NONE',  ( -6.615342224808819616, 6.750480251133848419, 0.3470571717737805373 ) ) ;
#202788=CARTESIAN_POINT ( 'NONE',  ( 5.083381250481017410, 4.895309311841474553, 0.7998128361456352531 ) ) ;
#202812=CARTESIAN_POINT ( 'NONE',  ( -0.3857294007042892936, 3.105957228677906024, 1.963430320088064063 ) ) ;
#202814=CARTESIAN_POINT ( 'NONE',  ( -3.512971199716682591, 7.112567143062499930, 0.000000000000000000 ) ) ;
#202826=DIRECTION ( 'NONE',  ( 0.000000000000000000, 0.000000000000000000, -1.000000000000000000 ) ) ;
#202838=CARTESIAN_POINT ( 'NONE',  ( -7.293360289508603600, 7.473618190706972086, 0.000000000000000000 ) ) ;
#202844=CARTESIAN_POINT ( 'NONE',  ( -4.981695098378565945, 4.776675467721892332, -0.7998128361456362523 ) ) ;
#202847=CARTESIAN_POINT ( 'NONE',  ( -4.858757509019071996, 5.629766575900002401, 7.500000000000000000 ) ) ;
#202852=CARTESIAN_POINT ( 'NONE',  ( -2.993318053567081360, 6.714231172462041819, 0.000000000000000000 ) ) ;
#202854=CARTESIAN_POINT ( 'NONE',  ( 5.253852870291571442, 7.792406146126436006, -1.285611862062207011 ) ) ;
#202858=CARTESIAN_POINT ( 'NONE',  ( 3.390420931869152721, 6.113185632892752075, -1.199719254218452047 ) ) ;
#202864=CARTESIAN_POINT ( 'NONE',  ( -5.315678745009726924, 8.359319748223434487, -1.199719254218453823 ) ) ;
#202867=CARTESIAN_POINT ( 'NONE',  ( -5.093022980588950865, 5.970890227889075419, -1.199719254218453823 ) ) ;
#202871=CARTESIAN_POINT ( 'NONE',  ( 3.540087506499646874, 7.144202834309300698, -0.7216878364870338292 ) ) ;
#202872=CARTESIAN_POINT ( 'NONE',  ( -4.448483798615272100, 8.203998508444197313, 0.000000000000000000 ) ) ;
#202877=CARTESIAN_POINT ( 'NONE',  ( -4.098307573080856692, 8.003385611894792362, 0.7998128361456350310 ) ) ;
#202886=VECTOR ( 'NONE', #93521, 1000.000000000000114 ) ;
#202887=CARTESIAN_POINT ( 'NONE',  ( 5.554000203453580475, 6.508696987897830688, -1.199719254218452047 ) ) ;
#202893=CARTESIAN_POINT ( 'NONE',  ( 5.004104291928844539, 8.031804922028364047, 1.127571413376940335 ) ) ;
#202898=CARTESIAN_POINT ( 'NONE',  ( 5.900277318768097246, 7.249539301847896411, -1.301905728482563251 ) ) ;
#202903=CARTESIAN_POINT ( 'NONE',  ( 7.225569521440261767, 7.394528961293920233, -0.7998128361456341429 ) ) ;
#202906=EDGE_CURVE ( 'NONE', #101986, #179040, #99653, .T. ) ;
#202914=CARTESIAN_POINT ( 'NONE',  ( 5.510920874727778696, 7.454463421478725316, 1.249874847645112697 ) ) ;
#202933=CARTESIAN_POINT ( 'NONE',  ( -6.306477729012051725, 7.386587434382707151, 1.199719254218452047 ) ) ;
#202946=CARTESIAN_POINT ( 'NONE',  ( 5.737035277238070385, 6.722237907313067140, -1.199719254218452047 ) ) ;
#202957=ORIENTED_EDGE ( 'NONE', *, *, #47152, .F. ) ;
#202960=CARTESIAN_POINT ( 'NONE',  ( 3.540087506499646874, 7.144202834309300698, -0.7216878364870338292 ) ) ;
#202974=CARTESIAN_POINT ( 'NONE',  ( -7.932929277771797238, 8.427708043588125975, 0.000000000000000000 ) ) ;
#202975=CARTESIAN_POINT ( 'NONE',  ( 7.214347136247488912, 7.589362211809770997, -0.7216878364870317197 ) ) ;
#202986=CARTESIAN_POINT ( 'NONE',  ( -6.147696309153835692, 6.137010213626392208, 0.7998128361456281477 ) ) ;
#202987=CARTESIAN_POINT ( 'NONE',  ( -3.284818356260900796, 7.054314858938165678, 0.7998128361456352531 ) ) ;
#202989=CARTESIAN_POINT ( 'NONE',  ( 5.139949632912227173, 8.050339434155988627, -1.082531754730548412 ) ) ;
#202992=ORIENTED_EDGE ( 'NONE', *, *, #186024, .F. ) ;
#202996=CARTESIAN_POINT ( 'NONE',  ( 4.367134876933267407, 8.109091433148536865, 0.000000000000000000 ) ) ;
#203001=CARTESIAN_POINT ( 'NONE',  ( -4.638545736399841246, 8.340143690112583386, 0.3695662286686048903 ) ) ;
#203009=CARTESIAN_POINT ( 'NONE',  ( -4.457598643843001973, 8.422558527783969851, 0.000000000000000000 ) ) ;
#203020=CARTESIAN_POINT ( 'NONE',  ( 4.878955176071345434, 6.785476686873604280, -1.599625672291269396 ) ) ;
#203026=VECTOR ( 'NONE', #48657, 1000.000000000000000 ) ;
#203055=CARTESIAN_POINT ( 'NONE',  ( 4.258669648468268676, 7.982548666606070320, 0.7216878364870257245 ) ) ;
#203061=CARTESIAN_POINT ( 'NONE',  ( 5.519577934094852978, 7.532869904567736974, 1.443375672974064550 ) ) ;
#203076=CARTESIAN_POINT ( 'NONE',  ( -7.930593509350902792, 8.217056947189661287, -0.7998128361456362523 ) ) ;
#203087=CARTESIAN_POINT ( 'NONE',  ( 5.356880090730872013, 6.382686539675070492, 1.082531754730549078 ) ) ;
#203093=CARTESIAN_POINT ( 'NONE',  ( -5.015590482412729756, 4.816220082428420923, 0.000000000000000000 ) ) ;
#203098=CARTESIAN_POINT ( 'NONE',  ( -6.238160076063538284, 9.331584951165851294, 1.082531754730549967 ) ) ;
#203101=CARTESIAN_POINT ( 'NONE',  ( -7.584860592202423035, 7.813701877183096833, -0.7998128361456362523 ) ) ;
#203106=CARTESIAN_POINT ( 'NONE',  ( -4.442231607132987925, 5.211633625523774960, -1.199719254218453823 ) ) ;
#203119=CARTESIAN_POINT ( 'NONE',  ( -5.008811405605897882, 4.808311159487113073, 0.7998128361456281477 ) ) ;
#203124=CARTESIAN_POINT ( 'NONE',  ( -4.177320726786315497, 7.887641591310407208, -0.7216878364870458196 ) ) ;
#203127=CARTESIAN_POINT ( 'NONE',  ( -6.089020385868876062, 6.276481003034692030, -0.7216878364870338292 ) ) ;
#203129=CARTESIAN_POINT ( 'NONE',  ( 4.224247379109608680, 7.085983154673295203, -1.199719254218452047 ) ) ;
#203130=EDGE_CURVE ( 'NONE', #40830, #96770, #71470, .T. ) ;
#203131=CARTESIAN_POINT ( 'NONE',  ( -4.457598643843001973, 8.422558527783969851, 0.000000000000000000 ) ) ;
#203132=CARTESIAN_POINT ( 'NONE',  ( -5.420227550413282636, 9.545625585449309725, 0.7998128361456291469 ) ) ;
#203133=CARTESIAN_POINT ( 'NONE',  ( -6.615342224808818727, 6.750480251133849308, 0.3470571717737805373 ) ) ;
#203135=DIRECTION ( 'NONE',  ( -0.7927788072572178324, 0.000000000000000000, 0.6095094443598253475 ) ) ;
#203178=CARTESIAN_POINT ( 'NONE',  ( 7.015401035077362124, 6.062865449010540253, -2.437084766375293476 ) ) ;
#203187=CARTESIAN_POINT ( 'NONE',  ( 5.845500506147374153, 6.848780674373954547, 1.199719254218453823 ) ) ;
#203203=CARTESIAN_POINT ( 'NONE',  ( 3.718679271898170491, 7.560485927181699317, 0.7998128361456271485 ) ) ;
#203209=CARTESIAN_POINT ( 'NONE',  ( -7.584860592202423035, 7.813701877183096833, -0.7998128361456362523 ) ) ;
#203215=CARTESIAN_POINT ( 'NONE',  ( 6.398522151006641678, 6.429640362454684954, 0.000000000000000000 ) ) ;
#203226=CARTESIAN_POINT ( 'NONE',  ( 7.702440666339465558, 8.158804663583751449, -0.7216878364870317197 ) ) ;
#203228=CARTESIAN_POINT ( 'NONE',  ( -3.038435823238377687, 6.558942537171132514, -0.7216878364870458196 ) ) ;
#203229=CARTESIAN_POINT ( 'NONE',  ( -4.936050443827081580, 7.916420063510339666, 1.199719254218452935 ) ) ;
#203240=CARTESIAN_POINT ( 'NONE',  ( 5.252858170651868441, 5.093032385374103299, -0.7998128361456481317 ) ) ;
#203241=CARTESIAN_POINT ( 'NONE',  ( 6.222266154028957885, 6.224008365980749247, 0.7998128361456352531 ) ) ;
#203242=ORIENTED_EDGE ( 'NONE', *, *, #183755, .F. ) ;
#203260=CARTESIAN_POINT ( 'NONE',  ( 5.561552386509557522, 7.525632394756676113, -1.337405013919689800 ) ) ;
#203268=CARTESIAN_POINT ( 'NONE',  ( 4.817943484809818600, 6.714296380401858499, 1.599625672291269396 ) ) ;
#203272=CARTESIAN_POINT ( 'NONE',  ( 8.167861197590044142, 8.493869250135347215, 0.000000000000000000 ) ) ;
#203277=CARTESIAN_POINT ( 'NONE',  ( 5.072158865288222351, 8.931619419562697004, 0.7216878364870317197 ) ) ;
#203280=CARTESIAN_POINT ( 'NONE',  ( 3.067887898442204442, 6.801229324816399746, 0.7998128361456271485 ) ) ;
#203291=CARTESIAN_POINT ( 'NONE',  ( 6.423677080210483226, 6.791898735554919853, -0.4454198846488600649 ) ) ;
#203292=CARTESIAN_POINT ( 'NONE',  ( -3.311934663488232733, 7.085950550703385531, -0.7998128361456481317 ) ) ;
#203324=CARTESIAN_POINT ( 'NONE',  ( 6.855582950365507244, 8.027210192628430718, -1.199719254218452047 ) ) ;
#203325=CARTESIAN_POINT ( 'NONE',  ( 7.049313524462606395, 7.188896964819984525, 0.000000000000000000 ) ) ;
#203331=( NAMED_UNIT ( * ) SI_UNIT ( $, .STERADIAN. ) SOLID_ANGLE_UNIT ( ) );
#203338=CARTESIAN_POINT ( 'NONE',  ( -4.339491684825780737, 7.220434844675483355, -1.199719254218455378 ) ) ;
#203340=CARTESIAN_POINT ( 'NONE',  ( 6.224601922005513543, 7.395028676162137771, -1.082531754730548412 ) ) ;
#203351=CARTESIAN_POINT ( 'NONE',  ( -3.474632506852224356, 7.275764701294714420, -0.7998128361456481317 ) ) ;
#203356=ORIENTED_EDGE ( 'NONE', *, *, #112616, .T. ) ;
#203359=CARTESIAN_POINT ( 'NONE',  ( -5.646044625448194410, 5.551749915969804938, 0.000000000000000000 ) ) ;
#203382=CARTESIAN_POINT ( 'NONE',  ( -6.805266759416629618, 6.904175738932996964, 0.000000000000000000 ) ) ;
#203392=CARTESIAN_POINT ( 'NONE',  ( -6.594145116354495961, 6.771750247812114765, -0.2697605348319087604 ) ) ;
#203414=CARTESIAN_POINT ( 'NONE',  ( 4.588833619725765978, 8.479441126791286365, 0.4148976642893330014 ) ) ;
#203424=CARTESIAN_POINT ( 'NONE',  ( 3.953084306836263995, 6.769626237021087789, 1.199719254218452047 ) ) ;
#203433=CARTESIAN_POINT ( 'NONE',  ( 6.607619761813720238, 8.802252036906432764, 1.599625672291268286 ) ) ;
#203435=CARTESIAN_POINT ( 'NONE',  ( 6.879836604291781121, 6.991173891287354003, -0.7998128361456341429 ) ) ;
#203448=CARTESIAN_POINT ( 'NONE',  ( 6.321627859881460587, 6.858947107989728842, -0.6823232096292205506 ) ) ;
#203450=CARTESIAN_POINT ( 'NONE',  ( 4.556949027968946631, 8.330541276023501140, -0.7216878364870357165 ) ) ;
#203459=CARTESIAN_POINT ( 'NONE',  ( -3.984117037569407938, 5.741498858621315371, 1.599625672291270506 ) ) ;
#203469=CARTESIAN_POINT ( 'NONE',  ( -5.275531169048911728, 6.287779464379406491, -1.082531754730549967 ) ) ;
#203474=CARTESIAN_POINT ( 'NONE',  ( 5.071631979963703962, 8.074598522336444262, 1.199719254218451159 ) ) ;
#203490=CARTESIAN_POINT ( 'NONE',  ( -2.795860172527854903, 2.967839529530329479, -2.452799336324934742 ) ) ;
#203512=LINE ( 'NONE', #195573, #169960 ) ;
#203529=CARTESIAN_POINT ( 'NONE',  ( 4.394251184604942573, 8.140727125432185574, -0.7216878364870246143 ) ) ;
#203531=CARTESIAN_POINT ( 'NONE',  ( 3.445180431648313224, 7.033477913649446300, 0.7216878364870257245 ) ) ;
#203537=CARTESIAN_POINT ( 'NONE',  ( -8.120407659942227241, 8.438506789546210030, 0.7998128361456341429 ) ) ;
#203539=CARTESIAN_POINT ( 'NONE',  ( 7.147083253059300922, 8.367293879104554577, 1.199719254218452935 ) ) ;
#203542=CARTESIAN_POINT ( 'NONE',  ( -4.014622883422322985, 7.697827440719083647, -0.7216878364870458196 ) ) ;
#203547=CYLINDRICAL_SURFACE ( 'NONE', #44461, 1.250000000000000000 ) ;
#203565=CARTESIAN_POINT ( 'NONE',  ( 6.749980374757213575, 8.968339418673846097, 1.599625672291268286 ) ) ;
#203576=CARTESIAN_POINT ( 'NONE',  ( 6.482206841109512396, 9.616306177052839743, -1.082531754730548412 ) ) ;
#203588=CARTESIAN_POINT ( 'NONE',  ( -6.021229618244897885, 7.157760988441397743, 1.082531754730548412 ) ) ;
#203591=CARTESIAN_POINT ( 'NONE',  ( 7.876360894896227371, 8.153785563659219804, -0.7998128361456341429 ) ) ;
#203596=CARTESIAN_POINT ( 'NONE',  ( -4.655245641445871385, 6.524482229810530498, 1.599625672291263179 ) ) ;
#203605=CARTESIAN_POINT ( 'NONE',  ( 2.878073747850912412, 6.579779482459851003, -0.7998128361456362523 ) ) ;
#203624=VERTEX_POINT ( 'NONE', #190533 ) ;
#203636=CARTESIAN_POINT ( 'NONE',  ( 3.268924434670684498, 6.827845917175511481, -1.734723475976807094E-15 ) ) ;
#203640=CARTESIAN_POINT ( 'NONE',  ( -6.740338644649361832, 7.892758502626242567, -1.199719254218452047 ) ) ;
#203644=CARTESIAN_POINT ( 'NONE',  ( -4.098307573080856692, 8.003385611894792362, 0.7998128361456352531 ) ) ;
#203645=CARTESIAN_POINT ( 'NONE',  ( -5.655686355556086120, 6.627330832017406692, 1.199719254218452935 ) ) ;
#203649=CARTESIAN_POINT ( 'NONE',  ( -7.078765599666485997, 7.431183752465250869, 0.000000000000000000 ) ) ;
#203652=B_SPLINE_CURVE_WITH_KNOTS ( 'NONE', 3,
 ( #69788, #119701, #166252, #52500, #87133, #153204 ),
 .UNSPECIFIED., .F., .F.,
 ( 4, 2, 4 ),
 ( 0.000000000000000000, 0.5000000000000001110, 1.000000000000000000 ),
 .UNSPECIFIED. ) ;
#203657=CARTESIAN_POINT ( 'NONE',  ( -3.709037541790315640, 6.484905011134099340, -1.199719254218450271 ) ) ;
#203665=CARTESIAN_POINT ( 'NONE',  ( -6.688968683495758683, 8.897159112202094988, -1.599625672291271394 ) ) ;
#203667=CARTESIAN_POINT ( 'NONE',  ( 4.681345713234763117, 8.384430392927429310, -0.5894114041281351968 ) ) ;
#203672=CARTESIAN_POINT ( 'NONE',  ( 4.492547798081839794, 6.334668079219206049, 1.599625672291262513 ) ) ;
#203683=CARTESIAN_POINT ( 'NONE',  ( -7.584860592202423035, 7.813701877183096833, -0.7998128361456362523 ) ) ;
#203685=ORIENTED_EDGE ( 'NONE', *, *, #6236, .T. ) ;
#203693=EDGE_CURVE ( 'NONE', #100096, #44672, #178573, .T. ) ;
#203696=CARTESIAN_POINT ( 'NONE',  ( 6.535912570239620578, 9.782925877658371405, 1.199719254218452047 ) ) ;
#203708=CARTESIAN_POINT ( 'NONE',  ( 0.3620597222943388038, 2.804586296877760621, 2.034343604466669397 ) ) ;
#203709=CARTESIAN_POINT ( 'NONE',  ( 5.803742400754204667, 7.332416669035665358, 1.290654366993408297 ) ) ;
#203737=CARTESIAN_POINT ( 'NONE',  ( -5.889893629278568632, 7.264407438959931795, 1.268144897863663356 ) ) ;
#203758=CARTESIAN_POINT ( 'NONE',  ( -5.631432701629818460, 7.663367133358481631, 1.599625672291263179 ) ) ;
#203774=CARTESIAN_POINT ( 'NONE',  ( 3.223806664999388172, 6.983134552466421674, -0.7998128361456362523 ) ) ;
#203790=CARTESIAN_POINT ( 'NONE',  ( 6.215487077222150880, 6.216099443039444949, 0.000000000000000000 ) ) ;
#203800=CARTESIAN_POINT ( 'NONE',  ( -3.630551273409382329, 7.457669928944732796, 0.7998128361456352531 ) ) ;
#203802=CARTESIAN_POINT ( 'NONE',  ( 3.573456005653643519, 6.326726552307992080, -1.199719254218453823 ) ) ;
#203807=CARTESIAN_POINT ( 'NONE',  ( -6.394605727500880299, 7.489403432619674561, -1.199719254218452047 ) ) ;
#203810=CARTESIAN_POINT ( 'NONE',  ( 5.189738938980948291, 9.276722205444929870, 0.000000000000000000 ) ) ;
#203815=CARTESIAN_POINT ( 'NONE',  ( -5.321855017605967575, 7.728530711523490027, 1.321107644836617467 ) ) ;
#203825=CARTESIAN_POINT ( 'NONE',  ( -5.465345319640241506, 5.548860092434608760, 0.7216878364870257245 ) ) ;
#203835=CARTESIAN_POINT ( 'NONE',  ( 4.584065335196260804, 6.441438539186039591, 1.443375672974065660 ) ) ;
#203839=CARTESIAN_POINT ( 'NONE',  ( -5.738844160334429567, 9.917344963690652548, 0.000000000000000000 ) ) ;
#203841=EDGE_LOOP ( 'NONE', ( #204035, #186901, #207422, #45858, #14339, #197827, #198217, #89840 ) ) ;
#203846=B_SPLINE_CURVE_WITH_KNOTS ( 'NONE', 3,
 ( #204490, #138468, #89731, #155779, #7364, #73441, #8441, #74529, #205571, #90792, #40975, #107086, #189336, #173108, #123369, #156856, #24688, #57209, #80327, #199383, #182070, #196221, #16368, #117152, #49961, #130227, #112903, #113974, #64084 ),
 .UNSPECIFIED., .F., .F.,
 ( 4, 2, 2, 2, 2, 2, 2, 2, 2, 2, 2, 1, 1, 1, 2, 4 ),
 ( 0.3664058785177394806, 0.3808373650965696244, 0.3952688516753998238, 0.4097003382542300232, 0.4241318248330601670, 0.4385633114118903109, 0.4457790547013054105, 0.4529947979907205102, 0.4674262845695507096, 0.4746420278589658093, 0.4782498995036733036, 0.4800538353260270785, 0.4809558032372039382, 0.4814067871927923403, 0.4816322791705865969, 0.4818577711483807979 ),
 .UNSPECIFIED. ) ;
#203854=CARTESIAN_POINT ( 'NONE',  ( 2.911969131885072670, 6.619324097166378706, 0.000000000000000000 ) ) ;
#203859=CARTESIAN_POINT ( 'NONE',  ( -4.891620403477875634, 4.880467829835995808, -0.5985276763357317842 ) ) ;
#203870=ORIENTED_EDGE ( 'NONE', *, *, #52880, .T. ) ;
#203882=CARTESIAN_POINT ( 'NONE',  ( -5.492461627311929995, 5.580495784718250363, 0.000000000000000000 ) ) ;
#203895=VERTEX_POINT ( 'NONE', #70116 ) ;
#203906=CARTESIAN_POINT ( 'NONE',  ( -8.120407659942227241, 8.438506789546210030, 0.7998128361456341429 ) ) ;
#203912=CARTESIAN_POINT ( 'NONE',  ( -3.311934663488232733, 7.085950550703385531, -0.7998128361456481317 ) ) ;
#203919=CARTESIAN_POINT ( 'NONE',  ( -4.787964524281469458, 5.614988695530339413, -1.199719254218453823 ) ) ;
#203925=CARTESIAN_POINT ( 'NONE',  ( 5.041653019435334393, 6.975290837464928728, -1.599625672291269396 ) ) ;
#203930=CARTESIAN_POINT ( 'NONE',  ( -6.017840079619296567, 8.114175741012878973, -1.599625672291271394 ) ) ;
#203933=CARTESIAN_POINT ( 'NONE',  ( -3.634467696915153034, 6.397906858779740524, 1.199719254218452935 ) ) ;
#203937=CARTESIAN_POINT ( 'NONE',  ( 3.716343503477301802, 7.349834830783237294, -1.734723475976807094E-15 ) ) ;
#203938=CARTESIAN_POINT ( 'NONE',  ( -5.953438849732214599, 6.118302544208584770, 0.7216878364870257245 ) ) ;
#203942=CARTESIAN_POINT ( 'NONE',  ( -6.310394152517828203, 6.326824364217715768, 0.7998128361456282587 ) ) ;
#203945=CARTESIAN_POINT ( 'NONE',  ( 5.090160327287878594, 4.903218234782778850, -0.7998128361456481317 ) ) ;
#203957=CARTESIAN_POINT ( 'NONE',  ( 5.355371708033295874, 7.701368364266228284, 1.317571137710125351 ) ) ;
#203962=DIRECTION ( 'NONE',  ( 0.2553790820074260948, 0.9650728656995758437, 0.05844560174600864355 ) ) ;
#203967=CARTESIAN_POINT ( 'NONE',  ( 5.352436782344940802, 9.466536356036257871, 0.000000000000000000 ) ) ;
#203976=CARTESIAN_POINT ( 'NONE',  ( 6.484283628081795037, 6.752753718119230975, 0.1579380340677779548 ) ) ;
#203991=CARTESIAN_POINT ( 'NONE',  ( -6.143779885648060102, 7.196773283791382703, 1.199719254218452047 ) ) ;
#204004=CARTESIAN_POINT ( 'NONE',  ( 5.712781623311797397, 7.758274208654143855, -1.599625672291283607 ) ) ;
#204017=CARTESIAN_POINT ( 'NONE',  ( 5.519577934094864524, 5.612131475965050242, 0.7216878364870328300 ) ) ;
#204026=VERTEX_POINT ( 'NONE', #186010 ) ;
#204029=CARTESIAN_POINT ( 'NONE',  ( -5.465345320084574965, 9.390336950158399532, 0.000000000000000000 ) ) ;
#204030=CARTESIAN_POINT ( 'NONE',  ( 7.349928672384120176, 7.747540670635879145, 0.7216878364870267237 ) ) ;
#204035=ORIENTED_EDGE ( 'NONE', *, *, #131165, .T. ) ;
#204040=CARTESIAN_POINT ( 'NONE',  ( -5.635349125135588721, 6.603604063193491136, 1.199719254218452935 ) ) ;
#204041=CARTESIAN_POINT ( 'NONE',  ( -7.485510208520816278, 8.866088343763324886, 1.082531754730549078 ) ) ;
#204043=CARTESIAN_POINT ( 'NONE',  ( 6.549997608733495902, 7.774656977344789333, -1.082531754730548412 ) ) ;
#204054=CARTESIAN_POINT ( 'NONE',  ( -4.900660301121059881, 8.037431844279481652, -0.9627648694432132670 ) ) ;
#204058=CARTESIAN_POINT ( 'NONE',  ( 4.584065335196260804, 6.441438539186039591, 1.443375672974065660 ) ) ;
#204063=CARTESIAN_POINT ( 'NONE',  ( -6.818824913030298696, 6.919993584815607335, 0.7998128361456341429 ) ) ;
#204075=CARTESIAN_POINT ( 'NONE',  ( 5.740951700743842423, 5.662474837148078421, -0.7998128361456481317 ) ) ;
#204112=CARTESIAN_POINT ( 'NONE',  ( 7.024532985656141371, 7.367912369453226695, 0.7216878364870328300 ) ) ;
#204116=SPHERICAL_SURFACE ( 'NONE', #133770, 0.08000000000000000167 ) ;
#204117=CARTESIAN_POINT ( 'NONE',  ( 6.495764994278797388, 8.671754808115688107, 1.443375672974063439 ) ) ;
#204131=CARTESIAN_POINT ( 'NONE',  ( -7.119966945832006289, 8.335658187339330283, 1.199719254218452047 ) ) ;
#204140=CARTESIAN_POINT ( 'NONE',  ( -3.006876207180748217, 6.730049018344652190, -0.7998128361456481317 ) ) ;
#204142=CARTESIAN_POINT ( 'NONE',  ( 3.241808126998965811, 6.796210224891872542, 0.7216878364870257245 ) ) ;
#204148=CARTESIAN_POINT ( 'NONE',  ( -3.006876207180748217, 6.730049018344652190, -0.7998128361456481317 ) ) ;
#204154=CARTESIAN_POINT ( 'NONE',  ( -5.478903473698241378, 9.406154796041011679, -0.7216878364870338292 ) ) ;
#204157=CARTESIAN_POINT ( 'NONE',  ( -8.072954122294394352, 8.383144328957069291, -0.7998128361456362523 ) ) ;
#204162=CARTESIAN_POINT ( 'NONE',  ( -6.120580001926503755, 6.105374521861167914, -0.7998128361456362523 ) ) ;
#204175=CARTESIAN_POINT ( 'NONE',  ( -3.689227196694341515, 7.318199139536432973, -0.7216878364870458196 ) ) ;
#204178=CARTESIAN_POINT ( 'NONE',  ( -4.299344108864953995, 7.069632989434141201, -1.082531754730551743 ) ) ;
#204180=CARTESIAN_POINT ( 'NONE',  ( 5.682802662783380754, 6.658966523782627434, 1.199719254218452935 ) ) ;
#204181=CARTESIAN_POINT ( 'NONE',  ( -4.956387674247580755, 7.940146832334256111, 1.199719254218452935 ) ) ;
#204182=CARTESIAN_POINT ( 'NONE',  ( -6.526270840131767059, 8.707344961610770540, -1.599625672291271394 ) ) ;
#204189=ORIENTED_EDGE ( 'NONE', *, *, #193885, .T. ) ;
#204195=ORIENTED_EDGE ( 'NONE', *, *, #16602, .T. ) ;
#204203=CARTESIAN_POINT ( 'NONE',  ( 5.254667053748194760, 8.288139441751686931, 1.199719254218452047 ) ) ;
#204235=CARTESIAN_POINT ( 'NONE',  ( 5.765600714192544274, 7.067438534623806667, -2.440103264412656348 ) ) ;
#204243=CARTESIAN_POINT ( 'NONE',  ( 6.547661840756936691, 6.603636667163397256, 0.7998128361456352531 ) ) ;
#204261=CARTESIAN_POINT ( 'NONE',  ( 3.393283585170187688, 7.180857625999046867, 0.7998128361456271485 ) ) ;
#204265=ORIENTED_EDGE ( 'NONE', *, *, #155084, .F. ) ;
#204266=CARTESIAN_POINT ( 'NONE',  ( -7.449279056065764237, 7.655523418356991350, 0.7998128361456341429 ) ) ;
#204271=CARTESIAN_POINT ( 'NONE',  ( 4.050854035433010480, 7.948023151305657841, 0.000000000000000000 ) ) ;
#204281=ORIENTED_EDGE ( 'NONE', *, *, #63015, .F. ) ;
#204282=CARTESIAN_POINT ( 'NONE',  ( 5.831415467653547680, 8.857049574687536619, -1.082531754730548412 ) ) ;
#204283=CARTESIAN_POINT ( 'NONE',  ( -3.499413046103020175, 7.096749297179887783, 0.7216878364870338292 ) ) ;
#204284=CARTESIAN_POINT ( 'NONE',  ( -6.798487682609798632, 6.896266815991691779, 0.7998128361456341429 ) ) ;
#204297=CARTESIAN_POINT ( 'NONE',  ( 4.030516805012513082, 7.924296382481737844, 0.000000000000000000 ) ) ;
#204298=CARTESIAN_POINT ( 'NONE',  ( 4.525389411911321602, 8.501647757197021704, -0.7998128361456381397 ) ) ;
#204301=CARTESIAN_POINT ( 'NONE',  ( 5.501576472095266901, 9.640532660744973725, -0.7998128361456481317 ) ) ;
#204315=CARTESIAN_POINT ( 'NONE',  ( 5.911136963822321455, 7.250628055112136039, -1.245581879728396846 ) ) ;
#204319=CARTESIAN_POINT ( 'NONE',  ( 4.869313445963426190, 5.709895770826003414, 1.199719254218452935 ) ) ;
#204324=CARTESIAN_POINT ( 'NONE',  ( 3.627688620108284745, 6.389997935838436227, 1.199719254218452047 ) ) ;
#204328=CARTESIAN_POINT ( 'NONE',  ( 6.668631453075247073, 8.873432343378178544, -1.599625672291281386 ) ) ;
#204333=CARTESIAN_POINT ( 'NONE',  ( 5.939880696562888751, 7.062853913145737295, -1.082531754730548412 ) ) ;
#204335=CARTESIAN_POINT ( 'NONE',  ( -6.479871072688648148, 6.524547437750345402, 0.000000000000000000 ) ) ;
#204337=CARTESIAN_POINT ( 'NONE',  ( 4.686278372178935392, 5.496354851410763409, 1.199719254218452047 ) ) ;
#204345=CARTESIAN_POINT ( 'NONE',  ( -5.487584206907313522, 6.516568040952106067, -1.094815266226579098 ) ) ;
#204348=CARTESIAN_POINT ( 'NONE',  ( 6.348661983278831578, 6.841051910588018536, 0.6299351563821649069 ) ) ;
#204349=CARTESIAN_POINT ( 'NONE',  ( -5.008811405605897882, 4.808311159487113073, 0.7998128361456281477 ) ) ;
#204370=ADVANCED_FACE ( 'NONE', ( #175137 ), #4200, .T. ) ;
#204386=CARTESIAN_POINT ( 'NONE',  ( 8.154303043976348420, 8.478051404252736845, 0.7998128361456281477 ) ) ;
#204388=ADVANCED_FACE ( 'NONE', ( #166936 ), #82465, .F. ) ;
#204389=CARTESIAN_POINT ( 'NONE',  ( 5.338878628731272613, 9.450718510153643948, -0.7998128361456481317 ) ) ;
#204404=CARTESIAN_POINT ( 'NONE',  ( -5.101610940492132151, 9.173906207207963348, -0.7998128361456362523 ) ) ;
#204406=CARTESIAN_POINT ( 'NONE',  ( 7.146556367734776316, 7.510272981878305387, 0.7216878364870267237 ) ) ;
#204415=CARTESIAN_POINT ( 'NONE',  ( -4.111865726694519552, 8.019203457777400956, 0.000000000000000000 ) ) ;
#204420=CARTESIAN_POINT ( 'NONE',  ( -3.634994582239682526, 6.294558541704648569, 1.082531754730549967 ) ) ;
#204423=CARTESIAN_POINT ( 'NONE',  ( -3.298376509874564988, 7.070132704820777825, 0.000000000000000000 ) ) ;
#204447=CARTESIAN_POINT ( 'NONE',  ( -5.224688093219839402, 7.188831756880171397, -1.599625672291271394 ) ) ;
#204459=FACE_OUTER_BOUND ( 'NONE', #154134, .T. ) ;
#204473=CARTESIAN_POINT ( 'NONE',  ( -4.145761110728687804, 8.058748072483927771, -0.7998128361456481317 ) ) ;
#204474=CARTESIAN_POINT ( 'NONE',  ( 7.013428937081384262, 5.939655416065873439, 2.436399677959149024 ) ) ;
#204490=CARTESIAN_POINT ( 'NONE',  ( -5.980802423990385641, 6.150226714305422782, 9.481663569016276247E-06 ) ) ;
#204494=CARTESIAN_POINT ( 'NONE',  ( 4.980641328173811999, 6.904110530993182948, 1.599625672291269396 ) ) ;
#204502=CARTESIAN_POINT ( 'NONE',  ( 7.198453214212898743, 7.362893269528701268, 0.7998128361456291469 ) ) ;
#204504=CARTESIAN_POINT ( 'NONE',  ( 4.844006021832467646, 8.873367135438366304, 0.000000000000000000 ) ) ;
#204517=CARTESIAN_POINT ( 'NONE',  ( 5.954584599377941601, 7.113081392617206511, -1.094866876611422235 ) ) ;
#204518=AXIS2_PLACEMENT_3D ( 'NONE', #123971, #170484, #5823 ) ;
#204520=CARTESIAN_POINT ( 'NONE',  ( 5.939880696562888751, 7.062853913145737295, -1.082531754730548412 ) ) ;
#204537=B_SPLINE_CURVE_WITH_KNOTS ( 'NONE', 3,
 ( #16187, #15132, #98539, #130057 ),
 .UNSPECIFIED., .F., .F.,
 ( 4, 4 ),
 ( 0.003367049630611286277, 0.004112888465975162409 ),
 .UNSPECIFIED. ) ;
#204540=CARTESIAN_POINT ( 'NONE',  ( -5.112833325684908559, 8.018703742390766109, -1.082531754730549967 ) ) ;
#204544=CARTESIAN_POINT ( 'NONE',  ( 5.982890925380405456, 10.20206618957764100, 0.000000000000000000 ) ) ;
#204561=CARTESIAN_POINT ( 'NONE',  ( 5.155843554946782703, 9.237177590738404831, -0.7998128361456481317 ) ) ;
#204577=EDGE_CURVE ( 'NONE', #89251, #38200, #72104, .T. ) ;
#204601=CARTESIAN_POINT ( 'NONE',  ( 4.828112100242277549, 6.726159765073026264, -1.443375672974068769 ) ) ;
#204607=CARTESIAN_POINT ( 'NONE',  ( -7.608060475923978494, 8.905100639113307182, 1.199719254218452047 ) ) ;
#204613=CARTESIAN_POINT ( 'NONE',  ( -3.675669043080673770, 7.302381293653823491, 0.000000000000000000 ) ) ;
#204643=CARTESIAN_POINT ( 'NONE',  ( 3.067887898442204442, 6.801229324816399746, 0.7998128361456271485 ) ) ;
#204645=EDGE_CURVE ( 'NONE', #23400, #139590, #120693, .T. ) ;
#204657=CARTESIAN_POINT ( 'NONE',  ( -5.695833931516914639, 6.778132687258748845, 1.082531754730549078 ) ) ;
#204659=CARTESIAN_POINT ( 'NONE',  ( 6.176621499477501054, 9.363752961769195693, -1.199719254218452047 ) ) ;
#204675=DIRECTION ( 'NONE',  ( 0.000000000000000000, 0.000000000000000000, -1.000000000000000000 ) ) ;
#204702=CARTESIAN_POINT ( 'NONE',  ( 5.099275172515607579, 5.121778254122544283, -0.7216878364870458196 ) ) ;
#204706=CARTESIAN_POINT ( 'NONE',  ( -5.908321080505254841, 10.11506803722328129, 0.7998128361456291469 ) ) ;
#204709=CARTESIAN_POINT ( 'NONE',  ( -5.424143973919053785, 8.485862515284315677, 1.199719254218454489 ) ) ;
#204710=CARTESIAN_POINT ( 'NONE',  ( -3.983063267364693960, 7.868933921892603323, -0.7998128361456481317 ) ) ;
#204712=ORIENTED_EDGE ( 'NONE', *, *, #138377, .F. ) ;
#204715=CARTESIAN_POINT ( 'NONE',  ( -7.417719440008134768, 7.826629899530511025, 0.7216878364870317197 ) ) ;
#204721=CARTESIAN_POINT ( 'NONE',  ( -4.248501033035892327, 6.049946853332221153, -1.599625672291271394 ) ) ;
#204728=VECTOR ( 'NONE', #49929, 1000.000000000000114 ) ;
#204729=CARTESIAN_POINT ( 'NONE',  ( -7.618755976236585958, 7.853246491889623648, 0.000000000000000000 ) ) ;
#204731=CARTESIAN_POINT ( 'NONE',  ( 4.890561790263044273, 8.149264200713410844, -1.004099907704804950 ) ) ;
#204737=CARTESIAN_POINT ( 'NONE',  ( 5.259637247458703868, 5.100941308315409373, 0.000000000000000000 ) ) ;
#204742=DIRECTION ( 'NONE',  ( 1.000000000000000000, 0.000000000000000000, 0.000000000000000000 ) ) ;
#204747=CARTESIAN_POINT ( 'NONE',  ( -5.912237504011027767, 9.055304967058290799, 1.199719254218454489 ) ) ;
#204750=CARTESIAN_POINT ( 'NONE',  ( 3.894033820048811823, 8.999999999999998224, -0.7749999999999996891 ) ) ;
#204759=CARTESIAN_POINT ( 'NONE',  ( 5.494797395288433250, 9.632623737803665875, 0.000000000000000000 ) ) ;
#204773=CARTESIAN_POINT ( 'NONE',  ( 5.753927575595171540, 7.371122731025397279, 1.306365966420112601 ) ) ;
#204780=FACE_OUTER_BOUND ( 'NONE', #200608, .T. ) ;
#204803=CARTESIAN_POINT ( 'NONE',  ( -6.584207447892295839, 6.778236197985048506, 0.3223495580488393575 ) ) ;
#204817=CARTESIAN_POINT ( 'NONE',  ( 3.568415406894422492, 7.340509688221367846, -0.2824851646710802022 ) ) ;
#204821=CARTESIAN_POINT ( 'NONE',  ( -5.875479466675803231, 7.948088359245467416, -1.599625672291271394 ) ) ;
#204832=ORIENTED_EDGE ( 'NONE', *, *, #84212, .T. ) ;
#204833=CARTESIAN_POINT ( 'NONE',  ( -5.346851039111035320, 6.199209027673978412, 2.420000000000001261 ) ) ;
#204839=CARTESIAN_POINT ( 'NONE',  ( 4.549643065837591038, 7.465611455855944101, -1.199719254218452047 ) ) ;
#204842=LINE ( 'NONE', #155061, #93891 ) ;
#204848=CARTESIAN_POINT ( 'NONE',  ( 5.054560120293923653, 7.862967615930308796, 1.113740650586869219 ) ) ;
#204849=CARTESIAN_POINT ( 'NONE',  ( -6.329444829450759258, 6.903589915222720919, 0.7840647185534960206 ) ) ;
#204866=CARTESIAN_POINT ( 'NONE',  ( -3.481411583659053566, 7.283673624236017830, 0.000000000000000000 ) ) ;
#204868=CARTESIAN_POINT ( 'NONE',  ( 3.711900195091365262, 7.552577004240394132, -0.7998128361456362523 ) ) ;
#204869=CARTESIAN_POINT ( 'NONE',  ( -3.147653791585729444, 8.920000000000001705, 2.419999999999999485 ) ) ;
#204871=CARTESIAN_POINT ( 'NONE',  ( -7.273023059088104425, 7.449891421883056530, 0.000000000000000000 ) ) ;
#204873=ORIENTED_EDGE ( 'NONE', *, *, #68379, .F. ) ;
#204874=CARTESIAN_POINT ( 'NONE',  ( 7.537407054554579489, 7.758339416593960536, 0.000000000000000000 ) ) ;
#204882=CARTESIAN_POINT ( 'NONE',  ( -4.607972389651186162, 8.469779238289159906, 0.3137405545926199579 ) ) ;
#204892=CARTESIAN_POINT ( 'NONE',  ( -4.462041952228954500, 6.299077925724123617, -1.443375672974066548 ) ) ;
#204902=CARTESIAN_POINT ( 'NONE',  ( 5.261973015879598314, 5.311592404713873172, -0.7216878364870458196 ) ) ;
#204907=CARTESIAN_POINT ( 'NONE',  ( -6.749980374757255319, 8.968339418673846097, 1.599625672291269396 ) ) ;
#204927=CARTESIAN_POINT ( 'NONE',  ( 6.547661840756935803, 6.603636667163397256, 0.7998128361456350310 ) ) ;
#204950=CARTESIAN_POINT ( 'NONE',  ( -5.153507786970276783, 6.145418851954329575, -1.082531754730549967 ) ) ;
#204975=CARTESIAN_POINT ( 'NONE',  ( -6.851666526859749418, 9.086973262793417661, -1.599625672291271394 ) ) ;
#204977=FACE_OUTER_BOUND ( 'NONE', #107943, .T. ) ;
#204983=CARTESIAN_POINT ( 'NONE',  ( -4.634908411025374875, 6.500755460986618495, 1.599625672291263179 ) ) ;
#204993=CARTESIAN_POINT ( 'NONE',  ( -5.517242166118370150, 5.401480380085008193, 0.7998128361456281477 ) ) ;
#204995=CARTESIAN_POINT ( 'NONE',  ( 6.246047416222394233, 7.008439898793222156, -0.9866338212708870570 ) ) ;
#204999=CARTESIAN_POINT ( 'NONE',  ( 3.854260808034858155, 7.718664386007802136, -0.7998128361456362523 ) ) ;
#205004=CARTESIAN_POINT ( 'NONE',  ( -6.961185525973791144, 7.086080966583015339, 0.7998128361456341429 ) ) ;
#205007=CARTESIAN_POINT ( 'NONE',  ( -3.149236820124241110, 6.896136400112061970, -0.7998128361456481317 ) ) ;
#205013=CARTESIAN_POINT ( 'NONE',  ( 4.678972410047582464, 8.472901888448573615, -0.7216878364870357165 ) ) ;
#205014=CARTESIAN_POINT ( 'NONE',  ( -3.960390268523300339, 7.634556056670224855, 1.214306433183764966E-14 ) ) ;
#205021=CARTESIAN_POINT ( 'NONE',  ( 5.564695703766185275, 5.456842840674144490, 0.000000000000000000 ) ) ;
#205028=CARTESIAN_POINT ( 'NONE',  ( 4.044074958626150185, 7.940114228364351767, 0.7998128361456271485 ) ) ;
#205033=CARTESIAN_POINT ( 'NONE',  ( 4.873468316212648865, 8.167532512703042258, 0.9812947938723035612 ) ) ;
#205039=EDGE_LOOP ( 'NONE', ( #142883, #199857, #96714, #177995 ) ) ;
#205043=CARTESIAN_POINT ( 'NONE',  ( 4.552505719138623341, 8.533283448962240669, 0.7998128361456341429 ) ) ;
#205051=EDGE_CURVE ( 'NONE', #80820, #39859, #6054, .T. ) ;
#205055=CARTESIAN_POINT ( 'NONE',  ( 5.309622429108474151, 7.625948988765205883, 1.230663689527239812 ) ) ;
#205072=CARTESIAN_POINT ( 'NONE',  ( -6.444921918449773024, 8.612437886315108315, 1.599625672291269396 ) ) ;
#205085=CARTESIAN_POINT ( 'NONE',  ( 5.306037014901791693, 7.283738832175834510, 1.599625672291269396 ) ) ;
#205092=CARTESIAN_POINT ( 'NONE',  ( -7.607533590599451223, 9.008448956188397361, 1.082531754730549078 ) ) ;
#205094=CARTESIAN_POINT ( 'NONE',  ( 4.553559489343365740, 6.405848385690952718, -1.599625672291269396 ) ) ;
#205097=CARTESIAN_POINT ( 'NONE',  ( 5.248414861821569133, 6.256143772614186638, -1.082531754730548412 ) ) ;
#205111=CARTESIAN_POINT ( 'NONE',  ( -6.780486220610184134, 9.003929572168926754, -1.443375672974066548 ) ) ;
#205112=CARTESIAN_POINT ( 'NONE',  ( 6.753369913382843315, 8.011924666102361314, -1.082531754730548412 ) ) ;
#205115=EDGE_CURVE ( 'NONE', #19980, #95167, #9818, .T. ) ;
#205122=CARTESIAN_POINT ( 'NONE',  ( -4.502189528189771472, 7.410248995266807803, -1.199719254218453823 ) ) ;
#205123=CARTESIAN_POINT ( 'NONE',  ( -6.455090533882193782, 9.584670485287619002, -1.082531754730549967 ) ) ;
#205124=CARTESIAN_POINT ( 'NONE',  ( 7.160114521348466710, 7.526090827760914870, 0.000000000000000000 ) ) ;
#205136=CARTESIAN_POINT ( 'NONE',  ( -4.896236220255085314, 8.042264628280536343, 0.9566786516278618091 ) ) ;
#205139=CARTESIAN_POINT ( 'NONE',  ( 4.095971805104285934, 6.832365301713403838, 1.082531754730549078 ) ) ;
#205141=DIRECTION ( 'NONE',  ( 0.000000000000000000, 0.000000000000000000, 1.000000000000000000 ) ) ;
#205144=CARTESIAN_POINT ( 'NONE',  ( -5.094831863685302942, 9.165997284266655498, 0.7998128361456291469 ) ) ;
#205157=CARTESIAN_POINT ( 'NONE',  ( 4.854701522145073334, 7.821512988214679218, -1.199719254218450271 ) ) ;
#205174=CARTESIAN_POINT ( 'NONE',  ( 3.811250579217332568, 5.539821323877241355, 1.214306433183764966E-14 ) ) ;
#205196=CARTESIAN_POINT ( 'NONE',  ( 5.397554552016204710, 9.311247720745345902, 0.7216878364870317197 ) ) ;
#205201=CARTESIAN_POINT ( 'NONE',  ( 6.143253000323500856, 10.18122924377050609, -0.7216878364870458196 ) ) ;
#205225=CARTESIAN_POINT ( 'NONE',  ( -4.034433228518296666, 6.864533312316751790, -1.199719254218450271 ) ) ;
#205227=CARTESIAN_POINT ( 'NONE',  ( 6.183927461164522299, 6.387205924212962849, 0.000000000000000000 ) ) ;
#205233=CARTESIAN_POINT ( 'NONE',  ( -4.411198876399886615, 6.239761003923544713, -1.599625672291271394 ) ) ;
#205238=CARTESIAN_POINT ( 'NONE',  ( -5.953438850176548947, 9.959779401932374654, 0.000000000000000000 ) ) ;
#205246=CARTESIAN_POINT ( 'NONE',  ( -3.623772196602547346, 7.449761006003425834, 0.000000000000000000 ) ) ;
#205254=CARTESIAN_POINT ( 'NONE',  ( -2.428612866367529932E-14, 2.999999999999999112, 2.420000000000000373 ) ) ;
#205260=CARTESIAN_POINT ( 'NONE',  ( -4.448483799059637533, 7.243629294661272588, 1.082531754730549967 ) ) ;
#205262=CARTESIAN_POINT ( 'NONE',  ( -5.383996397958228819, 8.335060660042973524, 1.082531754730550855 ) ) ;
#205264=CARTESIAN_POINT ( 'NONE',  ( 4.929271367020211514, 7.908511140569038922, 1.199719254218452047 ) ) ;
#205265=CARTESIAN_POINT ( 'NONE',  ( -4.308458954092677651, 8.248562223075252220, -0.7998128361456362523 ) ) ;
#205267=CARTESIAN_POINT ( 'NONE',  ( -7.795011973214244883, 8.058878488363559356, 0.7998128361456341429 ) ) ;
#205268=CARTESIAN_POINT ( 'NONE',  ( -6.567365632596091629, 6.787193466117722451, -0.4468828428391571350 ) ) ;
#205270=CARTESIAN_POINT ( 'NONE',  ( 3.147653791585717453, 8.920000000000001705, -2.420000000000002149 ) ) ;
#205275=ORIENTED_EDGE ( 'NONE', *, *, #105631, .F. ) ;
#205289=CARTESIAN_POINT ( 'NONE',  ( 5.691390622686558487, 9.861982503101517139, 0.7998128361456341429 ) ) ;
#205320=CARTESIAN_POINT ( 'NONE',  ( 3.853900823549051502, 8.531065964594045425, -2.447540105570114477 ) ) ;
#205327=CARTESIAN_POINT ( 'NONE',  ( 4.227110032410640095, 8.153655147779589996, 0.7998128361456271485 ) ) ;
#205330=CARTESIAN_POINT ( 'NONE',  ( -3.546339698426324460, 6.295090860542775779, -1.199719254218450271 ) ) ;
#205345=CARTESIAN_POINT ( 'NONE',  ( 5.123001941117305336, 7.070197912760590064, 1.599625672291268286 ) ) ;
#205354=CARTESIAN_POINT ( 'NONE',  ( -7.045397100956844127, 8.248660034984974132, -1.199719254218452047 ) ) ;
#205358=CARTESIAN_POINT ( 'NONE',  ( 5.387385936583818591, 7.378645907471495846, -1.599625672291283607 ) ) ;
#205369=CARTESIAN_POINT ( 'NONE',  ( 5.695833931516881776, 9.659240330162777610, -0.7216878364870458196 ) ) ;
#205370=CARTESIAN_POINT ( 'NONE',  ( -3.851925040058345573, 5.587274861525073355, -1.443375672974078761 ) ) ;
#205371=CARTESIAN_POINT ( 'NONE',  ( -5.611095471209320174, 7.639640364534566075, 1.599625672291263179 ) ) ;
#205383=CARTESIAN_POINT ( 'NONE',  ( 5.071631979963703962, 8.074598522336444262, 1.199719254218451159 ) ) ;
#205384=CARTESIAN_POINT ( 'NONE',  ( 4.701645408888975197, 8.707279753670952971, 0.000000000000000000 ) ) ;
#205387=CARTESIAN_POINT ( 'NONE',  ( 6.444921918449731280, 8.612437886315108315, 1.599625672291268286 ) ) ;
#205393=DIRECTION ( 'NONE',  ( -0.000000000000000000, -0.000000000000000000, 1.000000000000000000 ) ) ;
#205401=CARTESIAN_POINT ( 'NONE',  ( 5.612152705277200226, 7.484198595525810127, -1.333638438132278559 ) ) ;
#205405=CARTESIAN_POINT ( 'NONE',  ( 4.224247379109608680, 7.085983154673295203, -1.199719254218452047 ) ) ;
#205410=CARTESIAN_POINT ( 'NONE',  ( 4.278479993564246797, 7.149254538203735798, 1.199719254218452047 ) ) ;
#205413=ADVANCED_FACE ( 'NONE', ( #27659 ), #158566, .T. ) ;
#205417=CARTESIAN_POINT ( 'NONE',  ( 8.154303043976348420, 8.478051404252736845, 0.7998128361456281477 ) ) ;
#205421=CARTESIAN_POINT ( 'NONE',  ( 6.373741612200174878, 6.608655767087927124, 0.7216878364870328300 ) ) ;
#205423=CARTESIAN_POINT ( 'NONE',  ( -6.414942957921379474, 7.513130201443591005, -1.199719254218452047 ) ) ;
#205425=CARTESIAN_POINT ( 'NONE',  ( 4.903208829997618423, 5.749440385532527564, -1.199719254218450271 ) ) ;
#205436=ADVANCED_FACE ( 'NONE', ( #59092 ), #33312, .T. ) ;
#205437=CARTESIAN_POINT ( 'NONE',  ( -3.688700311369816909, 6.461178242310183784, -1.199719254218450271 ) ) ;
#205469=CARTESIAN_POINT ( 'NONE',  ( 3.553645660557675612, 6.199651466408984568, -1.082531754730549967 ) ) ;
#205476=CARTESIAN_POINT ( 'NONE',  ( 8.039058738260216330, 8.343599714250547805, -0.7998128361456341429 ) ) ;
#205487=CARTESIAN_POINT ( 'NONE',  ( -6.445975688654487001, 6.485002823043819475, -0.7998128361456362523 ) ) ;
#205489=CARTESIAN_POINT ( 'NONE',  ( 5.844973620822823790, 9.833236634353070826, 0.7216878364870317197 ) ) ;
#205499=CARTESIAN_POINT ( 'NONE',  ( -4.960304097753355457, 6.880383762169266504, 1.599625672291263179 ) ) ;
#205504=CARTESIAN_POINT ( 'NONE',  ( -4.258669648468323743, 6.061810238003387141, 1.443375672974065660 ) ) ;
#205509=CARTESIAN_POINT ( 'NONE',  ( -4.014095998097799267, 6.840806543492835345, -1.199719254218450271 ) ) ;
#205530=CARTESIAN_POINT ( 'NONE',  ( -4.294900800479008574, 8.232744377192641849, 0.000000000000000000 ) ) ;
#205554=CARTESIAN_POINT ( 'NONE',  ( -6.306477729012051725, 7.386587434382707151, 1.199719254218452047 ) ) ;
#205555=CARTESIAN_POINT ( 'NONE',  ( -5.546112223000226216, 5.929839062422638918, -0.8878705470019981894 ) ) ;
#205562=CARTESIAN_POINT ( 'NONE',  ( 7.960045584554727327, 8.459343734834927631, 0.7216878364870267237 ) ) ;
#205563=ADVANCED_FACE ( 'NONE', ( #200019 ), #51671, .T. ) ;
#205571=CARTESIAN_POINT ( 'NONE',  ( -5.175390966358026645, 6.917902677759380836, 1.252160023617815643 ) ) ;
#205576=CARTESIAN_POINT ( 'NONE',  ( 4.817943484809818600, 6.714296380401858499, 1.599625672291269396 ) ) ;
#205584=CARTESIAN_POINT ( 'NONE',  ( 6.875920180786008196, 8.050936961452347163, -1.199719254218452047 ) ) ;
#205586=CARTESIAN_POINT ( 'NONE',  ( 5.668190738965027897, 8.770583741171307679, -1.199719254218452047 ) ) ;
#205599=CARTESIAN_POINT ( 'NONE',  ( 6.492781079782697695, 6.747302000852300807, 0.03582484399037785816 ) ) ;
#205601=CARTESIAN_POINT ( 'NONE',  ( 4.394251184604957672, 8.140727125432173139, -0.7216878364870357165 ) ) ;
#205609=CARTESIAN_POINT ( 'NONE',  ( -4.659162064951642535, 5.464719159645540003, 1.199719254218452935 ) ) ;
#205610=CARTESIAN_POINT ( 'NONE',  ( 3.615147460157889903, 7.348606074266929689, 0.4009180521483968196 ) ) ;
#205617=CARTESIAN_POINT ( 'NONE',  ( -6.278834536460198734, 6.497930845391236332, 0.7216878364870257245 ) ) ;
#205621=CARTESIAN_POINT ( 'NONE',  ( 7.506374323821472849, 8.786466794993730289, -1.199719254218452047 ) ) ;
#205623=CARTESIAN_POINT ( 'NONE',  ( -5.081322649207705489, 6.519081843335746029, -1.217513467538652305 ) ) ;
#205640=CARTESIAN_POINT ( 'NONE',  ( 4.844006021832467646, 8.873367135438366304, 0.000000000000000000 ) ) ;
#205659=CARTESIAN_POINT ( 'NONE',  ( -7.259464905474441565, 7.434073576000447048, -0.7998128361456362523 ) ) ;
#205671=CARTESIAN_POINT ( 'NONE',  ( 4.549612403093820312, 8.500000000000243361, -0.2314049244472246580 ) ) ;
#205680=CARTESIAN_POINT ( 'NONE',  ( 3.757017964762656703, 7.397288368949487491, -1.734723475976807094E-15 ) ) ;
#205685=CARTESIAN_POINT ( 'NONE',  ( -6.420668264523499147, 9.648474187656182366, 1.199719254218452935 ) ) ;
#205692=CARTESIAN_POINT ( 'NONE',  ( -4.665414256878301025, 6.536345614481700927, -1.443375672974066548 ) ) ;
#205695=ORIENTED_EDGE ( 'NONE', *, *, #172187, .F. ) ;
#205709=DIRECTION ( 'NONE',  ( 0.000000000000000000, 0.000000000000000000, -1.000000000000000000 ) ) ;
#205710=CARTESIAN_POINT ( 'NONE',  ( 5.858531774436539052, 6.007577623030311287, 0.000000000000000000 ) ) ;
#205724=CARTESIAN_POINT ( 'NONE',  ( 3.366167277942881064, 7.149221934233827014, -0.7998128361456362523 ) ) ;
#205733=CIRCLE ( 'NONE', #146876, 0.08000000000000015432 ) ;
#205736=CARTESIAN_POINT ( 'NONE',  ( -6.075462232699549325, 9.141770800574526845, 1.082531754730549967 ) ) ;
#205739=CARTESIAN_POINT ( 'NONE',  ( 7.364013710877980401, 8.620379413226322285, -1.199719254218452047 ) ) ;
#205756=CARTESIAN_POINT ( 'NONE',  ( 2.891631901464575272, 6.595597328342462262, 0.000000000000000000 ) ) ;
#205757=ORIENTED_EDGE ( 'NONE', *, *, #162598, .T. ) ;
#205758=CARTESIAN_POINT ( 'NONE',  ( -4.855228407469635243, 4.837057028235559386, 0.7216878364870257245 ) ) ;
#205791=CARTESIAN_POINT ( 'NONE',  ( -7.767895665986912057, 8.027242796598338614, -0.7998128361456362523 ) ) ;
#205794=CARTESIAN_POINT ( 'NONE',  ( -6.069210040772897052, 7.109775131437022999, -1.199719254218453823 ) ) ;
#205797=ORIENTED_EDGE ( 'NONE', *, *, #204645, .T. ) ;
#205799=CARTESIAN_POINT ( 'NONE',  ( -6.902509602688818191, 9.146290184594002781, -1.443375672974066548 ) ) ;
#205800=CARTESIAN_POINT ( 'NONE',  ( 5.994113310573177422, 10.00723293906178846, 0.000000000000000000 ) ) ;
#205806=CARTESIAN_POINT ( 'NONE',  ( -6.912678218121246942, 9.158153569265168770, 1.599625672291269396 ) ) ;
#205814=CARTESIAN_POINT ( 'NONE',  ( -7.781453819600577582, 8.043060642480948985, 0.000000000000000000 ) ) ;
#205816=CARTESIAN_POINT ( 'NONE',  ( 5.348725299209624140, 7.591689785053232775, -1.238827213252717163 ) ) ;
#205821=CARTESIAN_POINT ( 'NONE',  ( 4.869313445963426190, 5.709895770826003414, 1.199719254218452935 ) ) ;
#205828=DIRECTION ( 'NONE',  ( 1.000000000000000000, 0.000000000000000000, 0.000000000000000000 ) ) ;
#205832=CARTESIAN_POINT ( 'NONE',  ( -7.937372586157736443, 8.224965870130965584, 0.7998128361456341429 ) ) ;
#205835=DIRECTION ( 'NONE',  ( -0.000000000000000000, -0.000000000000000000, 1.000000000000000000 ) ) ;
#205845=CARTESIAN_POINT ( 'NONE',  ( 5.820193082016415609, 10.01225203898631655, 0.000000000000000000 ) ) ;
#205860=CARTESIAN_POINT ( 'NONE',  ( 6.606590233575550641, 6.765807905838774339, 0.03828827652692379235 ) ) ;
#205861=CARTESIAN_POINT ( 'NONE',  ( -3.811250578772981346, 6.500190537660166079, -1.082531754730546636 ) ) ;
#205889=CARTESIAN_POINT ( 'NONE',  ( 4.041212305325117882, 6.872442235258051646, -1.199719254218448494 ) ) ;
#205903=CARTESIAN_POINT ( 'NONE',  ( 1.833030277982334422, 9.001999999999998892, -2.500000000000000444 ) ) ;
#205907=CARTESIAN_POINT ( 'NONE',  ( -5.010620288702242853, 8.003418215864698482, -1.199719254218453823 ) ) ;
#205924=CARTESIAN_POINT ( 'NONE',  ( 4.441177836928239309, 7.339068688795062911, 1.199719254218452047 ) ) ;
#205926=CARTESIAN_POINT ( 'NONE',  ( 6.604230223188150894, 9.758666789477915771, -1.082531754730548412 ) ) ;
#205927=CARTESIAN_POINT ( 'NONE',  ( 5.096939404094710468, 4.911127157724081371, 0.000000000000000000 ) ) ;
#205936=CARTESIAN_POINT ( 'NONE',  ( 5.582388601459258304, 7.396495182493852738, 1.242574333668546638 ) ) ;
#205937=CARTESIAN_POINT ( 'NONE',  ( 6.204464077730128757, 7.037555732820855781, 1.030856974308017149 ) ) ;
#205955=CARTESIAN_POINT ( 'NONE',  ( -4.411198876399886615, 6.239761003923544713, -1.599625672291271394 ) ) ;
#205957=CARTESIAN_POINT ( 'NONE',  ( 5.747730777550676073, 5.670383760089384495, 0.000000000000000000 ) ) ;
#205960=CARTESIAN_POINT ( 'NONE',  ( -6.622231685632140596, 6.690634819517756959, 0.000000000000000000 ) ) ;
#205963=CARTESIAN_POINT ( 'NONE',  ( 6.038177310039780643, 8.137902509836795417, -1.599625672291283607 ) ) ;
#205968=CARTESIAN_POINT ( 'NONE',  ( -5.031572470839103417, 8.001347149079229837, -1.166850223539055875 ) ) ;
#205976=CARTESIAN_POINT ( 'NONE',  ( -5.112833325684916552, 7.058334528089422300, -1.443375672974066548 ) ) ;
#205984=CARTESIAN_POINT ( 'NONE',  ( 3.919715808126649659, 7.587102519540811940, 0.000000000000000000 ) ) ;
#205988=CARTESIAN_POINT ( 'NONE',  ( -7.598418745816086783, 7.829519723065708092, 0.000000000000000000 ) ) ;
#206002=CARTESIAN_POINT ( 'NONE',  ( 4.760848217054122422, 5.583353003765119560, -1.199719254218452047 ) ) ;
#206006=CARTESIAN_POINT ( 'NONE',  ( 4.389807875774629942, 8.343469298370917997, 0.7998128361456271485 ) ) ;
#206030=CARTESIAN_POINT ( 'NONE',  ( -6.183927461608886844, 7.347575139032721303, 1.082531754730548412 ) ) ;
#206045=EDGE_LOOP ( 'NONE', ( #80785, #38094, #145530, #61259, #92788 ) ) ;
#206055=CARTESIAN_POINT ( 'NONE',  ( -5.126391479298592735, 5.153413945369351268, 0.000000000000000000 ) ) ;
#206060=CARTESIAN_POINT ( 'NONE',  ( -5.496904935697871863, 5.377753611261092637, 0.7998128361456281477 ) ) ;
#206063=CARTESIAN_POINT ( 'NONE',  ( 1.843739406749204335, 8.920000000000001705, 0.7750000000000004663 ) ) ;
#206064=EDGE_LOOP ( 'NONE', ( #152002, #39429, #61575, #192476 ) ) ;
#206069=CARTESIAN_POINT ( 'NONE',  ( -8.072954122294394352, 8.383144328957069291, -0.7998128361456362523 ) ) ;
#206071=CARTESIAN_POINT ( 'NONE',  ( 6.587573780899039555, 6.778200402807202707, -0.2451836268814889253 ) ) ;
#206075=CARTESIAN_POINT ( 'NONE',  ( 4.692003678781083487, 7.631698837623355658, -1.199719254218450271 ) ) ;
#206080=CARTESIAN_POINT ( 'NONE',  ( -6.261886844665283114, 8.398896966899865646, 1.599625672291269396 ) ) ;
#206084=CARTESIAN_POINT ( 'NONE',  ( -3.984117037569407938, 5.741498858621315371, 1.599625672291270506 ) ) ;
#206089=CARTESIAN_POINT ( 'NONE',  ( 4.543390873910903238, 7.354354215321133204, 1.082531754730548412 ) ) ;
#206091=CARTESIAN_POINT ( 'NONE',  ( -4.895902867866254837, 7.765618208269001066, 1.082531754730549967 ) ) ;
#206095=CARTESIAN_POINT ( 'NONE',  ( -4.878955176071358757, 6.785476686873604280, -1.599625672291271394 ) ) ;
#206098=CARTESIAN_POINT ( 'NONE',  ( 5.063044020060520900, 4.871582543017558109, 0.7998128361456352531 ) ) ;
#206110=CARTESIAN_POINT ( 'NONE',  ( 5.420206975164616026, 7.644856803259713729, 1.330009527941821368 ) ) ;
#206121=CARTESIAN_POINT ( 'NONE',  ( 5.631432701629774051, 7.663367133358481631, 1.599625672291269396 ) ) ;
#206131=CARTESIAN_POINT ( 'NONE',  ( 6.453003701063230402, 6.772902045581084884, 0.3391303328579304277 ) ) ;
#206141=CARTESIAN_POINT ( 'NONE',  ( -4.721755537811513470, 8.238515690766082145, -0.6557258408305451924 ) ) ;
#206150=CARTESIAN_POINT ( 'NONE',  ( -5.447343857640614573, 9.577261277214532242, -0.7998128361456362523 ) ) ;
#206163=CARTESIAN_POINT ( 'NONE',  ( 6.230854113932139171, 9.427024345299638952, 1.199719254218452047 ) ) ;
#206168=CARTESIAN_POINT ( 'NONE',  ( -6.522881301506166629, 9.663759714182251770, 1.082531754730549967 ) ) ;
#206170=CARTESIAN_POINT ( 'NONE',  ( 4.065465959251388206, 5.836405933916976707, -1.599625672291269396 ) ) ;
#206173=CARTESIAN_POINT ( 'NONE',  ( 5.194182247366878613, 6.192872389083746043, 1.082531754730549078 ) ) ;
#206174=CARTESIAN_POINT ( 'NONE',  ( 5.602074566136501232, 5.729665287594564838, 0.6253354971682704155 ) ) ;
#206175=ORIENTED_EDGE ( 'NONE', *, *, #169774, .T. ) ;
#206187=CARTESIAN_POINT ( 'NONE',  ( -7.621091744657483069, 8.063897588288083895, 0.7216878364870317197 ) ) ;
#206188=CARTESIAN_POINT ( 'NONE',  ( 6.455090533882185788, 8.624301270986276080, -1.443375672974078761 ) ) ;
#206200=CARTESIAN_POINT ( 'NONE',  ( -6.134138155540168391, 6.121192367743780949, 0.000000000000000000 ) ) ;
#206201=CARTESIAN_POINT ( 'NONE',  ( -4.773352600463090845, 7.726605912919016106, 1.199719254218452935 ) ) ;
#206203=CARTESIAN_POINT ( 'NONE',  ( 5.844973620822823790, 9.833236634353070826, 0.7216878364870317197 ) ) ;
#206209=FACE_OUTER_BOUND ( 'NONE', #60735, .T. ) ;
#206215=CARTESIAN_POINT ( 'NONE',  ( -5.250728612101474901, 7.694385777474874288, -1.211319784145984846 ) ) ;
#206216=FACE_BOUND ( 'NONE', #10872, .T. ) ;
#206219=CARTESIAN_POINT ( 'NONE',  ( 3.418064124421011041, 7.001842221884225559, -0.7216878364870338292 ) ) ;
#206221=AXIS2_PLACEMENT_3D ( 'NONE', #202260, #22445, #90698 ) ;
#206225=CARTESIAN_POINT ( 'NONE',  ( -5.498713818794216834, 8.572860667638675380, -1.199719254218452047 ) ) ;
#206239=CARTESIAN_POINT ( 'NONE',  ( 4.908934136599710563, 7.884784371745123366, 1.199719254218451159 ) ) ;
#206263=DIRECTION ( 'NONE',  ( -0.000000000000000000, -0.000000000000000000, -1.000000000000000000 ) ) ;
#206278=CARTESIAN_POINT ( 'NONE',  ( 6.590672070018850803, 7.822110515511036866, -1.082531754730548412 ) ) ;
#206282=CARTESIAN_POINT ( 'NONE',  ( 6.821160681006788629, 8.091013894996997635, 1.082531754730549967 ) ) ;
#206300=( BOUNDED_SURFACE ( )  B_SPLINE_SURFACE ( 1, 2, ( 
 ( #124127, #7048, #53697, #37440, #73124, #190089, #107853, #203119, #70980, #173879, #91560, #54761, #157616, #9213, #120910, #75284, #186882, #143528, #26523, #60094, #209524, #145666, #95828, #96898, #30819, #10270, #27594, #211664, #108919, #76345, #92632, #44942, #174941, #61165, #162947, #128397, #93692, #127327, #158673, #113190, #59027, #179196, #142453, #210610, #159735, #111049, #193297, #77412, #43874, #78477, #129460, #177056, #109990, #28673, #11333, #144596, #195443, #94758, #160807, #62238, #208461, #126253, #112125, #12398, #194364, #46006, #178129, #192212, #29745, #176002, #161885, #13472, #79548, #47073, #63300, #14527, #80624, #207408, #125185, #191146, #42812, #50248, #131548, #133668, #36109, #149892, #147761, #1458, #146714, #97957, #31879, #150959, #164013, #148813, #384, #83799, #66457, #197549, #199671, #115313, #183437, #100062, #213778, #64369, #15588, #212731, #180255, #32931, #49193, #99006, #181303, #48146, #17710, #130515, #67523, #51315, #196504, #165061, #117442, #101112, #35040, #118508, #16654, #116370, #114259, #82740, #132598, #198601, #182358, #167199, #18786, #33987, #84871, #65401, #166125, #2524, #81675, #68600, #134723, #200729, #52379, #184491, #102193, #168260, #19859, #186634, #202864, #201796, #171459, #152021, #23048, #205004, #135773, #54511, #6799, #40411, #188771, #57714, #38261, #203930, #53436, #104337, #71797, #5720, #170382, #122812, #172540, #70724, #106513, #87005, #55577, #154152, #85946, #137910, #21970, #153077, #88078, #206080, #4654, #136838, #121732, #187699, #119574, #120656, #39326, #24125, #90227, #189838, #123871, #103264, #105421, #156291, #185560, #169326, #37188, #89164, #20911, #155218, #41486, #72875, #138981, #56650, #7875, #107597, #3589, #173628, #73963, #140057, #69665, #143276, #93439, #109736, #76093, #110795, #161630, #27337, #142196, #77154, #191952, #176798, #13223, #43618, #209265, #28414, #141142, #108661, #144347, #60911, #127069, #193031, #44687, #58778, #94508, #208210, #59842, #128144, #124931, #79297, #174688, #26263, #175744 ),
 ( #92382, #190893, #210347, #78225, #125994, #25199, #157361, #160546, #159478, #12152, #158416, #207154, #11076, #42558, #8953, #61988, #194105, #45753, #111872, #10018, #177877, #29488, #95581, #145414, #211415, #63044, #129212, #195188, #46822, #112937, #91303, #75030, #32675, #48942, #180005, #131311, #84620, #31627, #15340, #197302, #115060, #212476, #97702, #181058, #117186, #67275, #68348, #2272, #196253, #213531, #183187, #80364, #47898, #64120, #16403, #146461, #98754, #134480, #99813, #65153, #164811, #130263, #150710, #30563, #200484, #114010, #182106, #82481, #148570, #139, #66204, #81429, #49995, #100867, #132349, #147511, #198355, #116116, #33735, #166953, #165878, #17465, #83549, #163762, #149629, #1212, #133413, #199420, #51063, #34792, #18544, #52130, #178950, #96643, #162698, #14270, #43105, #204473, #56126, #57193, #89714, #175230, #174171, #207701, #24672, #105993, #108146, #10559, #124415, #122284, #190374, #118257, #72350, #6279, #125478, #138454, #123354, #189320, #58259, #40958, #172013, #25743, #155764, #157911, #74512, #188242, #35867, #39882, #184240, #154695, #7348, #23606, #73427, #139529, #22528, #206628, #101942, #42033, #91854, #168008, #205554, #9506, #75578, #141687, #92918, #158963, #107066, #90778, #88637, #173091, #156840, #8426, #140616, #59321, #191439, #109219, #26815, #76632, #142747, #208756, #60381, #128681, #144885, #61454, #12685, #180535, #127621, #111344, #78761, #210891, #93986, #193585, #62518, #213016, #163235, #164290, #98235, #77702, #95046, #64651, #176287, #143822, #160028, #112409, #27891, #194650, #15878, #195729, #161096, #46293, #11628, #32158, #126544, #81963, #209819, #63590, #178420, #30030, #96115, #162171, #177349, #145942, #196787, #13757, #28962, #79833, #211953, #129746, #48428, #47366, #113479, #179486, #45229, #31108, #97180, #14817, #80909, #146999, #130792, #114542, #148048, #192506, #44157, #110278, #99298, #136061, #83020, #149094, #150183, #182653, #53734, #52663, #86231, #117735, #198887, #201017, #103554, #2813, #676, #68886, #214056 ) ),
 .UNSPECIFIED., .F., .F., .F. ) 
 B_SPLINE_SURFACE_WITH_KNOTS ( ( 2, 2 ),
 ( 3, 2, 2, 2, 2, 2, 2, 2, 2, 2, 2, 2, 2, 2, 2, 2, 2, 2, 2, 2, 2, 2, 2, 2, 2, 2, 2, 2, 2, 2, 2, 2, 2, 2, 2, 2, 2, 2, 2, 2, 2, 2, 2, 2, 2, 2, 2, 2, 2, 2, 2, 2, 2, 2, 2, 2, 2, 2, 2, 2, 2, 2, 2, 2, 2, 2, 2, 2, 2, 2, 2, 2, 2, 2, 2, 2, 2, 2, 2, 2, 2, 2, 2, 2, 2, 2, 2, 2, 2, 2, 2, 2, 2, 2, 2, 2, 2, 2, 2, 2, 2, 2, 2, 2, 2, 2, 2, 2, 2, 2, 2, 2, 2, 2, 2, 2, 2, 2, 2, 2, 3 ),
 ( 0.000000000000000000, 1.000000000000000000 ),
 ( 0.000000000000000000, 0.008333333333333333218, 0.01666666666666666644, 0.02500000000000000139, 0.03333333333333333287, 0.04166666666666666435, 0.05000000000000000278, 0.05833333333333333426, 0.06666666666666666574, 0.07499999999999999722, 0.08333333333333332871, 0.09166666666666666019, 0.1000000000000000056, 0.1083333333333333370, 0.1166666666666666685, 0.1250000000000000000, 0.1333333333333333315, 0.1416666666666666630, 0.1499999999999999944, 0.1583333333333333259, 0.1666666666666666574, 0.1749999999999999889, 0.1833333333333333204, 0.1916666666666666796, 0.2000000000000000111, 0.2083333333333333426, 0.2166666666666666741, 0.2250000000000000056, 0.2333333333333333370, 0.2416666666666666685, 0.2500000000000000000, 0.2583333333333333592, 0.2666666666666666630, 0.2750000000000000222, 0.2833333333333333259, 0.2916666666666666852, 0.2999999999999999889, 0.3083333333333333481, 0.3166666666666666519, 0.3250000000000000111, 0.3333333333333333148, 0.3416666666666666741, 0.3499999999999999778, 0.3583333333333333370, 0.3666666666666666408, 0.3750000000000000000, 0.3833333333333333592, 0.3916666666666666630, 0.4000000000000000222, 0.4083333333333333259, 0.4166666666666666852, 0.4249999999999999889, 0.4333333333333333481, 0.4416666666666666519, 0.4500000000000000111, 0.4583333333333333148, 0.4666666666666666741, 0.4749999999999999778, 0.4833333333333333370, 0.4916666666666666408, 0.5000000000000000000, 0.5083333333333333037, 0.5166666666666667185, 0.5250000000000000222, 0.5333333333333333259, 0.5416666666666666297, 0.5500000000000000444, 0.5583333333333333481, 0.5666666666666666519, 0.5749999999999999556, 0.5833333333333333703, 0.5916666666666666741, 0.5999999999999999778, 0.6083333333333332815, 0.6166666666666666963, 0.6250000000000000000, 0.6333333333333333037, 0.6416666666666667185, 0.6500000000000000222, 0.6583333333333333259, 0.6666666666666666297, 0.6750000000000000444, 0.6833333333333333481, 0.6916666666666666519, 0.6999999999999999556, 0.7083333333333333703, 0.7166666666666666741, 0.7249999999999999778, 0.7333333333333332815, 0.7416666666666666963, 0.7500000000000000000, 0.7583333333333333037, 0.7666666666666667185, 0.7750000000000000222, 0.7833333333333333259, 0.7916666666666666297, 0.8000000000000000444, 0.8083333333333333481, 0.8166666666666666519, 0.8249999999999999556, 0.8333333333333333703, 0.8416666666666666741, 0.8499999999999999778, 0.8583333333333332815, 0.8666666666666666963, 0.8750000000000000000, 0.8833333333333333037, 0.8916666666666667185, 0.9000000000000000222, 0.9083333333333333259, 0.9166666666666666297, 0.9250000000000000444, 0.9333333333333333481, 0.9416666666666666519, 0.9499999999999999556, 0.9583333333333333703, 0.9666666666666666741, 0.9749999999999999778, 0.9833333333333332815, 0.9916666666666666963, 1.000000000000000000 ),
 .UNSPECIFIED. ) 
 GEOMETRIC_REPRESENTATION_ITEM ( )  RATIONAL_B_SPLINE_SURFACE ( (
 ( 1.000000000000000000, 0.8660254037844387076, 1.000000000000000000, 0.8660254037844387076, 1.000000000000000000, 0.8660254037844387076, 1.000000000000000000, 0.8660254037844387076, 1.000000000000000000, 0.8660254037844387076, 1.000000000000000000, 0.8660254037844387076, 1.000000000000000000, 0.8660254037844387076, 1.000000000000000000, 0.8660254037844387076, 1.000000000000000000, 0.8660254037844387076, 1.000000000000000000, 0.8660254037844387076, 1.000000000000000000, 0.8660254037844387076, 1.000000000000000000, 0.8660254037844387076, 1.000000000000000000, 0.8660254037844387076, 1.000000000000000000, 0.8660254037844387076, 1.000000000000000000, 0.8660254037844387076, 1.000000000000000000, 0.8660254037844387076, 1.000000000000000000, 0.8660254037844387076, 1.000000000000000000, 0.8660254037844387076, 1.000000000000000000, 0.8660254037844387076, 1.000000000000000000, 0.8660254037844387076, 1.000000000000000000, 0.8660254037844387076, 1.000000000000000000, 0.8660254037844387076, 1.000000000000000000, 0.8660254037844387076, 1.000000000000000000, 0.8660254037844387076, 1.000000000000000000, 0.8660254037844387076, 1.000000000000000000, 0.8660254037844387076, 1.000000000000000000, 0.8660254037844387076, 1.000000000000000000, 0.8660254037844387076, 1.000000000000000000, 0.8660254037844387076, 1.000000000000000000, 0.8660254037844387076, 1.000000000000000000, 0.8660254037844387076, 1.000000000000000000, 0.8660254037844387076, 1.000000000000000000, 0.8660254037844387076, 1.000000000000000000, 0.8660254037844387076, 1.000000000000000000, 0.8660254037844387076, 1.000000000000000000, 0.8660254037844387076, 1.000000000000000000, 0.8660254037844387076, 1.000000000000000000, 0.8660254037844387076, 1.000000000000000000, 0.8660254037844387076, 1.000000000000000000, 0.8660254037844387076, 1.000000000000000000, 0.8660254037844387076, 1.000000000000000000, 0.8660254037844387076, 1.000000000000000000, 0.8660254037844387076, 1.000000000000000000, 0.8660254037844387076, 1.000000000000000000, 0.8660254037844387076, 1.000000000000000000, 0.8660254037844387076, 1.000000000000000000, 0.8660254037844387076, 1.000000000000000000, 0.8660254037844387076, 1.000000000000000000, 0.8660254037844387076, 1.000000000000000000, 0.8660254037844387076, 1.000000000000000000, 0.8660254037844387076, 1.000000000000000000, 0.8660254037844387076, 1.000000000000000000, 0.8660254037844387076, 1.000000000000000000, 0.8660254037844387076, 1.000000000000000000, 0.8660254037844387076, 1.000000000000000000, 0.8660254037844387076, 1.000000000000000000, 0.8660254037844387076, 1.000000000000000000, 0.8660254037844387076, 1.000000000000000000, 0.8660254037844387076, 1.000000000000000000, 0.8660254037844387076, 1.000000000000000000, 0.8660254037844387076, 1.000000000000000000, 0.8660254037844387076, 1.000000000000000000, 0.8660254037844387076, 1.000000000000000000, 0.8660254037844387076, 1.000000000000000000, 0.8660254037844387076, 1.000000000000000000, 0.8660254037844387076, 1.000000000000000000, 0.8660254037844387076, 1.000000000000000000, 0.8660254037844387076, 1.000000000000000000, 0.8660254037844387076, 1.000000000000000000, 0.8660254037844387076, 1.000000000000000000, 0.8660254037844387076, 1.000000000000000000, 0.8660254037844387076, 1.000000000000000000, 0.8660254037844387076, 1.000000000000000000, 0.8660254037844387076, 1.000000000000000000, 0.8660254037844387076, 1.000000000000000000, 0.8660254037844387076, 1.000000000000000000, 0.8660254037844387076, 1.000000000000000000, 0.8660254037844387076, 1.000000000000000000, 0.8660254037844387076, 1.000000000000000000, 0.8660254037844387076, 1.000000000000000000, 0.8660254037844387076, 1.000000000000000000, 0.8660254037844387076, 1.000000000000000000, 0.8660254037844387076, 1.000000000000000000, 0.8660254037844387076, 1.000000000000000000, 0.8660254037844387076, 1.000000000000000000, 0.8660254037844387076, 1.000000000000000000, 0.8660254037844387076, 1.000000000000000000, 0.8660254037844387076, 1.000000000000000000, 0.8660254037844387076, 1.000000000000000000, 0.8660254037844387076, 1.000000000000000000, 0.8660254037844387076, 1.000000000000000000, 0.8660254037844387076, 1.000000000000000000, 0.8660254037844387076, 1.000000000000000000, 0.8660254037844387076, 1.000000000000000000, 0.8660254037844387076, 1.000000000000000000, 0.8660254037844387076, 1.000000000000000000, 0.8660254037844387076, 1.000000000000000000, 0.8660254037844387076, 1.000000000000000000, 0.8660254037844387076, 1.000000000000000000, 0.8660254037844387076, 1.000000000000000000, 0.8660254037844387076, 1.000000000000000000, 0.8660254037844387076, 1.000000000000000000, 0.8660254037844387076, 1.000000000000000000, 0.8660254037844387076, 1.000000000000000000, 0.8660254037844387076, 1.000000000000000000, 0.8660254037844387076, 1.000000000000000000, 0.8660254037844387076, 1.000000000000000000, 0.8660254037844387076, 1.000000000000000000, 0.8660254037844387076, 1.000000000000000000, 0.8660254037844387076, 1.000000000000000000, 0.8660254037844387076, 1.000000000000000000, 0.8660254037844387076, 1.000000000000000000, 0.8660254037844387076, 1.000000000000000000, 0.8660254037844387076, 1.000000000000000000, 0.8660254037844387076, 1.000000000000000000, 0.8660254037844387076, 1.000000000000000000, 0.8660254037844387076, 1.000000000000000000, 0.8660254037844387076, 1.000000000000000000, 0.8660254037844387076, 1.000000000000000000, 0.8660254037844387076, 1.000000000000000000),
 ( 1.000000000000000000, 0.8660254037844387076, 1.000000000000000000, 0.8660254037844387076, 1.000000000000000000, 0.8660254037844387076, 1.000000000000000000, 0.8660254037844387076, 1.000000000000000000, 0.8660254037844387076, 1.000000000000000000, 0.8660254037844387076, 1.000000000000000000, 0.8660254037844387076, 1.000000000000000000, 0.8660254037844387076, 1.000000000000000000, 0.8660254037844387076, 1.000000000000000000, 0.8660254037844387076, 1.000000000000000000, 0.8660254037844387076, 1.000000000000000000, 0.8660254037844387076, 1.000000000000000000, 0.8660254037844387076, 1.000000000000000000, 0.8660254037844387076, 1.000000000000000000, 0.8660254037844387076, 1.000000000000000000, 0.8660254037844387076, 1.000000000000000000, 0.8660254037844387076, 1.000000000000000000, 0.8660254037844387076, 1.000000000000000000, 0.8660254037844387076, 1.000000000000000000, 0.8660254037844387076, 1.000000000000000000, 0.8660254037844387076, 1.000000000000000000, 0.8660254037844387076, 1.000000000000000000, 0.8660254037844387076, 1.000000000000000000, 0.8660254037844387076, 1.000000000000000000, 0.8660254037844387076, 1.000000000000000000, 0.8660254037844387076, 1.000000000000000000, 0.8660254037844387076, 1.000000000000000000, 0.8660254037844387076, 1.000000000000000000, 0.8660254037844387076, 1.000000000000000000, 0.8660254037844387076, 1.000000000000000000, 0.8660254037844387076, 1.000000000000000000, 0.8660254037844387076, 1.000000000000000000, 0.8660254037844387076, 1.000000000000000000, 0.8660254037844387076, 1.000000000000000000, 0.8660254037844387076, 1.000000000000000000, 0.8660254037844387076, 1.000000000000000000, 0.8660254037844387076, 1.000000000000000000, 0.8660254037844387076, 1.000000000000000000, 0.8660254037844387076, 1.000000000000000000, 0.8660254037844387076, 1.000000000000000000, 0.8660254037844387076, 1.000000000000000000, 0.8660254037844387076, 1.000000000000000000, 0.8660254037844387076, 1.000000000000000000, 0.8660254037844387076, 1.000000000000000000, 0.8660254037844387076, 1.000000000000000000, 0.8660254037844387076, 1.000000000000000000, 0.8660254037844387076, 1.000000000000000000, 0.8660254037844387076, 1.000000000000000000, 0.8660254037844387076, 1.000000000000000000, 0.8660254037844387076, 1.000000000000000000, 0.8660254037844387076, 1.000000000000000000, 0.8660254037844387076, 1.000000000000000000, 0.8660254037844387076, 1.000000000000000000, 0.8660254037844387076, 1.000000000000000000, 0.8660254037844387076, 1.000000000000000000, 0.8660254037844387076, 1.000000000000000000, 0.8660254037844387076, 1.000000000000000000, 0.8660254037844387076, 1.000000000000000000, 0.8660254037844387076, 1.000000000000000000, 0.8660254037844387076, 1.000000000000000000, 0.8660254037844387076, 1.000000000000000000, 0.8660254037844387076, 1.000000000000000000, 0.8660254037844387076, 1.000000000000000000, 0.8660254037844387076, 1.000000000000000000, 0.8660254037844387076, 1.000000000000000000, 0.8660254037844387076, 1.000000000000000000, 0.8660254037844387076, 1.000000000000000000, 0.8660254037844387076, 1.000000000000000000, 0.8660254037844387076, 1.000000000000000000, 0.8660254037844387076, 1.000000000000000000, 0.8660254037844387076, 1.000000000000000000, 0.8660254037844387076, 1.000000000000000000, 0.8660254037844387076, 1.000000000000000000, 0.8660254037844387076, 1.000000000000000000, 0.8660254037844387076, 1.000000000000000000, 0.8660254037844387076, 1.000000000000000000, 0.8660254037844387076, 1.000000000000000000, 0.8660254037844387076, 1.000000000000000000, 0.8660254037844387076, 1.000000000000000000, 0.8660254037844387076, 1.000000000000000000, 0.8660254037844387076, 1.000000000000000000, 0.8660254037844387076, 1.000000000000000000, 0.8660254037844387076, 1.000000000000000000, 0.8660254037844387076, 1.000000000000000000, 0.8660254037844387076, 1.000000000000000000, 0.8660254037844387076, 1.000000000000000000, 0.8660254037844387076, 1.000000000000000000, 0.8660254037844387076, 1.000000000000000000, 0.8660254037844387076, 1.000000000000000000, 0.8660254037844387076, 1.000000000000000000, 0.8660254037844387076, 1.000000000000000000, 0.8660254037844387076, 1.000000000000000000, 0.8660254037844387076, 1.000000000000000000, 0.8660254037844387076, 1.000000000000000000, 0.8660254037844387076, 1.000000000000000000, 0.8660254037844387076, 1.000000000000000000, 0.8660254037844387076, 1.000000000000000000, 0.8660254037844387076, 1.000000000000000000, 0.8660254037844387076, 1.000000000000000000, 0.8660254037844387076, 1.000000000000000000, 0.8660254037844387076, 1.000000000000000000, 0.8660254037844387076, 1.000000000000000000, 0.8660254037844387076, 1.000000000000000000, 0.8660254037844387076, 1.000000000000000000, 0.8660254037844387076, 1.000000000000000000, 0.8660254037844387076, 1.000000000000000000, 0.8660254037844387076, 1.000000000000000000, 0.8660254037844387076, 1.000000000000000000, 0.8660254037844387076, 1.000000000000000000, 0.8660254037844387076, 1.000000000000000000, 0.8660254037844387076, 1.000000000000000000, 0.8660254037844387076, 1.000000000000000000, 0.8660254037844387076, 1.000000000000000000, 0.8660254037844387076, 1.000000000000000000, 0.8660254037844387076, 1.000000000000000000, 0.8660254037844387076, 1.000000000000000000, 0.8660254037844387076, 1.000000000000000000, 0.8660254037844387076, 1.000000000000000000, 0.8660254037844387076, 1.000000000000000000, 0.8660254037844387076, 1.000000000000000000) ) ) 
 REPRESENTATION_ITEM ( '' )  SURFACE ( )  );
#206308=CARTESIAN_POINT ( 'NONE',  ( -4.492547798081878874, 6.334668079219206049, 1.599625672291263179 ) ) ;
#206310=CARTESIAN_POINT ( 'NONE',  ( 4.489158259456265121, 7.291082831790689056, -1.082531754730548412 ) ) ;
#206316=CARTESIAN_POINT ( 'NONE',  ( -3.654804927335652209, 6.421633627603656080, 1.199719254218452935 ) ) ;
#206320=CARTESIAN_POINT ( 'NONE',  ( -5.939880696562884310, 9.943961556049767836, 0.7216878364870267237 ) ) ;
#206323=CARTESIAN_POINT ( 'NONE',  ( -7.533490631048818109, 8.818102486758951031, -1.199719254218452047 ) ) ;
#206327=CARTESIAN_POINT ( 'NONE',  ( -4.447956913735107598, 7.346977611736363656, 1.199719254218452935 ) ) ;
#206339=CARTESIAN_POINT ( 'NONE',  ( -4.150204419558982671, 7.856005899545188242, 0.7216878364870338292 ) ) ;
#206341=CARTESIAN_POINT ( 'NONE',  ( -6.929625909916163451, 7.257187447756535903, 0.7216878364870317197 ) ) ;
#206342=CARTESIAN_POINT ( 'NONE',  ( 6.333594036239346359, 7.418223126147930557, 1.199719254218453823 ) ) ;
#206343=CARTESIAN_POINT ( 'NONE',  ( -7.130662446144611977, 7.283804040115648526, 0.000000000000000000 ) ) ;
#206364=CARTESIAN_POINT ( 'NONE',  ( 7.388267364804250725, 7.584343111885245570, -0.7998128361456341429 ) ) ;
#206365=ORIENTED_EDGE ( 'NONE', *, *, #41220, .T. ) ;
#206392=CARTESIAN_POINT ( 'NONE',  ( -1.887367962963634627, 8.990012987145949097, -0.7749999999999996891 ) ) ;
#206397=CIRCLE ( 'NONE', #189244, 0.08000000000000025147 ) ;
#206401=CARTESIAN_POINT ( 'NONE',  ( 4.766573523656222555, 7.718696989977711809, 1.199719254218452047 ) ) ;
#206407=CARTESIAN_POINT ( 'NONE',  ( -5.682275777458886346, 7.722684055159061423, 1.443375672974058777 ) ) ;
#206419=CARTESIAN_POINT ( 'NONE',  ( 3.088225128862704949, 6.824956093640315302, 0.7998128361456281477 ) ) ;
#206420=CARTESIAN_POINT ( 'NONE',  ( 4.908934136599710563, 7.884784371745123366, 1.199719254218451159 ) ) ;
#206426=VERTEX_POINT ( 'NONE', #71973 ) ;
#206432=CARTESIAN_POINT ( 'NONE',  ( 4.224247379109608680, 7.085983154673295203, -1.199719254218452047 ) ) ;
#206442=CARTESIAN_POINT ( 'NONE',  ( 6.699137298928145690, 8.909022496873262753, 1.443375672974065660 ) ) ;
#206443=CARTESIAN_POINT ( 'NONE',  ( -3.363831509966363598, 5.978201624052440266, -1.082531754730548412 ) ) ;
#206444=CARTESIAN_POINT ( 'NONE',  ( -7.273023059088104425, 7.449891421883056530, 0.000000000000000000 ) ) ;
#206450=VERTEX_POINT ( 'NONE', #67696 ) ;
#206455=CARTESIAN_POINT ( 'NONE',  ( 7.517069824134078537, 7.734612647770044092, 0.000000000000000000 ) ) ;
#206457=CARTESIAN_POINT ( 'NONE',  ( 6.039231080244466199, 6.010467446565510130, 0.7998128361456352531 ) ) ;
#206458=CARTESIAN_POINT ( 'NONE',  ( 5.664274315459256748, 9.830346811336296398, -0.7998128361456481317 ) ) ;
#206461=CARTESIAN_POINT ( 'NONE',  ( 6.393551957296131683, 9.616838495890963401, 1.199719254218452047 ) ) ;
#206480=CARTESIAN_POINT ( 'NONE',  ( 5.357406976055401948, 6.279338222599979424, 1.199719254218452935 ) ) ;
#206482=CARTESIAN_POINT ( 'NONE',  ( -5.029148636026397945, 4.832037928311032182, 0.7998128361456281477 ) ) ;
#206484=CARTESIAN_POINT ( 'NONE',  ( 6.086684617892325733, 6.065829907154645539, -0.7998128361456481317 ) ) ;
#206488=CARTESIAN_POINT ( 'NONE',  ( 4.549612403093820312, 8.500000000000243361, -0.2314049244472246580 ) ) ;
#206489=CARTESIAN_POINT ( 'NONE',  ( 3.464990776744291345, 6.200183785247111778, 1.199719254218452047 ) ) ;
#206490=DIRECTION ( 'NONE',  ( -0.3281536732072464768, -0.000000000000000000, 0.9446243521954066358 ) ) ;
#206493=CARTESIAN_POINT ( 'NONE',  ( 6.211043768836185031, 6.418841616496599123, 0.7216878364870328300 ) ) ;
#206495=CARTESIAN_POINT ( 'NONE',  ( -4.457598643843001973, 8.422558527783969851, 0.000000000000000000 ) ) ;
#206496=CARTESIAN_POINT ( 'NONE',  ( 3.366167277942881064, 7.149221934233827014, -0.7998128361456362523 ) ) ;
#206497=ORIENTED_EDGE ( 'NONE', *, *, #31198, .F. ) ;
#206503=CARTESIAN_POINT ( 'NONE',  ( -5.947207536862552324, 6.164775583291447703, -0.3409585216945008046 ) ) ;
#206506=CARTESIAN_POINT ( 'NONE',  ( -5.320648938720212051, 5.172121614787156929, 0.000000000000000000 ) ) ;
#206537=CARTESIAN_POINT ( 'NONE',  ( 2.957086901556340575, 6.464035461875470290, 0.7216878364870257245 ) ) ;
#206542=CARTESIAN_POINT ( 'NONE',  ( 7.828907357248368726, 8.098423103070084395, 0.7998128361456281477 ) ) ;
#206543=CARTESIAN_POINT ( 'NONE',  ( 4.055297343818933697, 5.824542549245813383, 1.443375672974058777 ) ) ;
#206558=CARTESIAN_POINT ( 'NONE',  ( -5.448397627845328550, 7.449826213943242514, 1.599625672291263179 ) ) ;
#206560=CARTESIAN_POINT ( 'NONE',  ( 6.739811759324814133, 8.956476034002680109, -1.443375672974078761 ) ) ;
#206571=CARTESIAN_POINT ( 'NONE',  ( -5.984998465789844069, 5.947196063035064206, 0.7998128361456281477 ) ) ;
#206579=CARTESIAN_POINT ( 'NONE',  ( -2.823841133396259639, 6.516508098929413961, -0.7998128361456481317 ) ) ;
#206595=CARTESIAN_POINT ( 'NONE',  ( -10.17567228521069467, -0.02076350362892331880, -2.500000000000000444 ) ) ;
#206601=ORIENTED_EDGE ( 'NONE', *, *, #72507, .T. ) ;
#206602=CARTESIAN_POINT ( 'NONE',  ( -5.336015975430226099, 8.383046517047350932, -1.199719254218453823 ) ) ;
#206604=CARTESIAN_POINT ( 'NONE',  ( -4.329849954717889915, 6.144853928627882489, 1.599625672291270506 ) ) ;
#206605=VERTEX_POINT ( 'NONE', #55748 ) ;
#206628=CARTESIAN_POINT ( 'NONE',  ( -5.712781623311813384, 7.758274208654143855, -1.599625672291271394 ) ) ;
#206636=CARTESIAN_POINT ( 'NONE',  ( 6.170369307550806148, 10.21286493553572328, 0.7216878364870317197 ) ) ;
#206637=DIRECTION ( 'NONE',  ( 1.000000000000000000, 0.000000000000000000, 0.000000000000000000 ) ) ;
#206646=CARTESIAN_POINT ( 'NONE',  ( 4.224247379109608680, 7.085983154673295203, -1.199719254218452047 ) ) ;
#206654=CARTESIAN_POINT ( 'NONE',  ( 7.201315867513990554, 8.430565262634994284, -1.199719254218452047 ) ) ;
#206656=CARTESIAN_POINT ( 'NONE',  ( 6.717138760927786834, 6.801359740696030443, -0.7998128361456481317 ) ) ;
#206665=CARTESIAN_POINT ( 'NONE',  ( 6.076298462418691315, 7.128931413452940014, -1.143247356662546732 ) ) ;
#206670=CARTESIAN_POINT ( 'NONE',  ( 6.438112759045284683, 6.782534085545247393, 0.3978009605737874432 ) ) ;
#206672=CARTESIAN_POINT ( 'NONE',  ( 5.560252395380206991, 7.580323442733986283, 1.443375672974065660 ) ) ;
#206674=TOROIDAL_SURFACE ( 'NONE', #75268, 0.8300000000000010703, 0.08000000000000000167 ) ;
#206680=CARTESIAN_POINT ( 'NONE',  ( -4.146814880933400005, 5.931313009212638931, 1.599625672291270506 ) ) ;
#206692=CARTESIAN_POINT ( 'NONE',  ( -5.085717018457573957, 8.947437264926888290, 0.7216878364870267237 ) ) ;
#206696=CARTESIAN_POINT ( 'NONE',  ( 7.991605200612358573, 8.288237253661408843, 0.7998128361456281477 ) ) ;
#206697=CARTESIAN_POINT ( 'NONE',  ( -4.953691873189081107, 6.621539441584240571, -1.250027308714734664 ) ) ;
#206712=CARTESIAN_POINT ( 'NONE',  ( 6.210516883511641772, 9.403297576475722508, 1.199719254218452047 ) ) ;
#206731=CARTESIAN_POINT ( 'NONE',  ( -7.449279056065764237, 7.655523418356991350, 0.7998128361456341429 ) ) ;
#206752=CARTESIAN_POINT ( 'NONE',  ( 5.397554552016216256, 7.390509292142662723, 1.443375672974065660 ) ) ;
#206758=CARTESIAN_POINT ( 'NONE',  ( 6.933015448541703485, 9.181880338089085214, 1.599625672291268286 ) ) ;
#206761=CARTESIAN_POINT ( 'NONE',  ( -3.689227196694346400, 6.357829925235092716, -1.082531754730546636 ) ) ;
#206770=CARTESIAN_POINT ( 'NONE',  ( -6.427974226210522168, 6.671927150099951298, 0.000000000000000000 ) ) ;
#206794=CARTESIAN_POINT ( 'NONE',  ( 5.578253857379852576, 5.472660686556754861, -0.7998128361456481317 ) ) ;
#206804=CARTESIAN_POINT ( 'NONE',  ( -6.834718835064852449, 8.106831741398025315, 1.082531754730549078 ) ) ;
#206806=CARTESIAN_POINT ( 'NONE',  ( 3.079110283634975964, 6.606396074300548982, 0.7216878364870257245 ) ) ;
#206816=AXIS2_PLACEMENT_3D ( 'NONE', #12775, #144968, #59416 ) ;
#206824=CARTESIAN_POINT ( 'NONE',  ( -4.665414256878304577, 5.575976400180357118, -1.082531754730549967 ) ) ;
#206856=CARTESIAN_POINT ( 'NONE',  ( -7.228432174741334038, 8.462200954400218578, -1.199719254218452047 ) ) ;
#206859=CARTESIAN_POINT ( 'NONE',  ( -6.798487682609798632, 6.896266815991691779, 0.7998128361456341429 ) ) ;
#206864=CARTESIAN_POINT ( 'NONE',  ( -5.763624699140874164, 8.777960344756069233, -1.082531754730549967 ) ) ;
#206866=CARTESIAN_POINT ( 'NONE',  ( 5.980555156959511898, 9.991415093179179863, -0.7216878364870458196 ) ) ;
#206868=CARTESIAN_POINT ( 'NONE',  ( -3.923105346307911745, 5.670318552149568703, -1.599625672291283607 ) ) ;
#206872=CARTESIAN_POINT ( 'NONE',  ( -3.654804927335652209, 6.421633627603656080, 1.199719254218452935 ) ) ;
#206879=CARTESIAN_POINT ( 'NONE',  ( -5.582925393777276035, 9.735439736040634173, 0.7998128361456291469 ) ) ;
#206881=CARTESIAN_POINT ( 'NONE',  ( 4.937886321289528979, 7.980522944944189234, -1.013380012275147291 ) ) ;
#206885=CARTESIAN_POINT ( 'NONE',  ( 3.627688620108284745, 6.389997935838436227, 1.199719254218452047 ) ) ;
#206898=CARTESIAN_POINT ( 'NONE',  ( -3.797692425159308716, 7.444741906078900406, 0.000000000000000000 ) ) ;
#206907=CARTESIAN_POINT ( 'NONE',  ( 6.994027139803230320, 9.253060644560830994, -1.599625672291267398 ) ) ;
#206914=DIRECTION ( 'NONE',  ( 0.7592566023653005702, 0.6507913734559639396, 0.000000000000000000 ) ) ;
#206918=DIRECTION ( 'NONE',  ( -1.000000000000000000, 0.000000000000000000, 0.000000000000000000 ) ) ;
#206921=CARTESIAN_POINT ( 'NONE',  ( -3.059665831784952651E-14, 3.479999999999999538, 2.000000000000000000 ) ) ;
#206925=CARTESIAN_POINT ( 'NONE',  ( 6.604365638557201379, 6.767254738080503706, -0.09251035838216993545 ) ) ;
#206926=CARTESIAN_POINT ( 'NONE',  ( -4.245111494410291897, 7.006361605903701495, 1.082531754730549967 ) ) ;
#206955=CARTESIAN_POINT ( 'NONE',  ( 3.715816618597135523, 6.492813934075403637, -1.199719254218453823 ) ) ;
#206973=CARTESIAN_POINT ( 'NONE',  ( -5.824109505522200081, 8.952488968821326054, -1.199719254218452047 ) ) ;
#206976=DIRECTION ( 'NONE',  ( 0.000000000000000000, -1.000000000000000000, 0.000000000000000000 ) ) ;
#206980=CARTESIAN_POINT ( 'NONE',  ( 5.721791708487565131, 5.640121512849101570, 0.3304596318965865587 ) ) ;
#206988=CARTESIAN_POINT ( 'NONE',  ( 5.520104819419390907, 6.469152373191302985, 1.199719254218452935 ) ) ;
#206998=CARTESIAN_POINT ( 'NONE',  ( 4.742863741006460465, 8.194075573275554802, 0.7225937585536055252 ) ) ;
#207000=CARTESIAN_POINT ( 'NONE',  ( 5.355423173304108886, 7.585870477640591858, 1.239999553246450725 ) ) ;
#207007=CARTESIAN_POINT ( 'NONE',  ( -3.888022742048568681, 7.337601240860233354, -0.7289588026271909271 ) ) ;
#207020=CARTESIAN_POINT ( 'NONE',  ( -3.332271893908731464, 7.109677319527304640, -0.7998128361456481317 ) ) ;
#207022=CARTESIAN_POINT ( 'NONE',  ( 3.901714345682657292, 7.774026846596938434, 0.7998128361456271485 ) ) ;
#207025=CARTESIAN_POINT ( 'NONE',  ( -7.123883369337781879, 7.275895117174344229, 0.7998128361456341429 ) ) ;
#207034=CARTESIAN_POINT ( 'NONE',  ( -5.249610431062532889, 7.793670086080374482, -1.296690129572550365 ) ) ;
#207044=CARTESIAN_POINT ( 'NONE',  ( -4.733205024502264102, 7.575804057677677505, 1.082531754730549967 ) ) ;
#207051=CARTESIAN_POINT ( 'NONE',  ( 4.990809943606266508, 6.915973915664348937, -1.443375672974068769 ) ) ;
#207052=DIRECTION ( 'NONE',  ( 0.7592566023652990159, -0.6507913734559659380, 0.000000000000000000 ) ) ;
#207055=CARTESIAN_POINT ( 'NONE',  ( -7.262327558775498737, 8.501745569106741840, 1.199719254218452047 ) ) ;
#207070=CARTESIAN_POINT ( 'NONE',  ( 4.655245641445829641, 6.524482229810530498, 1.599625672291269396 ) ) ;
#207073=CARTESIAN_POINT ( 'NONE',  ( 5.900277318768097246, 7.249539301847896411, -1.301905728482563251 ) ) ;
#207099=CARTESIAN_POINT ( 'NONE',  ( -4.963693636378939011, 8.805076652501815815, 0.7216878364870267237 ) ) ;
#207114=VERTEX_POINT ( 'NONE', #192136 ) ;
#207126=CARTESIAN_POINT ( 'NONE',  ( -8.093291352714894415, 8.406871097780989288, -0.7998128361456362523 ) ) ;
#207132=CARTESIAN_POINT ( 'NONE',  ( -5.646044625448194410, 5.551749915969804938, 0.000000000000000000 ) ) ;
#207141=CARTESIAN_POINT ( 'NONE',  ( -6.064239847062411926, 10.29697326487330500, 0.000000000000000000 ) ) ;
#207144=CARTESIAN_POINT ( 'NONE',  ( 6.098455030413784783, 7.112933956528650015, -1.126327413477963502 ) ) ;
#207148=CARTESIAN_POINT ( 'NONE',  ( 5.391302360089590628, 6.318882837306503575, -1.199719254218452047 ) ) ;
#207154=CARTESIAN_POINT ( 'NONE',  ( -2.979759899953417612, 6.698413326579433225, 0.7998128361456352531 ) ) ;
#207156=ORIENTED_EDGE ( 'NONE', *, *, #190135, .F. ) ;
#207158=CARTESIAN_POINT ( 'NONE',  ( -4.773352600463090845, 7.726605912919016106, 1.199719254218452935 ) ) ;
#207163=CARTESIAN_POINT ( 'NONE',  ( 4.651856102820254968, 7.480896982382013505, -1.082531754730548412 ) ) ;
#207164=CARTESIAN_POINT ( 'NONE',  ( -5.167065940139584868, 6.161236697318522637, 1.082531754730549078 ) ) ;
#207170=CARTESIAN_POINT ( 'NONE',  ( 4.065465959251388206, 5.836405933916976707, -1.599625672291269396 ) ) ;
#207178=EDGE_CURVE ( 'NONE', #53708, #203895, #86849, .T. ) ;
#207181=CARTESIAN_POINT ( 'NONE',  ( 5.652821694808577213, 7.451312062667313718, 1.328372732707931103 ) ) ;
#207190=CARTESIAN_POINT ( 'NONE',  ( 5.189738938980948291, 9.276722205444929870, 0.000000000000000000 ) ) ;
#207201=CARTESIAN_POINT ( 'NONE',  ( 4.661274270878652537, 8.290979908523663511, 0.5017903844357074483 ) ) ;
#207209=CARTESIAN_POINT ( 'NONE',  ( 7.693325821111733021, 7.940244644243982464, -0.7998128361456341429 ) ) ;
#207213=CARTESIAN_POINT ( 'NONE',  ( -5.076314662610137418, 7.858265529090583179, 1.124058833742283436 ) ) ;
#207220=CARTESIAN_POINT ( 'NONE',  ( -7.279802135894939852, 7.457800344824362604, -0.7998128361456362523 ) ) ;
#207233=CARTESIAN_POINT ( 'NONE',  ( 7.212011367826596242, 7.378711115411311638, 0.000000000000000000 ) ) ;
#207241=CARTESIAN_POINT ( 'NONE',  ( 5.401997860402196316, 5.267028690082820930, 0.000000000000000000 ) ) ;
#207243=CARTESIAN_POINT ( 'NONE',  ( 4.353576723319599218, 8.093273587265928271, -0.7216878364870357165 ) ) ;
#207258=CARTESIAN_POINT ( 'NONE',  ( -5.822300622425855110, 5.757381912443740646, 0.7998128361456281477 ) ) ;
#207259=CARTESIAN_POINT ( 'NONE',  ( 5.090160327287878594, 4.903218234782778850, -0.7998128361456481317 ) ) ;
#207271=CARTESIAN_POINT ( 'NONE',  ( -6.231907884136888676, 7.299589282028351001, -1.199719254218453823 ) ) ;
#207272=CARTESIAN_POINT ( 'NONE',  ( -5.093022980588950865, 5.970890227889075419, -1.199719254218453823 ) ) ;
#207274=CARTESIAN_POINT ( 'NONE',  ( 5.519577934094840543, 9.453608333170423705, 0.7216878364870317197 ) ) ;
#207287=CARTESIAN_POINT ( 'NONE',  ( -6.033312665451926904, 7.071988487544162538, -1.043104321438679039 ) ) ;
#207293=CARTESIAN_POINT ( 'NONE',  ( 4.909461021924254709, 5.860697626067345567, 1.082531754730549078 ) ) ;
#207297=CARTESIAN_POINT ( 'NONE',  ( -7.469616286486262524, 7.679250187180907794, 0.7998128361456341429 ) ) ;
#207313=CARTESIAN_POINT ( 'NONE',  ( 6.017840079619279692, 8.114175741012878973, -1.599625672291281386 ) ) ;
#207331=( BOUNDED_SURFACE ( )  B_SPLINE_SURFACE ( 3, 2, ( 
 ( #89970, #187441, #72618 ),
 ( #138717, #23863, #156022 ),
 ( #70465, #39068, #57452 ),
 ( #41223, #123612, #189575 ),
 ( #107328, #152818, #4394 ),
 ( #168685, #200100, #66877 ) ),
 .UNSPECIFIED., .F., .F., .F. ) 
 B_SPLINE_SURFACE_WITH_KNOTS ( ( 4, 2, 4 ),
 ( 3, 3 ),
 ( 6.938893903907228378E-18, 0.002403677751102688189, 0.004807355502205369439 ),
 ( 0.000000000000000000, 1.000000000000000000 ),
 .UNSPECIFIED. ) 
 GEOMETRIC_REPRESENTATION_ITEM ( )  RATIONAL_B_SPLINE_SURFACE ( (
 ( 1.000000000000000000, 0.7789607113619931855, 1.000000000000000000),
 ( 1.000000000000000000, 0.7844575505960370565, 1.000000000000000000),
 ( 1.000000000000000000, 0.7910273759749103517, 1.000000000000000000),
 ( 1.000000000000000000, 0.8087931444451713636, 1.000000000000000000),
 ( 1.000000000000000000, 0.8199986536747382315, 1.000000000000000000),
 ( 1.000000000000000000, 0.8356624583022107533, 1.000000000000000000) ) ) 
 REPRESENTATION_ITEM ( '' )  SURFACE ( )  );
#207342=EDGE_LOOP ( 'NONE', ( #201364, #36456 ) ) ;
#207352=CARTESIAN_POINT ( 'NONE',  ( 6.211043768836173484, 8.339580045099285854, 1.443375672974065660 ) ) ;
#207356=CARTESIAN_POINT ( 'NONE',  ( 7.200788982189461507, 8.533913579710086239, -1.082531754730548412 ) ) ;
#207380=CARTESIAN_POINT ( 'NONE',  ( -4.655245641445871385, 6.524482229810530498, 1.599625672291263179 ) ) ;
#207382=CARTESIAN_POINT ( 'NONE',  ( 6.170369307550831017, 6.371388078330353366, 0.7216878364870328300 ) ) ;
#207387=CARTESIAN_POINT ( 'NONE',  ( -5.387385936583832802, 7.378645907471495846, -1.599625672291271394 ) ) ;
#207392=CARTESIAN_POINT ( 'NONE',  ( -5.171509248969888617, 4.998125310078441075, 0.7998128361456281477 ) ) ;
#207400=CARTESIAN_POINT ( 'NONE',  ( -5.822300622425855110, 5.757381912443740646, 0.7998128361456281477 ) ) ;
#207408=CARTESIAN_POINT ( 'NONE',  ( -5.957882158562513908, 5.915560371269843465, -0.7998128361456362523 ) ) ;
#207411=CARTESIAN_POINT ( 'NONE',  ( -4.773879485787619892, 7.623257595843924150, 1.082531754730549967 ) ) ;
#207412=CARTESIAN_POINT ( 'NONE',  ( -5.682275777458886346, 7.722684055159061423, 1.443375672974058777 ) ) ;
#207413=CARTESIAN_POINT ( 'NONE',  ( 5.417364897112183719, 8.477953592343014932, 1.199719254218451159 ) ) ;
#207414=CARTESIAN_POINT ( 'NONE',  ( -5.498713818794216834, 8.572860667638675380, -1.199719254218452047 ) ) ;
#207422=ORIENTED_EDGE ( 'NONE', *, *, #41266, .T. ) ;
#207433=CARTESIAN_POINT ( 'NONE',  ( 6.984385409695311964, 8.177479728513226576, 1.199719254218452935 ) ) ;
#207454=CARTESIAN_POINT ( 'NONE',  ( 5.258270873920524835, 7.671714958958308017, -1.216365610458163715 ) ) ;
#207470=CARTESIAN_POINT ( 'NONE',  ( 5.203297092594585393, 9.292540051327542017, 0.7998128361456341429 ) ) ;
#207473=CARTESIAN_POINT ( 'NONE',  ( -4.516801452008150086, 5.298631777878131111, 1.199719254218452935 ) ) ;
#207476=CARTESIAN_POINT ( 'NONE',  ( -6.360183458142173230, 9.473945563590925545, 1.082531754730549967 ) ) ;
#207487=CARTESIAN_POINT ( 'NONE',  ( 4.934241560730721510, 4.721313007132757811, 0.000000000000000000 ) ) ;
#207488=CARTESIAN_POINT ( 'NONE',  ( 5.285699784481295183, 7.260012063351913625, 1.599625672291268286 ) ) ;
#207500=CARTESIAN_POINT ( 'NONE',  ( 3.901714345682657292, 7.774026846596938434, 0.7998128361456271485 ) ) ;
#207503=VECTOR ( 'NONE', #4788, 1000.000000000000000 ) ;
#207514=CARTESIAN_POINT ( 'NONE',  ( 5.533136088152891929, 9.469426179571447832, -0.7216878364870458196 ) ) ;
#207515=CARTESIAN_POINT ( 'NONE',  ( -4.123088112331656951, 6.864000993478624579, 1.082531754730549967 ) ) ;
#207516=CARTESIAN_POINT ( 'NONE',  ( -6.774234028683526532, 7.932303117332766718, 1.199719254218452047 ) ) ;
#207528=CARTESIAN_POINT ( 'NONE',  ( 6.052789233858158369, 6.026285292448116948, 0.000000000000000000 ) ) ;
#207529=CARTESIAN_POINT ( 'NONE',  ( 6.444921918449731280, 8.612437886315108315, 1.599625672291268286 ) ) ;
#207532=CARTESIAN_POINT ( 'NONE',  ( 4.462041952228939401, 6.299077925724123617, -1.443375672974068769 ) ) ;
#207538=CARTESIAN_POINT ( 'NONE',  ( 4.318600669050584706, 4.999583595936801572, 2.420000000000000373 ) ) ;
#207548=CARTESIAN_POINT ( 'NONE',  ( 3.953084306836263995, 6.769626237021087789, 1.199719254218452047 ) ) ;
#207551=CARTESIAN_POINT ( 'NONE',  ( 5.923986774528332333, 5.876015756563318426, -0.7998128361456481317 ) ) ;
#207556=CARTESIAN_POINT ( 'NONE',  ( 6.318982112420993502, 9.529840343536603697, -1.199719254218452047 ) ) ;
#207561=CARTESIAN_POINT ( 'NONE',  ( 4.895902868310594513, 8.725987423088758632, 0.000000000000000000 ) ) ;
#207564=CARTESIAN_POINT ( 'NONE',  ( -5.631432701629818460, 7.663367133358481631, 1.599625672291263179 ) ) ;
#207565=CARTESIAN_POINT ( 'NONE',  ( 4.041212305325117882, 6.872442235258051646, -1.199719254218448494 ) ) ;
#207576=CARTESIAN_POINT ( 'NONE',  ( -5.472651281771599763, 6.413789912602166687, 1.199719254218452935 ) ) ;
#207587=EDGE_CURVE ( 'NONE', #41289, #207114, #48521, .T. ) ;
#207594=VERTEX_POINT ( 'NONE', #45321 ) ;
#207608=CARTESIAN_POINT ( 'NONE',  ( 5.833751235630055376, 10.02806988486892514, 0.7998128361456331437 ) ) ;
#207609=CARTESIAN_POINT ( 'NONE',  ( 8.174640274396848483, 8.501778173076651512, 0.7998128361456291469 ) ) ;
#207622=CARTESIAN_POINT ( 'NONE',  ( -3.955946960137363799, 7.837298230127379917, 0.7998128361456352531 ) ) ;
#207624=CARTESIAN_POINT ( 'NONE',  ( -4.938913097128142304, 8.984092056616635347, -0.7998128361456362523 ) ) ;
#207626=CARTESIAN_POINT ( 'NONE',  ( 5.980555156959511898, 9.991415093179179863, -0.7216878364870458196 ) ) ;
#207635=CARTESIAN_POINT ( 'NONE',  ( -6.134138155540168391, 6.121192367743780949, 0.000000000000000000 ) ) ;
#207642=CARTESIAN_POINT ( 'NONE',  ( -5.655159470675923394, 5.770309935309573923, 0.000000000000000000 ) ) ;
#207646=CARTESIAN_POINT ( 'NONE',  ( -4.274563570058511175, 8.209017608368725405, 0.000000000000000000 ) ) ;
#207657=AXIS2_PLACEMENT_3D ( 'NONE', #97034, #60231, #142591 ) ;
#207664=DIRECTION ( 'NONE',  ( -1.000000000000000000, 0.000000000000000000, -2.168404344971003504E-14 ) ) ;
#207671=CARTESIAN_POINT ( 'NONE',  ( -6.469175572376043348, 7.576401584974034265, 1.199719254218452047 ) ) ;
#207673=CARTESIAN_POINT ( 'NONE',  ( -3.969505113751027547, 7.853116076009993840, 1.214306433183764966E-14 ) ) ;
#207674=ORIENTED_EDGE ( 'NONE', *, *, #75725, .F. ) ;
#207685=VERTEX_POINT ( 'NONE', #202996 ) ;
#207688=ADVANCED_FACE ( 'NONE', ( #120783 ), #186761, .F. ) ;
#207699=CARTESIAN_POINT ( 'NONE',  ( -4.970620135051034616, 8.062850052469723749, -1.111334424012894617 ) ) ;
#207701=CARTESIAN_POINT ( 'NONE',  ( -6.330731382938325602, 6.350551133041632212, 0.7998128361456281477 ) ) ;
#207726=CARTESIAN_POINT ( 'NONE',  ( 6.540882763950133238, 6.595727744222092959, 0.000000000000000000 ) ) ;
#207738=CARTESIAN_POINT ( 'NONE',  ( 5.638349000628050334, 7.351887578364292075, 1.232751772250343381 ) ) ;
#207740=CARTESIAN_POINT ( 'NONE',  ( 5.722950238744187956, 9.690876021928001904, 0.7216878364870317197 ) ) ;
#207746=CARTESIAN_POINT ( 'NONE',  ( -5.743814354044916470, 6.730146830254374990, -1.199719254218453823 ) ) ;
#207750=EDGE_CURVE ( 'NONE', #78850, #56668, #155313, .T. ) ;
#207755=CARTESIAN_POINT ( 'NONE',  ( -6.089020385868862739, 8.197219431637373432, -1.443375672974066548 ) ) ;
#207758=CARTESIAN_POINT ( 'NONE',  ( 8.167861197590044142, 8.493869250135347215, 0.000000000000000000 ) ) ;
#207771=CARTESIAN_POINT ( 'NONE',  ( 3.566232916275655640, 7.382631845622076305, 0.2048419657294417440 ) ) ;
#207773=CARTESIAN_POINT ( 'NONE',  ( 5.096939404094710468, 4.911127157724081371, 0.000000000000000000 ) ) ;
#207791=CARTESIAN_POINT ( 'NONE',  ( -5.478376588373717659, 8.549133898814758936, -1.199719254218452047 ) ) ;
#207793=CARTESIAN_POINT ( 'NONE',  ( 7.367930134383754215, 7.560616343061329125, -0.7998128361456341429 ) ) ;
#207813=CARTESIAN_POINT ( 'NONE',  ( 5.017926250833595780, 7.907978821730911712, -1.082531754730548412 ) ) ;
#207820=CARTESIAN_POINT ( 'NONE',  ( 7.526711554241970248, 8.810193563817646734, -1.199719254218452047 ) ) ;
#207824=CARTESIAN_POINT ( 'NONE',  ( -4.665414256878287702, 8.457084043084382330, -0.7216878364870338292 ) ) ;
#207835=FACE_OUTER_BOUND ( 'NONE', #209688, .T. ) ;
#207857=CARTESIAN_POINT ( 'NONE',  ( 5.391302360089590628, 6.318882837306503575, -1.199719254218452047 ) ) ;
#207869=CARTESIAN_POINT ( 'NONE',  ( -5.966997003790221576, 9.015228033513643879, -1.082531754730549967 ) ) ;
#207873=CARTESIAN_POINT ( 'NONE',  ( 3.214691819771663628, 6.764574533126651801, -0.7216878364870338292 ) ) ;
#207880=CARTESIAN_POINT ( 'NONE',  ( 0.000000000000000000, 6.062865449010541141, 0.000000000000000000 ) ) ;
#207889=CARTESIAN_POINT ( 'NONE',  ( -3.187575512988701565, 6.732938841879847480, 0.000000000000000000 ) ) ;
#207916=PRODUCT ( 'negative coil', 'negative coil', '', ( #105645 ) ) ;
#207922=CARTESIAN_POINT ( 'NONE',  ( -5.772739544368596043, 9.956889578397179363, -0.7998128361456362523 ) ) ;
#207925=CARTESIAN_POINT ( 'NONE',  ( -6.934069218746458318, 7.054445274817795486, -0.7998128361456362523 ) ) ;
#207926=CARTESIAN_POINT ( 'NONE',  ( -5.599738924909661186, 5.745725798494749625, 0.2540040342395213369 ) ) ;
#207930=CARTESIAN_POINT ( 'NONE',  ( -5.899206235277530297, 9.896508017883515862, 0.7216878364870267237 ) ) ;
#207936=ORIENTED_EDGE ( 'NONE', *, *, #108550, .F. ) ;
#207937=CARTESIAN_POINT ( 'NONE',  ( -5.679940009482361774, 5.591294530676332641, 0.7998128361456281477 ) ) ;
#207948=CARTESIAN_POINT ( 'NONE',  ( 5.819104682239041537, 7.212836251160942957, -1.171789181936284896 ) ) ;
#207952=CARTESIAN_POINT ( 'NONE',  ( 4.037295881819344956, 7.932205305423046582, -0.7998128361456362523 ) ) ;
#207972=CARTESIAN_POINT ( 'NONE',  ( 3.854260808034858155, 7.718664386007802136, -0.7998128361456362523 ) ) ;
#207973=CARTESIAN_POINT ( 'NONE',  ( 6.749980374757213575, 8.968339418673846097, 1.599625672291268286 ) ) ;
#207982=DIRECTION ( 'NONE',  ( -0.6507913734559641616, -0.7592566023653004592, 0.000000000000000000 ) ) ;
#207988=CARTESIAN_POINT ( 'NONE',  ( 6.296370465541430761, 6.973533528358998979, 0.9269300130883666444 ) ) ;
#207989=CARTESIAN_POINT ( 'NONE',  ( -5.763624699140894592, 5.896852701852039580, -0.7216878364870338292 ) ) ;
#207990=CARTESIAN_POINT ( 'NONE',  ( 2.929970594329034395, 6.432399770110250437, -0.7216878364870338292 ) ) ;
#207991=( BOUNDED_SURFACE ( )  B_SPLINE_SURFACE ( 1, 2, ( 
 ( #30316, #96401, #12972, #128956, #76909, #147266, #145164, #213298, #144108, #130024, #143035, #63869, #209030, #127909, #177639, #161389, #64925, #162451, #131074, #113762, #112691, #176563, #28172, #197062, #11912, #14027, #212236, #193861, #126828, #31382, #196015, #15099, #60665, #79048, #47651, #210102, #77985, #94268, #179766, #192785, #111626, #29247, #48700, #97458, #62794, #93203, #194935, #163513, #81188, #114814, #149385, #16154, #199169, #198119, #182941, #67032, #132111, #136349, #148330, #85444, #49750, #35619, #99571, #967, #50815, #17223, #115877, #65962, #3098, #151529, #133169, #32439, #164569, #200242, #19364, #69168, #54019, #116941, #181862, #86514, #2029, #202370, #83300, #52942, #68098, #34557, #84381, #100628, #201302, #134233, #36685, #185060, #98507, #120158, #119079, #102772, #33498, #166704, #82239, #70236, #51892, #18295, #150468, #135288, #118015, #184004, #165635, #101697, #214330, #167767, #168827, #20431, #152579, #4166, #170961, #22561, #141716, #88666, #9532, #104920, #207726, #8455, #75605, #91884, #154726, #59349, #72383, #108173, #87588, #103841, #190402, #71303, #122316, #206656, #186134, #173122, #174199, #6309, #138482, #37769, #189348, #187208, #40988, #169890, #137416, #203435, #42060, #74543, #25772, #38837, #204504, #56154, #188273, #39914, #55089, #24703, #121238, #90805, #89745, #106023, #21479, #156869, #157939, #153660, #5229, #172044, #23637, #155794, #73457, #140643, #7378, #139559, #205586, #57223, #58288, #123383, #107099, #124445, #194674, #63617, #47392, #31133, #13783, #211977, #144909, #126572, #111372, #79858, #129772, #78787, #28990, #125504, #193612, #209844, #192532, #60411, #162196, #26842, #113505, #208781, #179513, #195755, #44186, #96145, #160053, #177376, #45254, #145967, #80932, #191467, #147023, #97208, #163260, #76661, #95076, #175256, #14842, #161125, #127648, #12711, #112434, #176314, #27918, #142775, #94014, #109248, #110306, #11657, #77730, #210916, #143852, #61483, #62543, #213046, #128705, #43132, #46318, #92945, #158990, #10586, #178447 ),
 ( #30055, #117765, #164315, #67839, #131857, #181612, #16967, #49496, #148076, #98258, #35365, #183756, #165374, #64675, #196812, #18037, #51641, #101440, #86260, #99324, #214082, #118819, #34302, #167514, #15906, #36435, #184806, #83048, #66769, #19111, #33241, #85189, #149123, #100375, #20173, #130821, #81988, #1782, #132910, #182681, #84124, #115617, #114568, #705, #65709, #198915, #201047, #180560, #133985, #48455, #168573, #32182, #50561, #199992, #197864, #116682, #166445, #150210, #151272, #2845, #152331, #68914, #135034, #52690, #102511, #103585, #124190, #4969, #185873, #53766, #89485, #155540, #138230, #39644, #202106, #58026, #55895, #190153, #54833, #40729, #119899, #189096, #136089, #186951, #88405, #72122, #41808, #7119, #25519, #106835, #107921, #173946, #120983, #91627, #104660, #140382, #37509, #169643, #8202, #21227, #154473, #24437, #3908, #205327, #206401, #38583, #203187, #69978, #73192, #71047, #139298, #87331, #153398, #137163, #74287, #172866, #170707, #22292, #6051, #204243, #122052, #188016, #105752, #56965, #171779, #123138, #23375, #90548, #156612, #62296, #129519, #30879, #113252, #179257, #76402, #159790, #45000, #128455, #142511, #11393, #157679, #9277, #46064, #75348, #158733, #194423, #12461, #95891, #79606, #63363, #112185, #29805, #177114, #10328, #143590, #178189, #161944, #111110, #61228, #141463, #77471, #27656, #208520, #92687, #13536, #59089, #145725, #26586, #211725, #195499, #60155, #47135, #192271, #209582, #127383, #207470, #125249, #191210, #126311, #42873, #193356, #43932, #28731, #110047, #108981, #94816, #175000, #176060, #93752, #160867, #78536, #144653, #210668, #165123, #146776, #134785, #66516, #99070, #16714, #83861, #147823, #213841, #114317, #65460, #80685, #164074, #15654, #180315, #82799, #98019, #81741, #131611, #52443, #197610, #200792, #49254, #148875, #198663, #67585, #115375, #448, #184555, #163006, #199737, #118569, #181369, #133730, #166184, #35105, #18850, #2592, #51383, #183496, #116429, #32993, #132659, #117504, #101176, #50311, #182422, #96958 ) ),
 .UNSPECIFIED., .F., .F., .T. ) 
 B_SPLINE_SURFACE_WITH_KNOTS ( ( 2, 2 ),
 ( 3, 2, 2, 2, 2, 2, 2, 2, 2, 2, 2, 2, 2, 2, 2, 2, 2, 2, 2, 2, 2, 2, 2, 2, 2, 2, 2, 2, 2, 2, 2, 2, 2, 2, 2, 2, 2, 2, 2, 2, 2, 2, 2, 2, 2, 2, 2, 2, 2, 2, 2, 2, 2, 2, 2, 2, 2, 2, 2, 2, 2, 2, 2, 2, 2, 2, 2, 2, 2, 2, 2, 2, 2, 2, 2, 2, 2, 2, 2, 2, 2, 2, 2, 2, 2, 2, 2, 2, 2, 2, 2, 2, 2, 2, 2, 2, 2, 2, 2, 2, 2, 2, 2, 2, 2, 2, 2, 2, 2, 2, 2, 2, 2, 2, 2, 2, 2, 2, 2, 2, 3 ),
 ( 0.000000000000000000, 1.000000000000000000 ),
 ( 0.000000000000000000, 0.008333333333333333218, 0.01666666666666666644, 0.02500000000000000139, 0.03333333333333333287, 0.04166666666666666435, 0.05000000000000000278, 0.05833333333333333426, 0.06666666666666666574, 0.07499999999999999722, 0.08333333333333332871, 0.09166666666666666019, 0.1000000000000000056, 0.1083333333333333370, 0.1166666666666666685, 0.1250000000000000000, 0.1333333333333333315, 0.1416666666666666630, 0.1499999999999999944, 0.1583333333333333259, 0.1666666666666666574, 0.1749999999999999889, 0.1833333333333333204, 0.1916666666666666796, 0.2000000000000000111, 0.2083333333333333426, 0.2166666666666666741, 0.2250000000000000056, 0.2333333333333333370, 0.2416666666666666685, 0.2500000000000000000, 0.2583333333333333592, 0.2666666666666666630, 0.2750000000000000222, 0.2833333333333333259, 0.2916666666666666852, 0.2999999999999999889, 0.3083333333333333481, 0.3166666666666666519, 0.3250000000000000111, 0.3333333333333333148, 0.3416666666666666741, 0.3499999999999999778, 0.3583333333333333370, 0.3666666666666666408, 0.3750000000000000000, 0.3833333333333333592, 0.3916666666666666630, 0.4000000000000000222, 0.4083333333333333259, 0.4166666666666666852, 0.4249999999999999889, 0.4333333333333333481, 0.4416666666666666519, 0.4500000000000000111, 0.4583333333333333148, 0.4666666666666666741, 0.4749999999999999778, 0.4833333333333333370, 0.4916666666666666408, 0.5000000000000000000, 0.5083333333333333037, 0.5166666666666667185, 0.5250000000000000222, 0.5333333333333333259, 0.5416666666666666297, 0.5500000000000000444, 0.5583333333333333481, 0.5666666666666666519, 0.5749999999999999556, 0.5833333333333333703, 0.5916666666666666741, 0.5999999999999999778, 0.6083333333333332815, 0.6166666666666666963, 0.6250000000000000000, 0.6333333333333333037, 0.6416666666666667185, 0.6500000000000000222, 0.6583333333333333259, 0.6666666666666666297, 0.6750000000000000444, 0.6833333333333333481, 0.6916666666666666519, 0.6999999999999999556, 0.7083333333333333703, 0.7166666666666666741, 0.7249999999999999778, 0.7333333333333332815, 0.7416666666666666963, 0.7500000000000000000, 0.7583333333333333037, 0.7666666666666667185, 0.7750000000000000222, 0.7833333333333333259, 0.7916666666666666297, 0.8000000000000000444, 0.8083333333333333481, 0.8166666666666666519, 0.8249999999999999556, 0.8333333333333333703, 0.8416666666666666741, 0.8499999999999999778, 0.8583333333333332815, 0.8666666666666666963, 0.8750000000000000000, 0.8833333333333333037, 0.8916666666666667185, 0.9000000000000000222, 0.9083333333333333259, 0.9166666666666666297, 0.9250000000000000444, 0.9333333333333333481, 0.9416666666666666519, 0.9499999999999999556, 0.9583333333333333703, 0.9666666666666666741, 0.9749999999999999778, 0.9833333333333332815, 0.9916666666666666963, 1.000000000000000000 ),
 .UNSPECIFIED. ) 
 GEOMETRIC_REPRESENTATION_ITEM ( )  RATIONAL_B_SPLINE_SURFACE ( (
 ( 1.000000000000000000, 0.8660254037844387076, 1.000000000000000000, 0.8660254037844387076, 1.000000000000000000, 0.8660254037844387076, 1.000000000000000000, 0.8660254037844387076, 1.000000000000000000, 0.8660254037844387076, 1.000000000000000000, 0.8660254037844387076, 1.000000000000000000, 0.8660254037844387076, 1.000000000000000000, 0.8660254037844387076, 1.000000000000000000, 0.8660254037844387076, 1.000000000000000000, 0.8660254037844387076, 1.000000000000000000, 0.8660254037844387076, 1.000000000000000000, 0.8660254037844387076, 1.000000000000000000, 0.8660254037844387076, 1.000000000000000000, 0.8660254037844387076, 1.000000000000000000, 0.8660254037844387076, 1.000000000000000000, 0.8660254037844387076, 1.000000000000000000, 0.8660254037844387076, 1.000000000000000000, 0.8660254037844387076, 1.000000000000000000, 0.8660254037844387076, 1.000000000000000000, 0.8660254037844387076, 1.000000000000000000, 0.8660254037844387076, 1.000000000000000000, 0.8660254037844387076, 1.000000000000000000, 0.8660254037844387076, 1.000000000000000000, 0.8660254037844387076, 1.000000000000000000, 0.8660254037844387076, 1.000000000000000000, 0.8660254037844387076, 1.000000000000000000, 0.8660254037844387076, 1.000000000000000000, 0.8660254037844387076, 1.000000000000000000, 0.8660254037844387076, 1.000000000000000000, 0.8660254037844387076, 1.000000000000000000, 0.8660254037844387076, 1.000000000000000000, 0.8660254037844387076, 1.000000000000000000, 0.8660254037844387076, 1.000000000000000000, 0.8660254037844387076, 1.000000000000000000, 0.8660254037844387076, 1.000000000000000000, 0.8660254037844387076, 1.000000000000000000, 0.8660254037844387076, 1.000000000000000000, 0.8660254037844387076, 1.000000000000000000, 0.8660254037844387076, 1.000000000000000000, 0.8660254037844387076, 1.000000000000000000, 0.8660254037844387076, 1.000000000000000000, 0.8660254037844387076, 1.000000000000000000, 0.8660254037844387076, 1.000000000000000000, 0.8660254037844387076, 1.000000000000000000, 0.8660254037844387076, 1.000000000000000000, 0.8660254037844387076, 1.000000000000000000, 0.8660254037844387076, 1.000000000000000000, 0.8660254037844387076, 1.000000000000000000, 0.8660254037844387076, 1.000000000000000000, 0.8660254037844387076, 1.000000000000000000, 0.8660254037844387076, 1.000000000000000000, 0.8660254037844387076, 1.000000000000000000, 0.8660254037844387076, 1.000000000000000000, 0.8660254037844387076, 1.000000000000000000, 0.8660254037844387076, 1.000000000000000000, 0.8660254037844387076, 1.000000000000000000, 0.8660254037844387076, 1.000000000000000000, 0.8660254037844387076, 1.000000000000000000, 0.8660254037844387076, 1.000000000000000000, 0.8660254037844387076, 1.000000000000000000, 0.8660254037844387076, 1.000000000000000000, 0.8660254037844387076, 1.000000000000000000, 0.8660254037844387076, 1.000000000000000000, 0.8660254037844387076, 1.000000000000000000, 0.8660254037844387076, 1.000000000000000000, 0.8660254037844387076, 1.000000000000000000, 0.8660254037844387076, 1.000000000000000000, 0.8660254037844387076, 1.000000000000000000, 0.8660254037844387076, 1.000000000000000000, 0.8660254037844387076, 1.000000000000000000, 0.8660254037844387076, 1.000000000000000000, 0.8660254037844387076, 1.000000000000000000, 0.8660254037844387076, 1.000000000000000000, 0.8660254037844387076, 1.000000000000000000, 0.8660254037844387076, 1.000000000000000000, 0.8660254037844387076, 1.000000000000000000, 0.8660254037844387076, 1.000000000000000000, 0.8660254037844387076, 1.000000000000000000, 0.8660254037844387076, 1.000000000000000000, 0.8660254037844387076, 1.000000000000000000, 0.8660254037844387076, 1.000000000000000000, 0.8660254037844387076, 1.000000000000000000, 0.8660254037844387076, 1.000000000000000000, 0.8660254037844387076, 1.000000000000000000, 0.8660254037844387076, 1.000000000000000000, 0.8660254037844387076, 1.000000000000000000, 0.8660254037844387076, 1.000000000000000000, 0.8660254037844387076, 1.000000000000000000, 0.8660254037844387076, 1.000000000000000000, 0.8660254037844387076, 1.000000000000000000, 0.8660254037844387076, 1.000000000000000000, 0.8660254037844387076, 1.000000000000000000, 0.8660254037844387076, 1.000000000000000000, 0.8660254037844387076, 1.000000000000000000, 0.8660254037844387076, 1.000000000000000000, 0.8660254037844387076, 1.000000000000000000, 0.8660254037844387076, 1.000000000000000000, 0.8660254037844387076, 1.000000000000000000, 0.8660254037844387076, 1.000000000000000000, 0.8660254037844387076, 1.000000000000000000, 0.8660254037844387076, 1.000000000000000000, 0.8660254037844387076, 1.000000000000000000, 0.8660254037844387076, 1.000000000000000000, 0.8660254037844387076, 1.000000000000000000, 0.8660254037844387076, 1.000000000000000000, 0.8660254037844387076, 1.000000000000000000, 0.8660254037844387076, 1.000000000000000000, 0.8660254037844387076, 1.000000000000000000, 0.8660254037844387076, 1.000000000000000000, 0.8660254037844387076, 1.000000000000000000, 0.8660254037844387076, 1.000000000000000000, 0.8660254037844387076, 1.000000000000000000, 0.8660254037844387076, 1.000000000000000000, 0.8660254037844387076, 1.000000000000000000, 0.8660254037844387076, 1.000000000000000000, 0.8660254037844387076, 1.000000000000000000, 0.8660254037844387076, 1.000000000000000000, 0.8660254037844387076, 1.000000000000000000, 0.8660254037844387076, 1.000000000000000000, 0.8660254037844387076, 1.000000000000000000),
 ( 1.000000000000000000, 0.8660254037844387076, 1.000000000000000000, 0.8660254037844387076, 1.000000000000000000, 0.8660254037844387076, 1.000000000000000000, 0.8660254037844387076, 1.000000000000000000, 0.8660254037844387076, 1.000000000000000000, 0.8660254037844387076, 1.000000000000000000, 0.8660254037844387076, 1.000000000000000000, 0.8660254037844387076, 1.000000000000000000, 0.8660254037844387076, 1.000000000000000000, 0.8660254037844387076, 1.000000000000000000, 0.8660254037844387076, 1.000000000000000000, 0.8660254037844387076, 1.000000000000000000, 0.8660254037844387076, 1.000000000000000000, 0.8660254037844387076, 1.000000000000000000, 0.8660254037844387076, 1.000000000000000000, 0.8660254037844387076, 1.000000000000000000, 0.8660254037844387076, 1.000000000000000000, 0.8660254037844387076, 1.000000000000000000, 0.8660254037844387076, 1.000000000000000000, 0.8660254037844387076, 1.000000000000000000, 0.8660254037844387076, 1.000000000000000000, 0.8660254037844387076, 1.000000000000000000, 0.8660254037844387076, 1.000000000000000000, 0.8660254037844387076, 1.000000000000000000, 0.8660254037844387076, 1.000000000000000000, 0.8660254037844387076, 1.000000000000000000, 0.8660254037844387076, 1.000000000000000000, 0.8660254037844387076, 1.000000000000000000, 0.8660254037844387076, 1.000000000000000000, 0.8660254037844387076, 1.000000000000000000, 0.8660254037844387076, 1.000000000000000000, 0.8660254037844387076, 1.000000000000000000, 0.8660254037844387076, 1.000000000000000000, 0.8660254037844387076, 1.000000000000000000, 0.8660254037844387076, 1.000000000000000000, 0.8660254037844387076, 1.000000000000000000, 0.8660254037844387076, 1.000000000000000000, 0.8660254037844387076, 1.000000000000000000, 0.8660254037844387076, 1.000000000000000000, 0.8660254037844387076, 1.000000000000000000, 0.8660254037844387076, 1.000000000000000000, 0.8660254037844387076, 1.000000000000000000, 0.8660254037844387076, 1.000000000000000000, 0.8660254037844387076, 1.000000000000000000, 0.8660254037844387076, 1.000000000000000000, 0.8660254037844387076, 1.000000000000000000, 0.8660254037844387076, 1.000000000000000000, 0.8660254037844387076, 1.000000000000000000, 0.8660254037844387076, 1.000000000000000000, 0.8660254037844387076, 1.000000000000000000, 0.8660254037844387076, 1.000000000000000000, 0.8660254037844387076, 1.000000000000000000, 0.8660254037844387076, 1.000000000000000000, 0.8660254037844387076, 1.000000000000000000, 0.8660254037844387076, 1.000000000000000000, 0.8660254037844387076, 1.000000000000000000, 0.8660254037844387076, 1.000000000000000000, 0.8660254037844387076, 1.000000000000000000, 0.8660254037844387076, 1.000000000000000000, 0.8660254037844387076, 1.000000000000000000, 0.8660254037844387076, 1.000000000000000000, 0.8660254037844387076, 1.000000000000000000, 0.8660254037844387076, 1.000000000000000000, 0.8660254037844387076, 1.000000000000000000, 0.8660254037844387076, 1.000000000000000000, 0.8660254037844387076, 1.000000000000000000, 0.8660254037844387076, 1.000000000000000000, 0.8660254037844387076, 1.000000000000000000, 0.8660254037844387076, 1.000000000000000000, 0.8660254037844387076, 1.000000000000000000, 0.8660254037844387076, 1.000000000000000000, 0.8660254037844387076, 1.000000000000000000, 0.8660254037844387076, 1.000000000000000000, 0.8660254037844387076, 1.000000000000000000, 0.8660254037844387076, 1.000000000000000000, 0.8660254037844387076, 1.000000000000000000, 0.8660254037844387076, 1.000000000000000000, 0.8660254037844387076, 1.000000000000000000, 0.8660254037844387076, 1.000000000000000000, 0.8660254037844387076, 1.000000000000000000, 0.8660254037844387076, 1.000000000000000000, 0.8660254037844387076, 1.000000000000000000, 0.8660254037844387076, 1.000000000000000000, 0.8660254037844387076, 1.000000000000000000, 0.8660254037844387076, 1.000000000000000000, 0.8660254037844387076, 1.000000000000000000, 0.8660254037844387076, 1.000000000000000000, 0.8660254037844387076, 1.000000000000000000, 0.8660254037844387076, 1.000000000000000000, 0.8660254037844387076, 1.000000000000000000, 0.8660254037844387076, 1.000000000000000000, 0.8660254037844387076, 1.000000000000000000, 0.8660254037844387076, 1.000000000000000000, 0.8660254037844387076, 1.000000000000000000, 0.8660254037844387076, 1.000000000000000000, 0.8660254037844387076, 1.000000000000000000, 0.8660254037844387076, 1.000000000000000000, 0.8660254037844387076, 1.000000000000000000, 0.8660254037844387076, 1.000000000000000000, 0.8660254037844387076, 1.000000000000000000, 0.8660254037844387076, 1.000000000000000000, 0.8660254037844387076, 1.000000000000000000, 0.8660254037844387076, 1.000000000000000000, 0.8660254037844387076, 1.000000000000000000, 0.8660254037844387076, 1.000000000000000000, 0.8660254037844387076, 1.000000000000000000, 0.8660254037844387076, 1.000000000000000000, 0.8660254037844387076, 1.000000000000000000, 0.8660254037844387076, 1.000000000000000000, 0.8660254037844387076, 1.000000000000000000, 0.8660254037844387076, 1.000000000000000000, 0.8660254037844387076, 1.000000000000000000, 0.8660254037844387076, 1.000000000000000000, 0.8660254037844387076, 1.000000000000000000, 0.8660254037844387076, 1.000000000000000000, 0.8660254037844387076, 1.000000000000000000, 0.8660254037844387076, 1.000000000000000000, 0.8660254037844387076, 1.000000000000000000, 0.8660254037844387076, 1.000000000000000000, 0.8660254037844387076, 1.000000000000000000) ) ) 
 REPRESENTATION_ITEM ( '' )  SURFACE ( )  );
#208019=CARTESIAN_POINT ( 'NONE',  ( 3.528865121306874464, 7.339036084825155015, -0.7998128361456362523 ) ) ;
#208037=CARTESIAN_POINT ( 'NONE',  ( -6.981522756394290319, 7.109807735406931783, 0.7998128361456341429 ) ) ;
#208051=CARTESIAN_POINT ( 'NONE',  ( 5.585032934186686226, 5.480569609498057382, 0.000000000000000000 ) ) ;
#208060=CARTESIAN_POINT ( 'NONE',  ( -4.136646265500965924, 7.840188053144151681, -0.7216878364870512597 ) ) ;
#208062=CARTESIAN_POINT ( 'NONE',  ( 4.798147134389644464, 8.131168186839138556, 0.8272934513729796047 ) ) ;
#208081=ORIENTED_EDGE ( 'NONE', *, *, #180932, .T. ) ;
#208083=CARTESIAN_POINT ( 'NONE',  ( -4.847922445338252118, 7.813604065273374921, -1.199719254218453823 ) ) ;
#208085=CARTESIAN_POINT ( 'NONE',  ( 4.923546060418115822, 5.773167154356443120, -1.199719254218452047 ) ) ;
#208089=CARTESIAN_POINT ( 'NONE',  ( -6.608673532018475960, 6.674816973635147477, -0.7998128361456362523 ) ) ;
#208093=CARTESIAN_POINT ( 'NONE',  ( 5.688757509019037428, 5.629766575900002401, 2.500000000000000000 ) ) ;
#208098=CARTESIAN_POINT ( 'NONE',  ( -4.953783236630994402, 8.080086878320878796, -1.094444140625696837 ) ) ;
#208099=DIRECTION ( 'NONE',  ( 0.000000000000000000, 1.000000000000000000, 0.000000000000000000 ) ) ;
#208109=ADVANCED_FACE ( 'NONE', ( #206209 ), #160680, .F. ) ;
#208115=CARTESIAN_POINT ( 'NONE',  ( 3.757017964762656703, 7.397288368949487491, -1.734723475976807094E-15 ) ) ;
#208116=CARTESIAN_POINT ( 'NONE',  ( 5.398914348987510436, 6.259949555863199677, -2.420000000000000373 ) ) ;
#208119=CARTESIAN_POINT ( 'NONE',  ( -7.937372586157736443, 8.224965870130965584, 0.7998128361456341429 ) ) ;
#208127=CARTESIAN_POINT ( 'NONE',  ( -2.875737979874388284, 6.369128386579808954, -0.7216878364870458196 ) ) ;
#208133=CARTESIAN_POINT ( 'NONE',  ( 4.899292406491845497, 6.809203455697518947, -1.599625672291273171 ) ) ;
#208148=ORIENTED_EDGE ( 'NONE', *, *, #19773, .F. ) ;
#208158=LINE ( 'NONE', #90179, #118339 ) ;
#208162=EDGE_CURVE ( 'NONE', #105939, #35911, #51574, .T. ) ;
#208179=CARTESIAN_POINT ( 'NONE',  ( 5.076602173674213070, 4.887400388900169368, 0.000000000000000000 ) ) ;
#208183=CARTESIAN_POINT ( 'NONE',  ( -7.795011973214244883, 8.058878488363559356, 0.7998128361456341429 ) ) ;
#208188=ORIENTED_EDGE ( 'NONE', *, *, #83083, .T. ) ;
#208189=CARTESIAN_POINT ( 'NONE',  ( -5.472651281771599763, 6.413789912602166687, 1.199719254218452935 ) ) ;
#208197=CARTESIAN_POINT ( 'NONE',  ( -3.806807270387036368, 7.663301925418665839, 0.000000000000000000 ) ) ;
#208199=CARTESIAN_POINT ( 'NONE',  ( 5.612152705277200226, 7.484198595525810127, -1.333638438132278559 ) ) ;
#208204=CARTESIAN_POINT ( 'NONE',  ( 3.932747076415766596, 6.745899468197171345, 1.199719254218451159 ) ) ;
#208210=CARTESIAN_POINT ( 'NONE',  ( -8.072954122294394352, 8.383144328957069291, -0.7998128361456362523 ) ) ;
#208215=CARTESIAN_POINT ( 'NONE',  ( -3.949167883330528372, 7.829389307186077396, 1.214306433183764966E-14 ) ) ;
#208219=CARTESIAN_POINT ( 'NONE',  ( 6.522881301506172846, 6.782652071278222117, -0.7216878364870458196 ) ) ;
#208220=CARTESIAN_POINT ( 'NONE',  ( -5.872089928050201024, 8.904503111816948646, 1.082531754730550855 ) ) ;
#208224=CARTESIAN_POINT ( 'NONE',  ( -5.285699784481336927, 7.260012063351913625, 1.599625672291263401 ) ) ;
#208228=CARTESIAN_POINT ( 'NONE',  ( 3.203469434578891661, 6.959407783642502565, -0.7998128361456362523 ) ) ;
#208236=CARTESIAN_POINT ( 'NONE',  ( 4.193214648376505593, 8.114110533073061404, 0.000000000000000000 ) ) ;
#208256=CARTESIAN_POINT ( 'NONE',  ( 4.614363445337835934, 8.349151705029461468, -0.2795175495247017583 ) ) ;
#208264=CARTESIAN_POINT ( 'NONE',  ( 6.587282531393223728, 8.778525268082516320, 1.599625672291268286 ) ) ;
#208269=CARTESIAN_POINT ( 'NONE',  ( -4.651028767811522080, 8.324525799487361155, 0.4279074293446327171 ) ) ;
#208272=EDGE_CURVE ( 'NONE', #41470, #75032, #134624, .T. ) ;
#208275=CARTESIAN_POINT ( 'NONE',  ( -5.921879234118920365, 10.13088588310589699, 0.000000000000000000 ) ) ;
#208279=CARTESIAN_POINT ( 'NONE',  ( -3.730655187671924722, 7.355891203230078723, 0.6115009643793259952 ) ) ;
#208287=CARTESIAN_POINT ( 'NONE',  ( 6.444921918449731280, 8.612437886315108315, 1.599625672291268286 ) ) ;
#208298=CARTESIAN_POINT ( 'NONE',  ( 5.578253857379852576, 5.472660686556754861, -0.7998128361456481317 ) ) ;
#208302=CARTESIAN_POINT ( 'NONE',  ( 5.356880090730863131, 7.343055753976412525, 1.443375672974064550 ) ) ;
#208310=CARTESIAN_POINT ( 'NONE',  ( -6.232040409365024125, 6.934648621905299848, 0.8351839086257698552 ) ) ;
#208317=CARTESIAN_POINT ( 'NONE',  ( -3.797165540279144214, 6.587721009371067638, 1.199719254218452935 ) ) ;
#208318=CARTESIAN_POINT ( 'NONE',  ( 5.533136088152891929, 9.469426179571447832, -0.7216878364870458196 ) ) ;
#208327=EDGE_LOOP ( 'NONE', ( #99905, #36391, #112621, #22231, #89137, #15955 ) ) ;
#208330=CARTESIAN_POINT ( 'NONE',  ( -6.448838341955544173, 7.552674816150118708, 1.199719254218452047 ) ) ;
#208331=CARTESIAN_POINT ( 'NONE',  ( -5.635349125135588721, 6.603604063193491136, 1.199719254218452935 ) ) ;
#208333=CARTESIAN_POINT ( 'NONE',  ( 6.739811759324814133, 8.956476034002680109, -1.443375672974078761 ) ) ;
#208345=CARTESIAN_POINT ( 'NONE',  ( -5.826481282663010575, 7.222486169913409526, -1.172043233395845485 ) ) ;
#208346=DIRECTION ( 'NONE',  ( -1.000000000000000000, 0.000000000000000000, 0.000000000000000000 ) ) ;
#208350=CARTESIAN_POINT ( 'NONE',  ( 5.560252395380222090, 5.659585014131299552, 0.7216878364870328300 ) ) ;
#208354=CARTESIAN_POINT ( 'NONE',  ( -6.038177310039794854, 8.137902509836795417, -1.599625672291271394 ) ) ;
#208370=CARTESIAN_POINT ( 'NONE',  ( 7.015418140428412386, 7.149352350113456822, 0.7998128361456331437 ) ) ;
#208377=DIRECTION ( 'NONE',  ( 0.7592566023653005702, -0.6507913734559640506, 0.000000000000000000 ) ) ;
#208403=CARTESIAN_POINT ( 'NONE',  ( 6.536439455564164724, 7.758839131980592718, 1.082531754730549967 ) ) ;
#208432=CARTESIAN_POINT ( 'NONE',  ( -3.156015896931072540, 6.904045323053366268, 0.000000000000000000 ) ) ;
#208434=CARTESIAN_POINT ( 'NONE',  ( 5.031484404002879884, 6.963427452793765404, 1.443375672974065660 ) ) ;
#208439=CARTESIAN_POINT ( 'NONE',  ( -5.061990249855848667, 6.999017606288844284, -1.599625672291271394 ) ) ;
#208443=CARTESIAN_POINT ( 'NONE',  ( -4.981695098378565945, 4.776675467721892332, -0.7998128361456362523 ) ) ;
#208452=CARTESIAN_POINT ( 'NONE',  ( -3.786470039966538970, 7.639575156594750283, 0.000000000000000000 ) ) ;
#208461=CARTESIAN_POINT ( 'NONE',  ( -3.623772196602547346, 7.449761006003425834, 0.000000000000000000 ) ) ;
#208464=CARTESIAN_POINT ( 'NONE',  ( -7.119440060951841787, 7.478637290631501067, 0.000000000000000000 ) ) ;
#208465=CARTESIAN_POINT ( 'NONE',  ( -5.844973620822877969, 7.912498205750389424, 1.443375672974058777 ) ) ;
#208466=CARTESIAN_POINT ( 'NONE',  ( 5.037736595929563244, 8.035053907629919223, -1.199719254218452047 ) ) ;
#208467=CARTESIAN_POINT ( 'NONE',  ( -7.391130018105325661, 8.652015104991543026, -1.199719254218452047 ) ) ;
#208485=CARTESIAN_POINT ( 'NONE',  ( 6.502017186205484300, 9.743381262951846367, -1.199719254218452047 ) ) ;
#208505=CARTESIAN_POINT ( 'NONE',  ( 4.601164721245145195, 8.482418317249249995, 0.1585857521721554253 ) ) ;
#208520=CARTESIAN_POINT ( 'NONE',  ( 5.027041095616958444, 9.086908054853605421, 0.000000000000000000 ) ) ;
#208523=CARTESIAN_POINT ( 'NONE',  ( -4.950662367645459305, 5.804802846121667415, -1.199719254218453823 ) ) ;
#208526=CARTESIAN_POINT ( 'NONE',  ( -5.587368702163209910, 9.532697562583475559, 0.000000000000000000 ) ) ;
#208537=CARTESIAN_POINT ( 'NONE',  ( 5.671053392266061977, 9.838255734277600695, 0.7998128361456331437 ) ) ;
#208538=CARTESIAN_POINT ( 'NONE',  ( 4.854701522145073334, 7.821512988214679218, -1.199719254218450271 ) ) ;
#208552=CARTESIAN_POINT ( 'NONE',  ( 6.119526231721748033, 8.232809585132461194, 1.599625672291269396 ) ) ;
#208556=DIRECTION ( 'NONE',  ( 0.000000000000000000, 1.000000000000000000, 1.496258514059622730E-16 ) ) ;
#208564=CARTESIAN_POINT ( 'NONE',  ( -5.207740401424942434, 6.208690235484773723, 1.082531754730549078 ) ) ;
#208565=CARTESIAN_POINT ( 'NONE',  ( -7.761116589180078407, 8.019333873657032541, 0.000000000000000000 ) ) ;
#208567=CARTESIAN_POINT ( 'NONE',  ( -4.842962054798890748, 4.879744820279569240, 0.4763033239258877560 ) ) ;
#208570=( BOUNDED_CURVE ( )  B_SPLINE_CURVE ( 2, ( #202489, #105040, #4284, #134359, #70355 ),
 .UNSPECIFIED., .F., .T. ) 
 B_SPLINE_CURVE_WITH_KNOTS ( ( 3, 2, 3 ),
 ( 0.02164518822461731357, 0.02500000000000000139, 0.02792328123870144521 ),
 .UNSPECIFIED. ) 
 CURVE ( )  GEOMETRIC_REPRESENTATION_ITEM ( )  RATIONAL_B_SPLINE_CURVE ( ( 0.9355558506697161381, 0.9460648536416673693, 1.000000000000000000, 0.9530025491704537943, 0.9389779222473411124 ) ) 
 REPRESENTATION_ITEM ( '' )  );
#208578=CARTESIAN_POINT ( 'NONE',  ( 6.527324610336440180, 6.579909898339485252, 0.7998128361456331437 ) ) ;
#208579=CARTESIAN_POINT ( 'NONE',  ( 6.713222337422018349, 7.861122810861019161, -1.199719254218452047 ) ) ;
#208582=CARTESIAN_POINT ( 'NONE',  ( 8.011942431032855083, 8.311964022485323511, 0.7998128361456291469 ) ) ;
#208600=B_SPLINE_CURVE_WITH_KNOTS ( 'NONE', 3,
 ( #1627, #67686, #133832, #52538, #69825, #51485 ),
 .UNSPECIFIED., .F., .F.,
 ( 4, 2, 4 ),
 ( 0.001525776914076238918, 0.001915068532333861259, 0.002304360150591483816 ),
 .UNSPECIFIED. ) ;
#208603=CARTESIAN_POINT ( 'NONE',  ( 4.248501033035879004, 6.049946853332221153, -1.599625672291273171 ) ) ;
#208605=CARTESIAN_POINT ( 'NONE',  ( -2.830620210203090181, 6.524417021870718258, 0.000000000000000000 ) ) ;
#208607=CARTESIAN_POINT ( 'NONE',  ( 3.874598038455354665, 7.742391154831717692, -0.7998128361456362523 ) ) ;
#208613=LINE ( 'NONE', #74376, #56372 ) ;
#208617=CARTESIAN_POINT ( 'NONE',  ( 5.885648082108177803, 9.880690172519326353, 0.7216878364870317197 ) ) ;
#208619=CARTESIAN_POINT ( 'NONE',  ( -5.433785704026946384, 9.561443431331920095, 0.000000000000000000 ) ) ;
#208620=CARTESIAN_POINT ( 'NONE',  ( 3.705121118284530279, 7.544668081299086282, -1.734723475976807094E-15 ) ) ;
#208628=EDGE_CURVE ( 'NONE', #88097, #188712, #158964, .T. ) ;
#208631=CARTESIAN_POINT ( 'NONE',  ( -5.808742468812186033, 5.741564066561132940, 0.000000000000000000 ) ) ;
#208646=( BOUNDED_SURFACE ( )  B_SPLINE_SURFACE ( 3, 2, ( 
 ( #84894, #66479, #31902 ),
 ( #166145, #53462, #67546 ),
 ( #81702, #182379, #115337 ),
 ( #198625, #50272, #34009 ),
 ( #150982, #68621, #17731 ),
 ( #133690, #199694, #183457 ),
 ( #35063, #101134, #36133 ),
 ( #167222, #147784, #131572 ),
 ( #200753, #52402, #168284 ),
 ( #152041, #19882, #85966 ) ),
 .UNSPECIFIED., .F., .F., .T. ) 
 B_SPLINE_SURFACE_WITH_KNOTS ( ( 4, 2, 2, 2, 4 ),
 ( 3, 3 ),
 ( 0.000000000000000000, 0.0003762414628101696688, 0.0007524829256203393376, 0.001128724388430508898, 0.001504965851240678675 ),
 ( 0.000000000000000000, 1.000000000000000000 ),
 .UNSPECIFIED. ) 
 GEOMETRIC_REPRESENTATION_ITEM ( )  RATIONAL_B_SPLINE_SURFACE ( (
 ( 1.000000000000000000, 0.7796368470575135712, 1.000000000000000000),
 ( 1.000000000000000000, 0.7902951223000224124, 1.000000000000000000),
 ( 1.000000000000000000, 0.7826420995578321493, 1.000000000000000000),
 ( 1.000000000000000000, 0.7484677895294554739, 1.000000000000000000),
 ( 1.000000000000000000, 0.7229395345770123216, 1.000000000000000000),
 ( 1.000000000000000000, 0.7019560918380093328, 1.000000000000000000),
 ( 1.000000000000000000, 0.7093811322644433259, 1.000000000000000000),
 ( 1.000000000000000000, 0.7456665127358711453, 1.000000000000000000),
 ( 1.000000000000000000, 0.7703623356575411973, 1.000000000000000000),
 ( 1.000000000000000000, 0.7796377409682134774, 1.000000000000000000) ) ) 
 REPRESENTATION_ITEM ( '' )  SURFACE ( )  );
#208666=CARTESIAN_POINT ( 'NONE',  ( 7.343676480457483002, 8.596652644402405841, -1.199719254218452047 ) ) ;
#208667=CARTESIAN_POINT ( 'NONE',  ( 4.760321331729593375, 5.686701320840210627, -1.082531754730548412 ) ) ;
#208679=CARTESIAN_POINT ( 'NONE',  ( -4.308458954092677651, 8.248562223075252220, -0.7998128361456362523 ) ) ;
#208681=CARTESIAN_POINT ( 'NONE',  ( -5.855142236255304944, 7.924361590421551860, -1.599625672291271394 ) ) ;
#208683=CARTESIAN_POINT ( 'NONE',  ( 7.824464048418096951, 8.301165276008827476, -0.7216878364870317197 ) ) ;
#208694=CARTESIAN_POINT ( 'NONE',  ( -4.423703259808839938, 8.383013913077441259, 0.7998128361456352531 ) ) ;
#208701=CARTESIAN_POINT ( 'NONE',  ( -5.980555157403903976, 6.149938236492225485, 0.000000000000000000 ) ) ;
#208703=ORIENTED_EDGE ( 'NONE', *, *, #106933, .F. ) ;
#208705=CARTESIAN_POINT ( 'NONE',  ( -4.450819567036169211, 8.414649604842665553, -0.7998128361456362523 ) ) ;
#208714=CARTESIAN_POINT ( 'NONE',  ( 4.663288057535367237, 8.288536188413402783, 0.5084364831346009916 ) ) ;
#208727=CARTESIAN_POINT ( 'NONE',  ( -6.038177310039794854, 8.137902509836795417, -1.599625672291271394 ) ) ;
#208729=CARTESIAN_POINT ( 'NONE',  ( -4.132202957115018727, 8.042930226601317401, 0.000000000000000000 ) ) ;
#208756=CARTESIAN_POINT ( 'NONE',  ( -6.038177310039794854, 8.137902509836795417, -1.599625672291271394 ) ) ;
#208781=CARTESIAN_POINT ( 'NONE',  ( 5.508355548902068577, 9.648441583686274470, 0.7998128361456331437 ) ) ;
#208790=B_SPLINE_CURVE_WITH_KNOTS ( 'NONE', 3,
 ( #189559, #201517, #70449, #136564 ),
 .UNSPECIFIED., .F., .F.,
 ( 4, 4 ),
 ( 0.000000000000000000, 0.0001618775200852311160 ),
 .UNSPECIFIED. ) ;
#208795=CARTESIAN_POINT ( 'NONE',  ( 5.279289985772466665, 7.652873027719338417, 1.222721368963412214 ) ) ;
#208797=CARTESIAN_POINT ( 'NONE',  ( 5.221298555038576872, 9.105615724271411082, 0.000000000000000000 ) ) ;
#208804=CARTESIAN_POINT ( 'NONE',  ( -3.935609729716867289, 7.813571461303467913, 0.7998128361456352531 ) ) ;
#208809=CARTESIAN_POINT ( 'NONE',  ( -7.255021596644144921, 7.636815748939187465, 0.7216878364870317197 ) ) ;
#208813=CARTESIAN_POINT ( 'NONE',  ( 6.481679955784983349, 9.719654494127929922, -1.199719254218452047 ) ) ;
#208815=CARTESIAN_POINT ( 'NONE',  ( 4.868390568588833567, 4.879779592243221664, -0.3669954890176479467 ) ) ;
#208821=CARTESIAN_POINT ( 'NONE',  ( -4.390861645979385663, 6.216034235099629157, -1.599625672291271394 ) ) ;
#208831=CARTESIAN_POINT ( 'NONE',  ( 4.947799714344386146, 4.737130853015369958, -0.7998128361456481317 ) ) ;
#208847=CARTESIAN_POINT ( 'NONE',  ( -6.947627372360122955, 7.070263120700404968, 0.000000000000000000 ) ) ;
#208849=CARTESIAN_POINT ( 'NONE',  ( -5.000000000000013323, 8.499999999999996447, 0.7750000000000004663 ) ) ;
#208850=CARTESIAN_POINT ( 'NONE',  ( 5.318541398310776103, 9.426991741329731056, -0.7998128361456481317 ) ) ;
#208852=CARTESIAN_POINT ( 'NONE',  ( -6.500216601102190239, 6.758717457939978246, 0.07576745652920421903 ) ) ;
#208858=CARTESIAN_POINT ( 'NONE',  ( 5.554000203453580475, 6.508696987897830688, -1.199719254218452047 ) ) ;
#208866=CARTESIAN_POINT ( 'NONE',  ( 4.475600106286968582, 5.354526557823810151, -1.082531754730548412 ) ) ;
#208870=CARTESIAN_POINT ( 'NONE',  ( 5.180624094197585627, 8.097792972322238825, -1.082531754730548412 ) ) ;
#208877=CARTESIAN_POINT ( 'NONE',  ( -6.328041841479842056, 6.870487382198048998, 0.6860574420480938240 ) ) ;
#208881=CARTESIAN_POINT ( 'NONE',  ( -4.814553946628611136, 8.631080347793099961, 0.000000000000000000 ) ) ;
#208886=CARTESIAN_POINT ( 'NONE',  ( 2.972444473424885381, 6.543659789869906263, -0.5046856791834258837 ) ) ;
#208903=CARTESIAN_POINT ( 'NONE',  ( -5.239262321155076840, 6.291427928779091516, 1.253643227873025179 ) ) ;
#208913=CARTESIAN_POINT ( 'NONE',  ( 3.203469434578891661, 6.959407783642502565, -0.7998128361456362523 ) ) ;
#208917=DIRECTION ( 'NONE',  ( 0.7592566023653005702, -0.6507913734559639396, 0.000000000000000000 ) ) ;
#208924=CARTESIAN_POINT ( 'NONE',  ( -6.211043768836215229, 8.339580045099285854, 1.443375672974064550 ) ) ;
#208926=CARTESIAN_POINT ( 'NONE',  ( 3.404505970362959655, 6.986024375483197879, 0.7216878364870257245 ) ) ;
#208943=ORIENTED_EDGE ( 'NONE', *, *, #77981, .F. ) ;
#208947=CARTESIAN_POINT ( 'NONE',  ( 4.542476715900265916, 4.951051008190067826, -0.8264431066547142102 ) ) ;
#208950=CARTESIAN_POINT ( 'NONE',  ( -6.098824340890369733, 6.672706474115194908, -0.7681833417966426047 ) ) ;
#208979=CARTESIAN_POINT ( 'NONE',  ( -4.586401103172829785, 8.572828063668767484, 0.7998128361456281477 ) ) ;
#208980=CARTESIAN_POINT ( 'NONE',  ( -4.733024909954385073, 8.320217716143888609, 0.7565452571775049817 ) ) ;
#208981=CARTESIAN_POINT ( 'NONE',  ( -6.466312919074983512, 6.508729591867735031, -0.7998128361456361413 ) ) ;
#208988=CARTESIAN_POINT ( 'NONE',  ( -4.462568837553487100, 5.235360394347691404, -1.199719254218453823 ) ) ;
#208991=CARTESIAN_POINT ( 'NONE',  ( -4.980641328173854632, 6.904110530993182948, 1.599625672291263179 ) ) ;
#208999=CARTESIAN_POINT ( 'NONE',  ( -3.062251564868939457, 6.240124004417943127, -0.7724295644362719759 ) ) ;
#209004=CARTESIAN_POINT ( 'NONE',  ( 4.655245641445829641, 6.524482229810530498, 1.599625672291269396 ) ) ;
#209011=CIRCLE ( 'NONE', #105313, 0.08000000000000041800 ) ;
#209027=CARTESIAN_POINT ( 'NONE',  ( 4.960304097753311936, 6.880383762169266504, 1.599625672291268286 ) ) ;
#209028=CARTESIAN_POINT ( 'NONE',  ( 4.980641328173811999, 6.904110530993182948, 1.599625672291269396 ) ) ;
#209030=CARTESIAN_POINT ( 'NONE',  ( 5.076602173674213070, 4.887400388900169368, 0.000000000000000000 ) ) ;
#209038=CARTESIAN_POINT ( 'NONE',  ( -4.123088111887291518, 7.824370207261548416, 0.000000000000000000 ) ) ;
#209042=CARTESIAN_POINT ( 'NONE',  ( 4.774898309648160755, 8.276035162536045320, 0.8191430224755236189 ) ) ;
#209043=CARTESIAN_POINT ( 'NONE',  ( -5.112833325684920993, 6.097965313788082931, -1.082531754730549967 ) ) ;
#209044=CARTESIAN_POINT ( 'NONE',  ( 4.475600106286968582, 5.354526557823810151, -1.082531754730548412 ) ) ;
#209065=ORIENTED_EDGE ( 'NONE', *, *, #177202, .T. ) ;
#209070=CARTESIAN_POINT ( 'NONE',  ( 5.090160327287878594, 4.903218234782778850, -0.7998128361456481317 ) ) ;
#209079=DIRECTION ( 'NONE',  ( 0.6507913734559641616, -0.7592566023653004592, 0.000000000000000000 ) ) ;
#209091=CARTESIAN_POINT ( 'NONE',  ( -7.014364370223741929, 9.276787413384745662, -1.599625672291271394 ) ) ;
#209093=EDGE_LOOP ( 'NONE', ( #67204, #74318, #151234, #143374 ) ) ;
#209106=CARTESIAN_POINT ( 'NONE',  ( 4.736594563127852098, 6.619389305106191834, -1.599625672291273171 ) ) ;
#209119=CARTESIAN_POINT ( 'NONE',  ( 6.003728048595398548, 7.077753126805482076, 1.059392881431284961 ) ) ;
#209123=CIRCLE ( 'NONE', #12001, 4.022469383779238683 ) ;
#209136=AXIS2_PLACEMENT_3D ( 'NONE', #3216, #86629, #153768 ) ;
#209141=CARTESIAN_POINT ( 'NONE',  ( -6.967964602780620353, 7.093989889524320525, 0.000000000000000000 ) ) ;
#209143=CARTESIAN_POINT ( 'NONE',  ( 3.953084306836263995, 6.769626237021087789, 1.199719254218452047 ) ) ;
#209147=CARTESIAN_POINT ( 'NONE',  ( -7.208094944320834863, 8.438474185576302133, -1.199719254218452047 ) ) ;
#209150=CARTESIAN_POINT ( 'NONE',  ( 8.188198428010544205, 8.517596018959260107, 0.000000000000000000 ) ) ;
#209155=CARTESIAN_POINT ( 'NONE',  ( -4.762026763822442277, 8.287006692039220468, -0.8189809589772244491 ) ) ;
#209173=CARTESIAN_POINT ( 'NONE',  ( 4.665414256878284149, 6.536345614481700927, -1.443375672974068769 ) ) ;
#209175=CARTESIAN_POINT ( 'NONE',  ( -7.587723245503481095, 8.881373870289390737, 1.199719254218452047 ) ) ;
#209185=CARTESIAN_POINT ( 'NONE',  ( -3.838578530388868426, 7.492387228696840040, -0.009810069892855370621 ) ) ;
#209186=CARTESIAN_POINT ( 'NONE',  ( -4.841670253855968831, 4.821239182352949904, 0.000000000000000000 ) ) ;
#209190=CARTESIAN_POINT ( 'NONE',  ( 3.874598038455354665, 7.742391154831717692, -0.7998128361456362523 ) ) ;
#209194=DIRECTION ( 'NONE',  ( 0.7592566023653005702, 0.6507913734559639396, 0.000000000000000000 ) ) ;
#209235=ORIENTED_EDGE ( 'NONE', *, *, #135294, .F. ) ;
#209236=CARTESIAN_POINT ( 'NONE',  ( -4.624739795592943459, 6.488892076315448065, -1.443375672974066548 ) ) ;
#209243=CARTESIAN_POINT ( 'NONE',  ( -5.098748287191073203, 8.106234214101666780, 1.199719254218452935 ) ) ;
#209253=CARTESIAN_POINT ( 'NONE',  ( -4.281342646865346602, 8.216926531310035031, 0.7998128361456352531 ) ) ;
#209255=CARTESIAN_POINT ( 'NONE',  ( 6.562153376633583335, 6.794832157118596783, -0.3727171428496069971 ) ) ;
#209260=CARTESIAN_POINT ( 'NONE',  ( 6.690022453700429139, 6.769724048930809701, 0.7998128361456331437 ) ) ;
#209265=CARTESIAN_POINT ( 'NONE',  ( -7.923814432544069142, 8.209148024248356990, 0.000000000000000000 ) ) ;
#209268=ORIENTED_EDGE ( 'NONE', *, *, #77102, .F. ) ;
#209272=CARTESIAN_POINT ( 'NONE',  ( -5.418418667316934112, 6.350518529071726981, -1.199719254218453823 ) ) ;
#209275=CARTESIAN_POINT ( 'NONE',  ( 5.872089928050205465, 6.023395468912922546, -0.7216878364870458196 ) ) ;
#209276=CARTESIAN_POINT ( 'NONE',  ( -5.600926855776888758, 7.627776979863398310, -1.443375672974066548 ) ) ;
#209284=CARTESIAN_POINT ( 'NONE',  ( 4.960304097753311936, 6.880383762169266504, 1.599625672291268286 ) ) ;
#209285=ORIENTED_EDGE ( 'NONE', *, *, #125435, .F. ) ;
#209309=CARTESIAN_POINT ( 'NONE',  ( 3.855102659575539548, 8.506872032340217160, -2.500000000000707878 ) ) ;
#209313=CARTESIAN_POINT ( 'NONE',  ( 5.067666882003905471, 7.850148838107081417, 1.122879199148843377 ) ) ;
#209319=TOROIDAL_SURFACE ( 'NONE', #46709, 0.8299999999999999600, 0.08000000000000000167 ) ;
#209320=CARTESIAN_POINT ( 'NONE',  ( 5.020262018810099924, 9.078999131912302900, 0.7998128361456331437 ) ) ;
#209325=CARTESIAN_POINT ( 'NONE',  ( -4.613315975161869531, 8.372148359400446438, -0.1986654441144524719 ) ) ;
#209332=CARTESIAN_POINT ( 'NONE',  ( -8.093291352714894415, 8.406871097780989288, -0.7998128361456362523 ) ) ;
#209344=CARTESIAN_POINT ( 'NONE',  ( -7.075376061485238566, 9.347967719856493218, 1.599625672291269396 ) ) ;
#209346=CARTESIAN_POINT ( 'NONE',  ( 7.537407054554579489, 7.758339416593960536, 0.000000000000000000 ) ) ;
#209356=CARTESIAN_POINT ( 'NONE',  ( 4.634908411025333130, 6.500755460986618495, 1.599625672291268286 ) ) ;
#209359=CARTESIAN_POINT ( 'NONE',  ( 4.367134876933267407, 8.109091433148536865, 0.000000000000000000 ) ) ;
#209368=CARTESIAN_POINT ( 'NONE',  ( -5.394899524673852476, 7.567224757263017132, 1.245178244268474010 ) ) ;
#209376=CARTESIAN_POINT ( 'NONE',  ( -4.014095998097799267, 6.840806543492835345, -1.199719254218450271 ) ) ;
#209377=CARTESIAN_POINT ( 'NONE',  ( 7.404161286838808920, 8.771181268467660885, -1.082531754730548412 ) ) ;
#209388=CARTESIAN_POINT ( 'NONE',  ( -6.017840079619296567, 8.114175741012878973, -1.599625672291271394 ) ) ;
#209389=CARTESIAN_POINT ( 'NONE',  ( -6.134138155540168391, 6.121192367743780949, 0.000000000000000000 ) ) ;
#209391=CARTESIAN_POINT ( 'NONE',  ( 6.170369307550816806, 9.252495721234380355, 1.082531754730549967 ) ) ;
#209402=CARTESIAN_POINT ( 'NONE',  ( -5.479780979625591186, 7.495630219063617261, -1.250153324542001343 ) ) ;
#209410=CARTESIAN_POINT ( 'NONE',  ( -7.228432174741334038, 8.462200954400218578, -1.199719254218452047 ) ) ;
#209428=CARTESIAN_POINT ( 'NONE',  ( 5.505492895601038938, 8.580769590579979678, -1.199719254218452047 ) ) ;
#209463=CARTESIAN_POINT ( 'NONE',  ( 4.309512724297349884, 6.121127159803966933, 1.599625672291261402 ) ) ;
#209494=CARTESIAN_POINT ( 'NONE',  ( -3.494969737272722643, 7.299491470118629088, -0.7998128361456481317 ) ) ;
#209497=CARTESIAN_POINT ( 'NONE',  ( 4.380693030546905398, 8.124909279031149012, 0.7216878364870247253 ) ) ;
#209502=CARTESIAN_POINT ( 'NONE',  ( -4.118644803501354978, 8.027112380718707030, 0.7998128361456352531 ) ) ;
#209507=CARTESIAN_POINT ( 'NONE',  ( -7.946487431385463651, 8.443525889470736345, 0.7216878364870317197 ) ) ;
#209509=CARTESIAN_POINT ( 'NONE',  ( 5.398914348987485567, 6.259949555863199677, 2.499999999999999556 ) ) ;
#209514=CARTESIAN_POINT ( 'NONE',  ( -4.664887371553763096, 7.600063145858131364, -1.199719254218453823 ) ) ;
#209524=CARTESIAN_POINT ( 'NONE',  ( -4.659162064951642535, 5.464719159645540003, 1.199719254218452935 ) ) ;
#209528=CARTESIAN_POINT ( 'NONE',  ( -6.183927461608886844, 7.347575139032721303, 1.082531754730548412 ) ) ;
#209529=CARTESIAN_POINT ( 'NONE',  ( -6.427974226210522168, 6.671927150099951298, 0.000000000000000000 ) ) ;
#209530=CARTESIAN_POINT ( 'NONE',  ( 6.886615681098613884, 6.999082814228660077, 0.000000000000000000 ) ) ;
#209531=CARTESIAN_POINT ( 'NONE',  ( -7.456058132872594335, 7.663432341298296535, 0.000000000000000000 ) ) ;
#209567=CARTESIAN_POINT ( 'NONE',  ( 4.666526410304530970, 8.402211131567142388, 0.5382107299411863499 ) ) ;
#209582=CARTESIAN_POINT ( 'NONE',  ( 5.176180785367283654, 9.260904359562321275, -0.7998128361456481317 ) ) ;
#209585=CARTESIAN_POINT ( 'NONE',  ( -2.993318053567081360, 6.714231172462041819, 0.000000000000000000 ) ) ;
#209589=CARTESIAN_POINT ( 'NONE',  ( -6.739811759324828344, 8.956476034002674780, -1.443375672974066548 ) ) ;
#209601=CARTESIAN_POINT ( 'NONE',  ( 4.543917759235442944, 5.330267469643351852, 1.199719254218452935 ) ) ;
#209602=CARTESIAN_POINT ( 'NONE',  ( 5.936491157937257235, 8.019268665717216749, 1.599625672291268286 ) ) ;
#209610=ORIENTED_EDGE ( 'NONE', *, *, #178698, .T. ) ;
#209618=CARTESIAN_POINT ( 'NONE',  ( 6.062430963966053632, 7.101866208495718702, -1.199719254218452047 ) ) ;
#209619=VERTEX_POINT ( 'NONE', #171333 ) ;
#209633=CARTESIAN_POINT ( 'NONE',  ( -4.014622883422322985, 7.697827440719083647, -0.7216878364870458196 ) ) ;
#209634=CARTESIAN_POINT ( 'NONE',  ( -6.720001414228860881, 7.869031733802326123, -1.199719254218452047 ) ) ;
#209642=CARTESIAN_POINT ( 'NONE',  ( 6.183927461164522299, 6.387205924212962849, 0.000000000000000000 ) ) ;
#209646=CARTESIAN_POINT ( 'NONE',  ( -3.902768115887413014, 5.646591783325653147, -1.599625672291283607 ) ) ;
#209647=CARTESIAN_POINT ( 'NONE',  ( 5.501576472095266901, 9.640532660744973725, -0.7998128361456481317 ) ) ;
#209650=CARTESIAN_POINT ( 'NONE',  ( 4.543390873910913896, 5.433615786718446472, 1.082531754730549078 ) ) ;
#209668=CARTESIAN_POINT ( 'NONE',  ( 5.899733120602060232, 6.912052057904395141, -1.199719254218452047 ) ) ;
#209673=CARTESIAN_POINT ( 'NONE',  ( 5.845500506147374153, 6.848780674373954547, 1.199719254218453823 ) ) ;
#209684=CARTESIAN_POINT ( 'NONE',  ( 5.994113311017540191, 9.046863725278862844, -1.082531754730548412 ) ) ;
#209686=CARTESIAN_POINT ( 'NONE',  ( -5.420227550413282636, 9.545625585449309725, 0.7998128361456291469 ) ) ;
#209687=CARTESIAN_POINT ( 'NONE',  ( 4.634908411025333130, 6.500755460986618495, 1.599625672291268286 ) ) ;
#209688=EDGE_LOOP ( 'NONE', ( #102227, #72173, #30328, #172142, #21807 ) ) ;
#209697=CARTESIAN_POINT ( 'NONE',  ( -3.461074353238556167, 7.259946855412102273, 0.000000000000000000 ) ) ;
#209733=CARTESIAN_POINT ( 'NONE',  ( 5.826972158823246595, 10.02016096192762085, -0.7998128361456481317 ) ) ;
#209739=ADVANCED_FACE ( 'NONE', ( #58659 ), #73842, .F. ) ;
#209745=CARTESIAN_POINT ( 'NONE',  ( -4.145761110728687804, 8.058748072483927771, -0.7998128361456481317 ) ) ;
#209747=CARTESIAN_POINT ( 'NONE',  ( -7.533490631048818109, 8.818102486758951031, -1.199719254218452047 ) ) ;
#209757=CARTESIAN_POINT ( 'NONE',  ( -2.428612866367529932E-14, 8.920000000000001705, 2.420000000000000373 ) ) ;
#209758=CARTESIAN_POINT ( 'NONE',  ( -5.101610940492132151, 9.173906207207963348, -0.7998128361456362523 ) ) ;
#209765=CARTESIAN_POINT ( 'NONE',  ( -4.123088112331656951, 6.864000993478624579, 1.082531754730549967 ) ) ;
#209770=CARTESIAN_POINT ( 'NONE',  ( -4.176793841461789114, 7.030620694084159794, -1.199719254218455378 ) ) ;
#209791=CARTESIAN_POINT ( 'NONE',  ( -6.526270840131767059, 8.707344961610770540, -1.599625672291271394 ) ) ;
#209794=CARTESIAN_POINT ( 'NONE',  ( -5.167592825464113915, 6.057888380243431570, 1.199719254218452935 ) ) ;
#209806=ORIENTED_EDGE ( 'NONE', *, *, #161304, .F. ) ;
#209819=CARTESIAN_POINT ( 'NONE',  ( -5.986807348886189040, 9.142303119412650503, -1.199719254218452047 ) ) ;
#209821=ORIENTED_EDGE ( 'NONE', *, *, #140883, .T. ) ;
#209842=CARTESIAN_POINT ( 'NONE',  ( 6.016786309414542622, 10.24161080428416426, 0.7998128361456341429 ) ) ;
#209844=CARTESIAN_POINT ( 'NONE',  ( 7.530627977747744062, 7.750430493652658015, -0.7998128361456341429 ) ) ;
#209857=CARTESIAN_POINT ( 'NONE',  ( 5.309622429108474151, 7.625948988765205883, 1.230663689527239812 ) ) ;
#209859=CARTESIAN_POINT ( 'NONE',  ( 5.207740401424913124, 9.089797878388800711, -0.7216878364870458196 ) ) ;
#209866=CARTESIAN_POINT ( 'NONE',  ( -5.822300622425855110, 5.757381912443740646, 0.7998128361456281477 ) ) ;
#209873=CARTESIAN_POINT ( 'NONE',  ( -6.577113915960841162, 7.806292669110006521, -1.082531754730549967 ) ) ;
#209877=CARTESIAN_POINT ( 'NONE',  ( -4.989511253089500720, 4.785794314884651790, -0.3387278650471270969 ) ) ;
#209878=CARTESIAN_POINT ( 'NONE',  ( -5.426654608689173820, 6.244223002735716399, -0.9996599858201720146 ) ) ;
#209883=CARTESIAN_POINT ( 'NONE',  ( -4.442231607132987925, 5.211633625523774960, -1.199719254218453823 ) ) ;
#209893=CARTESIAN_POINT ( 'NONE',  ( 5.508355548902068577, 9.648441583686274470, 0.7998128361456331437 ) ) ;
#209905=( BOUNDED_SURFACE ( )  B_SPLINE_SURFACE ( 1, 2, ( 
 ( #5811, #187786, #71887, #39415, #192045, #24207, #173716, #59929, #90310, #122903, #109826, #156381, #123960, #155304, #6886, #206170, #77242, #27428, #171542, #158507, #140146, #41573, #106603, #188861, #56735, #142287, #7963, #57800, #40499, #175837, #92469, #190980, #44778, #23135, #75122, #172631, #207241, #189928, #42644, #141231, #139069, #74054, #193129, #26353, #108754, #72964, #174778, #143359, #107687, #208298, #43708, #205094, #58865, #89252, #25292, #76180, #9047, #209356, #10107, #91392, #61002, #157453, #125022, #126084, #93526, #159568, #11165, #127158, #63139, #95668, #131394, #177965, #147599, #46910, #197391, #129301, #45843, #163852, #113027, #162786, #47986, #110884, #62077, #179034, #213617, #30652, #111962, #195277, #146553, #212573, #96738, #64211, #14364, #98849, #145504, #29578, #15432, #115153, #161720, #181148, #13312, #194197, #144434, #79385, #128234, #211502, #80455, #148661, #130352, #180093, #164900, #196343, #114102, #31717, #176890, #94593, #97792, #81521, #65243, #160635, #132449, #49033, #32770, #16493, #82574, #228, #66300, #198447, #28503, #12236, #78310, #210436, #41044, #167044, #35960, #23693, #56209, #89803, #73515, #184336, #156924, #8513, #102038, #151865, #1304, #6367, #100954, #117279, #139617, #118349, #205640, #168107, #106077, #74594, #19706, #140698, #122373, #99908, #90860, #50093, #133508, #72436, #85785, #18636, #188330, #138537, #116215, #165968, #24758, #17553, #83639, #84716, #172100, #204561, #182202, #39970, #150803, #155847, #7434, #57279, #149726, #2367, #200574, #123440, #68444, #189402, #173178, #107153, #33829, #67364, #34881, #51157, #199512, #183277, #134573, #52220, #124496, #125556, #75658, #209893, #25823, #92995, #178491, #58340, #46362, #61531, #30101, #79903, #127697, #112482, #45300, #177423, #206712, #190455, #142824, #42114, #160102, #193657, #27968, #26891, #62587, #162242, #108226, #94062, #78833, #111419, #174251, #144954, #141765, #59400, #96191, #191517, #13828, #43182, #159039, #110357, #29041, #95124, #77779, #9582, #210960 ),
 ( #11705, #208831, #143900, #60461, #194723, #10632, #109295, #161173, #128750, #175304, #91933, #76708, #207773, #157993, #126618, #192581, #12759, #44236, #176361, #51694, #131904, #115666, #113553, #130862, #147069, #181660, #67890, #752, #80980, #63665, #64720, #14885, #149175, #179556, #32231, #117816, #212022, #200043, #66818, #183806, #19164, #132961, #35416, #198964, #116733, #146011, #129819, #82034, #195801, #99371, #50608, #33287, #180606, #1831, #101494, #47438, #165423, #18086, #182732, #31177, #84174, #213090, #196858, #167564, #48496, #97250, #114615, #98302, #49540, #34351, #100424, #17020, #163304, #150263, #164367, #15951, #83096, #197912, #148128, #214129, #166495, #134035, #65757, #6105, #22353, #123190, #152384, #55954, #122107, #53821, #71103, #3962, #188072, #137221, #37562, #203241, #39701, #88465, #105810, #171836, #5028, #189151, #40790, #54885, #187006, #36487, #38637, #136145, #70030, #23429, #153455, #89540, #121039, #138283, #106895, #104716, #172921, #154525, #135086, #85238, #151326, #168624, #170764, #72175, #119951, #204298, #155591, #2894, #201100, #57023, #52740, #118874, #202163, #7176, #73247, #68967, #139354, #185926, #205384, #184860, #102564, #20227, #86312, #103642, #169694, #21282, #87388, #76463, #62354, #11458, #157738, #210728, #25574, #142572, #193420, #111175, #92747, #59148, #128515, #191264, #9335, #45064, #91685, #61288, #175059, #177176, #42930, #174003, #77531, #26646, #208579, #176120, #24497, #190205, #158791, #127449, #10388, #75408, #109040, #60212, #126373, #192332, #43991, #110109, #12523, #125306, #141521, #143652, #28793, #207529, #94877, #27720, #107974, #58085, #93814, #41865, #159855, #209647, #194483, #160929, #78596, #144716, #46126, #112243, #90608, #156667, #8259, #74343, #140447, #206458, #124247, #199794, #48262, #195563, #197670, #179320, #166244, #116490, #98076, #95950, #31995, #163070, #47199, #17834, #80745, #180371, #66574, #30941, #129576, #182479, #14651, #130631, #162005, #13594, #212852, #83917, #34107, #178254, #165179, #146833, #114376 ) ),
 .UNSPECIFIED., .F., .F., .T. ) 
 B_SPLINE_SURFACE_WITH_KNOTS ( ( 2, 2 ),
 ( 3, 2, 2, 2, 2, 2, 2, 2, 2, 2, 2, 2, 2, 2, 2, 2, 2, 2, 2, 2, 2, 2, 2, 2, 2, 2, 2, 2, 2, 2, 2, 2, 2, 2, 2, 2, 2, 2, 2, 2, 2, 2, 2, 2, 2, 2, 2, 2, 2, 2, 2, 2, 2, 2, 2, 2, 2, 2, 2, 2, 2, 2, 2, 2, 2, 2, 2, 2, 2, 2, 2, 2, 2, 2, 2, 2, 2, 2, 2, 2, 2, 2, 2, 2, 2, 2, 2, 2, 2, 2, 2, 2, 2, 2, 2, 2, 2, 2, 2, 2, 2, 2, 2, 2, 2, 2, 2, 2, 2, 2, 2, 2, 2, 2, 2, 2, 2, 2, 2, 2, 3 ),
 ( 0.000000000000000000, 1.000000000000000000 ),
 ( 0.000000000000000000, 0.008333333333333333218, 0.01666666666666666644, 0.02500000000000000139, 0.03333333333333333287, 0.04166666666666666435, 0.05000000000000000278, 0.05833333333333333426, 0.06666666666666666574, 0.07499999999999999722, 0.08333333333333332871, 0.09166666666666666019, 0.1000000000000000056, 0.1083333333333333370, 0.1166666666666666685, 0.1250000000000000000, 0.1333333333333333315, 0.1416666666666666630, 0.1499999999999999944, 0.1583333333333333259, 0.1666666666666666574, 0.1749999999999999889, 0.1833333333333333204, 0.1916666666666666796, 0.2000000000000000111, 0.2083333333333333426, 0.2166666666666666741, 0.2250000000000000056, 0.2333333333333333370, 0.2416666666666666685, 0.2500000000000000000, 0.2583333333333333592, 0.2666666666666666630, 0.2750000000000000222, 0.2833333333333333259, 0.2916666666666666852, 0.2999999999999999889, 0.3083333333333333481, 0.3166666666666666519, 0.3250000000000000111, 0.3333333333333333148, 0.3416666666666666741, 0.3499999999999999778, 0.3583333333333333370, 0.3666666666666666408, 0.3750000000000000000, 0.3833333333333333592, 0.3916666666666666630, 0.4000000000000000222, 0.4083333333333333259, 0.4166666666666666852, 0.4249999999999999889, 0.4333333333333333481, 0.4416666666666666519, 0.4500000000000000111, 0.4583333333333333148, 0.4666666666666666741, 0.4749999999999999778, 0.4833333333333333370, 0.4916666666666666408, 0.5000000000000000000, 0.5083333333333333037, 0.5166666666666667185, 0.5250000000000000222, 0.5333333333333333259, 0.5416666666666666297, 0.5500000000000000444, 0.5583333333333333481, 0.5666666666666666519, 0.5749999999999999556, 0.5833333333333333703, 0.5916666666666666741, 0.5999999999999999778, 0.6083333333333332815, 0.6166666666666666963, 0.6250000000000000000, 0.6333333333333333037, 0.6416666666666667185, 0.6500000000000000222, 0.6583333333333333259, 0.6666666666666666297, 0.6750000000000000444, 0.6833333333333333481, 0.6916666666666666519, 0.6999999999999999556, 0.7083333333333333703, 0.7166666666666666741, 0.7249999999999999778, 0.7333333333333332815, 0.7416666666666666963, 0.7500000000000000000, 0.7583333333333333037, 0.7666666666666667185, 0.7750000000000000222, 0.7833333333333333259, 0.7916666666666666297, 0.8000000000000000444, 0.8083333333333333481, 0.8166666666666666519, 0.8249999999999999556, 0.8333333333333333703, 0.8416666666666666741, 0.8499999999999999778, 0.8583333333333332815, 0.8666666666666666963, 0.8750000000000000000, 0.8833333333333333037, 0.8916666666666667185, 0.9000000000000000222, 0.9083333333333333259, 0.9166666666666666297, 0.9250000000000000444, 0.9333333333333333481, 0.9416666666666666519, 0.9499999999999999556, 0.9583333333333333703, 0.9666666666666666741, 0.9749999999999999778, 0.9833333333333332815, 0.9916666666666666963, 1.000000000000000000 ),
 .UNSPECIFIED. ) 
 GEOMETRIC_REPRESENTATION_ITEM ( )  RATIONAL_B_SPLINE_SURFACE ( (
 ( 1.000000000000000000, 0.8660254037844387076, 1.000000000000000000, 0.8660254037844387076, 1.000000000000000000, 0.8660254037844387076, 1.000000000000000000, 0.8660254037844387076, 1.000000000000000000, 0.8660254037844387076, 1.000000000000000000, 0.8660254037844387076, 1.000000000000000000, 0.8660254037844387076, 1.000000000000000000, 0.8660254037844387076, 1.000000000000000000, 0.8660254037844387076, 1.000000000000000000, 0.8660254037844387076, 1.000000000000000000, 0.8660254037844387076, 1.000000000000000000, 0.8660254037844387076, 1.000000000000000000, 0.8660254037844387076, 1.000000000000000000, 0.8660254037844387076, 1.000000000000000000, 0.8660254037844387076, 1.000000000000000000, 0.8660254037844387076, 1.000000000000000000, 0.8660254037844387076, 1.000000000000000000, 0.8660254037844387076, 1.000000000000000000, 0.8660254037844387076, 1.000000000000000000, 0.8660254037844387076, 1.000000000000000000, 0.8660254037844387076, 1.000000000000000000, 0.8660254037844387076, 1.000000000000000000, 0.8660254037844387076, 1.000000000000000000, 0.8660254037844387076, 1.000000000000000000, 0.8660254037844387076, 1.000000000000000000, 0.8660254037844387076, 1.000000000000000000, 0.8660254037844387076, 1.000000000000000000, 0.8660254037844387076, 1.000000000000000000, 0.8660254037844387076, 1.000000000000000000, 0.8660254037844387076, 1.000000000000000000, 0.8660254037844387076, 1.000000000000000000, 0.8660254037844387076, 1.000000000000000000, 0.8660254037844387076, 1.000000000000000000, 0.8660254037844387076, 1.000000000000000000, 0.8660254037844387076, 1.000000000000000000, 0.8660254037844387076, 1.000000000000000000, 0.8660254037844387076, 1.000000000000000000, 0.8660254037844387076, 1.000000000000000000, 0.8660254037844387076, 1.000000000000000000, 0.8660254037844387076, 1.000000000000000000, 0.8660254037844387076, 1.000000000000000000, 0.8660254037844387076, 1.000000000000000000, 0.8660254037844387076, 1.000000000000000000, 0.8660254037844387076, 1.000000000000000000, 0.8660254037844387076, 1.000000000000000000, 0.8660254037844387076, 1.000000000000000000, 0.8660254037844387076, 1.000000000000000000, 0.8660254037844387076, 1.000000000000000000, 0.8660254037844387076, 1.000000000000000000, 0.8660254037844387076, 1.000000000000000000, 0.8660254037844387076, 1.000000000000000000, 0.8660254037844387076, 1.000000000000000000, 0.8660254037844387076, 1.000000000000000000, 0.8660254037844387076, 1.000000000000000000, 0.8660254037844387076, 1.000000000000000000, 0.8660254037844387076, 1.000000000000000000, 0.8660254037844387076, 1.000000000000000000, 0.8660254037844387076, 1.000000000000000000, 0.8660254037844387076, 1.000000000000000000, 0.8660254037844387076, 1.000000000000000000, 0.8660254037844387076, 1.000000000000000000, 0.8660254037844387076, 1.000000000000000000, 0.8660254037844387076, 1.000000000000000000, 0.8660254037844387076, 1.000000000000000000, 0.8660254037844387076, 1.000000000000000000, 0.8660254037844387076, 1.000000000000000000, 0.8660254037844387076, 1.000000000000000000, 0.8660254037844387076, 1.000000000000000000, 0.8660254037844387076, 1.000000000000000000, 0.8660254037844387076, 1.000000000000000000, 0.8660254037844387076, 1.000000000000000000, 0.8660254037844387076, 1.000000000000000000, 0.8660254037844387076, 1.000000000000000000, 0.8660254037844387076, 1.000000000000000000, 0.8660254037844387076, 1.000000000000000000, 0.8660254037844387076, 1.000000000000000000, 0.8660254037844387076, 1.000000000000000000, 0.8660254037844387076, 1.000000000000000000, 0.8660254037844387076, 1.000000000000000000, 0.8660254037844387076, 1.000000000000000000, 0.8660254037844387076, 1.000000000000000000, 0.8660254037844387076, 1.000000000000000000, 0.8660254037844387076, 1.000000000000000000, 0.8660254037844387076, 1.000000000000000000, 0.8660254037844387076, 1.000000000000000000, 0.8660254037844387076, 1.000000000000000000, 0.8660254037844387076, 1.000000000000000000, 0.8660254037844387076, 1.000000000000000000, 0.8660254037844387076, 1.000000000000000000, 0.8660254037844387076, 1.000000000000000000, 0.8660254037844387076, 1.000000000000000000, 0.8660254037844387076, 1.000000000000000000, 0.8660254037844387076, 1.000000000000000000, 0.8660254037844387076, 1.000000000000000000, 0.8660254037844387076, 1.000000000000000000, 0.8660254037844387076, 1.000000000000000000, 0.8660254037844387076, 1.000000000000000000, 0.8660254037844387076, 1.000000000000000000, 0.8660254037844387076, 1.000000000000000000, 0.8660254037844387076, 1.000000000000000000, 0.8660254037844387076, 1.000000000000000000, 0.8660254037844387076, 1.000000000000000000, 0.8660254037844387076, 1.000000000000000000, 0.8660254037844387076, 1.000000000000000000, 0.8660254037844387076, 1.000000000000000000, 0.8660254037844387076, 1.000000000000000000, 0.8660254037844387076, 1.000000000000000000, 0.8660254037844387076, 1.000000000000000000, 0.8660254037844387076, 1.000000000000000000, 0.8660254037844387076, 1.000000000000000000, 0.8660254037844387076, 1.000000000000000000, 0.8660254037844387076, 1.000000000000000000, 0.8660254037844387076, 1.000000000000000000, 0.8660254037844387076, 1.000000000000000000, 0.8660254037844387076, 1.000000000000000000, 0.8660254037844387076, 1.000000000000000000, 0.8660254037844387076, 1.000000000000000000, 0.8660254037844387076, 1.000000000000000000, 0.8660254037844387076, 1.000000000000000000, 0.8660254037844387076, 1.000000000000000000),
 ( 1.000000000000000000, 0.8660254037844387076, 1.000000000000000000, 0.8660254037844387076, 1.000000000000000000, 0.8660254037844387076, 1.000000000000000000, 0.8660254037844387076, 1.000000000000000000, 0.8660254037844387076, 1.000000000000000000, 0.8660254037844387076, 1.000000000000000000, 0.8660254037844387076, 1.000000000000000000, 0.8660254037844387076, 1.000000000000000000, 0.8660254037844387076, 1.000000000000000000, 0.8660254037844387076, 1.000000000000000000, 0.8660254037844387076, 1.000000000000000000, 0.8660254037844387076, 1.000000000000000000, 0.8660254037844387076, 1.000000000000000000, 0.8660254037844387076, 1.000000000000000000, 0.8660254037844387076, 1.000000000000000000, 0.8660254037844387076, 1.000000000000000000, 0.8660254037844387076, 1.000000000000000000, 0.8660254037844387076, 1.000000000000000000, 0.8660254037844387076, 1.000000000000000000, 0.8660254037844387076, 1.000000000000000000, 0.8660254037844387076, 1.000000000000000000, 0.8660254037844387076, 1.000000000000000000, 0.8660254037844387076, 1.000000000000000000, 0.8660254037844387076, 1.000000000000000000, 0.8660254037844387076, 1.000000000000000000, 0.8660254037844387076, 1.000000000000000000, 0.8660254037844387076, 1.000000000000000000, 0.8660254037844387076, 1.000000000000000000, 0.8660254037844387076, 1.000000000000000000, 0.8660254037844387076, 1.000000000000000000, 0.8660254037844387076, 1.000000000000000000, 0.8660254037844387076, 1.000000000000000000, 0.8660254037844387076, 1.000000000000000000, 0.8660254037844387076, 1.000000000000000000, 0.8660254037844387076, 1.000000000000000000, 0.8660254037844387076, 1.000000000000000000, 0.8660254037844387076, 1.000000000000000000, 0.8660254037844387076, 1.000000000000000000, 0.8660254037844387076, 1.000000000000000000, 0.8660254037844387076, 1.000000000000000000, 0.8660254037844387076, 1.000000000000000000, 0.8660254037844387076, 1.000000000000000000, 0.8660254037844387076, 1.000000000000000000, 0.8660254037844387076, 1.000000000000000000, 0.8660254037844387076, 1.000000000000000000, 0.8660254037844387076, 1.000000000000000000, 0.8660254037844387076, 1.000000000000000000, 0.8660254037844387076, 1.000000000000000000, 0.8660254037844387076, 1.000000000000000000, 0.8660254037844387076, 1.000000000000000000, 0.8660254037844387076, 1.000000000000000000, 0.8660254037844387076, 1.000000000000000000, 0.8660254037844387076, 1.000000000000000000, 0.8660254037844387076, 1.000000000000000000, 0.8660254037844387076, 1.000000000000000000, 0.8660254037844387076, 1.000000000000000000, 0.8660254037844387076, 1.000000000000000000, 0.8660254037844387076, 1.000000000000000000, 0.8660254037844387076, 1.000000000000000000, 0.8660254037844387076, 1.000000000000000000, 0.8660254037844387076, 1.000000000000000000, 0.8660254037844387076, 1.000000000000000000, 0.8660254037844387076, 1.000000000000000000, 0.8660254037844387076, 1.000000000000000000, 0.8660254037844387076, 1.000000000000000000, 0.8660254037844387076, 1.000000000000000000, 0.8660254037844387076, 1.000000000000000000, 0.8660254037844387076, 1.000000000000000000, 0.8660254037844387076, 1.000000000000000000, 0.8660254037844387076, 1.000000000000000000, 0.8660254037844387076, 1.000000000000000000, 0.8660254037844387076, 1.000000000000000000, 0.8660254037844387076, 1.000000000000000000, 0.8660254037844387076, 1.000000000000000000, 0.8660254037844387076, 1.000000000000000000, 0.8660254037844387076, 1.000000000000000000, 0.8660254037844387076, 1.000000000000000000, 0.8660254037844387076, 1.000000000000000000, 0.8660254037844387076, 1.000000000000000000, 0.8660254037844387076, 1.000000000000000000, 0.8660254037844387076, 1.000000000000000000, 0.8660254037844387076, 1.000000000000000000, 0.8660254037844387076, 1.000000000000000000, 0.8660254037844387076, 1.000000000000000000, 0.8660254037844387076, 1.000000000000000000, 0.8660254037844387076, 1.000000000000000000, 0.8660254037844387076, 1.000000000000000000, 0.8660254037844387076, 1.000000000000000000, 0.8660254037844387076, 1.000000000000000000, 0.8660254037844387076, 1.000000000000000000, 0.8660254037844387076, 1.000000000000000000, 0.8660254037844387076, 1.000000000000000000, 0.8660254037844387076, 1.000000000000000000, 0.8660254037844387076, 1.000000000000000000, 0.8660254037844387076, 1.000000000000000000, 0.8660254037844387076, 1.000000000000000000, 0.8660254037844387076, 1.000000000000000000, 0.8660254037844387076, 1.000000000000000000, 0.8660254037844387076, 1.000000000000000000, 0.8660254037844387076, 1.000000000000000000, 0.8660254037844387076, 1.000000000000000000, 0.8660254037844387076, 1.000000000000000000, 0.8660254037844387076, 1.000000000000000000, 0.8660254037844387076, 1.000000000000000000, 0.8660254037844387076, 1.000000000000000000, 0.8660254037844387076, 1.000000000000000000, 0.8660254037844387076, 1.000000000000000000, 0.8660254037844387076, 1.000000000000000000, 0.8660254037844387076, 1.000000000000000000, 0.8660254037844387076, 1.000000000000000000, 0.8660254037844387076, 1.000000000000000000, 0.8660254037844387076, 1.000000000000000000, 0.8660254037844387076, 1.000000000000000000, 0.8660254037844387076, 1.000000000000000000, 0.8660254037844387076, 1.000000000000000000, 0.8660254037844387076, 1.000000000000000000, 0.8660254037844387076, 1.000000000000000000, 0.8660254037844387076, 1.000000000000000000, 0.8660254037844387076, 1.000000000000000000, 0.8660254037844387076, 1.000000000000000000) ) ) 
 REPRESENTATION_ITEM ( '' )  SURFACE ( )  );
#209907=DIRECTION ( 'NONE',  ( -1.000000000000000000, 0.000000000000000000, 0.000000000000000000 ) ) ;
#209913=DIRECTION ( 'NONE',  ( -0.000000000000000000, 1.000000000000000000, -0.000000000000000000 ) ) ;
#209916=CARTESIAN_POINT ( 'NONE',  ( 5.342795052237045539, 8.390955439988655229, -1.199719254218450271 ) ) ;
#209918=CARTESIAN_POINT ( 'NONE',  ( -5.896403733238388511, 7.170697087194168873, 1.136063563240964802 ) ) ;
#209924=CARTESIAN_POINT ( 'NONE',  ( 6.042093733545556233, 7.078139439671806699, -1.199719254218452047 ) ) ;
#209927=DIRECTION ( 'NONE',  ( 0.000000000000000000, -1.000000000000000000, 0.000000000000000000 ) ) ;
#209936=CARTESIAN_POINT ( 'NONE',  ( 6.102578539926878598, 7.252668063737060855, -1.082531754730548412 ) ) ;
#209946=CARTESIAN_POINT ( 'NONE',  ( -4.150204419558982671, 7.856005899545188242, 0.7216878364870338292 ) ) ;
#209977=CARTESIAN_POINT ( 'NONE',  ( 4.030516805012513082, 7.924296382481737844, 0.000000000000000000 ) ) ;
#209983=EDGE_CURVE ( 'NONE', #38200, #69383, #195260, .T. ) ;
#209991=CARTESIAN_POINT ( 'NONE',  ( -5.804299160426224624, 9.785783097223662352, -0.7216878364870338292 ) ) ;
#209994=CARTESIAN_POINT ( 'NONE',  ( 7.635176783151273128, 8.936736330878529699, 1.199719254218452935 ) ) ;
#210003=EDGE_CURVE ( 'NONE', #123093, #136751, #210333, .T. ) ;
#210015=CARTESIAN_POINT ( 'NONE',  ( -5.602498012743507338, 5.726462300312828546, -0.1687859242097844992 ) ) ;
#210025=CONICAL_SURFACE ( 'NONE', #116712, 1249.999999999991587, 0.8960553845713407073 ) ;
#210032=ADVANCED_FACE ( 'NONE', ( #160425 ), #111745, .T. ) ;
#210047=CARTESIAN_POINT ( 'NONE',  ( -5.646044625448194410, 5.551749915969804938, 0.000000000000000000 ) ) ;
#210050=CARTESIAN_POINT ( 'NONE',  ( -7.910256278930404505, 8.193330178365746619, -0.7998128361456362523 ) ) ;
#210051=CARTESIAN_POINT ( 'NONE',  ( -4.709679585977568195, 8.347295923589904021, 0.7007048023343342980 ) ) ;
#210052=CARTESIAN_POINT ( 'NONE',  ( -4.847922445338252118, 7.813604065273374921, -1.199719254218453823 ) ) ;
#210053=CARTESIAN_POINT ( 'NONE',  ( -5.851773230888425381, 7.216290455326334730, 1.198155855505623535 ) ) ;
#210057=CARTESIAN_POINT ( 'NONE',  ( -5.346851039111045978, 6.199209027673978412, -1.060622344683157747 ) ) ;
#210059=CARTESIAN_POINT ( 'NONE',  ( -5.178288325776719603, 5.006034233019745372, 0.000000000000000000 ) ) ;
#210062=CARTESIAN_POINT ( 'NONE',  ( -5.829079699232685208, 5.765290835385048496, 0.000000000000000000 ) ) ;
#210076=CARTESIAN_POINT ( 'NONE',  ( 6.086684617892325733, 6.065829907154645539, -0.7998128361456481317 ) ) ;
#210099=CARTESIAN_POINT ( 'NONE',  ( 5.529746549527311039, 7.544733289238903851, -1.599625672291281386 ) ) ;
#210100=CARTESIAN_POINT ( 'NONE',  ( 3.413620815590684199, 7.204584394822967752, 0.7998128361456281477 ) ) ;
#210102=CARTESIAN_POINT ( 'NONE',  ( 5.388439706788500594, 5.251210844200210559, 0.7998128361456352531 ) ) ;
#210112=EDGE_LOOP ( 'NONE', ( #179215, #171432 ) ) ;
#210115=CARTESIAN_POINT ( 'NONE',  ( 4.666526410304530970, 8.402211131567142388, 0.5382107299411863499 ) ) ;
#210116=CARTESIAN_POINT ( 'NONE',  ( -5.031484404002922517, 6.963427452793760963, 1.443375672974058777 ) ) ;
#210117=CARTESIAN_POINT ( 'NONE',  ( -2.985343197443135033, 6.427599869489915463, 0.3821323783160038290 ) ) ;
#210142=CARTESIAN_POINT ( 'NONE',  ( 5.011674058906918638, 5.875983152593414971, 1.199719254218452047 ) ) ;
#210156=ADVANCED_BREP_SHAPE_REPRESENTATION ( '', ( #23845, #200407 ), #193485 ) ;
#210162=CARTESIAN_POINT ( 'NONE',  ( -7.065734331377342414, 8.272386803808890576, -1.199719254218452047 ) ) ;
#210167=EDGE_CURVE ( 'NONE', #92970, #758, #172317, .T. ) ;
#210174=CARTESIAN_POINT ( 'NONE',  ( 5.006703865196457492, 9.063181286029688977, 0.000000000000000000 ) ) ;
#210180=CARTESIAN_POINT ( 'NONE',  ( 5.200434439293556643, 8.224868058221247225, -1.199719254218452047 ) ) ;
#210191=CARTESIAN_POINT ( 'NONE',  ( -4.123088111887291518, 7.824370207261548416, 0.000000000000000000 ) ) ;
#210194=CARTESIAN_POINT ( 'NONE',  ( 4.596293493935747598, 8.372084169494645067, 0.08663659024946840370 ) ) ;
#210207=DIRECTION ( 'NONE',  ( 0.000000000000000000, 1.000000000000000000, 0.000000000000000000 ) ) ;
#210208=FACE_OUTER_BOUND ( 'NONE', #117817, .T. ) ;
#210213=CARTESIAN_POINT ( 'NONE',  ( -5.444481204339554736, 8.509589284108232121, 1.199719254218454489 ) ) ;
#210215=CARTESIAN_POINT ( 'NONE',  ( 6.886615681098613884, 6.999082814228660077, 0.000000000000000000 ) ) ;
#210219=CARTESIAN_POINT ( 'NONE',  ( -6.454563648557663846, 9.688018802362710957, -1.199719254218452047 ) ) ;
#210227=CARTESIAN_POINT ( 'NONE',  ( -5.492869780704572769, 7.580512000422499952, -1.348893862496753249 ) ) ;
#210245=CARTESIAN_POINT ( 'NONE',  ( 4.421367491832258523, 8.172362817197399210, 0.7216878364870257245 ) ) ;
#210255=CYLINDRICAL_SURFACE ( 'NONE', #86180, 1.250000000000000000 ) ;
#210261=CARTESIAN_POINT ( 'NONE',  ( -4.394251184604987870, 5.259619482528146150, 1.082531754730549078 ) ) ;
#210265=CARTESIAN_POINT ( 'NONE',  ( 5.682802662783380754, 6.658966523782627434, 1.199719254218452935 ) ) ;
#210268=CARTESIAN_POINT ( 'NONE',  ( -7.065207446497166366, 9.336104335703744539, 0.000000000000000000 ) ) ;
#210280=CARTESIAN_POINT ( 'NONE',  ( 3.188928480291387313, 8.980740528189222971, 2.451733079074398969 ) ) ;
#210288=CARTESIAN_POINT ( 'NONE',  ( 5.594708818112484217, 5.774250729507366842, 0.6894988139244704328 ) ) ;
#210318=CARTESIAN_POINT ( 'NONE',  ( -4.462041952228954500, 6.299077925724123617, -1.443375672974066548 ) ) ;
#210324=CARTESIAN_POINT ( 'NONE',  ( -4.776215253764153346, 8.794277906025310898, -0.7998128361456362523 ) ) ;
#210333=CIRCLE ( 'NONE', #85720, 0.7500000000000006661 ) ;
#210334=CARTESIAN_POINT ( 'NONE',  ( -4.305596300791617814, 7.180890229968955651, 1.199719254218452935 ) ) ;
#210336=CARTESIAN_POINT ( 'NONE',  ( 6.296370465541430761, 6.973533528358998979, 0.9269300130883666444 ) ) ;
#210341=CARTESIAN_POINT ( 'NONE',  ( 6.527324610336440180, 6.579909898339485252, 0.7998128361456331437 ) ) ;
#210347=CARTESIAN_POINT ( 'NONE',  ( -3.383641855062333281, 6.105276709951447778, -1.199719254218452047 ) ) ;
#210354=CARTESIAN_POINT ( 'NONE',  ( -4.423703259808839938, 8.383013913077441259, 0.7998128361456352531 ) ) ;
#210358=CARTESIAN_POINT ( 'NONE',  ( 5.926322542504858681, 8.007405281046052536, -1.443375672974078761 ) ) ;
#210359=CARTESIAN_POINT ( 'NONE',  ( -5.112833325684908559, 8.018703742390766109, -1.082531754730549967 ) ) ;
#210363=CARTESIAN_POINT ( 'NONE',  ( -6.445975688654486113, 6.485002823043818587, -0.7998128361456361413 ) ) ;
#210366=CARTESIAN_POINT ( 'NONE',  ( 3.867818961648523235, 7.734482231890414283, 1.040834085586084257E-14 ) ) ;
#210372=( LENGTH_UNIT ( ) NAMED_UNIT ( * ) SI_UNIT ( .MILLI., .METRE. ) );
#210396=CARTESIAN_POINT ( 'NONE',  ( 4.802738015080052492, 8.126035781178083894, 0.8349615142884360131 ) ) ;
#210404=CARTESIAN_POINT ( 'NONE',  ( 5.885121196783658526, 9.023669275293071834, 1.199719254218452047 ) ) ;
#210409=CARTESIAN_POINT ( 'NONE',  ( -4.896236220255085314, 8.042264628280536343, 0.9566786516278618091 ) ) ;
#210416=CARTESIAN_POINT ( 'NONE',  ( -3.309598895067336510, 6.875299454304925284, 0.000000000000000000 ) ) ;
#210426=CARTESIAN_POINT ( 'NONE',  ( -3.383641855062333281, 6.105276709951447778, -1.199719254218452047 ) ) ;
#210436=CARTESIAN_POINT ( 'NONE',  ( 6.690022453700429139, 6.769724048930809701, 0.7998128361456331437 ) ) ;
#210439=CARTESIAN_POINT ( 'NONE',  ( 5.682275777458846377, 7.722684055159064975, 1.443375672974064550 ) ) ;
#210449=CARTESIAN_POINT ( 'NONE',  ( -6.457230086593013674, 6.786253674495239530, 0.3580049749655131452 ) ) ;
#210456=CARTESIAN_POINT ( 'NONE',  ( -3.149236820124241110, 6.896136400112061970, -0.7998128361456481317 ) ) ;
#210457=CARTESIAN_POINT ( 'NONE',  ( 4.740510986633625024, 5.559626234941203116, -1.199719254218450271 ) ) ;
#210469=CARTESIAN_POINT ( 'NONE',  ( -5.803772275101700906, 8.928762199997411386, -1.199719254218452047 ) ) ;
#210470=CARTESIAN_POINT ( 'NONE',  ( 5.006703865196457492, 9.063181286029688977, 0.000000000000000000 ) ) ;
#210472=CARTESIAN_POINT ( 'NONE',  ( 7.146556367734771875, 8.470642196179646533, 1.082531754730549967 ) ) ;
#210474=ORIENTED_EDGE ( 'NONE', *, *, #159272, .T. ) ;
#210484=CARTESIAN_POINT ( 'NONE',  ( -6.165548087794384458, 6.979908488848794335, -0.9162763116292941268 ) ) ;
#210494=CARTESIAN_POINT ( 'NONE',  ( -7.445362632559989535, 8.715286488521982733, 1.199719254218452047 ) ) ;
#210511=CARTESIAN_POINT ( 'NONE',  ( 6.150558962454855561, 7.204682206732687000, 1.199719254218452047 ) ) ;
#210530=( BOUNDED_CURVE ( )  B_SPLINE_CURVE ( 2, ( #127481, #157765, #206488 ),
 .UNSPECIFIED., .F., .T. ) 
 B_SPLINE_CURVE_WITH_KNOTS ( ( 3, 3 ),
 ( 0.5204868702216902676, 0.5236290400471614870 ),
 .UNSPECIFIED. ) 
 CURVE ( )  GEOMETRIC_REPRESENTATION_ITEM ( )  RATIONAL_B_SPLINE_CURVE ( ( 0.9334758596551839815, 0.9292753537475906267, 0.9631703981915431534 ) ) 
 REPRESENTATION_ITEM ( '' )  );
#210547=CARTESIAN_POINT ( 'NONE',  ( 8.014278199453778839, 8.522615118883788199, 0.000000000000000000 ) ) ;
#210562=FACE_BOUND ( 'NONE', #88203, .T. ) ;
#210576=B_SPLINE_CURVE_WITH_KNOTS ( 'NONE', 3,
 ( #40022, #106134, #121347, #124554, #38952, #57332, #105034, #155905, #42169, #189460 ),
 .UNSPECIFIED., .F., .F.,
 ( 4, 3, 3, 4 ),
 ( 0.000000000000000000, 0.0001239189758929266515, 0.0002508800143817408444, 0.0003785579584827512443 ),
 .UNSPECIFIED. ) ;
#210578=ADVANCED_FACE ( 'NONE', ( #117062 ), #69284, .T. ) ;
#210580=CARTESIAN_POINT ( 'NONE',  ( -4.620296487206990932, 8.612372678375294299, 0.000000000000000000 ) ) ;
#210582=CARTESIAN_POINT ( 'NONE',  ( 6.549997608733495902, 7.774656977344789333, -1.082531754730548412 ) ) ;
#210588=CARTESIAN_POINT ( 'NONE',  ( -4.522526758610270647, 7.433975764090723359, -1.199719254218453823 ) ) ;
#210593=CARTESIAN_POINT ( 'NONE',  ( -2.959422669532919326, 6.674686557755516780, 0.7998128361456352531 ) ) ;
#210600=CARTESIAN_POINT ( 'NONE',  ( -5.448397627845328550, 7.449826213943242514, 1.599625672291263179 ) ) ;
#210610=CARTESIAN_POINT ( 'NONE',  ( -5.496904935697871863, 5.377753611261092637, 0.7998128361456281477 ) ) ;
#210611=ADVANCED_FACE ( 'NONE', ( #201419 ), #199293, .T. ) ;
#210614=CARTESIAN_POINT ( 'NONE',  ( -5.641601317062247212, 7.675230518029648508, -1.443375672974066548 ) ) ;
#210615=CARTESIAN_POINT ( 'NONE',  ( -5.438229012412888252, 9.358701257874761481, -0.7216878364870338292 ) ) ;
#210616=CARTESIAN_POINT ( 'NONE',  ( 6.062430963966053632, 7.101866208495718702, -1.199719254218452047 ) ) ;
#210617=CARTESIAN_POINT ( 'NONE',  ( -7.632314129850253259, 7.869064337772231355, 0.7998128361456341429 ) ) ;
#210654=CARTESIAN_POINT ( 'NONE',  ( 4.807910157829258679, 8.239027388120819140, -0.8806314816870459694 ) ) ;
#210658=AXIS2_PLACEMENT_3D ( 'NONE', #75162, #125064, #189967 ) ;
#210668=CARTESIAN_POINT ( 'NONE',  ( 7.537407054554579489, 7.758339416593960536, 0.000000000000000000 ) ) ;
#210671=CARTESIAN_POINT ( 'NONE',  ( -3.793249116773374396, 7.647484079536056356, 0.7998128361456352531 ) ) ;
#210675=CARTESIAN_POINT ( 'NONE',  ( -7.417719440008134768, 7.826629899530511025, 0.7216878364870317197 ) ) ;
#210685=CARTESIAN_POINT ( 'NONE',  ( 5.969332771766739931, 10.18624834369502885, -0.7998128361456481317 ) ) ;
#210686=CARTESIAN_POINT ( 'NONE',  ( 6.204791576909545192, 7.267953590263130259, -1.199719254218452047 ) ) ;
#210694=CARTESIAN_POINT ( 'NONE',  ( 3.464990776744291345, 6.200183785247111778, 1.199719254218452047 ) ) ;
#210700=CARTESIAN_POINT ( 'NONE',  ( 6.200875153403774043, 8.327716660428123419, -1.599625672291283607 ) ) ;
#210714=CARTESIAN_POINT ( 'NONE',  ( -5.316205630334268406, 6.335233002545657577, -1.082531754730549967 ) ) ;
#210715=CARTESIAN_POINT ( 'NONE',  ( -6.291865805193673111, 9.498204651771386509, -1.199719254218452047 ) ) ;
#210727=CARTESIAN_POINT ( 'NONE',  ( -2.959422669532919326, 6.674686557755516780, 0.7998128361456352531 ) ) ;
#210728=CARTESIAN_POINT ( 'NONE',  ( 4.877901405866606588, 8.912911750144889567, 0.7998128361456341429 ) ) ;
#210731=CARTESIAN_POINT ( 'NONE',  ( 3.214691819771663628, 6.764574533126651801, -0.7216878364870338292 ) ) ;
#210733=VERTEX_POINT ( 'NONE', #85557 ) ;
#210749=CARTESIAN_POINT ( 'NONE',  ( 4.050854035433010480, 7.948023151305657841, 0.000000000000000000 ) ) ;
#210751=CARTESIAN_POINT ( 'NONE',  ( -5.167592825464113915, 6.057888380243431570, 1.199719254218452935 ) ) ;
#210755=CARTESIAN_POINT ( 'NONE',  ( 6.235824307642648279, 6.239826211863360506, 0.000000000000000000 ) ) ;
#210765=CARTESIAN_POINT ( 'NONE',  ( 6.373741612200160667, 9.489763409991955001, 1.082531754730549078 ) ) ;
#210767=CARTESIAN_POINT ( 'NONE',  ( -7.282664789195997912, 8.525472337930658284, 1.199719254218452047 ) ) ;
#210768=CARTESIAN_POINT ( 'NONE',  ( 5.611095471209277541, 7.639640364534566075, 1.599625672291268286 ) ) ;
#210777=CARTESIAN_POINT ( 'NONE',  ( -3.935609729716867289, 7.813571461303467913, 0.7998128361456352531 ) ) ;
#210794=ORIENTED_EDGE ( 'NONE', *, *, #139645, .F. ) ;
#210803=CARTESIAN_POINT ( 'NONE',  ( 5.899206235721897507, 6.055031161196562373, 0.000000000000000000 ) ) ;
#210804=ORIENTED_EDGE ( 'NONE', *, *, #203693, .F. ) ;
#210809=CARTESIAN_POINT ( 'NONE',  ( 5.872089928050205465, 6.023395468912922546, -0.7216878364870458196 ) ) ;
#210821=CARTESIAN_POINT ( 'NONE',  ( -6.818824913030298696, 6.919993584815607335, 0.7998128361456341429 ) ) ;
#210823=CARTESIAN_POINT ( 'NONE',  ( -6.774234028683526532, 7.932303117332766718, 1.199719254218452047 ) ) ;
#210830=CARTESIAN_POINT ( 'NONE',  ( 6.393551957296131683, 9.616838495890963401, 1.199719254218452047 ) ) ;
#210835=CARTESIAN_POINT ( 'NONE',  ( -5.448397627845328550, 7.449826213943242514, 1.599625672291263179 ) ) ;
#210842=CARTESIAN_POINT ( 'NONE',  ( -3.960390268967665328, 6.674186842887300131, 1.082531754730549967 ) ) ;
#210844=ORIENTED_EDGE ( 'NONE', *, *, #72882, .F. ) ;
#210846=CARTESIAN_POINT ( 'NONE',  ( -5.743814354044916470, 6.730146830254374990, -1.199719254218453823 ) ) ;
#210865=CARTESIAN_POINT ( 'NONE',  ( -6.444921918449773024, 8.612437886315108315, 1.599625672291269396 ) ) ;
#210867=CARTESIAN_POINT ( 'NONE',  ( -5.503684012504701961, 5.385662534202396934, 0.000000000000000000 ) ) ;
#210891=CARTESIAN_POINT ( 'NONE',  ( -5.121948170912633991, 9.197632976031879792, -0.7998128361456362523 ) ) ;
#210915=CARTESIAN_POINT ( 'NONE',  ( 6.770317605177710085, 8.992066187497757213, 1.599625672291268286 ) ) ;
#210916=CARTESIAN_POINT ( 'NONE',  ( 8.018721507839716267, 8.319872945426633137, -0.7998128361456341429 ) ) ;
#210929=CARTESIAN_POINT ( 'NONE',  ( 5.685886686578042415, 7.314606927785019863, 1.221034997698521307 ) ) ;
#210931=CARTESIAN_POINT ( 'NONE',  ( 5.966997003790217136, 8.054858819212300958, -1.443375672974078761 ) ) ;
#210937=CARTESIAN_POINT ( 'NONE',  ( -3.959863383643135393, 6.777535159962392086, 1.199719254218452935 ) ) ;
#210940=ADVANCED_FACE ( 'NONE', ( #2146 ), #49870, .F. ) ;
#210943=CARTESIAN_POINT ( 'NONE',  ( -4.923019175093582334, 8.757623114335565617, 0.7216878364870267237 ) ) ;
#210951=CARTESIAN_POINT ( 'NONE',  ( -4.659162064951642535, 5.464719159645540003, 1.199719254218452935 ) ) ;
#210960=CARTESIAN_POINT ( 'NONE',  ( 8.167861197590044142, 8.493869250135347215, 0.000000000000000000 ) ) ;
#210967=AXIS2_PLACEMENT_3D ( 'NONE', #177377, #144910, #80933 ) ;
#210981=CARTESIAN_POINT ( 'NONE',  ( 7.205232291019763480, 7.370802192470005565, -0.7998128361456341429 ) ) ;
#210983=CARTESIAN_POINT ( 'NONE',  ( -5.850575378433040541, 7.204527765336914413, 1.160475518089182811 ) ) ;
#210990=CARTESIAN_POINT ( 'NONE',  ( 4.369470645354133431, 8.319742529546998000, 0.7998128361456271485 ) ) ;
#210996=ADVANCED_FACE ( 'NONE', ( #156980 ), #203547, .F. ) ;
#211003=CARTESIAN_POINT ( 'NONE',  ( 6.712695452541852070, 7.004101914153185504, 0.000000000000000000 ) ) ;
#211015=CARTESIAN_POINT ( 'NONE',  ( -6.021229618244897885, 7.157760988441397743, 1.082531754730548412 ) ) ;
#211041=ORIENTED_EDGE ( 'NONE', *, *, #3651, .F. ) ;
#211045=CARTESIAN_POINT ( 'NONE',  ( 6.527324610336440180, 6.579909898339485252, 0.7998128361456331437 ) ) ;
#211047=CARTESIAN_POINT ( 'NONE',  ( 6.235824307642648279, 6.239826211863360506, 0.000000000000000000 ) ) ;
#211059=CARTESIAN_POINT ( 'NONE',  ( -7.783789588021474692, 8.253711738879413673, 0.7216878364870317197 ) ) ;
#211062=CARTESIAN_POINT ( 'NONE',  ( 3.702785349863636277, 7.334016984900627811, -0.7216878364870338292 ) ) ;
#211064=B_SPLINE_CURVE_WITH_KNOTS ( 'NONE', 3,
 ( #13267, #163804, #44730, #12195, #177917, #172859 ),
 .UNSPECIFIED., .F., .F.,
 ( 4, 2, 4 ),
 ( 1.087951779939714852E-13, 0.0004226202102664585575, 0.0008452404204241236070 ),
 .UNSPECIFIED. ) ;
#211073=CARTESIAN_POINT ( 'NONE',  ( 5.305644874903189034, 7.627616123249468139, -1.238305686157632701 ) ) ;
#211079=CARTESIAN_POINT ( 'NONE',  ( -5.804299160426237059, 7.865044668620976509, -1.443375672974066548 ) ) ;
#211080=ORIENTED_EDGE ( 'NONE', *, *, #111897, .T. ) ;
#211081=CARTESIAN_POINT ( 'NONE',  ( -3.851925040058333582, 7.508013290127760087, -0.7216878364870458196 ) ) ;
#211082=CARTESIAN_POINT ( 'NONE',  ( 4.294896950644969458, 7.100883960644856607, 1.224551608757080245 ) ) ;
#211118=CARTESIAN_POINT ( 'NONE',  ( -6.454563648557663846, 9.688018802362710957, -1.199719254218452047 ) ) ;
#211119=CARTESIAN_POINT ( 'NONE',  ( -4.611335679197930304, 8.465601755996580380, 0.3353434889079315862 ) ) ;
#211127=CARTESIAN_POINT ( 'NONE',  ( -3.817502770699643388, 6.611447778194983194, 1.199719254218452935 ) ) ;
#211130=CARTESIAN_POINT ( 'NONE',  ( -4.573896719763875574, 6.429575154514868274, -1.599625672291271394 ) ) ;
#211144=CARTESIAN_POINT ( 'NONE',  ( 3.888156192069020634, 7.758209000714329839, 1.040834085586084257E-14 ) ) ;
#211166=CARTESIAN_POINT ( 'NONE',  ( 6.391743074199808916, 6.421731439513382433, -0.7998128361456481317 ) ) ;
#211167=CARTESIAN_POINT ( 'NONE',  ( 3.790386463472274148, 6.579812086429759788, 1.199719254218452047 ) ) ;
#211182=CARTESIAN_POINT ( 'NONE',  ( 4.978670620768666844, 8.057607364700732688, 1.103355461389814662 ) ) ;
#211183=AXIS2_PLACEMENT_3D ( 'NONE', #94896, #128532, #213918 ) ;
#211184=CARTESIAN_POINT ( 'NONE',  ( -6.089020385868867180, 7.236850217336030511, -1.082531754730549967 ) ) ;
#211185=CARTESIAN_POINT ( 'NONE',  ( 5.099275172515607579, 5.121778254122544283, -0.7216878364870458196 ) ) ;
#211207=CARTESIAN_POINT ( 'NONE',  ( -5.607353961982827428, 5.583904275368083425, -0.3699160404166280114 ) ) ;
#211213=CARTESIAN_POINT ( 'NONE',  ( 4.908934136599710563, 7.884784371745123366, 1.199719254218451159 ) ) ;
#211215=CARTESIAN_POINT ( 'NONE',  ( 4.543917759235442944, 5.330267469643351852, 1.199719254218452935 ) ) ;
#211231=CARTESIAN_POINT ( 'NONE',  ( -6.444921918449773024, 8.612437886315108315, 1.599625672291269396 ) ) ;
#211242=CARTESIAN_POINT ( 'NONE',  ( 5.611095471209277541, 7.639640364534566075, 1.599625672291268286 ) ) ;
#211248=CARTESIAN_POINT ( 'NONE',  ( 5.899733120602060232, 6.912052057904395141, -1.199719254218452047 ) ) ;
#211255=ORIENTED_EDGE ( 'NONE', *, *, #134736, .F. ) ;
#211260=CARTESIAN_POINT ( 'NONE',  ( 4.605417112443645600, 8.360468292628990383, 0.2083848827989076002 ) ) ;
#211269=CARTESIAN_POINT ( 'NONE',  ( 3.125598124496329360E-16, 2.519999999999999130, 2.000000000000000000 ) ) ;
#211275=CARTESIAN_POINT ( 'NONE',  ( -6.269955220449294764, 6.909144929749425401, 0.7818200943594469932 ) ) ;
#211282=CARTESIAN_POINT ( 'NONE',  ( -6.469175572376043348, 7.576401584974034265, 1.199719254218452047 ) ) ;
#211284=CARTESIAN_POINT ( 'NONE',  ( 6.008198349511364000, 7.038594824965278995, 1.199719254218453823 ) ) ;
#211288=CARTESIAN_POINT ( 'NONE',  ( -7.747558435566414659, 8.003516027774422170, -0.7998128361456362523 ) ) ;
#211292=CARTESIAN_POINT ( 'NONE',  ( 4.042376459914751585, 3.868111981006289835, -2.500000000000000444 ) ) ;
#211296=EDGE_CURVE ( 'NONE', #80951, #22839, #210576, .T. ) ;
#211297=CARTESIAN_POINT ( 'NONE',  ( -6.087900257701670981, 7.118292344597175081, -1.149031449265491167 ) ) ;
#211313=VERTEX_POINT ( 'NONE', #6422 ) ;
#211314=CARTESIAN_POINT ( 'NONE',  ( 6.211043768836181478, 7.379210830797944709, 1.082531754730549967 ) ) ;
#211316=DIRECTION ( 'NONE',  ( 0.000000000000000000, 0.000000000000000000, -1.000000000000000000 ) ) ;
#211319=ORIENTED_EDGE ( 'NONE', *, *, #82890, .F. ) ;
#211326=CARTESIAN_POINT ( 'NONE',  ( -3.838364070418780027, 7.492192144726518954, 0.0001517565043702621237 ) ) ;
#211327=CARTESIAN_POINT ( 'NONE',  ( -4.123088112331656951, 6.864000993478624579, 1.082531754730549967 ) ) ;
#211331=CARTESIAN_POINT ( 'NONE',  ( 3.711900195091365262, 7.552577004240394132, -0.7998128361456362523 ) ) ;
#211346=ORIENTED_EDGE ( 'NONE', *, *, #168152, .F. ) ;
#211347=CARTESIAN_POINT ( 'NONE',  ( 7.015401035077338143, 6.062865449010541141, 2.437084766375292144 ) ) ;
#211350=CARTESIAN_POINT ( 'NONE',  ( 6.739811759324814133, 8.956476034002680109, -1.443375672974078761 ) ) ;
#211374=CARTESIAN_POINT ( 'NONE',  ( 4.936577329151614180, 4.931964103531220722, -0.7216878364870458196 ) ) ;
#211383=CARTESIAN_POINT ( 'NONE',  ( -3.485854892044994102, 7.080931450778859215, -0.7216878364870458196 ) ) ;
#211389=CARTESIAN_POINT ( 'NONE',  ( -6.622231685632140596, 6.690634819517756959, 0.000000000000000000 ) ) ;
#211400=CARTESIAN_POINT ( 'NONE',  ( -5.276058054373441664, 6.184431147304315424, -1.199719254218453823 ) ) ;
#211402=CARTESIAN_POINT ( 'NONE',  ( 6.468016842275610578, 6.857101109195174793, 0.6445861549769070775 ) ) ;
#211407=CARTESIAN_POINT ( 'NONE',  ( 6.879836604291781121, 6.991173891287354003, -0.7998128361456341429 ) ) ;
#211415=CARTESIAN_POINT ( 'NONE',  ( -3.156015896931072540, 6.904045323053366268, 0.000000000000000000 ) ) ;
#211419=CARTESIAN_POINT ( 'NONE',  ( -5.957882158562513908, 5.915560371269843465, -0.7998128361456362523 ) ) ;
#211421=B_SPLINE_CURVE_WITH_KNOTS ( 'NONE', 3,
 ( #60674, #190663, #144116, #74807, #30326, #157134, #8725, #206921 ),
 .UNSPECIFIED., .F., .F.,
 ( 4, 2, 2, 4 ),
 ( 0.001370800379555754591, 0.001589083288849510098, 0.001807366198143265388, 0.002243932016730776184 ),
 .UNSPECIFIED. ) ;
#211424=CARTESIAN_POINT ( 'NONE',  ( 6.549997608733495902, 7.774656977344789333, -1.082531754730548412 ) ) ;
#211426=CARTESIAN_POINT ( 'NONE',  ( -7.092323753280154186, 7.447001598347859463, 0.7216878364870317197 ) ) ;
#211432=CARTESIAN_POINT ( 'NONE',  ( 5.825163275726873202, 6.825053905550038991, 1.199719254218452047 ) ) ;
#211458=CARTESIAN_POINT ( 'NONE',  ( 5.234661009243278151, 7.693064604033777343, 1.208367059251337361 ) ) ;
#211467=CARTESIAN_POINT ( 'NONE',  ( 5.936491157937257235, 8.019268665717216749, 1.599625672291268286 ) ) ;
#211472=CARTESIAN_POINT ( 'NONE',  ( -5.947459870766462764, 7.133493745255431229, -1.104964307564069603 ) ) ;
#211479=CARTESIAN_POINT ( 'NONE',  ( -6.084577077482911101, 10.32070003369722144, 0.000000000000000000 ) ) ;
#211489=CARTESIAN_POINT ( 'NONE',  ( -4.492547798081878874, 6.334668079219206049, 1.599625672291263179 ) ) ;
#211491=CARTESIAN_POINT ( 'NONE',  ( 6.393551957296131683, 9.616838495890963401, 1.199719254218452047 ) ) ;
#211502=CARTESIAN_POINT ( 'NONE',  ( 5.285699784481295183, 7.260012063351913625, 1.599625672291268286 ) ) ;
#211505=CARTESIAN_POINT ( 'NONE',  ( 6.061904078641523697, 7.205214525570814210, -1.082531754730548412 ) ) ;
#211508=VERTEX_POINT ( 'NONE', #11762 ) ;
#211519=CARTESIAN_POINT ( 'NONE',  ( -3.637330350216213759, 7.465578851886037093, -0.7998128361456481317 ) ) ;
#211520=CARTESIAN_POINT ( 'NONE',  ( 3.542423274920540432, 7.354853930707762721, -1.734723475976807094E-15 ) ) ;
#211530=VERTEX_POINT ( 'NONE', #179615 ) ;
#211531=CARTESIAN_POINT ( 'NONE',  ( -7.286581212701773502, 7.465709267765667789, 0.7998128361456341429 ) ) ;
#211532=CARTESIAN_POINT ( 'NONE',  ( 5.722423353419669567, 8.833855124701747386, 1.199719254218451159 ) ) ;
#211534=CARTESIAN_POINT ( 'NONE',  ( -3.188928480291339795, 8.980740528189214089, -2.451733079074510879 ) ) ;
#211545=CARTESIAN_POINT ( 'NONE',  ( -6.605427497552981642, 6.764401258476403278, 0.1916688254133581959 ) ) ;
#211555=CARTESIAN_POINT ( 'NONE',  ( -3.160459205317013076, 6.701303149596211206, -0.7216878364870458196 ) ) ;
#211566=DIRECTION ( 'NONE',  ( -0.7592566023652995710, -0.6507913734559650498, 0.000000000000000000 ) ) ;
#211570=CARTESIAN_POINT ( 'NONE',  ( 7.340813827156391191, 7.528980651296110160, 0.7998128361456281477 ) ) ;
#211603=CARTESIAN_POINT ( 'NONE',  ( 4.390861645979372341, 6.216034235099629157, -1.599625672291269396 ) ) ;
#211604=CARTESIAN_POINT ( 'NONE',  ( -4.502716413514313842, 5.386162249589033557, -1.082531754730549967 ) ) ;
#211634=CARTESIAN_POINT ( 'NONE',  ( -6.805266759416629618, 6.904175738932996964, 0.000000000000000000 ) ) ;
#211636=CARTESIAN_POINT ( 'NONE',  ( 5.017926250389229459, 8.868348035513836436, 0.000000000000000000 ) ) ;
#211642=CARTESIAN_POINT ( 'NONE',  ( -6.493429226302317225, 6.540365283632955773, 0.7998128361456341429 ) ) ;
#211647=CARTESIAN_POINT ( 'NONE',  ( -5.320648938720212051, 5.172121614787156929, 0.000000000000000000 ) ) ;
#211652=CARTESIAN_POINT ( 'NONE',  ( -6.448838341955544173, 7.552674816150118708, 1.199719254218452047 ) ) ;
#211664=CARTESIAN_POINT ( 'NONE',  ( -4.228163802615396705, 6.026220084508304708, -1.599625672291271394 ) ) ;
#211667=CARTESIAN_POINT ( 'NONE',  ( -5.099275172515603138, 8.002885897026576600, 1.082531754730549967 ) ) ;
#211668=CARTESIAN_POINT ( 'NONE',  ( -6.333067150914850174, 8.481940657524365434, 1.443375672974064550 ) ) ;
#211669=CARTESIAN_POINT ( 'NONE',  ( 7.472478939787284169, 8.746922180287201698, 1.199719254218452935 ) ) ;
#211670=CARTESIAN_POINT ( 'NONE',  ( -7.293360289508603600, 7.473618190706972086, 0.000000000000000000 ) ) ;
#211679=ORIENTED_EDGE ( 'NONE', *, *, #98746, .T. ) ;
#211710=CARTESIAN_POINT ( 'NONE',  ( 5.061762083669725243, 7.855803969722688684, -1.119403510469544782 ) ) ;
#211725=CARTESIAN_POINT ( 'NONE',  ( 7.212011367826596242, 7.378711115411311638, 0.000000000000000000 ) ) ;
#211728=CARTESIAN_POINT ( 'NONE',  ( -6.154475385960665790, 6.144919136567696505, 0.000000000000000000 ) ) ;
#211732=CARTESIAN_POINT ( 'NONE',  ( -7.390603132780803719, 7.794994207765291172, -0.7216878364870338292 ) ) ;
#211742=CARTESIAN_POINT ( 'NONE',  ( 4.386945222473598527, 7.275797305264619652, -1.199719254218452047 ) ) ;
#211745=CARTESIAN_POINT ( 'NONE',  ( 7.367930134383754215, 7.560616343061329125, -0.7998128361456341429 ) ) ;
#211759=CARTESIAN_POINT ( 'NONE',  ( 5.550083779947807550, 7.568460058062819407, -1.599625672291283607 ) ) ;
#211768=LINE ( 'NONE', #63406, #112331 ) ;
#211772=CARTESIAN_POINT ( 'NONE',  ( -5.641601317062259646, 5.754492089426966217, -0.7216878364870338292 ) ) ;
#211773=CARTESIAN_POINT ( 'NONE',  ( 5.017926250833595780, 7.907978821730911712, -1.082531754730548412 ) ) ;
#211783=ORIENTED_EDGE ( 'NONE', *, *, #65745, .T. ) ;
#211785=CARTESIAN_POINT ( 'NONE',  ( -5.750066545971566079, 8.762142499391876171, 1.082531754730550855 ) ) ;
#211789=CARTESIAN_POINT ( 'NONE',  ( 4.055297343818931033, 6.784911763547157193, 1.082531754730549078 ) ) ;
#211798=( BOUNDED_SURFACE ( )  B_SPLINE_SURFACE ( 1, 2, ( 
 ( #193695, #143937, #176400, #10671, #29077, #113591, #28005, #95162, #112516, #111458, #97289, #46400, #179594, #163346, #208866, #194763, #129855, #45339, #76742, #61571, #161211, #78871, #12798, #144994, #128784, #178530, #32272, #142864, #30140, #44274, #60496, #130903, #110395, #81017, #96228, #11741, #79944, #213130, #196896, #48535, #114654, #98339, #94102, #185968, #164404, #115706, #18124, #201140, #17056, #66857, #70071, #37601, #51729, #166536, #117851, #84213, #131942, #49581, #136184, #165461, #183843, #181696, #197953, #36522, #33326, #99408, #790, #83137, #149215, #102609, #202204, #133003, #199003, #50647, #116774, #20268, #35455, #1867, #150301, #148165, #19201, #53858, #182771, #101533, #34388, #200081, #119991, #100460, #85280, #4002, #2935, #135124, #167603, #151366, #67927, #15988, #134072, #69007, #52778, #82073, #214168, #65793, #118917, #184898, #168664, #86352, #152423, #206493, #72210, #6140, #24536, #123223, #59184, #154564, #55991, #7211, #71140, #122142, #23469, #205421, #190242, #38674, #204333, #40824, #106934, #22392, #75442, #73285, #156705, #172957, #90644, #8295, #104753, #140481, #5064, #25610, #125339, #170802, #137257, #157773, #89577, #188110, #155626, #74379, #58123, #124282, #41900, #139388, #141554, #108011, #207561, #174037, #54923, #57059, #138317, #88501, #191302, #91722, #21320, #39741, #153494, #9371, #103682, #203277, #169731, #105845, #87427, #121075, #187042, #171872, #189187, #64522, #93853, #26682, #110144, #176157, #195598, #130668, #159890, #63458, #44026, #160965, #112276, #29900, #27757, #42970, #79701, #80781, #163105, #11498, #146869, #143692, #113349, #12555, #77569, #28827, #209684, #14685, #78629, #95985, #46163, #178293, #194515, #192370, #145816, #158829, #179354, #212891, #61328, #10425, #97051, #94916, #127487, #144754, #13628, #162037, #211821, #129612, #177214, #109080, #47234, #175095, #30976, #208617, #210765, #193458, #45102, #92784, #76497, #142609, #111212, #60251, #126408, #62385, #128550, #18942, #33088, #168414, #184645, #68753, #65554 ),
 ( #35196, #36265, #99162, #199831, #166280, #115466, #148966, #165215, #49347, #16805, #82891, #539, #180408, #66605, #147916, #164163, #101270, #200882, #17869, #132751, #131700, #98112, #133818, #83953, #198754, #117596, #197705, #50403, #181458, #213933, #196656, #116521, #85027, #182512, #34142, #150043, #100211, #134875, #1614, #151115, #52527, #32026, #67674, #183587, #51472, #48297, #167355, #2682, #118662, #102343, #20011, #86097, #152171, #3740, #114408, #69815, #15749, #81833, #189994, #37343, #8033, #204075, #136993, #71952, #156449, #154306, #70881, #104495, #39478, #138062, #157521, #135921, #87159, #55727, #172696, #203020, #124027, #155365, #91459, #6950, #54662, #201941, #119731, #121882, #9116, #41644, #107758, #185709, #188928, #38414, #171610, #120810, #186787, #5878, #53596, #122968, #106673, #170538, #103417, #187852, #90380, #22123, #88235, #153230, #74124, #40565, #173784, #105577, #139129, #23204, #89318, #73031, #205157, #56799, #24274, #140219, #206239, #169478, #57865, #4800, #21062, #25359, #79455, #110955, #43783, #10177, #191051, #12303, #44849, #109896, #210511, #76251, #175908, #142361, #26428, #75191, #93599, #112032, #92538, #27499, #176962, #159643, #161789, #28578, #178035, #13380, #58936, #94667, #62147, #11241, #141303, #60002, #126155, #143432, #192118, #208370, #77319, #160709, #30722, #207313, #209428, #108824, #125093, #129368, #42716, #145572, #61073, #127232, #193202, #95738, #78384, #144504, #128306, #194268, #45914, #96805, #174849, #158578, #29652, #211570, #63204, #195346, #46979, #165771, #113095, #179100, #119205, #19496, #199305, #117075, #137547, #18433, #185191, #183074, #50951, #103975, #100755, #34686, #68235, #166837, #84507, #135410, #55218, #2158, #36815, #187338, #102897, #150596, #17354, #1104, #85571, #105053, #71435, #203565, #67163, #70364, #134369, #53072, #200373, #52021, #101828, #83436, #4293, #202500, #118146, #184131, #69298, #186263, #35754, #167896, #151661, #37898, #136478, #121363, #3233, #20560, #201432, #168956, #86643, #152710, #54151 ) ),
 .UNSPECIFIED., .F., .F., .F. ) 
 B_SPLINE_SURFACE_WITH_KNOTS ( ( 2, 2 ),
 ( 3, 2, 2, 2, 2, 2, 2, 2, 2, 2, 2, 2, 2, 2, 2, 2, 2, 2, 2, 2, 2, 2, 2, 2, 2, 2, 2, 2, 2, 2, 2, 2, 2, 2, 2, 2, 2, 2, 2, 2, 2, 2, 2, 2, 2, 2, 2, 2, 2, 2, 2, 2, 2, 2, 2, 2, 2, 2, 2, 2, 2, 2, 2, 2, 2, 2, 2, 2, 2, 2, 2, 2, 2, 2, 2, 2, 2, 2, 2, 2, 2, 2, 2, 2, 2, 2, 2, 2, 2, 2, 2, 2, 2, 2, 2, 2, 2, 2, 2, 2, 2, 2, 2, 2, 2, 2, 2, 2, 2, 2, 2, 2, 2, 2, 2, 2, 2, 2, 2, 2, 3 ),
 ( 0.000000000000000000, 1.000000000000000000 ),
 ( 0.000000000000000000, 0.008333333333333333218, 0.01666666666666666644, 0.02500000000000000139, 0.03333333333333333287, 0.04166666666666666435, 0.05000000000000000278, 0.05833333333333333426, 0.06666666666666666574, 0.07499999999999999722, 0.08333333333333332871, 0.09166666666666666019, 0.1000000000000000056, 0.1083333333333333370, 0.1166666666666666685, 0.1250000000000000000, 0.1333333333333333315, 0.1416666666666666630, 0.1499999999999999944, 0.1583333333333333259, 0.1666666666666666574, 0.1749999999999999889, 0.1833333333333333204, 0.1916666666666666796, 0.2000000000000000111, 0.2083333333333333426, 0.2166666666666666741, 0.2250000000000000056, 0.2333333333333333370, 0.2416666666666666685, 0.2500000000000000000, 0.2583333333333333592, 0.2666666666666666630, 0.2750000000000000222, 0.2833333333333333259, 0.2916666666666666852, 0.2999999999999999889, 0.3083333333333333481, 0.3166666666666666519, 0.3250000000000000111, 0.3333333333333333148, 0.3416666666666666741, 0.3499999999999999778, 0.3583333333333333370, 0.3666666666666666408, 0.3750000000000000000, 0.3833333333333333592, 0.3916666666666666630, 0.4000000000000000222, 0.4083333333333333259, 0.4166666666666666852, 0.4249999999999999889, 0.4333333333333333481, 0.4416666666666666519, 0.4500000000000000111, 0.4583333333333333148, 0.4666666666666666741, 0.4749999999999999778, 0.4833333333333333370, 0.4916666666666666408, 0.5000000000000000000, 0.5083333333333333037, 0.5166666666666667185, 0.5250000000000000222, 0.5333333333333333259, 0.5416666666666666297, 0.5500000000000000444, 0.5583333333333333481, 0.5666666666666666519, 0.5749999999999999556, 0.5833333333333333703, 0.5916666666666666741, 0.5999999999999999778, 0.6083333333333332815, 0.6166666666666666963, 0.6250000000000000000, 0.6333333333333333037, 0.6416666666666667185, 0.6500000000000000222, 0.6583333333333333259, 0.6666666666666666297, 0.6750000000000000444, 0.6833333333333333481, 0.6916666666666666519, 0.6999999999999999556, 0.7083333333333333703, 0.7166666666666666741, 0.7249999999999999778, 0.7333333333333332815, 0.7416666666666666963, 0.7500000000000000000, 0.7583333333333333037, 0.7666666666666667185, 0.7750000000000000222, 0.7833333333333333259, 0.7916666666666666297, 0.8000000000000000444, 0.8083333333333333481, 0.8166666666666666519, 0.8249999999999999556, 0.8333333333333333703, 0.8416666666666666741, 0.8499999999999999778, 0.8583333333333332815, 0.8666666666666666963, 0.8750000000000000000, 0.8833333333333333037, 0.8916666666666667185, 0.9000000000000000222, 0.9083333333333333259, 0.9166666666666666297, 0.9250000000000000444, 0.9333333333333333481, 0.9416666666666666519, 0.9499999999999999556, 0.9583333333333333703, 0.9666666666666666741, 0.9749999999999999778, 0.9833333333333332815, 0.9916666666666666963, 1.000000000000000000 ),
 .UNSPECIFIED. ) 
 GEOMETRIC_REPRESENTATION_ITEM ( )  RATIONAL_B_SPLINE_SURFACE ( (
 ( 1.000000000000000000, 0.8660254037844387076, 1.000000000000000000, 0.8660254037844387076, 1.000000000000000000, 0.8660254037844387076, 1.000000000000000000, 0.8660254037844387076, 1.000000000000000000, 0.8660254037844387076, 1.000000000000000000, 0.8660254037844387076, 1.000000000000000000, 0.8660254037844387076, 1.000000000000000000, 0.8660254037844387076, 1.000000000000000000, 0.8660254037844387076, 1.000000000000000000, 0.8660254037844387076, 1.000000000000000000, 0.8660254037844387076, 1.000000000000000000, 0.8660254037844387076, 1.000000000000000000, 0.8660254037844387076, 1.000000000000000000, 0.8660254037844387076, 1.000000000000000000, 0.8660254037844387076, 1.000000000000000000, 0.8660254037844387076, 1.000000000000000000, 0.8660254037844387076, 1.000000000000000000, 0.8660254037844387076, 1.000000000000000000, 0.8660254037844387076, 1.000000000000000000, 0.8660254037844387076, 1.000000000000000000, 0.8660254037844387076, 1.000000000000000000, 0.8660254037844387076, 1.000000000000000000, 0.8660254037844387076, 1.000000000000000000, 0.8660254037844387076, 1.000000000000000000, 0.8660254037844387076, 1.000000000000000000, 0.8660254037844387076, 1.000000000000000000, 0.8660254037844387076, 1.000000000000000000, 0.8660254037844387076, 1.000000000000000000, 0.8660254037844387076, 1.000000000000000000, 0.8660254037844387076, 1.000000000000000000, 0.8660254037844387076, 1.000000000000000000, 0.8660254037844387076, 1.000000000000000000, 0.8660254037844387076, 1.000000000000000000, 0.8660254037844387076, 1.000000000000000000, 0.8660254037844387076, 1.000000000000000000, 0.8660254037844387076, 1.000000000000000000, 0.8660254037844387076, 1.000000000000000000, 0.8660254037844387076, 1.000000000000000000, 0.8660254037844387076, 1.000000000000000000, 0.8660254037844387076, 1.000000000000000000, 0.8660254037844387076, 1.000000000000000000, 0.8660254037844387076, 1.000000000000000000, 0.8660254037844387076, 1.000000000000000000, 0.8660254037844387076, 1.000000000000000000, 0.8660254037844387076, 1.000000000000000000, 0.8660254037844387076, 1.000000000000000000, 0.8660254037844387076, 1.000000000000000000, 0.8660254037844387076, 1.000000000000000000, 0.8660254037844387076, 1.000000000000000000, 0.8660254037844387076, 1.000000000000000000, 0.8660254037844387076, 1.000000000000000000, 0.8660254037844387076, 1.000000000000000000, 0.8660254037844387076, 1.000000000000000000, 0.8660254037844387076, 1.000000000000000000, 0.8660254037844387076, 1.000000000000000000, 0.8660254037844387076, 1.000000000000000000, 0.8660254037844387076, 1.000000000000000000, 0.8660254037844387076, 1.000000000000000000, 0.8660254037844387076, 1.000000000000000000, 0.8660254037844387076, 1.000000000000000000, 0.8660254037844387076, 1.000000000000000000, 0.8660254037844387076, 1.000000000000000000, 0.8660254037844387076, 1.000000000000000000, 0.8660254037844387076, 1.000000000000000000, 0.8660254037844387076, 1.000000000000000000, 0.8660254037844387076, 1.000000000000000000, 0.8660254037844387076, 1.000000000000000000, 0.8660254037844387076, 1.000000000000000000, 0.8660254037844387076, 1.000000000000000000, 0.8660254037844387076, 1.000000000000000000, 0.8660254037844387076, 1.000000000000000000, 0.8660254037844387076, 1.000000000000000000, 0.8660254037844387076, 1.000000000000000000, 0.8660254037844387076, 1.000000000000000000, 0.8660254037844387076, 1.000000000000000000, 0.8660254037844387076, 1.000000000000000000, 0.8660254037844387076, 1.000000000000000000, 0.8660254037844387076, 1.000000000000000000, 0.8660254037844387076, 1.000000000000000000, 0.8660254037844387076, 1.000000000000000000, 0.8660254037844387076, 1.000000000000000000, 0.8660254037844387076, 1.000000000000000000, 0.8660254037844387076, 1.000000000000000000, 0.8660254037844387076, 1.000000000000000000, 0.8660254037844387076, 1.000000000000000000, 0.8660254037844387076, 1.000000000000000000, 0.8660254037844387076, 1.000000000000000000, 0.8660254037844387076, 1.000000000000000000, 0.8660254037844387076, 1.000000000000000000, 0.8660254037844387076, 1.000000000000000000, 0.8660254037844387076, 1.000000000000000000, 0.8660254037844387076, 1.000000000000000000, 0.8660254037844387076, 1.000000000000000000, 0.8660254037844387076, 1.000000000000000000, 0.8660254037844387076, 1.000000000000000000, 0.8660254037844387076, 1.000000000000000000, 0.8660254037844387076, 1.000000000000000000, 0.8660254037844387076, 1.000000000000000000, 0.8660254037844387076, 1.000000000000000000, 0.8660254037844387076, 1.000000000000000000, 0.8660254037844387076, 1.000000000000000000, 0.8660254037844387076, 1.000000000000000000, 0.8660254037844387076, 1.000000000000000000, 0.8660254037844387076, 1.000000000000000000, 0.8660254037844387076, 1.000000000000000000, 0.8660254037844387076, 1.000000000000000000, 0.8660254037844387076, 1.000000000000000000, 0.8660254037844387076, 1.000000000000000000, 0.8660254037844387076, 1.000000000000000000, 0.8660254037844387076, 1.000000000000000000, 0.8660254037844387076, 1.000000000000000000, 0.8660254037844387076, 1.000000000000000000, 0.8660254037844387076, 1.000000000000000000, 0.8660254037844387076, 1.000000000000000000, 0.8660254037844387076, 1.000000000000000000, 0.8660254037844387076, 1.000000000000000000, 0.8660254037844387076, 1.000000000000000000, 0.8660254037844387076, 1.000000000000000000, 0.8660254037844387076, 1.000000000000000000, 0.8660254037844387076, 1.000000000000000000),
 ( 1.000000000000000000, 0.8660254037844387076, 1.000000000000000000, 0.8660254037844387076, 1.000000000000000000, 0.8660254037844387076, 1.000000000000000000, 0.8660254037844387076, 1.000000000000000000, 0.8660254037844387076, 1.000000000000000000, 0.8660254037844387076, 1.000000000000000000, 0.8660254037844387076, 1.000000000000000000, 0.8660254037844387076, 1.000000000000000000, 0.8660254037844387076, 1.000000000000000000, 0.8660254037844387076, 1.000000000000000000, 0.8660254037844387076, 1.000000000000000000, 0.8660254037844387076, 1.000000000000000000, 0.8660254037844387076, 1.000000000000000000, 0.8660254037844387076, 1.000000000000000000, 0.8660254037844387076, 1.000000000000000000, 0.8660254037844387076, 1.000000000000000000, 0.8660254037844387076, 1.000000000000000000, 0.8660254037844387076, 1.000000000000000000, 0.8660254037844387076, 1.000000000000000000, 0.8660254037844387076, 1.000000000000000000, 0.8660254037844387076, 1.000000000000000000, 0.8660254037844387076, 1.000000000000000000, 0.8660254037844387076, 1.000000000000000000, 0.8660254037844387076, 1.000000000000000000, 0.8660254037844387076, 1.000000000000000000, 0.8660254037844387076, 1.000000000000000000, 0.8660254037844387076, 1.000000000000000000, 0.8660254037844387076, 1.000000000000000000, 0.8660254037844387076, 1.000000000000000000, 0.8660254037844387076, 1.000000000000000000, 0.8660254037844387076, 1.000000000000000000, 0.8660254037844387076, 1.000000000000000000, 0.8660254037844387076, 1.000000000000000000, 0.8660254037844387076, 1.000000000000000000, 0.8660254037844387076, 1.000000000000000000, 0.8660254037844387076, 1.000000000000000000, 0.8660254037844387076, 1.000000000000000000, 0.8660254037844387076, 1.000000000000000000, 0.8660254037844387076, 1.000000000000000000, 0.8660254037844387076, 1.000000000000000000, 0.8660254037844387076, 1.000000000000000000, 0.8660254037844387076, 1.000000000000000000, 0.8660254037844387076, 1.000000000000000000, 0.8660254037844387076, 1.000000000000000000, 0.8660254037844387076, 1.000000000000000000, 0.8660254037844387076, 1.000000000000000000, 0.8660254037844387076, 1.000000000000000000, 0.8660254037844387076, 1.000000000000000000, 0.8660254037844387076, 1.000000000000000000, 0.8660254037844387076, 1.000000000000000000, 0.8660254037844387076, 1.000000000000000000, 0.8660254037844387076, 1.000000000000000000, 0.8660254037844387076, 1.000000000000000000, 0.8660254037844387076, 1.000000000000000000, 0.8660254037844387076, 1.000000000000000000, 0.8660254037844387076, 1.000000000000000000, 0.8660254037844387076, 1.000000000000000000, 0.8660254037844387076, 1.000000000000000000, 0.8660254037844387076, 1.000000000000000000, 0.8660254037844387076, 1.000000000000000000, 0.8660254037844387076, 1.000000000000000000, 0.8660254037844387076, 1.000000000000000000, 0.8660254037844387076, 1.000000000000000000, 0.8660254037844387076, 1.000000000000000000, 0.8660254037844387076, 1.000000000000000000, 0.8660254037844387076, 1.000000000000000000, 0.8660254037844387076, 1.000000000000000000, 0.8660254037844387076, 1.000000000000000000, 0.8660254037844387076, 1.000000000000000000, 0.8660254037844387076, 1.000000000000000000, 0.8660254037844387076, 1.000000000000000000, 0.8660254037844387076, 1.000000000000000000, 0.8660254037844387076, 1.000000000000000000, 0.8660254037844387076, 1.000000000000000000, 0.8660254037844387076, 1.000000000000000000, 0.8660254037844387076, 1.000000000000000000, 0.8660254037844387076, 1.000000000000000000, 0.8660254037844387076, 1.000000000000000000, 0.8660254037844387076, 1.000000000000000000, 0.8660254037844387076, 1.000000000000000000, 0.8660254037844387076, 1.000000000000000000, 0.8660254037844387076, 1.000000000000000000, 0.8660254037844387076, 1.000000000000000000, 0.8660254037844387076, 1.000000000000000000, 0.8660254037844387076, 1.000000000000000000, 0.8660254037844387076, 1.000000000000000000, 0.8660254037844387076, 1.000000000000000000, 0.8660254037844387076, 1.000000000000000000, 0.8660254037844387076, 1.000000000000000000, 0.8660254037844387076, 1.000000000000000000, 0.8660254037844387076, 1.000000000000000000, 0.8660254037844387076, 1.000000000000000000, 0.8660254037844387076, 1.000000000000000000, 0.8660254037844387076, 1.000000000000000000, 0.8660254037844387076, 1.000000000000000000, 0.8660254037844387076, 1.000000000000000000, 0.8660254037844387076, 1.000000000000000000, 0.8660254037844387076, 1.000000000000000000, 0.8660254037844387076, 1.000000000000000000, 0.8660254037844387076, 1.000000000000000000, 0.8660254037844387076, 1.000000000000000000, 0.8660254037844387076, 1.000000000000000000, 0.8660254037844387076, 1.000000000000000000, 0.8660254037844387076, 1.000000000000000000, 0.8660254037844387076, 1.000000000000000000, 0.8660254037844387076, 1.000000000000000000, 0.8660254037844387076, 1.000000000000000000, 0.8660254037844387076, 1.000000000000000000, 0.8660254037844387076, 1.000000000000000000, 0.8660254037844387076, 1.000000000000000000, 0.8660254037844387076, 1.000000000000000000, 0.8660254037844387076, 1.000000000000000000, 0.8660254037844387076, 1.000000000000000000, 0.8660254037844387076, 1.000000000000000000, 0.8660254037844387076, 1.000000000000000000, 0.8660254037844387076, 1.000000000000000000, 0.8660254037844387076, 1.000000000000000000, 0.8660254037844387076, 1.000000000000000000, 0.8660254037844387076, 1.000000000000000000, 0.8660254037844387076, 1.000000000000000000) ) ) 
 REPRESENTATION_ITEM ( '' )  SURFACE ( )  );
#211806=CARTESIAN_POINT ( 'NONE',  ( 5.387385936583818591, 7.378645907471495846, -1.599625672291283607 ) ) ;
#211808=CARTESIAN_POINT ( 'NONE',  ( -5.991777542596674166, 5.955104985976372944, 0.000000000000000000 ) ) ;
#211809=B_SPLINE_CURVE_WITH_KNOTS ( 'NONE', 3,
 ( #213996, #211889, #62454, #47301 ),
 .UNSPECIFIED., .F., .F.,
 ( 4, 4 ),
 ( 5.438330430075821877E-18, 0.0005229773533087089940 ),
 .UNSPECIFIED. ) ;
#211821=CARTESIAN_POINT ( 'NONE',  ( 7.688882512725796481, 8.142986817701137525, 0.000000000000000000 ) ) ;
#211823=CARTESIAN_POINT ( 'NONE',  ( -5.257529707049291900, 9.355811434857983500, 0.7998128361456291469 ) ) ;
#211824=CARTESIAN_POINT ( 'NONE',  ( 5.448397627845284141, 7.449826213943242514, 1.599625672291268286 ) ) ;
#211825=ORIENTED_EDGE ( 'NONE', *, *, #28177, .T. ) ;
#211833=CARTESIAN_POINT ( 'NONE',  ( -3.623772196602547346, 7.449761006003425834, 0.000000000000000000 ) ) ;
#211862=CARTESIAN_POINT ( 'NONE',  ( 4.095971805104276164, 7.792734516014745871, 0.7216878364870257245 ) ) ;
#211868=CARTESIAN_POINT ( 'NONE',  ( 4.651856102820254968, 7.480896982382013505, -1.082531754730548412 ) ) ;
#211881=CARTESIAN_POINT ( 'NONE',  ( -6.791708605802965870, 6.888357893050385705, -0.7998128361456362523 ) ) ;
#211883=CARTESIAN_POINT ( 'NONE',  ( -7.208094944320834863, 8.438474185576302133, -1.199719254218452047 ) ) ;
#211885=CARTESIAN_POINT ( 'NONE',  ( 4.601997573603133773, 4.922373501976976762, -0.8019421930630143969 ) ) ;
#211889=CARTESIAN_POINT ( 'NONE',  ( 3.548584350011782185, 7.336486228343999549, 0.1164461989974732298 ) ) ;
#211890=CARTESIAN_POINT ( 'NONE',  ( 7.713663051532233972, 7.963971413067895355, -0.7998128361456341429 ) ) ;
#211896=CARTESIAN_POINT ( 'NONE',  ( -5.608322021959554426, 5.603804175593484871, 0.4115828475494631156 ) ) ;
#211897=CARTESIAN_POINT ( 'NONE',  ( -4.911796789900812144, 8.952456364851418158, 0.7998128361456291469 ) ) ;
#211903=CARTESIAN_POINT ( 'NONE',  ( -4.014622883422322985, 7.697827440719083647, -0.7216878364870458196 ) ) ;
#211906=CARTESIAN_POINT ( 'NONE',  ( -4.936050443827081580, 7.916420063510339666, 1.199719254218452935 ) ) ;
#211928=CARTESIAN_POINT ( 'NONE',  ( -8.106849506328558164, 8.422688943663599659, 0.000000000000000000 ) ) ;
#211929=CARTESIAN_POINT ( 'NONE',  ( 3.627688620108284745, 6.389997935838436227, 1.199719254218452047 ) ) ;
#211930=CARTESIAN_POINT ( 'NONE',  ( -5.004894982100124068, 5.868074229652107121, 1.199719254218452935 ) ) ;
#211953=CARTESIAN_POINT ( 'NONE',  ( -6.149505192250180663, 9.332117270003974951, -1.199719254218452047 ) ) ;
#211976=CARTESIAN_POINT ( 'NONE',  ( 5.691390622686558487, 9.861982503101517139, 0.7998128361456341429 ) ) ;
#211977=CARTESIAN_POINT ( 'NONE',  ( 6.343235766347262938, 8.493804042195527870, -1.599625672291281386 ) ) ;
#211991=CARTESIAN_POINT ( 'NONE',  ( 5.748548729368831545, 7.266256959964179529, 1.200940202139972435 ) ) ;
#211993=CARTESIAN_POINT ( 'NONE',  ( 5.506019780925567986, 8.477421273504887722, -1.082531754730548412 ) ) ;
#211999=CARTESIAN_POINT ( 'NONE',  ( -5.957882158562513908, 5.915560371269843465, -0.7998128361456362523 ) ) ;
#212005=CARTESIAN_POINT ( 'NONE',  ( -7.607533590599451223, 9.008448956188397361, 1.082531754730549078 ) ) ;
#212008=CARTESIAN_POINT ( 'NONE',  ( -5.712738193804302256, 6.079813188454783024, 0.6294087663294201107 ) ) ;
#212012=CARTESIAN_POINT ( 'NONE',  ( -4.502189528189771472, 7.410248995266807803, -1.199719254218453823 ) ) ;
#212020=EDGE_CURVE ( 'NONE', #136449, #45344, #168899, .T. ) ;
#212022=CARTESIAN_POINT ( 'NONE',  ( 5.422335090822693715, 5.290755458906732933, 0.000000000000000000 ) ) ;
#212043=CARTESIAN_POINT ( 'NONE',  ( 6.156284269057003655, 9.340026192945279249, -1.199719254218452047 ) ) ;
#212046=( BOUNDED_SURFACE ( )  B_SPLINE_SURFACE ( 1, 2, ( 
 ( #103522, #2785, #132854, #101380, #183696, #150151, #115563, #116628, #166383, #134976, #182622, #167455, #136028, #1721, #199933, #197811, #34245, #149067, #51580, #152272, #85129, #165317, #148020, #100317, #99269, #151215, #102448, #117705, #168514, #200984, #69917, #118759, #53702, #81934, #184744, #202041, #20114, #119834, #67778, #133927, #185813, #37445, #65655, #131802, #49444, #33187, #181559, #155469, #7054, #107856, #41745, #72056, #171713, #57964, #22229, #120915, #173882, #154406, #121988, #153334, #4908, #204175, #75287, #25459, #169581, #156549, #138167, #39582, #104598, #186888, #54767, #140321, #88342, #55832, #38520, #91566, #90485, #189031, #42818, #21164, #73127, #170644, #205260, #187954, #40669, #139229, #137098, #5985, #105684, #157619, #87268, #70985, #106773, #141402, #23310, #206339, #9216, #203124, #56901, #89420, #123075, #172801, #24372, #8144, #74227, #124130, #207411, #190091, #59030, #125188, #191149, #177059, #143532, #80627, #61170, #93696, #129463, #176005, #145670, #44945, #195447, #127331, #43879, #161889, #111053, #160810, #46009, #108923, #60099, #28676, #211667, #94763, #109993, #193300, #144599, #210614, #12401, #62241, #78482, #96901, #209528, #27597, #13476, #113194, #159738, #179199, #11336, #192216, #142456, #77417, #126257, #128400, #194367, #146719, #112130, #158676, #95832, #178133, #196507, #29748, #174945, #92635, #79552, #30823, #162952, #10273, #14530, #63303, #47076, #212735, #64372, #130518, #26527, #76349, #208464, #116373, #32935, #65404, #36114, #85949, #115318, #18791, #84874, #16657, #33990, #181308, #150963, #100065, #388, #166128, #2528, #51318, #68603, #134726, #182361, #50253, #83802, #17714, #132601, #213781, #1463, #99009, #165065, #183440, #164018, #149895, #200732, #101115, #3592, #67528, #135776, #117445, #97960, #152024, #69669, #131551, #133671, #199675, #82743, #35044, #167202, #48149, #15592, #19864, #81678, #147765, #148816, #52383, #118511, #114262, #184495, #66460, #102197, #168263, #180259, #197553, #198607, #31883, #49197, #38264, #155221 ),
 ( #105426, #87009, #23051, #5723, #6802, #171463, #169330, #153080, #186638, #206084, #119579, #37192, #138986, #173632, #170385, #24128, #73967, #185563, #89169, #103268, #54515, #53441, #203933, #88083, #72878, #205007, #140062, #90230, #156295, #7879, #157365, #55581, #21973, #25203, #154156, #104341, #57718, #120659, #123877, #137913, #189842, #71802, #136842, #40414, #121736, #39330, #56654, #201799, #4657, #187702, #41489, #122817, #202867, #188775, #106517, #172543, #107601, #91308, #8959, #75034, #20914, #70729, #174695, #191958, #158422, #76097, #44692, #178954, #125999, #190898, #128149, #110800, #14274, #142200, #141148, #124935, #209272, #211419, #63051, #42562, #129216, #11083, #10021, #160551, #208215, #195192, #79303, #60917, #58781, #127076, #43625, #59847, #46828, #109740, #143281, #29494, #175751, #92386, #145419, #27342, #93444, #108664, #26269, #159483, #112941, #30568, #207158, #194109, #77159, #193038, #176803, #28420, #94513, #111877, #12159, #78230, #144352, #96648, #61993, #210354, #45758, #177881, #95586, #161635, #13229, #162702, #99818, #49999, #47904, #31631, #65159, #84624, #212482, #130268, #17469, #52133, #48946, #117191, #166958, #64125, #116122, #196257, #147515, #146465, #82487, #181062, #198359, #83553, #18548, #183191, #34797, #100871, #35872, #148574, #115066, #118261, #32680, #131315, #150716, #213536, #2276, #16407, #68352, #98759, #15344, #133418, #143, #132356, #149635, #80369, #97708, #66209, #134485, #182110, #81436, #164815, #33739, #165883, #1216, #67279, #199424, #200487, #51068, #197307, #184245, #101947, #168013, #114014, #180009, #163766, #204747, #22798, #56398, #40152, #153904, #21722, #55331, #203683, #104088, #185312, #187453, #70479, #86761, #154967, #135525, #121482, #172287, #72630, #189588, #5474, #107341, #88913, #69418, #57464, #41234, #103017, #39081, #71554, #202618, #6552, #137662, #123624, #201549, #205832, #53195, #119326, #136594, #138729, #105166, #19617, #122559, #54268, #171205, #188520, #87833, #36934, #120404, #170137, #106265, #186380, #23875 ) ),
 .UNSPECIFIED., .F., .F., .T. ) 
 B_SPLINE_SURFACE_WITH_KNOTS ( ( 2, 2 ),
 ( 3, 2, 2, 2, 2, 2, 2, 2, 2, 2, 2, 2, 2, 2, 2, 2, 2, 2, 2, 2, 2, 2, 2, 2, 2, 2, 2, 2, 2, 2, 2, 2, 2, 2, 2, 2, 2, 2, 2, 2, 2, 2, 2, 2, 2, 2, 2, 2, 2, 2, 2, 2, 2, 2, 2, 2, 2, 2, 2, 2, 2, 2, 2, 2, 2, 2, 2, 2, 2, 2, 2, 2, 2, 2, 2, 2, 2, 2, 2, 2, 2, 2, 2, 2, 2, 2, 2, 2, 2, 2, 2, 2, 2, 2, 2, 2, 2, 2, 2, 2, 2, 2, 2, 2, 2, 2, 2, 2, 2, 2, 2, 2, 2, 2, 2, 2, 2, 2, 2, 2, 3 ),
 ( 0.000000000000000000, 1.000000000000000000 ),
 ( 0.000000000000000000, 0.008333333333333333218, 0.01666666666666666644, 0.02500000000000000139, 0.03333333333333333287, 0.04166666666666666435, 0.05000000000000000278, 0.05833333333333333426, 0.06666666666666666574, 0.07499999999999999722, 0.08333333333333332871, 0.09166666666666666019, 0.1000000000000000056, 0.1083333333333333370, 0.1166666666666666685, 0.1250000000000000000, 0.1333333333333333315, 0.1416666666666666630, 0.1499999999999999944, 0.1583333333333333259, 0.1666666666666666574, 0.1749999999999999889, 0.1833333333333333204, 0.1916666666666666796, 0.2000000000000000111, 0.2083333333333333426, 0.2166666666666666741, 0.2250000000000000056, 0.2333333333333333370, 0.2416666666666666685, 0.2500000000000000000, 0.2583333333333333592, 0.2666666666666666630, 0.2750000000000000222, 0.2833333333333333259, 0.2916666666666666852, 0.2999999999999999889, 0.3083333333333333481, 0.3166666666666666519, 0.3250000000000000111, 0.3333333333333333148, 0.3416666666666666741, 0.3499999999999999778, 0.3583333333333333370, 0.3666666666666666408, 0.3750000000000000000, 0.3833333333333333592, 0.3916666666666666630, 0.4000000000000000222, 0.4083333333333333259, 0.4166666666666666852, 0.4249999999999999889, 0.4333333333333333481, 0.4416666666666666519, 0.4500000000000000111, 0.4583333333333333148, 0.4666666666666666741, 0.4749999999999999778, 0.4833333333333333370, 0.4916666666666666408, 0.5000000000000000000, 0.5083333333333333037, 0.5166666666666667185, 0.5250000000000000222, 0.5333333333333333259, 0.5416666666666666297, 0.5500000000000000444, 0.5583333333333333481, 0.5666666666666666519, 0.5749999999999999556, 0.5833333333333333703, 0.5916666666666666741, 0.5999999999999999778, 0.6083333333333332815, 0.6166666666666666963, 0.6250000000000000000, 0.6333333333333333037, 0.6416666666666667185, 0.6500000000000000222, 0.6583333333333333259, 0.6666666666666666297, 0.6750000000000000444, 0.6833333333333333481, 0.6916666666666666519, 0.6999999999999999556, 0.7083333333333333703, 0.7166666666666666741, 0.7249999999999999778, 0.7333333333333332815, 0.7416666666666666963, 0.7500000000000000000, 0.7583333333333333037, 0.7666666666666667185, 0.7750000000000000222, 0.7833333333333333259, 0.7916666666666666297, 0.8000000000000000444, 0.8083333333333333481, 0.8166666666666666519, 0.8249999999999999556, 0.8333333333333333703, 0.8416666666666666741, 0.8499999999999999778, 0.8583333333333332815, 0.8666666666666666963, 0.8750000000000000000, 0.8833333333333333037, 0.8916666666666667185, 0.9000000000000000222, 0.9083333333333333259, 0.9166666666666666297, 0.9250000000000000444, 0.9333333333333333481, 0.9416666666666666519, 0.9499999999999999556, 0.9583333333333333703, 0.9666666666666666741, 0.9749999999999999778, 0.9833333333333332815, 0.9916666666666666963, 1.000000000000000000 ),
 .UNSPECIFIED. ) 
 GEOMETRIC_REPRESENTATION_ITEM ( )  RATIONAL_B_SPLINE_SURFACE ( (
 ( 1.000000000000000000, 0.8660254037844387076, 1.000000000000000000, 0.8660254037844387076, 1.000000000000000000, 0.8660254037844387076, 1.000000000000000000, 0.8660254037844387076, 1.000000000000000000, 0.8660254037844387076, 1.000000000000000000, 0.8660254037844387076, 1.000000000000000000, 0.8660254037844387076, 1.000000000000000000, 0.8660254037844387076, 1.000000000000000000, 0.8660254037844387076, 1.000000000000000000, 0.8660254037844387076, 1.000000000000000000, 0.8660254037844387076, 1.000000000000000000, 0.8660254037844387076, 1.000000000000000000, 0.8660254037844387076, 1.000000000000000000, 0.8660254037844387076, 1.000000000000000000, 0.8660254037844387076, 1.000000000000000000, 0.8660254037844387076, 1.000000000000000000, 0.8660254037844387076, 1.000000000000000000, 0.8660254037844387076, 1.000000000000000000, 0.8660254037844387076, 1.000000000000000000, 0.8660254037844387076, 1.000000000000000000, 0.8660254037844387076, 1.000000000000000000, 0.8660254037844387076, 1.000000000000000000, 0.8660254037844387076, 1.000000000000000000, 0.8660254037844387076, 1.000000000000000000, 0.8660254037844387076, 1.000000000000000000, 0.8660254037844387076, 1.000000000000000000, 0.8660254037844387076, 1.000000000000000000, 0.8660254037844387076, 1.000000000000000000, 0.8660254037844387076, 1.000000000000000000, 0.8660254037844387076, 1.000000000000000000, 0.8660254037844387076, 1.000000000000000000, 0.8660254037844387076, 1.000000000000000000, 0.8660254037844387076, 1.000000000000000000, 0.8660254037844387076, 1.000000000000000000, 0.8660254037844387076, 1.000000000000000000, 0.8660254037844387076, 1.000000000000000000, 0.8660254037844387076, 1.000000000000000000, 0.8660254037844387076, 1.000000000000000000, 0.8660254037844387076, 1.000000000000000000, 0.8660254037844387076, 1.000000000000000000, 0.8660254037844387076, 1.000000000000000000, 0.8660254037844387076, 1.000000000000000000, 0.8660254037844387076, 1.000000000000000000, 0.8660254037844387076, 1.000000000000000000, 0.8660254037844387076, 1.000000000000000000, 0.8660254037844387076, 1.000000000000000000, 0.8660254037844387076, 1.000000000000000000, 0.8660254037844387076, 1.000000000000000000, 0.8660254037844387076, 1.000000000000000000, 0.8660254037844387076, 1.000000000000000000, 0.8660254037844387076, 1.000000000000000000, 0.8660254037844387076, 1.000000000000000000, 0.8660254037844387076, 1.000000000000000000, 0.8660254037844387076, 1.000000000000000000, 0.8660254037844387076, 1.000000000000000000, 0.8660254037844387076, 1.000000000000000000, 0.8660254037844387076, 1.000000000000000000, 0.8660254037844387076, 1.000000000000000000, 0.8660254037844387076, 1.000000000000000000, 0.8660254037844387076, 1.000000000000000000, 0.8660254037844387076, 1.000000000000000000, 0.8660254037844387076, 1.000000000000000000, 0.8660254037844387076, 1.000000000000000000, 0.8660254037844387076, 1.000000000000000000, 0.8660254037844387076, 1.000000000000000000, 0.8660254037844387076, 1.000000000000000000, 0.8660254037844387076, 1.000000000000000000, 0.8660254037844387076, 1.000000000000000000, 0.8660254037844387076, 1.000000000000000000, 0.8660254037844387076, 1.000000000000000000, 0.8660254037844387076, 1.000000000000000000, 0.8660254037844387076, 1.000000000000000000, 0.8660254037844387076, 1.000000000000000000, 0.8660254037844387076, 1.000000000000000000, 0.8660254037844387076, 1.000000000000000000, 0.8660254037844387076, 1.000000000000000000, 0.8660254037844387076, 1.000000000000000000, 0.8660254037844387076, 1.000000000000000000, 0.8660254037844387076, 1.000000000000000000, 0.8660254037844387076, 1.000000000000000000, 0.8660254037844387076, 1.000000000000000000, 0.8660254037844387076, 1.000000000000000000, 0.8660254037844387076, 1.000000000000000000, 0.8660254037844387076, 1.000000000000000000, 0.8660254037844387076, 1.000000000000000000, 0.8660254037844387076, 1.000000000000000000, 0.8660254037844387076, 1.000000000000000000, 0.8660254037844387076, 1.000000000000000000, 0.8660254037844387076, 1.000000000000000000, 0.8660254037844387076, 1.000000000000000000, 0.8660254037844387076, 1.000000000000000000, 0.8660254037844387076, 1.000000000000000000, 0.8660254037844387076, 1.000000000000000000, 0.8660254037844387076, 1.000000000000000000, 0.8660254037844387076, 1.000000000000000000, 0.8660254037844387076, 1.000000000000000000, 0.8660254037844387076, 1.000000000000000000, 0.8660254037844387076, 1.000000000000000000, 0.8660254037844387076, 1.000000000000000000, 0.8660254037844387076, 1.000000000000000000, 0.8660254037844387076, 1.000000000000000000, 0.8660254037844387076, 1.000000000000000000, 0.8660254037844387076, 1.000000000000000000, 0.8660254037844387076, 1.000000000000000000, 0.8660254037844387076, 1.000000000000000000, 0.8660254037844387076, 1.000000000000000000, 0.8660254037844387076, 1.000000000000000000, 0.8660254037844387076, 1.000000000000000000, 0.8660254037844387076, 1.000000000000000000, 0.8660254037844387076, 1.000000000000000000, 0.8660254037844387076, 1.000000000000000000, 0.8660254037844387076, 1.000000000000000000, 0.8660254037844387076, 1.000000000000000000, 0.8660254037844387076, 1.000000000000000000, 0.8660254037844387076, 1.000000000000000000, 0.8660254037844387076, 1.000000000000000000, 0.8660254037844387076, 1.000000000000000000, 0.8660254037844387076, 1.000000000000000000, 0.8660254037844387076, 1.000000000000000000, 0.8660254037844387076, 1.000000000000000000),
 ( 1.000000000000000000, 0.8660254037844387076, 1.000000000000000000, 0.8660254037844387076, 1.000000000000000000, 0.8660254037844387076, 1.000000000000000000, 0.8660254037844387076, 1.000000000000000000, 0.8660254037844387076, 1.000000000000000000, 0.8660254037844387076, 1.000000000000000000, 0.8660254037844387076, 1.000000000000000000, 0.8660254037844387076, 1.000000000000000000, 0.8660254037844387076, 1.000000000000000000, 0.8660254037844387076, 1.000000000000000000, 0.8660254037844387076, 1.000000000000000000, 0.8660254037844387076, 1.000000000000000000, 0.8660254037844387076, 1.000000000000000000, 0.8660254037844387076, 1.000000000000000000, 0.8660254037844387076, 1.000000000000000000, 0.8660254037844387076, 1.000000000000000000, 0.8660254037844387076, 1.000000000000000000, 0.8660254037844387076, 1.000000000000000000, 0.8660254037844387076, 1.000000000000000000, 0.8660254037844387076, 1.000000000000000000, 0.8660254037844387076, 1.000000000000000000, 0.8660254037844387076, 1.000000000000000000, 0.8660254037844387076, 1.000000000000000000, 0.8660254037844387076, 1.000000000000000000, 0.8660254037844387076, 1.000000000000000000, 0.8660254037844387076, 1.000000000000000000, 0.8660254037844387076, 1.000000000000000000, 0.8660254037844387076, 1.000000000000000000, 0.8660254037844387076, 1.000000000000000000, 0.8660254037844387076, 1.000000000000000000, 0.8660254037844387076, 1.000000000000000000, 0.8660254037844387076, 1.000000000000000000, 0.8660254037844387076, 1.000000000000000000, 0.8660254037844387076, 1.000000000000000000, 0.8660254037844387076, 1.000000000000000000, 0.8660254037844387076, 1.000000000000000000, 0.8660254037844387076, 1.000000000000000000, 0.8660254037844387076, 1.000000000000000000, 0.8660254037844387076, 1.000000000000000000, 0.8660254037844387076, 1.000000000000000000, 0.8660254037844387076, 1.000000000000000000, 0.8660254037844387076, 1.000000000000000000, 0.8660254037844387076, 1.000000000000000000, 0.8660254037844387076, 1.000000000000000000, 0.8660254037844387076, 1.000000000000000000, 0.8660254037844387076, 1.000000000000000000, 0.8660254037844387076, 1.000000000000000000, 0.8660254037844387076, 1.000000000000000000, 0.8660254037844387076, 1.000000000000000000, 0.8660254037844387076, 1.000000000000000000, 0.8660254037844387076, 1.000000000000000000, 0.8660254037844387076, 1.000000000000000000, 0.8660254037844387076, 1.000000000000000000, 0.8660254037844387076, 1.000000000000000000, 0.8660254037844387076, 1.000000000000000000, 0.8660254037844387076, 1.000000000000000000, 0.8660254037844387076, 1.000000000000000000, 0.8660254037844387076, 1.000000000000000000, 0.8660254037844387076, 1.000000000000000000, 0.8660254037844387076, 1.000000000000000000, 0.8660254037844387076, 1.000000000000000000, 0.8660254037844387076, 1.000000000000000000, 0.8660254037844387076, 1.000000000000000000, 0.8660254037844387076, 1.000000000000000000, 0.8660254037844387076, 1.000000000000000000, 0.8660254037844387076, 1.000000000000000000, 0.8660254037844387076, 1.000000000000000000, 0.8660254037844387076, 1.000000000000000000, 0.8660254037844387076, 1.000000000000000000, 0.8660254037844387076, 1.000000000000000000, 0.8660254037844387076, 1.000000000000000000, 0.8660254037844387076, 1.000000000000000000, 0.8660254037844387076, 1.000000000000000000, 0.8660254037844387076, 1.000000000000000000, 0.8660254037844387076, 1.000000000000000000, 0.8660254037844387076, 1.000000000000000000, 0.8660254037844387076, 1.000000000000000000, 0.8660254037844387076, 1.000000000000000000, 0.8660254037844387076, 1.000000000000000000, 0.8660254037844387076, 1.000000000000000000, 0.8660254037844387076, 1.000000000000000000, 0.8660254037844387076, 1.000000000000000000, 0.8660254037844387076, 1.000000000000000000, 0.8660254037844387076, 1.000000000000000000, 0.8660254037844387076, 1.000000000000000000, 0.8660254037844387076, 1.000000000000000000, 0.8660254037844387076, 1.000000000000000000, 0.8660254037844387076, 1.000000000000000000, 0.8660254037844387076, 1.000000000000000000, 0.8660254037844387076, 1.000000000000000000, 0.8660254037844387076, 1.000000000000000000, 0.8660254037844387076, 1.000000000000000000, 0.8660254037844387076, 1.000000000000000000, 0.8660254037844387076, 1.000000000000000000, 0.8660254037844387076, 1.000000000000000000, 0.8660254037844387076, 1.000000000000000000, 0.8660254037844387076, 1.000000000000000000, 0.8660254037844387076, 1.000000000000000000, 0.8660254037844387076, 1.000000000000000000, 0.8660254037844387076, 1.000000000000000000, 0.8660254037844387076, 1.000000000000000000, 0.8660254037844387076, 1.000000000000000000, 0.8660254037844387076, 1.000000000000000000, 0.8660254037844387076, 1.000000000000000000, 0.8660254037844387076, 1.000000000000000000, 0.8660254037844387076, 1.000000000000000000, 0.8660254037844387076, 1.000000000000000000, 0.8660254037844387076, 1.000000000000000000, 0.8660254037844387076, 1.000000000000000000, 0.8660254037844387076, 1.000000000000000000, 0.8660254037844387076, 1.000000000000000000, 0.8660254037844387076, 1.000000000000000000, 0.8660254037844387076, 1.000000000000000000, 0.8660254037844387076, 1.000000000000000000, 0.8660254037844387076, 1.000000000000000000, 0.8660254037844387076, 1.000000000000000000, 0.8660254037844387076, 1.000000000000000000, 0.8660254037844387076, 1.000000000000000000, 0.8660254037844387076, 1.000000000000000000, 0.8660254037844387076, 1.000000000000000000) ) ) 
 REPRESENTATION_ITEM ( '' )  SURFACE ( )  );
#212048=CARTESIAN_POINT ( 'NONE',  ( -5.536209915801717507, 7.449110030843877794, 1.248366777010925910 ) ) ;
#212055=CARTESIAN_POINT ( 'NONE',  ( 5.448397627845284141, 7.449826213943242514, 1.599625672291268286 ) ) ;
#212063=VECTOR ( 'NONE', #131022, 1000.000000000000114 ) ;
#212065=CARTESIAN_POINT ( 'NONE',  ( 6.536439455564164724, 7.758839131980592718, 1.082531754730549967 ) ) ;
#212075=CARTESIAN_POINT ( 'NONE',  ( -6.482206841109545259, 6.735198534148810090, 0.7216878364870257245 ) ) ;
#212099=CARTESIAN_POINT ( 'NONE',  ( 5.597249624757115960, 5.760645890509660916, 0.6703580308099268414 ) ) ;
#212109=CARTESIAN_POINT ( 'NONE',  ( 4.908934136599710563, 7.884784371745123366, 1.199719254218451159 ) ) ;
#212111=CARTESIAN_POINT ( 'NONE',  ( 6.222266154028957885, 6.224008365980749247, 0.7998128361456352531 ) ) ;
#212122=CARTESIAN_POINT ( 'NONE',  ( -4.065465959251405081, 5.836405933916976707, -1.599625672291271394 ) ) ;
#212125=CARTESIAN_POINT ( 'NONE',  ( 4.814553946184248368, 7.670711132973337065, -1.082531754730548412 ) ) ;
#212141=CARTESIAN_POINT ( 'NONE',  ( -4.638297949650955765, 8.425448351319163365, 0.7216878364870267237 ) ) ;
#212143=CARTESIAN_POINT ( 'NONE',  ( -5.655159470675923394, 5.770309935309573923, 0.000000000000000000 ) ) ;
#212144=CARTESIAN_POINT ( 'NONE',  ( 4.367922837034013739, 7.038290343739964428, 1.270857420505863367 ) ) ;
#212161=CARTESIAN_POINT ( 'NONE',  ( -2.986538976760251263, 6.706322249520737522, -0.7998128361456481317 ) ) ;
#212173=CARTESIAN_POINT ( 'NONE',  ( -3.467853430045390706, 7.267855778353407459, 0.7998128361456352531 ) ) ;
#212179=CARTESIAN_POINT ( 'NONE',  ( -6.116136693540540570, 10.14959355252369910, 0.000000000000000000 ) ) ;
#212182=CARTESIAN_POINT ( 'NONE',  ( -7.598418745816086783, 7.829519723065708092, 0.000000000000000000 ) ) ;
#212183=CARTESIAN_POINT ( 'NONE',  ( -5.672142842012183550, 7.433492730264275927, 1.337035701138490351 ) ) ;
#212191=CARTESIAN_POINT ( 'NONE',  ( -6.168033539574333979, 6.160736982450306876, 0.7998128361456281477 ) ) ;
#212201=ORIENTED_EDGE ( 'NONE', *, *, #23600, .T. ) ;
#212205=CARTESIAN_POINT ( 'NONE',  ( 4.875038752565570732, 7.845239757038595663, -1.199719254218452047 ) ) ;
#212219=CIRCLE ( 'NONE', #181160, 0.07999999999999998779 ) ;
#212227=EDGE_CURVE ( 'NONE', #123208, #128754, #94376, .T. ) ;
#212233=CARTESIAN_POINT ( 'NONE',  ( 6.150558962454855561, 7.204682206732687000, 1.199719254218452047 ) ) ;
#212234=CARTESIAN_POINT ( 'NONE',  ( 5.585032934186686226, 5.480569609498057382, 0.000000000000000000 ) ) ;
#212236=CARTESIAN_POINT ( 'NONE',  ( 4.740510986633625024, 5.559626234941203116, -1.199719254218450271 ) ) ;
#212247=CARTESIAN_POINT ( 'NONE',  ( 4.941988244637107286, 8.095350367992509177, 1.064974588601754757 ) ) ;
#212248=CARTESIAN_POINT ( 'NONE',  ( -4.448483798615272100, 8.203998508444197313, 0.000000000000000000 ) ) ;
#212261=ORIENTED_EDGE ( 'NONE', *, *, #169187, .T. ) ;
#212273=CARTESIAN_POINT ( 'NONE',  ( 5.903649544107831382, 5.852288987739402870, -0.7998128361456481317 ) ) ;
#212275=CARTESIAN_POINT ( 'NONE',  ( 3.088225128862704949, 6.824956093640315302, 0.7998128361456281477 ) ) ;
#212288=APPLICATION_CONTEXT ( 'automotive_design' ) ;
#212295=CARTESIAN_POINT ( 'NONE',  ( -6.084577077482911101, 10.32070003369722144, 0.000000000000000000 ) ) ;
#212305=CARTESIAN_POINT ( 'NONE',  ( 4.342354338126830804, 8.288106837781779035, -0.7998128361456381397 ) ) ;
#212309=CARTESIAN_POINT ( 'NONE',  ( 4.538947565524982686, 8.517465603079630299, 0.000000000000000000 ) ) ;
#212319=CARTESIAN_POINT ( 'NONE',  ( 4.614363445337835934, 8.349151705029461468, -0.2795175495247017583 ) ) ;
#212334=CARTESIAN_POINT ( 'NONE',  ( -6.100232733750003078, 7.025055339219893114, 0.9836300112023097508 ) ) ;
#212341=CARTESIAN_POINT ( 'NONE',  ( -4.444040490229335560, 8.406740681901359480, 0.7998128361456352531 ) ) ;
#212343=CARTESIAN_POINT ( 'NONE',  ( 4.701645408888975197, 8.707279753670952971, 0.000000000000000000 ) ) ;
#212344=LINE ( 'NONE', #82351, #84733 ) ;
#212347=CARTESIAN_POINT ( 'NONE',  ( -6.129167961829681488, 9.308390501180058507, -1.199719254218452047 ) ) ;
#212355=CARTESIAN_POINT ( 'NONE',  ( -0.09935801671627322862, 2.598252772099167274, -1.999773316424213965 ) ) ;
#212372=CARTESIAN_POINT ( 'NONE',  ( 6.861835142292147083, 7.178098218861903135, 0.7216878364870328300 ) ) ;
#212376=CARTESIAN_POINT ( 'NONE',  ( -6.050681693448748177, 10.28115541899069463, 0.7998128361456291469 ) ) ;
#212378=ORIENTED_EDGE ( 'NONE', *, *, #213932, .T. ) ;
#212387=CARTESIAN_POINT ( 'NONE',  ( -3.846355548915592504, 7.490793684076796133, -0.1425745578392398905 ) ) ;
#212388=CARTESIAN_POINT ( 'NONE',  ( -4.990809943606286048, 5.955604701363006015, -1.082531754730549967 ) ) ;
#212390=CARTESIAN_POINT ( 'NONE',  ( 5.027041095616958444, 9.086908054853605421, 0.000000000000000000 ) ) ;
#212393=CYLINDRICAL_SURFACE ( 'NONE', #14158, 1.250000000000000000 ) ;
#212396=CARTESIAN_POINT ( 'NONE',  ( 5.553597010146855695, 5.912075037831448832, 0.6282849591137803502 ) ) ;
#212419=VECTOR ( 'NONE', #184231, 1000.000000000000000 ) ;
#212444=ORIENTED_EDGE ( 'NONE', *, *, #194283, .T. ) ;
#212445=CARTESIAN_POINT ( 'NONE',  ( -4.109529958273628658, 7.808552361378938045, 0.7216878364870338292 ) ) ;
#212451=CARTESIAN_POINT ( 'NONE',  ( -4.111865726694519552, 8.019203457777400956, 0.000000000000000000 ) ) ;
#212457=CARTESIAN_POINT ( 'NONE',  ( 7.614839552730775729, 8.913009562054615031, 1.199719254218452047 ) ) ;
#212458=( BOUNDED_CURVE ( )  B_SPLINE_CURVE ( 2, ( #147518, #65162, #182113, #12162, #30571 ),
 .UNSPECIFIED., .F., .T. ) 
 B_SPLINE_CURVE_WITH_KNOTS ( ( 3, 2, 3 ),
 ( 0.2465812307583980512, 0.2500000000000000000, 0.2539810465305627485 ),
 .UNSPECIFIED. ) 
 CURVE ( )  GEOMETRIC_REPRESENTATION_ITEM ( )  RATIONAL_B_SPLINE_CURVE ( ( 0.9351709383301824996, 0.9450366125562636999, 1.000000000000000000, 0.9359969078262996289, 0.9331456447830145384 ) ) 
 REPRESENTATION_ITEM ( '' )  );
#212459=CARTESIAN_POINT ( 'NONE',  ( -6.303615075710993665, 6.318915441276411471, -0.7998128361456362523 ) ) ;
#212462=CARTESIAN_POINT ( 'NONE',  ( 5.652821694808577213, 7.451312062667313718, 1.328372732707931103 ) ) ;
#212468=CARTESIAN_POINT ( 'NONE',  ( 6.540882763950133238, 6.595727744222092959, 0.000000000000000000 ) ) ;
#212476=CARTESIAN_POINT ( 'NONE',  ( -5.490125858891038213, 5.369844688319787451, -0.7998128361456362523 ) ) ;
#212482=CARTESIAN_POINT ( 'NONE',  ( -4.599959256786493533, 8.588645909551377855, 0.000000000000000000 ) ) ;
#212487=CARTESIAN_POINT ( 'NONE',  ( 5.031484404002867450, 8.884165881396448583, 0.7216878364870317197 ) ) ;
#212489=CARTESIAN_POINT ( 'NONE',  ( -7.227905289416814760, 7.605180057173966723, -0.7216878364870338292 ) ) ;
#212496=CARTESIAN_POINT ( 'NONE',  ( 5.499767588998890844, 6.445425604367387429, 1.199719254218451159 ) ) ;
#212499=CARTESIAN_POINT ( 'NONE',  ( 0.000000000000000000, 8.920000000000001705, 0.000000000000000000 ) ) ;
#212503=CARTESIAN_POINT ( 'NONE',  ( 4.369470645354133431, 8.319742529546998000, 0.7998128361456271485 ) ) ;
#212521=CARTESIAN_POINT ( 'NONE',  ( 4.496171506534161644, 8.048216686630889072, -2.444650791391918876 ) ) ;
#212524=VERTEX_POINT ( 'NONE', #123246 ) ;
#212537=ORIENTED_EDGE ( 'NONE', *, *, #188786, .F. ) ;
#212542=CARTESIAN_POINT ( 'NONE',  ( -5.479780979625591186, 7.495630219063617261, -1.250153324542001343 ) ) ;
#212549=CARTESIAN_POINT ( 'NONE',  ( -4.787437638956939523, 5.718337012605431369, -1.082531754730549967 ) ) ;
#212562=CARTESIAN_POINT ( 'NONE',  ( -3.654804927335652209, 6.421633627603656080, 1.199719254218452935 ) ) ;
#212569=ORIENTED_EDGE ( 'NONE', *, *, #169514, .F. ) ;
#212573=CARTESIAN_POINT ( 'NONE',  ( 4.016958651398847557, 7.908478536599129249, -0.7998128361456362523 ) ) ;
#212576=CARTESIAN_POINT ( 'NONE',  ( 5.004368096775565711, 8.852530189631227842, -0.7216878364870458196 ) ) ;
#212579=ORIENTED_EDGE ( 'NONE', *, *, #16602, .F. ) ;
#212589=CARTESIAN_POINT ( 'NONE',  ( -4.098307573080856692, 8.003385611894792362, 0.7998128361456352531 ) ) ;
#212591=CARTESIAN_POINT ( 'NONE',  ( 5.876533236880477240, 5.820653295974182129, 0.7998128361456352531 ) ) ;
#212601=CARTESIAN_POINT ( 'NONE',  ( -5.966470118465691641, 9.118576350588734059, -1.199719254218452047 ) ) ;
#212602=CARTESIAN_POINT ( 'NONE',  ( 6.180537922983273091, 8.303989891604203422, -1.599625672291281386 ) ) ;
#212604=CARTESIAN_POINT ( 'NONE',  ( 4.370663978927085580, 5.060324124126027279, 7.500000000000000000 ) ) ;
#212607=EDGE_LOOP ( 'NONE', ( #109165, #92920, #193573, #156234 ) ) ;
#212608=CARTESIAN_POINT ( 'NONE',  ( 5.890091390494168522, 5.836471141856793388, 0.000000000000000000 ) ) ;
#212610=CARTESIAN_POINT ( 'NONE',  ( 3.125598124496329360E-16, 2.519999999999999130, 2.000000000000000000 ) ) ;
#212614=CARTESIAN_POINT ( 'NONE',  ( -6.317530715954224441, 6.956803165068716766, 0.9171252194158643345 ) ) ;
#212622=CARTESIAN_POINT ( 'NONE',  ( -7.608060475923978494, 8.905100639113307182, 1.199719254218452047 ) ) ;
#212661=ORIENTED_EDGE ( 'NONE', *, *, #26463, .T. ) ;
#212670=CARTESIAN_POINT ( 'NONE',  ( 3.379725431556547477, 7.165039780116438273, -1.734723475976807094E-15 ) ) ;
#212671=CARTESIAN_POINT ( 'NONE',  ( -3.187575512988701565, 6.732938841879847480, 0.000000000000000000 ) ) ;
#212702=CARTESIAN_POINT ( 'NONE',  ( -4.444040490229335560, 8.406740681901359480, 0.7998128361456352531 ) ) ;
#212704=CARTESIAN_POINT ( 'NONE',  ( 6.834718834620487016, 7.146462526578263308, 0.000000000000000000 ) ) ;
#212709=CARTESIAN_POINT ( 'NONE',  ( -6.629010762438975135, 6.698543742459062145, -0.7998128361456362523 ) ) ;
#212719=CARTESIAN_POINT ( 'NONE',  ( -6.069210040772897052, 7.109775131437022999, -1.199719254218453823 ) ) ;
#212731=CARTESIAN_POINT ( 'NONE',  ( -5.285699784481336927, 7.260012063351913625, 1.599625672291263179 ) ) ;
#212735=CARTESIAN_POINT ( 'NONE',  ( -5.153507786970262572, 9.026526494858359229, -0.7216878364870338292 ) ) ;
#212737=CARTESIAN_POINT ( 'NONE',  ( -6.089020385868856522, 9.157588645938716354, -1.082531754730549967 ) ) ;
#212738=CARTESIAN_POINT ( 'NONE',  ( 6.339319342841494453, 9.553567112360518365, -1.199719254218452047 ) ) ;
#212740=CARTESIAN_POINT ( 'NONE',  ( -7.930593509350902792, 8.217056947189661287, -0.7998128361456362523 ) ) ;
#212760=CARTESIAN_POINT ( 'NONE',  ( -1.849151978240317185, 2.492296139600388205, -2.488099065827154899 ) ) ;
#212778=CARTESIAN_POINT ( 'NONE',  ( 6.132331002353889282, 6.987295666328819266, -0.9434213173033257904 ) ) ;
#212794=CARTESIAN_POINT ( 'NONE',  ( -5.829079699232685208, 5.765290835385048496, 0.000000000000000000 ) ) ;
#212802=DIRECTION ( 'NONE',  ( 0.000000000000000000, 1.000000000000000000, 0.000000000000000000 ) ) ;
#212809=CARTESIAN_POINT ( 'NONE',  ( 3.739016502318667445, 7.584212696005614873, 0.7998128361456271485 ) ) ;
#212811=CARTESIAN_POINT ( 'NONE',  ( 7.530627977747744062, 7.750430493652658015, -0.7998128361456341429 ) ) ;
#212820=CARTESIAN_POINT ( 'NONE',  ( 5.259637247458703868, 5.100941308315409373, 0.000000000000000000 ) ) ;
#212826=CARTESIAN_POINT ( 'NONE',  ( 6.574778147984297938, 6.635272358928617997, -0.7998128361456481317 ) ) ;
#212831=DIRECTION ( 'NONE',  ( 0.000000000000000000, 0.000000000000000000, -1.000000000000000000 ) ) ;
#212840=CARTESIAN_POINT ( 'NONE',  ( -6.292392690518223475, 6.513748691792265788, -0.7216878364870338292 ) ) ;
#212841=CARTESIAN_POINT ( 'NONE',  ( 4.909461021924240498, 7.781436054670031410, 1.082531754730549078 ) ) ;
#212849=VERTEX_POINT ( 'NONE', #195619 ) ;
#212851=CARTESIAN_POINT ( 'NONE',  ( -6.834718835064852449, 8.106831741398025315, 1.082531754730549078 ) ) ;
#212852=CARTESIAN_POINT ( 'NONE',  ( 6.003228155800906407, 10.22579295840155744, 0.000000000000000000 ) ) ;
#212855=CARTESIAN_POINT ( 'NONE',  ( 4.041739190205284160, 7.729463131965888856, 0.000000000000000000 ) ) ;
#212857=ORIENTED_EDGE ( 'NONE', *, *, #73552, .T. ) ;
#212867=LINE ( 'NONE', #178270, #66307 ) ;
#212874=CARTESIAN_POINT ( 'NONE',  ( 4.538947565524982686, 8.517465603079630299, 0.000000000000000000 ) ) ;
#212876=CARTESIAN_POINT ( 'NONE',  ( -5.490125858891038213, 5.369844688319787451, -0.7998128361456362523 ) ) ;
#212880=CIRCLE ( 'NONE', #60756, 0.07999999999999998779 ) ;
#212891=CARTESIAN_POINT ( 'NONE',  ( 6.617788377246179188, 8.814115421577600529, -1.443375672974078761 ) ) ;
#212893=CARTESIAN_POINT ( 'NONE',  ( -6.200875153403786477, 8.327716660428123419, -1.599625672291271394 ) ) ;
#212894=CARTESIAN_POINT ( 'NONE',  ( 4.681308178468477799, 8.683552984847038303, 0.000000000000000000 ) ) ;
#212902=CARTESIAN_POINT ( 'NONE',  ( -6.448838341955544173, 7.552674816150118708, 1.199719254218452047 ) ) ;
#212927=CARTESIAN_POINT ( 'NONE',  ( 5.885648082108200896, 6.039213315313952002, 0.7216878364870328300 ) ) ;
#212933=CARTESIAN_POINT ( 'NONE',  ( 5.112833325684902341, 7.058334528089426740, -1.443375672974078761 ) ) ;
#212945=CARTESIAN_POINT ( 'NONE',  ( -4.769436176957319695, 8.786368983084006601, 0.7998128361456281477 ) ) ;
#212947=CARTESIAN_POINT ( 'NONE',  ( -6.261886844665283114, 8.398896966899865646, 1.599625672291269396 ) ) ;
#212958=CARTESIAN_POINT ( 'NONE',  ( -5.586841817283045408, 8.675676665875643678, 1.199719254218454489 ) ) ;
#212964=CARTESIAN_POINT ( 'NONE',  ( -6.292392690518223475, 6.513748691792265788, -0.7216878364870338292 ) ) ;
#212967=CARTESIAN_POINT ( 'NONE',  ( -6.017840079619296567, 8.114175741012878973, -1.599625672291271394 ) ) ;
#212989=CARTESIAN_POINT ( 'NONE',  ( -5.759181390754928742, 9.941071732514568993, 0.000000000000000000 ) ) ;
#212990=CARTESIAN_POINT ( 'NONE',  ( 3.898851692381625877, 6.706354853490643642, -1.199719254218452047 ) ) ;
#212991=CARTESIAN_POINT ( 'NONE',  ( -6.642568916052639771, 6.714361588341672515, 0.000000000000000000 ) ) ;
#213008=CARTESIAN_POINT ( 'NONE',  ( -5.531188331362556276, 5.962015196429335973, -0.9252058187971325953 ) ) ;
#213016=CARTESIAN_POINT ( 'NONE',  ( -7.279802135894939852, 7.457800344824362604, -0.7998128361456362523 ) ) ;
#213031=B_SPLINE_CURVE_WITH_KNOTS ( 'NONE', 3,
 ( #56720, #139051, #92453, #90294, #27412, #192030 ),
 .UNSPECIFIED., .F., .F.,
 ( 4, 2, 4 ),
 ( 0.000000000000000000, 0.0003072753182893358343, 0.0006145506365786716687 ),
 .UNSPECIFIED. ) ;
#213046=CARTESIAN_POINT ( 'NONE',  ( 5.969332771766739931, 10.18624834369502885, -0.7998128361456481317 ) ) ;
#213058=CARTESIAN_POINT ( 'NONE',  ( 4.759808938472720463, 8.174556087920027636, -0.7576060450402433144 ) ) ;
#213060=CARTESIAN_POINT ( 'NONE',  ( 6.034787771858531435, 10.05468647722803865, 0.000000000000000000 ) ) ;
#213066=CARTESIAN_POINT ( 'NONE',  ( -7.096767062110449942, 7.244259425409119046, -0.7998128361456362523 ) ) ;
#213079=CARTESIAN_POINT ( 'NONE',  ( -4.960304097753355457, 6.880383762169266504, 1.599625672291263179 ) ) ;
#213090=CARTESIAN_POINT ( 'NONE',  ( 5.761288931164342486, 5.686201605971993978, -0.7998128361456481317 ) ) ;
#213111=CARTESIAN_POINT ( 'NONE',  ( -7.774674742793745708, 8.035151719539642912, 0.7998128361456341429 ) ) ;
#213123=CARTESIAN_POINT ( 'NONE',  ( 5.529746549527311039, 7.544733289238903851, -1.599625672291281386 ) ) ;
#213130=CARTESIAN_POINT ( 'NONE',  ( 5.261973015879598314, 5.311592404713873172, -0.7216878364870458196 ) ) ;
#213133=CARTESIAN_POINT ( 'NONE',  ( -4.970620135051034616, 8.062850052469723749, -1.111334424012894617 ) ) ;
#213134=CARTESIAN_POINT ( 'NONE',  ( 6.861835142292143530, 8.138467433163244280, 1.082531754730549967 ) ) ;
#213146=CARTESIAN_POINT ( 'NONE',  ( -5.424670859243583720, 8.382514198209223721, 1.082531754730550855 ) ) ;
#213169=CARTESIAN_POINT ( 'NONE',  ( 4.204437033569277560, 7.919277282557212416, 0.000000000000000000 ) ) ;
#213179=CARTESIAN_POINT ( 'NONE',  ( 5.529746549527311039, 7.544733289238903851, -1.599625672291281386 ) ) ;
#213181=CARTESIAN_POINT ( 'NONE',  ( 6.886615681098613884, 6.999082814228660077, 0.000000000000000000 ) ) ;
#213195=CARTESIAN_POINT ( 'NONE',  ( -3.122120512896910505, 6.864500708346841229, 0.7998128361456352531 ) ) ;
#213198=CARTESIAN_POINT ( 'NONE',  ( 4.651856102820254968, 7.480896982382013505, -1.082531754730548412 ) ) ;
#213210=CARTESIAN_POINT ( 'NONE',  ( -6.319508997745553636, 6.545384383557486530, 0.7216878364870257245 ) ) ;
#213212=CARTESIAN_POINT ( 'NONE',  ( -3.689227196694341515, 7.318199139536432973, -0.7216878364870458196 ) ) ;
#213227=CARTESIAN_POINT ( 'NONE',  ( -3.471769853551161411, 6.208092708188416076, 1.199719254218452935 ) ) ;
#213238=EDGE_CURVE ( 'NONE', #123093, #207594, #72240, .T. ) ;
#213240=CARTESIAN_POINT ( 'NONE',  ( -4.492547798081878874, 6.334668079219206049, 1.599625672291263179 ) ) ;
#213241=CARTESIAN_POINT ( 'NONE',  ( -5.604008600195527379, 5.714843533513091600, -0.1954433161525123697 ) ) ;
#213249=CARTESIAN_POINT ( 'NONE',  ( -7.370792787684826486, 8.628288336167626582, -1.199719254218452047 ) ) ;
#213250=CARTESIAN_POINT ( 'NONE',  ( -4.912146588114373991, 8.123387011080156483, 1.048141424314027237 ) ) ;
#213257=EDGE_CURVE ( 'NONE', #25034, #156131, #120711, .T. ) ;
#213270=CARTESIAN_POINT ( 'NONE',  ( 5.363132282657546490, 8.414682208812571673, -1.199719254218452047 ) ) ;
#213295=CARTESIAN_POINT ( 'NONE',  ( 5.345657705538078730, 9.458627433094950021, 0.7998128361456331437 ) ) ;
#213296=CARTESIAN_POINT ( 'NONE',  ( 6.225128807330042591, 7.291680359087043151, -1.199719254218452047 ) ) ;
#213298=CARTESIAN_POINT ( 'NONE',  ( 2.905190055078214595, 6.611415174225076186, 0.7998128361456271485 ) ) ;
#213302=FACE_OUTER_BOUND ( 'NONE', #62210, .T. ) ;
#213310=CARTESIAN_POINT ( 'NONE',  ( 4.598366155629488361, 8.485928551783258555, 0.1149073004905968448 ) ) ;
#213311=CARTESIAN_POINT ( 'NONE',  ( -6.251718229232857915, 7.426664367927358512, -1.082531754730549967 ) ) ;
#213312=CARTESIAN_POINT ( 'NONE',  ( 4.095971805104285934, 6.832365301713403838, 1.082531754730549078 ) ) ;
#213334=CARTESIAN_POINT ( 'NONE',  ( 4.206772801990143584, 8.129928378955675328, 0.7998128361456271485 ) ) ;
#213336=CARTESIAN_POINT ( 'NONE',  ( 3.237364818613055473, 6.998952398349030268, -1.734723475976807094E-15 ) ) ;
#213356=CARTESIAN_POINT ( 'NONE',  ( -6.312203035614172286, 9.521931420595302953, -1.199719254218452047 ) ) ;
#213358=ORIENTED_EDGE ( 'NONE', *, *, #130359, .F. ) ;
#213366=CARTESIAN_POINT ( 'NONE',  ( 6.540882763950133238, 6.595727744222092959, 0.000000000000000000 ) ) ;
#213370=CARTESIAN_POINT ( 'NONE',  ( 4.877901405866606588, 8.912911750144889567, 0.7998128361456341429 ) ) ;
#213379=CARTESIAN_POINT ( 'NONE',  ( -1.853667714121317367, 8.957164077253494838, 0.7750000000000013545 ) ) ;
#213380=CARTESIAN_POINT ( 'NONE',  ( 4.794097012578165007, 8.135614534340449566, -0.8214339667521903809 ) ) ;
#213388=DIRECTION ( 'NONE',  ( 1.000000000000000000, 0.000000000000000000, 0.000000000000000000 ) ) ;
#213395=CARTESIAN_POINT ( 'NONE',  ( -6.109845972839394790, 7.018363806889529322, 0.9744278291697535677 ) ) ;
#213398=CARTESIAN_POINT ( 'NONE',  ( 3.933273961740298752, 5.682181936820735579, 1.443375672974058777 ) ) ;
#213404=CARTESIAN_POINT ( 'NONE',  ( -5.769876891067536206, 8.889217585290882795, 1.199719254218454489 ) ) ;
#213406=CARTESIAN_POINT ( 'NONE',  ( 4.850785098639300408, 8.881276058379668825, -0.7998128361456481317 ) ) ;
#213409=CARTESIAN_POINT ( 'NONE',  ( -6.400331034103001748, 9.624747418832267698, 1.199719254218452935 ) ) ;
#213416=CARTESIAN_POINT ( 'NONE',  ( 0.1216811705908979330, 2.536982183874235908, -1.996294991408742003 ) ) ;
#213432=CARTESIAN_POINT ( 'NONE',  ( 6.549997609177859559, 6.814287763561861944, 0.000000000000000000 ) ) ;
#213447=CARTESIAN_POINT ( 'NONE',  ( -4.448483799059637533, 7.243629294661272588, 1.082531754730549967 ) ) ;
#213449=CARTESIAN_POINT ( 'NONE',  ( 4.864343252252968597, 8.897093904262280972, 0.000000000000000000 ) ) ;
#213466=CARTESIAN_POINT ( 'NONE',  ( 7.146556367734764770, 9.431011410480991231, 1.443375672974063439 ) ) ;
#213497=CARTESIAN_POINT ( 'NONE',  ( 4.041212305325117882, 6.872442235258051646, -1.199719254218448494 ) ) ;
#213501=CARTESIAN_POINT ( 'NONE',  ( -3.973948422136968084, 7.650373902552835226, -0.7216878364870458196 ) ) ;
#213509=CARTESIAN_POINT ( 'NONE',  ( -6.445975688654487001, 6.485002823043819475, -0.7998128361456362523 ) ) ;
#213516=CARTESIAN_POINT ( 'NONE',  ( -4.782994330570982555, 8.802186828966616972, 0.000000000000000000 ) ) ;
#213518=CARTESIAN_POINT ( 'NONE',  ( 6.578229047358968629, 6.784305542873760864, 0.2988042929856441488 ) ) ;
#213523=CARTESIAN_POINT ( 'NONE',  ( 5.006703865196457492, 9.063181286029688977, 0.000000000000000000 ) ) ;
#213531=CARTESIAN_POINT ( 'NONE',  ( -3.494969737272722643, 7.299491470118629088, -0.7998128361456481317 ) ) ;
#213536=CARTESIAN_POINT ( 'NONE',  ( -6.017840079619296567, 8.114175741012878973, -1.599625672291271394 ) ) ;
#213540=CARTESIAN_POINT ( 'NONE',  ( 6.495764994278797388, 8.671754808115688107, 1.443375672974063439 ) ) ;
#213542=CARTESIAN_POINT ( 'NONE',  ( -7.404161286394468355, 7.810812053647902431, 0.000000000000000000 ) ) ;
#213548=CARTESIAN_POINT ( 'NONE',  ( 4.692003678781083487, 7.631698837623355658, -1.199719254218450271 ) ) ;
#213589=CARTESIAN_POINT ( 'NONE',  ( -5.250728612101474901, 7.694385777474874288, -1.211319784145984846 ) ) ;
#213606=CARTESIAN_POINT ( 'NONE',  ( -6.064239847062411926, 10.29697326487330500, 0.000000000000000000 ) ) ;
#213608=CARTESIAN_POINT ( 'NONE',  ( 7.472478939787284169, 8.746922180287201698, 1.199719254218452935 ) ) ;
#213616=ORIENTED_EDGE ( 'NONE', *, *, #77330, .F. ) ;
#213617=CARTESIAN_POINT ( 'NONE',  ( 6.052789233858158369, 6.026285292448116948, 0.000000000000000000 ) ) ;
#213620=CARTESIAN_POINT ( 'NONE',  ( 4.855228407025239612, 8.678533884922511987, 0.000000000000000000 ) ) ;
#213636=CARTESIAN_POINT ( 'NONE',  ( -5.984998465789844069, 5.947196063035064206, 0.7998128361456281477 ) ) ;
#213637=EDGE_CURVE ( 'NONE', #41470, #53161, #127709, .T. ) ;
#213638=CARTESIAN_POINT ( 'NONE',  ( 4.390861645979372341, 6.216034235099629157, -1.599625672291269396 ) ) ;
#213645=ORIENTED_EDGE ( 'NONE', *, *, #167257, .F. ) ;
#213647=CARTESIAN_POINT ( 'NONE',  ( -4.679499295372141709, 5.488445928469455559, 1.199719254218452935 ) ) ;
#213648=CARTESIAN_POINT ( 'NONE',  ( 5.481239241674765950, 9.616805891921051952, -0.7998128361456481317 ) ) ;
#213654=CARTESIAN_POINT ( 'NONE',  ( 4.472210567661338843, 6.310941310395290493, 1.599625672291261402 ) ) ;
#213661=CARTESIAN_POINT ( 'NONE',  ( -5.922807744518227224, 7.239652023730190677, 1.252291340712426981 ) ) ;
#213670=CARTESIAN_POINT ( 'NONE',  ( -4.963693635934603776, 4.963599794778024155, 0.000000000000000000 ) ) ;
#213671=CARTESIAN_POINT ( 'NONE',  ( -6.071018923869249129, 10.30488218781460574, 0.7998128361456291469 ) ) ;
#213681=CARTESIAN_POINT ( 'NONE',  ( -4.370663978927098015, 5.060324124126027279, 1.009771797811723326 ) ) ;
#213720=CARTESIAN_POINT ( 'NONE',  ( 3.067887898442204442, 6.801229324816399746, 0.7998128361456271485 ) ) ;
#213722=CARTESIAN_POINT ( 'NONE',  ( -3.363831509966360489, 6.938570838353784076, -0.7216878364870458196 ) ) ;
#213748=VERTEX_POINT ( 'NONE', #82389 ) ;
#213749=CARTESIAN_POINT ( 'NONE',  ( -5.794130544993808307, 7.853181283949808744, 1.599625672291263179 ) ) ;
#213752=CARTESIAN_POINT ( 'NONE',  ( 5.356880090730857802, 8.303424968277756335, 1.082531754730548412 ) ) ;
#213757=CARTESIAN_POINT ( 'NONE',  ( -5.712781623311813384, 7.758274208654143855, -1.599625672291271394 ) ) ;
#213761=DIRECTION ( 'NONE',  ( 0.000000000000000000, 0.000000000000000000, -1.000000000000000000 ) ) ;
#213767=CARTESIAN_POINT ( 'NONE',  ( -5.098748287191073203, 8.106234214101666780, 1.199719254218452935 ) ) ;
#213778=CARTESIAN_POINT ( 'NONE',  ( -6.296835998904160014, 6.311006518335105397, 0.000000000000000000 ) ) ;
#213781=CARTESIAN_POINT ( 'NONE',  ( -7.458393901293492334, 7.874083437696761223, 0.7216878364870317197 ) ) ;
#213783=CARTESIAN_POINT ( 'NONE',  ( -6.251718229232846369, 9.347402796530044355, -1.082531754730549967 ) ) ;
#213784=CARTESIAN_POINT ( 'NONE',  ( 7.862802741282558294, 8.137967717776607657, 0.000000000000000000 ) ) ;
#213785=CARTESIAN_POINT ( 'NONE',  ( -4.136646265500964148, 6.879818838842817641, -1.082531754730551743 ) ) ;
#213805=CARTESIAN_POINT ( 'NONE',  ( 6.599791786788117953, 6.770233575417231364, 0.1470628079319712123 ) ) ;
#213826=ADVANCED_FACE ( 'NONE', ( #80268 ), #210255, .F. ) ;
#213828=CARTESIAN_POINT ( 'NONE',  ( 5.631620320865258655, 7.357208097040313532, -1.234165276361798735 ) ) ;
#213841=CARTESIAN_POINT ( 'NONE',  ( 6.607619761813720238, 8.802252036906432764, 1.599625672291268286 ) ) ;
#213845=CARTESIAN_POINT ( 'NONE',  ( -5.978219388983010418, 5.939287140093762574, -0.7998128361456362523 ) ) ;
#213858=CARTESIAN_POINT ( 'NONE',  ( 3.874598038455354665, 7.742391154831717692, -0.7998128361456362523 ) ) ;
#213860=CARTESIAN_POINT ( 'NONE',  ( 7.205232291019763480, 7.370802192470005565, -0.7998128361456341429 ) ) ;
#213865=CARTESIAN_POINT ( 'NONE',  ( -5.248414861821563804, 9.137251415518218067, 0.7216878364870267237 ) ) ;
#213873=CARTESIAN_POINT ( 'NONE',  ( 6.933015448541703485, 9.181880338089085214, 1.599625672291268286 ) ) ;
#213879=CARTESIAN_POINT ( 'NONE',  ( 5.608757509019036469, 5.629766575900002401, 2.420000000000000373 ) ) ;
#213885=CARTESIAN_POINT ( 'NONE',  ( -6.943184063974186415, 7.273005294157565359, -0.7216878364870338292 ) ) ;
#213887=CARTESIAN_POINT ( 'NONE',  ( 4.231553341240963384, 7.950912974840849579, -0.7216878364870357165 ) ) ;
#213898=CARTESIAN_POINT ( 'NONE',  ( -6.699137298928187434, 8.909022496873262753, 1.443375672974064550 ) ) ;
#213899=CARTESIAN_POINT ( 'NONE',  ( 1.833030277982334422, 2.525853874188491055, -2.500000000000000444 ) ) ;
#213903=CARTESIAN_POINT ( 'NONE',  ( 3.716343503477301802, 7.349834830783237294, -1.734723475976807094E-15 ) ) ;
#213918=DIRECTION ( 'NONE',  ( -1.000000000000000000, 0.000000000000000000, 0.000000000000000000 ) ) ;
#213921=CARTESIAN_POINT ( 'NONE',  ( -4.736594563127865420, 6.619389305106191834, -1.599625672291271394 ) ) ;
#213932=EDGE_CURVE ( 'NONE', #71711, #34262, #52905, .T. ) ;
#213933=CARTESIAN_POINT ( 'NONE',  ( 3.203469434578891661, 6.959407783642502565, -0.7998128361456362523 ) ) ;
#213936=CARTESIAN_POINT ( 'NONE',  ( 6.703580607314123085, 6.785541894813420072, 0.000000000000000000 ) ) ;
#213944=CARTESIAN_POINT ( 'NONE',  ( -5.261446130555064826, 8.296048364692991228, 1.199719254218452935 ) ) ;
#213967=FACE_OUTER_BOUND ( 'NONE', #119925, .T. ) ;
#213970=CARTESIAN_POINT ( 'NONE',  ( 3.418064124421011041, 7.001842221884225559, -0.7216878364870338292 ) ) ;
#213971=VERTEX_POINT ( 'NONE', #194010 ) ;
#213976=CARTESIAN_POINT ( 'NONE',  ( 4.367134876933267407, 8.109091433148536865, 0.000000000000000000 ) ) ;
#213987=CARTESIAN_POINT ( 'NONE',  ( -4.796552484184649856, 8.818004674849227342, -0.7998128361456362523 ) ) ;
#213989=CARTESIAN_POINT ( 'NONE',  ( -7.761116589180078407, 8.019333873657032541, 0.000000000000000000 ) ) ;
#213996=CARTESIAN_POINT ( 'NONE',  ( 3.570880328030153539, 7.341005539872356600, 0.2896471194287209006 ) ) ;
#213997=CARTESIAN_POINT ( 'NONE',  ( 7.309781096423290769, 8.557108029695882578, 1.199719254218452935 ) ) ;
#214003=CARTESIAN_POINT ( 'NONE',  ( -6.912678218121246942, 9.158153569265168770, 1.599625672291269396 ) ) ;
#214009=CARTESIAN_POINT ( 'NONE',  ( -4.977251789992602760, 8.820894498384422633, 0.000000000000000000 ) ) ;
#214013=CARTESIAN_POINT ( 'NONE',  ( -6.394605727500880299, 7.489403432619674561, -1.199719254218452047 ) ) ;
#214032=CARTESIAN_POINT ( 'NONE',  ( -6.583366107887490770, 9.838288338247510367, 1.199719254218452935 ) ) ;
#214033=CARTESIAN_POINT ( 'NONE',  ( 4.248501033035879004, 6.049946853332221153, -1.599625672291273171 ) ) ;
#214034=CARTESIAN_POINT ( 'NONE',  ( -5.498713818794216834, 8.572860667638675380, -1.199719254218452047 ) ) ;
#214056=CARTESIAN_POINT ( 'NONE',  ( -6.084577077482911101, 10.32070003369722144, 0.000000000000000000 ) ) ;
#214082=CARTESIAN_POINT ( 'NONE',  ( 3.627688620108284745, 6.389997935838436227, 1.199719254218452047 ) ) ;
#214095=CARTESIAN_POINT ( 'NONE',  ( 4.600487305768355739, 8.366733224642864286, -0.1591645125929436189 ) ) ;
#214097=CARTESIAN_POINT ( 'NONE',  ( 2.905190055078214595, 6.611415174225076186, 0.7998128361456271485 ) ) ;
#214102=CARTESIAN_POINT ( 'NONE',  ( -7.110325215724114578, 7.260077271291732082, 0.000000000000000000 ) ) ;
#214109=CARTESIAN_POINT ( 'NONE',  ( -7.553300976144787349, 8.945177572657957654, -1.082531754730549967 ) ) ;
#214119=CARTESIAN_POINT ( 'NONE',  ( -4.176793841461789114, 7.030620694084159794, -1.199719254218455378 ) ) ;
#214128=B_SPLINE_CURVE_WITH_KNOTS ( 'NONE', 3,
 ( #83247, #197010, #131018, #100578, #166651, #149332 ),
 .UNSPECIFIED., .F., .F.,
 ( 4, 2, 4 ),
 ( 2.354250779258689971E-08, 0.0004384930979466261560, 0.0008769626533854597882 ),
 .UNSPECIFIED. ) ;
#214129=CARTESIAN_POINT ( 'NONE',  ( 3.901714345682657292, 7.774026846596938434, 0.7998128361456271485 ) ) ;
#214149=ORIENTED_EDGE ( 'NONE', *, *, #102547, .F. ) ;
#214150=CARTESIAN_POINT ( 'NONE',  ( -7.075376061485238566, 9.347967719856493218, 1.599625672291269396 ) ) ;
#214152=CARTESIAN_POINT ( 'NONE',  ( 6.994027139803230320, 9.253060644560830994, -1.599625672291267398 ) ) ;
#214159=CARTESIAN_POINT ( 'NONE',  ( 5.180097208873055692, 8.201141289397330780, -1.199719254218450271 ) ) ;
#214168=CARTESIAN_POINT ( 'NONE',  ( 4.692530564105613422, 7.528350520548263702, -1.082531754730548412 ) ) ;
#214171=CARTESIAN_POINT ( 'NONE',  ( 5.397554552016204710, 9.311247720745345902, 0.7216878364870317197 ) ) ;
#214181=CARTESIAN_POINT ( 'NONE',  ( -6.048345925472225382, 8.149765894507963182, 1.443375672974058777 ) ) ;
#214206=CARTESIAN_POINT ( 'NONE',  ( 5.598800414281360993, 5.751655211587324956, 0.6575274206139459787 ) ) ;
#214217=CARTESIAN_POINT ( 'NONE',  ( 5.554000203453580475, 6.508696987897830688, -1.199719254218452047 ) ) ;
#214219=CARTESIAN_POINT ( 'NONE',  ( 6.561219994370630637, 6.619454513046008515, 0.000000000000000000 ) ) ;
#214221=FACE_OUTER_BOUND ( 'NONE', #6497, .T. ) ;
#214231=CARTESIAN_POINT ( 'NONE',  ( -4.604929450496978660, 5.401447776115099408, -1.199719254218453823 ) ) ;
#214234=CARTESIAN_POINT ( 'NONE',  ( 5.356880090730872013, 6.382686539675070492, 1.082531754730549078 ) ) ;
#214241=CARTESIAN_POINT ( 'NONE',  ( -4.930325137224961907, 5.781076077297750970, -1.199719254218453823 ) ) ;
#214247=CARTESIAN_POINT ( 'NONE',  ( -7.607533591043815768, 8.048079742405473525, 0.000000000000000000 ) ) ;
#214249=CARTESIAN_POINT ( 'NONE',  ( -4.312902262922974295, 8.045820050136510915, 0.7216878364870338292 ) ) ;
#214275=CARTESIAN_POINT ( 'NONE',  ( -3.332271893908731464, 7.109677319527304640, -0.7998128361456481317 ) ) ;
#214276=CARTESIAN_POINT ( 'NONE',  ( -5.602498012743508227, 5.726462300312828546, -0.1687859242097844992 ) ) ;
#214282=CARTESIAN_POINT ( 'NONE',  ( -5.608135385276092677, 5.599224824533728828, 0.4022279080854191391 ) ) ;
#214286=CARTESIAN_POINT ( 'NONE',  ( -5.897079639132071449, 7.258985838325384243, -1.264812401031592204 ) ) ;
#214288=ORIENTED_EDGE ( 'NONE', *, *, #106262, .T. ) ;
#214304=CARTESIAN_POINT ( 'NONE',  ( 5.417364897112183719, 8.477953592343014932, 1.199719254218451159 ) ) ;
#214327=CARTESIAN_POINT ( 'NONE',  ( 5.020262018810099924, 9.078999131912302900, 0.7998128361456331437 ) ) ;
#214328=CARTESIAN_POINT ( 'NONE',  ( 6.723917837734620484, 6.809268663637336516, 0.000000000000000000 ) ) ;
#214330=CARTESIAN_POINT ( 'NONE',  ( 6.378184920586140727, 6.405913593630768510, 0.000000000000000000 ) ) ;
#214342=CARTESIAN_POINT ( 'NONE',  ( 4.648548116941726427, 8.423941524322412278, -0.4686463081053967583 ) ) ;
#214344=CARTESIAN_POINT ( 'NONE',  ( -5.682275777458886346, 7.722684055159061423, 1.443375672974058777 ) ) ;
#214345=CARTESIAN_POINT ( 'NONE',  ( 5.248414862265931902, 5.295774558831261913, 0.000000000000000000 ) ) ;
#214360=AXIS2_PLACEMENT_3D ( 'NONE', #138527, #70282, #139606 ) ;
#214370=CARTESIAN_POINT ( 'NONE',  ( 4.797606254389322089, 6.690569611577942943, 1.599625672291268286 ) ) ;
#214372=CARTESIAN_POINT ( 'NONE',  ( 4.947799714344386146, 4.737130853015369958, -0.7998128361456481317 ) ) ;
#214383=CARTESIAN_POINT ( 'NONE',  ( 4.924072945520472366, 4.709449622720799589, 0.000000000000000000 ) ) ;
#214393=CARTESIAN_POINT ( 'NONE',  ( -5.469769711976988802, 6.852634337065973469, -1.200242106353874627 ) ) ;
#214402=CARTESIAN_POINT ( 'NONE',  ( 4.518610335104485287, 8.493738834255713854, 0.000000000000000000 ) ) ;
#214406=CARTESIAN_POINT ( 'NONE',  ( -6.452141306522730879, 6.789529044577018446, 0.3774816029595753353 ) ) ;
#214407=CARTESIAN_POINT ( 'NONE',  ( 6.333594036239346359, 7.418223126147930557, 1.199719254218453823 ) ) ;
#214410=CARTESIAN_POINT ( 'NONE',  ( -6.231486212180770146, 6.935029357745537304, 0.8357456600066525132 ) ) ;
ENDSEC;
END-ISO-10303-21;
